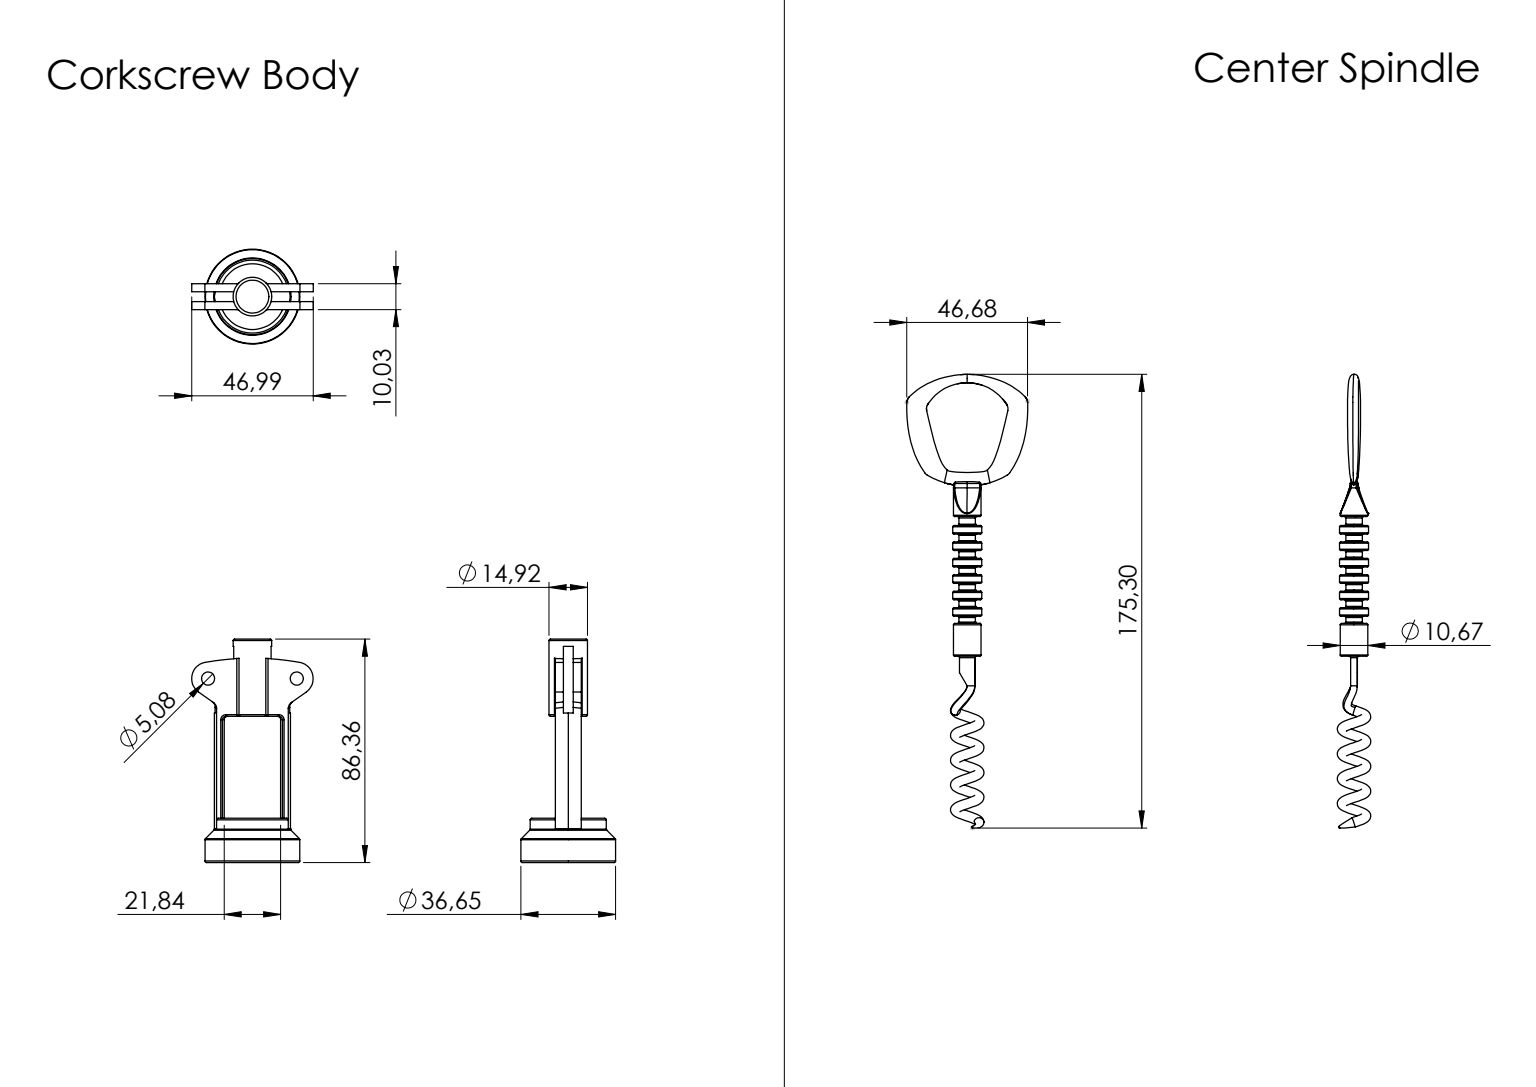
ISO-10303-21;
HEADER;
FILE_DESCRIPTION (('STEP AP214'),
    '1' );
FILE_NAME ('Center Spindle.step',
    '2026-10-06T14:27:08',
    ( '' ),
    ( '' ),
    'SwSTEP 2.0',
    'SolidWorks 2020',
    '' );
FILE_SCHEMA (( 'AUTOMOTIVE_DESIGN' ));
ENDSEC;

DATA;
#1=CARTESIAN_POINT ( 'NONE',  ( -2.902940568641317665, 107.8364052097302306, -4.470325690468441415 ) ) ;
#2=CARTESIAN_POINT ( 'NONE',  ( 4.750191988411978095, 117.8920247151937843, 0.9103219801276267731 ) ) ;
#3=CARTESIAN_POINT ( 'NONE',  ( 3.177488185987922709, -14.13217061847354472, 2.003775387181677026 ) ) ;
#4=CARTESIAN_POINT ( 'NONE',  ( -6.473539731754439863, 155.4519854478747902, -1.179574399179393440 ) ) ;
#5=CARTESIAN_POINT ( 'NONE',  ( -2.402553827781328089, 115.7029513687917017, -1.700315609833690900 ) ) ;
#6=CARTESIAN_POINT ( 'NONE',  ( -3.112628982284441737, 108.2625926757257844, 4.181986096990026880 ) ) ;
#8=CARTESIAN_POINT ( 'NONE',  ( 0.1065646865914872399, 105.8844662015456777, -5.332932678536313809 ) ) ;
#9=CARTESIAN_POINT ( 'NONE',  ( -8.921947645407078298, 154.9128698100208794, -1.713759150786742458 ) ) ;
#10=CARTESIAN_POINT ( 'NONE',  ( 15.73471677570929117, 120.8416612192442159, 0.3144170877234249706 ) ) ;
#11=CARTESIAN_POINT ( 'NONE',  ( -0.02969003158485089208, 157.1787724364823760, 1.485810588193620552 ) ) ;
#12=CARTESIAN_POINT ( 'NONE',  ( -2.946616183681363133, 115.7030909710271231, 1.559688585259455307 ) ) ;
#13=CARTESIAN_POINT ( 'NONE',  ( -5.328734912435950655, 121.3512789622145931, -0.03376412672994712899 ) ) ;
#14=CARTESIAN_POINT ( 'NONE',  ( 3.102408547967445696, -0.5812848888516047863, -3.453265078539196509 ) ) ;
#15=CARTESIAN_POINT ( 'NONE',  ( 22.61937536341548238, 150.3405807453409579, 1.175526429919688587 ) ) ;
#18=CARTESIAN_POINT ( 'NONE',  ( 3.256234316240316229, -15.49904601598017706, 3.966862439782909533 ) ) ;
#19=CARTESIAN_POINT ( 'NONE',  ( -19.06441997122223597, 145.0145856610025987, 1.755053680361626567 ) ) ;
#20=CARTESIAN_POINT ( 'NONE',  ( 0.9007433063219677516, 2.300345052497278608, 0.3717552062572989091 ) ) ;
#21=CARTESIAN_POINT ( 'NONE',  ( 0.003746264460233806812, 116.6481217037470373, -0.1874783927187336496 ) ) ;
#22=CARTESIAN_POINT ( 'NONE',  ( -0.8226642509504364931, 2.890957568680109446, -0.5268263738024351328 ) ) ;
#27=CARTESIAN_POINT ( 'NONE',  ( 4.040061035763102382, 117.6466181296975151, 0.9125624508345167030 ) ) ;
#29=CARTESIAN_POINT ( 'NONE',  ( -1.787077659700294863, 156.4219299504922844, 0.8362026816545217178 ) ) ;
#30=CARTESIAN_POINT ( 'NONE',  ( 3.821280252649200460, -11.76149679029331274, 0.6556923638117722053 ) ) ;
#31=CARTESIAN_POINT ( 'NONE',  ( 12.33128838443251674, 153.5964916033214820, -1.587645809864455471 ) ) ;
#32=CARTESIAN_POINT ( 'NONE',  ( -1.237267194679803950, 118.7146927282448132, -0.6928808259403732572 ) ) ;
#33=CARTESIAN_POINT ( 'NONE',  ( -5.946078212987909062, 28.42590610009758123, 0.3016625663984517924 ) ) ;
#34=CARTESIAN_POINT ( 'NONE',  ( 2.671714809844681238, -14.97371442308345380, 4.574436322856921144 ) ) ;
#35=CARTESIAN_POINT ( 'NONE',  ( -2.623680569203113766, 34.84621527371866989, 1.140749429358363987 ) ) ;
#36=CARTESIAN_POINT ( 'NONE',  ( 14.28939804845276740, 138.9852717218771261, -0.04639197223238045870 ) ) ;
#37=ORIENTED_EDGE ( 'NONE', *, *, #18826, .T. ) ;
#42=CARTESIAN_POINT ( 'NONE',  ( 15.65715779584547462, 120.8241032224722176, 0.2083191676592779373 ) ) ;
#43=CARTESIAN_POINT ( 'NONE',  ( -6.321818188556177276, 120.0717973201777511, 0.2011600071967686865 ) ) ;
#45=CARTESIAN_POINT ( 'NONE',  ( -1.563156853714933625, 118.1287640443500351, 0.8777957133630984732 ) ) ;
#47=CARTESIAN_POINT ( 'NONE',  ( -0.1480340175562135652, 37.01381769933495747, -0.7398847138023396663 ) ) ;
#48=CARTESIAN_POINT ( 'NONE',  ( 20.93418857319365500, 149.0309112320384486, 2.352213276463849034 ) ) ;
#49=CARTESIAN_POINT ( 'NONE',  ( -2.673854242087471356, 19.56896771519852862, 3.769861741755948348 ) ) ;
#50=CARTESIAN_POINT ( 'NONE',  ( -8.093932337251422027, 31.18171294578705854, -2.467657647566553258 ) ) ;
#51=CARTESIAN_POINT ( 'NONE',  ( -2.171567613555696941, 116.7785827647842751, -0.5120155132742859605 ) ) ;
#52=CARTESIAN_POINT ( 'NONE',  ( -2.327868625978157358, 124.9344662015457175, -0.04651635516647353863 ) ) ;
#55=CARTESIAN_POINT ( 'NONE',  ( 3.195898997675873598, 105.1238757837674314, 4.272339236703191823 ) ) ;
#56=CARTESIAN_POINT ( 'NONE',  ( 4.419457123578296454, 17.78516144714274105, -1.360477052881604143 ) ) ;
#59=CARTESIAN_POINT ( 'NONE',  ( 2.461817612451524084, -15.00653475910608492, 4.866425834902347702 ) ) ;
#60=CARTESIAN_POINT ( 'NONE',  ( 1.642663419667585778, 119.5945091202099348, -0.5769171603192788655 ) ) ;
#61=CARTESIAN_POINT ( 'NONE',  ( -19.82178279981189206, 128.7876384977266468, 0.3398896782655025928 ) ) ;
#62=ORIENTED_EDGE ( 'NONE', *, *, #26845, .T. ) ;
#66=DIRECTION ( 'NONE',  ( -4.017660918040594346E-17, 1.000000000000000000, 2.376309959284834438E-19 ) ) ;
#67=CARTESIAN_POINT ( 'NONE',  ( 6.083905389560601229, -14.65912421694762280, 0.09720023197589457153 ) ) ;
#68=CARTESIAN_POINT ( 'NONE',  ( -10.16662615958544258, 120.4647147465577461, 1.171017801134732306 ) ) ;
#70=CARTESIAN_POINT ( 'NONE',  ( 8.033985789952966527, 118.2752802814886053, -0.7207832311977435680 ) ) ;
#71=CARTESIAN_POINT ( 'NONE',  ( -0.9211762648548540433, 10.43857344512876040, -4.529598961101950927 ) ) ;
#74=EDGE_LOOP ( 'NONE', ( #32492, #14883, #24594, #27507 ) ) ;
#76=CARTESIAN_POINT ( 'NONE',  ( 0.4140400251255503261, 124.3520329708341023, 0.07144784443200485891 ) ) ;
#77=B_SPLINE_SURFACE_WITH_KNOTS ( 'NONE', 3, 3, ( 
 ( #14540, #40555, #8162, #21131, #40760, #17945, #30947, #37549, #8372, #19416, #22802, #3464, #6441, #12415, #15798, #3049, #32000, #22177, #35627, #273, #26019, #36045, #39028, #2839, #28807, #25407, #22595, #41823, #16428, #16007, #12820, #12617, #29006, #29432, #18996 ),
 ( #19831, #22385, #25604, #6860, #6034, #10045, #59, #38612, #9418, #35839, #19618, #35410, #16212, #32422, #23017, #6238, #6654, #19208, #2632, #3252, #41605, #32631, #32216, #38814, #42023, #29216, #13247, #25808, #13027, #9628, #26231, #38409, #9220, #39235, #9836 ),
 ( #15591, #28596, #35208, #26870, #26447, #30479, #39450, #29856, #33061, #694, #17063, #40089, #23872, #20042, #16640, #10253, #37096, #7710, #36677, #36467, #7498, #36892, #10469, #3892, #23226, #24086, #36258, #17280, #4316, #20458, #33274, #39878, #16856, #33487, #486 ),
 ( #4103, #13666, #30066, #7286, #903, #7914, #13877, #26658, #32846, #23438, #29648, #27081, #30269, #10884, #33696, #1110, #13459, #39665, #10675, #20248, #7079, #23657, #1323, #14078, #3676, #20672, #4520, #17482, #14280, #27290, #40305, #11098, #21294, #31110, #4939 ),
 ( #27704, #34322, #1947, #34530, #27909, #30900, #11305, #40711, #21497, #37923, #37498, #30685, #33904, #41344, #41127, #8113, #17898, #18520, #8746, #5150, #11507, #24493, #21088, #14906, #34732, #40916, #21708, #12146, #2370, #8323, #18105, #31311, #15115, #5356, #8537 ),
 ( #5563, #1740, #11722, #24709, #1535, #37714, #25138, #24925, #18309, #31526, #14490, #27503, #4733, #2155, #28118, #11933, #15328, #28335, #38142, #20879, #17685, #40511, #24290, #37295, #34112, #14699, #592, #26769, #26338, #33171, #13564, #29110, #29753, #3999, #6755 ),
 ( #10149, #19309, #22701, #16957, #32313, #6542, #9939, #19943, #29326, #23119, #22910, #25915, #35943, #35731, #35517, #19517, #6972, #20148, #10365, #3143, #38923, #29956, #26554, #23336, #13348, #16106, #32525, #19724, #9733, #42128, #382, #7189, #32962, #796, #3788 ),
 ( #32743, #170, #39344, #3356, #13140, #39560, #36155, #13772, #36373, #16323, #3576, #16537, #16748, #29548, #26132, #12924, #39133, #9522, #22489, #6338, #7389, #10573, #17998, #17787, #26978, #36783, #37396, #27595, #40197, #4423, #1220, #39988, #20775, #11404, #7813 ),
 ( #10779, #1425, #40604, #10992, #37191, #30371, #21185, #33374, #36573, #24391, #23760, #4627, #27183, #20350, #14382, #30996, #1636, #30586, #8213, #4206, #17170, #23552, #27391, #40402, #8013, #20984, #5043, #23974, #34005, #34214, #17582, #36992, #17381, #30169, #14179 ),
 ( #11196, #1837, #30786, #1010, #14590, #14801, #33799, #24182, #4835, #13974, #39779, #7599, #20561, #33590, #28228, #28442, #31422, #28011, #12468, #41234, #38459, #34415, #31637, #9277, #11830, #18415, #12037, #2687, #18203, #25028, #2264, #38031, #32055, #8851, #41020 ),
 ( #12253, #15228, #2893, #15439, #5675, #21815, #18633, #34841, #41448, #25246, #2047, #2478, #38249, #21389, #25463, #5248, #24817, #37812, #8637, #9066, #35060, #18843, #15012, #11613, #31204, #27804, #15644, #22032, #5881, #31847, #28649, #5455, #21600, #34628, #19050 ),
 ( #41660, #22235, #35263, #6087, #40812, #24597, #37604, #8431, #10316, #38669, #12878, #16274, #26288, #35685, #29494, #29278, #32271, #123, #29064, #41874, #42084, #13301, #26506, #16697, #25662, #3101, #39511, #20097, #32908, #6494, #335, #7140, #22651, #39296, #19472 ),
 ( #36109, #29702, #19678, #9476, #25867, #13087, #16062, #35469, #6710, #13517, #10103, #33121, #23075, #38873, #9685, #22440, #35899, #32479, #543, #26079, #39087, #3308, #9889, #23285, #22862, #36322, #32694, #15855, #3528, #16488, #28862, #19263, #12673, #6923, #19893 ),
 ( #6292, #3739, #33328, #961, #1591, #33962, #4373, #10730, #7553, #4158, #27134, #17742, #14132, #20937, #24347, #27557, #23711, #36730, #14335, #40357, #30538, #33541, #40147, #39727, #14548, #10526, #13930, #17120, #26925, #30324, #11152, #37147, #30121, #29912, #23496 ),
 ( #23929, #17333, #20513, #36523, #1168, #7969, #21140, #20729, #40564, #4791, #7342, #24139, #11362, #10940, #36944, #7765, #13725, #33753, #4579, #17537, #39938, #1377, #27345, #30742, #37354, #8172, #3950, #16911, #20301, #751, #26719, #18160, #24770, #5413, #9020 ),
 ( #2640, #38416, #21983, #11780, #5627, #25415, #40977, #18585, #37768, #9228, #8592, #18790, #18368, #21556, #5836, #17954, #28603, #12423, #31803, #27758, #1795, #25198, #31375, #34584, #40769, #2219, #15178, #21767, #14966, #28182, #12209, #24985, #34169, #35016, #41187 ),
 ( #31593, #11990, #2004, #24552, #37984, #34794, #15600, #8809, #14758, #4996, #30955, #38203, #21346, #31163, #41613, #11567, #2430, #15391, #28397, #34372, #41402, #37557, #8382, #5205, #27968, #3687, #42033, #12828, #32640, #16435, #6662, #9843, #67, #32429, #13037 ),
 ( #9635, #2847, #26027, #6246, #22810, #32007, #35418, #16648, #15807, #19215, #22603, #3473, #25816, #35848, #35635, #38622, #6449, #32225, #6042, #3057, #19625, #32855, #23025, #28815, #9425, #29655, #26456, #39245, #38824, #29442, #13467, #29013, #281, #19423, #39460 ),
 ( #36055, #39036, #41830, #16014, #3260, #22395, #12624, #13254, #19841, #26238, #22186, #10054, #16220, #29226, #25612, #6868, #495, #35216, #19004, #20465, #36474, #10683, #37103, #26666, #11104, #7506, #27510, #30074, #33282, #1541, #13675, #17692, #7717, #39674, #10477 ),
 ( #30486, #23446, #7294, #7921, #40311, #23664, #17071, #13885, #20255, #33494, #24093, #4324, #27296, #30691, #33911, #911, #26878, #20681, #4526, #36898, #40096, #30277, #17288, #1118, #14087, #23879, #10892, #4111, #39886, #27088, #3901, #20887, #16864, #36684, #33705 ),
 ( #17490, #1329, #14287, #14496, #4739, #10261, #23234, #36269, #7089, #20051, #29864, #33070, #704, #15553, #15125, #21933, #31536, #17905, #18531, #34962, #37723, #34742, #28128, #2380, #41354, #2166, #8120, #11515, #40924, #27711, #30909, #31322, #38152, #21718, #31750 ),
 ( #40720, #21094, #18320, #24500, #12156, #11730, #8547, #37505, #24719, #25148, #14706, #8965, #21506, #40518, #18112, #21301, #2593, #1747, #5785, #37933, #8331, #34330, #15340, #28345, #5158, #11944, #41138, #18740, #31117, #11310, #1954, #24297, #24935, #37303, #34118 ),
 ( #4945, #14914, #27918, #34539, #8756, #5573, #5365, #16167, #6400, #38774, #19370, #9585, #18, #29172, #2799, #15964, #22554, #22135, #26189, #35164, #25562, #28761, #38566, #12777, #35794, #19577, #15756, #12371, #5991, #32804, #3418, #32376, #32169, #3205, #32585 ),
 ( #18954, #19785, #31960, #12984, #25977, #38985, #28962, #35584, #12575, #9794, #38364, #41775, #22973, #9178, #9379, #41978, #22761, #6196, #6606, #25767, #22343, #16385, #35366, #25359, #19165, #29390, #39193, #230, #3005, #13206, #10001, #3635, #36003, #6815, #28555 ),
 ( #41563, #13413, #26831, #7457, #39838, #30229, #4270, #33021, #4062, #10635, #10210, #14240, #23180, #13623, #16814, #26614, #860, #23827, #7666, #3850, #443, #36215, #20836, #33654, #20414, #20207, #33443, #20624, #36429, #29816, #7036, #7874, #20003, #1068, #14036 ),
 ( #13833, #33234, #23614, #26402, #17233, #23397, #17021, #39621, #30020, #27040, #36635, #655, #1282, #40049, #27246, #10427, #10842, #40262, #7248, #36847, #4479, #17439, #30436, #11056, #24041, #37056, #33860, #16599, #29608, #39407, #24452, #1490, #41086, #21453, #24883 ),
 ( #8280, #18477, #30647, #41299, #25092, #31482, #40470, #14447, #37880, #31064, #21250, #11261, #18061, #37456, #34483, #27659, #34280, #8703, #37673, #8912, #5519, #11462, #5109, #14865, #18266, #11677, #14655, #37255, #1902, #5315, #21666, #27868, #27457, #17645, #38097 ),
 ( #31269, #2111, #12103, #34072, #34690, #21047, #21878, #15075, #24247, #2327, #40876, #24664, #4899, #8496, #15287, #28075, #11894, #28292, #4689, #8073, #17854, #30855, #1700, #40670, #12937, #29341, #32120, #38515, #15914, #2541, #22503, #41718, #35320, #2749, #6147 ) ),
 .UNSPECIFIED., .T., .F., .F.,
 ( 4, 2, 2, 2, 1, 2, 2, 2, 2, 2, 2, 1, 2, 2, 4 ),
 ( 4, 1, 1, 1, 1, 1, 1, 1, 1, 1, 1, 1, 1, 1, 1, 1, 1, 1, 1, 1, 1, 1, 1, 1, 1, 1, 1, 1, 1, 1, 1, 1, 4 ),
 ( 0.000000000000000000, 0.06249999999999900080, 0.1249999999999978906, 0.2499999999999956701, 0.2812499999999951150, 0.3749999999999934497, 0.4374999999999933387, 0.5000000000000000000, 0.5624999999999930056, 0.6249999999999928946, 0.7500000000000000000, 0.7812499999999951150, 0.8749999999999963363, 0.9374999999999982236, 1.000000000000000000 ),
 ( 0.000000000000000000, 0.02711375962671787321, 0.05385523109991235263, 0.08027126036152537614, 0.1064096946071439176, 0.1323192412471900226, 0.1580495177521483718, 0.1882118685537063907, 0.2182788543618764954, 0.2483346178351386324, 0.2784631806910429774, 0.3054937156393619513, 0.3327069032348308197, 0.3601597580799023035, 0.3879077415152338837, 0.4160045136367338525, 0.4445017332217630623, 0.4734489055539064517, 0.5028932750457014711, 0.5328797594123376724, 0.5634509204570880003, 0.5946469669818265080, 0.6265057848166851739, 0.6590629893014032792, 0.6923519956652609553, 0.7264041031822485728, 0.7612485893105871426, 0.7986318966073006065, 0.8369441774603861850, 0.8762126957585177900, 0.9164627945539034481, 0.9577180065289634392, 1.000000000000000000 ),
 .UNSPECIFIED. ) ;
#78=CARTESIAN_POINT ( 'NONE',  ( -11.07124803888946296, 123.5714170083676748, 1.086458317614992231 ) ) ;
#80=CARTESIAN_POINT ( 'NONE',  ( 14.75721126660338811, 152.8628051715174365, -1.735400109512246880 ) ) ;
#82=CARTESIAN_POINT ( 'NONE',  ( -13.57054970571782704, 121.9345505566020194, -1.704910367088877221 ) ) ;
#85=CARTESIAN_POINT ( 'NONE',  ( 4.532197386373657544, 118.1209942587670980, -0.4791226501333581411 ) ) ;
#87=CARTESIAN_POINT ( 'NONE',  ( 16.10174665100975488, 146.3760696504137684, -0.5323012926561621061 ) ) ;
#89=CARTESIAN_POINT ( 'NONE',  ( -17.42038752474488561, 148.2779598588913643, -2.227836471057101697 ) ) ;
#90=CARTESIAN_POINT ( 'NONE',  ( 3.162278034637682200, -15.50568859125470134, 4.121945908858189789 ) ) ;
#91=CARTESIAN_POINT ( 'NONE',  ( -3.552207995971087051, 105.1233060067599610, -3.981573230609858793 ) ) ;
#93=B_SPLINE_CURVE_WITH_KNOTS ( 'NONE', 3,
 ( #362, #13328, #570, #10344 ),
 .UNSPECIFIED., .F., .F.,
 ( 4, 4 ),
 ( 0.5010344700412979746, 1.000000000000000000 ),
 .UNSPECIFIED. ) ;
#94=CARTESIAN_POINT ( 'NONE',  ( -4.827457070893626856, 117.7658616683732618, 0.8357213340295019943 ) ) ;
#95=CARTESIAN_POINT ( 'NONE',  ( 7.266810130343707819, 121.1388872696715282, 1.097806971394259312 ) ) ;
#97=AXIS2_PLACEMENT_3D ( 'NONE', #15136, #24944, #28139 ) ;
#98=CARTESIAN_POINT ( 'NONE',  ( 1.523114390242035210, -9.429190846093893796, -8.291516064885865234 ) ) ;
#99=CARTESIAN_POINT ( 'NONE',  ( 4.578033532675482853, 121.1907927009877000, 0.1597499619731680698 ) ) ;
#105=CARTESIAN_POINT ( 'NONE',  ( -2.180832807216472435, 116.2031176879599599, -0.1302529176791268339 ) ) ;
#106=CARTESIAN_POINT ( 'NONE',  ( 13.43845804798103316, 156.9141898299356512, 0.2685323735513602261 ) ) ;
#110=CARTESIAN_POINT ( 'NONE',  ( 5.078986093043053707, 79.34146620154574236, 0.1014902294541244060 ) ) ;
#113=CYLINDRICAL_SURFACE ( 'NONE', #28014, 3.175000000000001155 ) ;
#116=CARTESIAN_POINT ( 'NONE',  ( -23.30518390908433091, 149.0397177335360652, -0.1341373440727923194 ) ) ;
#119=CARTESIAN_POINT ( 'NONE',  ( 6.067968699521611775, 121.4399612899160843, 0.1149339127001053201 ) ) ;
#121=CARTESIAN_POINT ( 'NONE',  ( 4.588798433226582318, 115.7029491485453150, -1.333296534009075662 ) ) ;
#122=CARTESIAN_POINT ( 'NONE',  ( -5.931002064882670233, 121.5392726388429168, -0.1896088198168328631 ) ) ;
#123=CARTESIAN_POINT ( 'NONE',  ( 4.852936394019410571, -14.31369683153947747, 4.236952399839363892 ) ) ;
#124=CARTESIAN_POINT ( 'NONE',  ( -13.60293432442229999, 121.5020190402118203, 1.066732574264078748 ) ) ;
#126=CARTESIAN_POINT ( 'NONE',  ( 16.12231377365572982, 121.3783152868344075, 0.5570369914769761621 ) ) ;
#127=CARTESIAN_POINT ( 'NONE',  ( 9.090272512956175888, 124.2201288364615266, 0.2714231486187235198 ) ) ;
#129=CARTESIAN_POINT ( 'NONE',  ( 0.7643174330569572072, 9.588751494893990923, -0.6113830025413525826 ) ) ;
#130=CARTESIAN_POINT ( 'NONE',  ( -13.61156529719784558, 119.6358206793323404, -0.4233406866235920885 ) ) ;
#131=DIRECTION ( 'NONE',  ( -5.206863593109713661E-17, 1.000000000000000000, -1.077750396879097183E-30 ) ) ;
#132=DIRECTION ( 'NONE',  ( -0.1538570343431813203, -0.9876883405951371042, -0.02827993697916746443 ) ) ;
#133=CARTESIAN_POINT ( 'NONE',  ( 8.672122787176258285, 118.2242029276344510, 0.9375713879804109530 ) ) ;
#134=ORIENTED_EDGE ( 'NONE', *, *, #31655, .T. ) ;
#136=CARTESIAN_POINT ( 'NONE',  ( 14.23594795111937295, 121.8555783441548073, 1.592150851459066319 ) ) ;
#137=CARTESIAN_POINT ( 'NONE',  ( 19.51325853822217127, 141.0981142166620259, -1.725252114789138203 ) ) ;
#138=CARTESIAN_POINT ( 'NONE',  ( -0.1482875670852983607, 5.528424516503947395, -0.9633795868741713564 ) ) ;
#139=CARTESIAN_POINT ( 'NONE',  ( -0.4581589521676752153, 10.92003791307801208, 8.418874016967684781 ) ) ;
#141=CARTESIAN_POINT ( 'NONE',  ( -12.23848595143957141, 156.6574886424908470, -1.779988832801368437 ) ) ;
#142=CARTESIAN_POINT ( 'NONE',  ( 4.767275108742798473, 117.8956358391749717, -0.7413279629693602102 ) ) ;
#144=CARTESIAN_POINT ( 'NONE',  ( 9.138499898145592937, 117.7878261280527425, 0.1826089763859914672 ) ) ;
#145=CARTESIAN_POINT ( 'NONE',  ( 4.403754988258198111, 120.5100497556178567, -0.5130326506441984513 ) ) ;
#146=CARTESIAN_POINT ( 'NONE',  ( -11.83770080265077951, 152.0103986367769551, -0.1887002032782128802 ) ) ;
#148=CARTESIAN_POINT ( 'NONE',  ( -16.28588378367234313, 151.0861551944122141, -2.361334407247334788 ) ) ;
#149=CARTESIAN_POINT ( 'NONE',  ( 5.396943489592968213, -15.24705710738187570, 2.503009974473451749 ) ) ;
#150=CARTESIAN_POINT ( 'NONE',  ( 4.782580095254411745, 118.5931160184169073, 0.9661571381561826488 ) ) ;
#153=CARTESIAN_POINT ( 'NONE',  ( 4.244755607818279763, 119.7015364213435333, 0.9259100998607280308 ) ) ;
#154=DIRECTION ( 'NONE',  ( -0.9998004120163609398, 0.000000000000000000, -0.01997839162482749689 ) ) ;
#157=CARTESIAN_POINT ( 'NONE',  ( -5.575611629172074757, 123.3023672762779910, -0.03632235649590531690 ) ) ;
#158=CARTESIAN_POINT ( 'NONE',  ( 7.184910528696541121, -14.53812136005497280, -4.413989948622978332 ) ) ;
#159=CARTESIAN_POINT ( 'NONE',  ( 9.525206088249063896, 124.2661852542617709, 0.6183897905712308907 ) ) ;
#160=CARTESIAN_POINT ( 'NONE',  ( 4.852593915752285270, 117.2114307359545649, -0.4396237197203589631 ) ) ;
#161=CARTESIAN_POINT ( 'NONE',  ( -4.854186777038641765, 117.7557277303023966, -0.9091791526384296329 ) ) ;
#164=ADVANCED_FACE ( 'NONE', ( #34633 ), #16332, .T. ) ;
#165=CARTESIAN_POINT ( 'NONE',  ( -15.96050253218469983, 121.0385544001969436, -0.3018840724360822847 ) ) ;
#167=CARTESIAN_POINT ( 'NONE',  ( 8.259156552716179434, 120.4369397177006960, -1.103309705185253842 ) ) ;
#168=CARTESIAN_POINT ( 'NONE',  ( 23.29144772315967771, 149.3526176766912101, 0.4654185560736371352 ) ) ;
#169=CARTESIAN_POINT ( 'NONE',  ( -9.418980095613695980, 123.9587481073520223, -0.7032982658115916053 ) ) ;
#170=CARTESIAN_POINT ( 'NONE',  ( 2.004955844419833877, -15.09631637516548075, 5.820374350103214134 ) ) ;
#172=CARTESIAN_POINT ( 'NONE',  ( 20.51686376604209983, 129.1072961674477710, 0.4099757654675942331 ) ) ;
#173=ORIENTED_EDGE ( 'NONE', *, *, #9182, .T. ) ;
#174=CARTESIAN_POINT ( 'NONE',  ( -0.9211762648548540433, 10.43857344512876040, -4.529598961101950927 ) ) ;
#175=CARTESIAN_POINT ( 'NONE',  ( -8.216926545874587262, 117.5004104479096583, -0.1641937475849288286 ) ) ;
#176=CARTESIAN_POINT ( 'NONE',  ( -16.86202032626315628, 155.2029898760372646, -0.3369432954968343275 ) ) ;
#178=CARTESIAN_POINT ( 'NONE',  ( -6.120715547033301007, 121.1078720221529466, 0.4856508595550485530 ) ) ;
#180=CARTESIAN_POINT ( 'NONE',  ( 3.087053954869741101, 14.59627045569285286, -3.440871586639639990 ) ) ;
#181=CARTESIAN_POINT ( 'NONE',  ( 21.46783008853678609, 136.6907720476960435, 1.692068800591147282 ) ) ;
#182=CARTESIAN_POINT ( 'NONE',  ( -0.08519874065850288614, 108.5751225745497948, 4.263693374914160117 ) ) ;
#184=CARTESIAN_POINT ( 'NONE',  ( 2.800559387825661606, 158.6924860557018064, -1.442603686385967032 ) ) ;
#185=CARTESIAN_POINT ( 'NONE',  ( 4.506137822554599381, 3.376467715207942533, 1.027655576270160243 ) ) ;
#186=CARTESIAN_POINT ( 'NONE',  ( -14.63850908477053991, 156.0817623197167450, -1.342817726712510318 ) ) ;
#188=CARTESIAN_POINT ( 'NONE',  ( -15.46148294186166439, 147.8441550597069352, 0.1409636975754419985 ) ) ;
#189=CARTESIAN_POINT ( 'NONE',  ( 3.228727248129140026, -15.23899909574484646, 5.612614099740361517 ) ) ;
#190=CARTESIAN_POINT ( 'NONE',  ( -6.615214180512292604E-14, 94.32746620154571815, -2.829521569843129660E-18 ) ) ;
#191=CARTESIAN_POINT ( 'NONE',  ( 2.969447359227861405, -13.80100253337253946, 0.9847735008004718793 ) ) ;
#193=CARTESIAN_POINT ( 'NONE',  ( 2.329084838958874748, 118.9063233352275972, 0.7992829875212342783 ) ) ;
#196=CARTESIAN_POINT ( 'NONE',  ( -22.74464968533201414, 149.4207734315791072, 0.6238039466385616461 ) ) ;
#197=CARTESIAN_POINT ( 'NONE',  ( 23.16228472148464235, 149.2833505036244048, -0.1324855245534189985 ) ) ;
#202=CARTESIAN_POINT ( 'NONE',  ( 2.109804961112711652, -15.28918944155240034, 5.362628413980365494 ) ) ;
#203=ADVANCED_FACE ( 'NONE', ( #18208 ), #14201, .F. ) ;
#205=DIRECTION ( 'NONE',  ( -5.206863593109713661E-17, 1.000000000000000000, -1.077750396879097183E-30 ) ) ;
#206=CARTESIAN_POINT ( 'NONE',  ( -4.535815920756029129, 118.0878757016629521, 0.6031417657034798818 ) ) ;
#209=ORIENTED_EDGE ( 'NONE', *, *, #20675, .T. ) ;
#210=CARTESIAN_POINT ( 'NONE',  ( -0.3650308193387738487, 118.7629491485454025, -1.279690690685891807 ) ) ;
#211=CARTESIAN_POINT ( 'NONE',  ( 6.034264073414651541, 119.2911550975486676, -1.026770045858946823 ) ) ;
#212=CARTESIAN_POINT ( 'NONE',  ( -3.903247448917784190, 109.8183322527596602, -3.677532532511333052 ) ) ;
#213=CARTESIAN_POINT ( 'NONE',  ( 4.607970095737445426, 117.9806936862427449, 0.9111728063042895398 ) ) ;
#215=CARTESIAN_POINT ( 'NONE',  ( -10.17133788503933900, 124.0743415861677903, -1.120692231141950934 ) ) ;
#217=CARTESIAN_POINT ( 'NONE',  ( -2.225528185412928295, 115.7029491485453576, -1.707866438218498040 ) ) ;
#218=CARTESIAN_POINT ( 'NONE',  ( -2.874359970738451509, 107.8415691140158543, 4.365465615796717103 ) ) ;
#219=CARTESIAN_POINT ( 'NONE',  ( -4.791894246051028539, 117.8359990171110780, -0.9363294005345770277 ) ) ;
#220=CARTESIAN_POINT ( 'NONE',  ( 5.257173101725930664, 116.1034411669277375, -1.028648520082846352 ) ) ;
#221=CARTESIAN_POINT ( 'NONE',  ( -10.56433624517455705, 123.7931190674884050, -1.348085882050163331 ) ) ;
#223=CARTESIAN_POINT ( 'NONE',  ( -0.01596947694136538129, 156.4635559983122448, 0.7991779281049289363 ) ) ;
#224=CARTESIAN_POINT ( 'NONE',  ( -2.827941042956166662, 115.7033332087140138, 1.571145331901102171 ) ) ;
#225=CARTESIAN_POINT ( 'NONE',  ( -15.78496548096122076, 146.2362003282640615, -0.2482417383768280028 ) ) ;
#226=CARTESIAN_POINT ( 'NONE',  ( 1.360477052538118681, -3.804838552850991817, 4.419457122809256511 ) ) ;
#227=CARTESIAN_POINT ( 'NONE',  ( 23.03149411880787767, 148.7220611141358404, 1.316198435982438797 ) ) ;
#230=CARTESIAN_POINT ( 'NONE',  ( 3.491209331645790837, -14.97137451562302601, 1.144833103274278230 ) ) ;
#231=CARTESIAN_POINT ( 'NONE',  ( -8.255438862926547827, 156.5149677146980309, 1.736665298733278906 ) ) ;
#232=CARTESIAN_POINT ( 'NONE',  ( 0.5639076275445228381, 13.94848098472073161, -0.7944722417661187475 ) ) ;
#233=CARTESIAN_POINT ( 'NONE',  ( -21.68922513019262510, 151.4054434770023363, -1.149106048033103011 ) ) ;
#235=CARTESIAN_POINT ( 'NONE',  ( 0.6857505489063979720, -9.425274534614802135, -0.6942005185601292094 ) ) ;
#236=ORIENTED_EDGE ( 'NONE', *, *, #38437, .F. ) ;
#238=CARTESIAN_POINT ( 'NONE',  ( 7.588497335288401757, 124.2943531750336490, 0.1606663149101728583 ) ) ;
#240=CARTESIAN_POINT ( 'NONE',  ( -11.01086703061210414, 126.1652090859982707, 0.5547642914263289926 ) ) ;
#241=CARTESIAN_POINT ( 'NONE',  ( 2.933303798676236696, -14.66982100897798524, 5.370674165220748364 ) ) ;
#242=CARTESIAN_POINT ( 'NONE',  ( 4.329049305160035388, 120.0471566133196291, -0.6733469523851639549 ) ) ;
#243=CARTESIAN_POINT ( 'NONE',  ( -16.05419991788312473, 128.5601350900737998, -2.191829208737125612 ) ) ;
#245=CARTESIAN_POINT ( 'NONE',  ( 2.663950356258127705, -13.19741034273377878, 0.1528337951401303463 ) ) ;
#246=CARTESIAN_POINT ( 'NONE',  ( -5.943370056925232348, 31.21256582444267380, 0.1301312493255015745 ) ) ;
#247=CARTESIAN_POINT ( 'NONE',  ( 11.97065782032992587, 130.4318746828361100, 0.03484989721007641927 ) ) ;
#249=CARTESIAN_POINT ( 'NONE',  ( -4.780654621982846741, 111.8765634536314906, 2.439804913899639605 ) ) ;
#251=CIRCLE ( 'NONE', #36280, 5.588000000000006295 ) ;
#254=AXIS2_PLACEMENT_3D ( 'NONE', #10805, #1032, #33194 ) ;
#255=CARTESIAN_POINT ( 'NONE',  ( 3.297133786507668418, 159.4684106755469202, 0.01890815954692008985 ) ) ;
#256=CARTESIAN_POINT ( 'NONE',  ( -6.540839804427584170, 120.6338824379019172, 0.1347920106280767472 ) ) ;
#258=CARTESIAN_POINT ( 'NONE',  ( -1.044188858242598439, 115.6909491485452435, 1.710615210114453166 ) ) ;
#259=CARTESIAN_POINT ( 'NONE',  ( 4.529186081025091681, -11.15152372915077095, -0.9203776863585164669 ) ) ;
#260=CARTESIAN_POINT ( 'NONE',  ( -2.340953058884871485, 34.37024003021338103, 0.7097582906893736832 ) ) ;
#262=CARTESIAN_POINT ( 'NONE',  ( 14.62144676724393300, 123.3142630313093377, 1.799443978378394648 ) ) ;
#263=CARTESIAN_POINT ( 'NONE',  ( -2.394960105286914942, 16.54535949628658997, -3.951836011466995036 ) ) ;
#264=CARTESIAN_POINT ( 'NONE',  ( -4.020893062959163267, -8.947226795047690473, 7.425401991387179379 ) ) ;
#265=CARTESIAN_POINT ( 'NONE',  ( -5.483673445576510375, 117.2147343480241091, -0.8092650553969497063 ) ) ;
#266=CARTESIAN_POINT ( 'NONE',  ( -0.8420595575569044255, 109.5507526474568607, -3.867914470699519658 ) ) ;
#269=CARTESIAN_POINT ( 'NONE',  ( -2.880622083164609215, 104.6144662015456959, 4.502939351893831876 ) ) ;
#270=CARTESIAN_POINT ( 'NONE',  ( 3.979181138743986601, 26.09377549647152961, 2.406711837290479661 ) ) ;
#271=CARTESIAN_POINT ( 'NONE',  ( 2.081416901521091933, -15.50639809317535089, 5.943648939154567934 ) ) ;
#273=CARTESIAN_POINT ( 'NONE',  ( 3.216700609619024931, -14.42020774479446921, 2.887214088933996337 ) ) ;
#274=CARTESIAN_POINT ( 'NONE',  ( 2.327868625978029016, 124.9344662015457175, 0.04651635516647314311 ) ) ;
#275=CARTESIAN_POINT ( 'NONE',  ( -14.42641459765142820, 120.3907653763288579, 0.3011401359519875198 ) ) ;
#276=VERTEX_POINT ( 'NONE', #11409 ) ;
#278=ORIENTED_EDGE ( 'NONE', *, *, #32111, .F. ) ;
#279=CARTESIAN_POINT ( 'NONE',  ( -5.174735437441460917, 115.7029491485453576, 1.071059064073374589 ) ) ;
#280=AXIS2_PLACEMENT_3D ( 'NONE', #23824, #4267, #36844 ) ;
#281=CARTESIAN_POINT ( 'NONE',  ( 5.898825546834660649, -14.84738759216856785, 0.02597052417917125600 ) ) ;
#282=CARTESIAN_POINT ( 'NONE',  ( -13.14453721617490523, 122.4605402651681487, 1.292199650740640138 ) ) ;
#283=CARTESIAN_POINT ( 'NONE',  ( 9.329873057606279829, 118.8811571165754941, -0.8296725728930305355 ) ) ;
#284=CARTESIAN_POINT ( 'NONE',  ( -4.627450822138572839, 2.892058097378844117, -0.1328416527703782657 ) ) ;
#288=CARTESIAN_POINT ( 'NONE',  ( 0.2094794444022589075, 111.5577547982948801, 3.149697633913104866 ) ) ;
#289=CARTESIAN_POINT ( 'NONE',  ( -4.765692302950382597, 117.6625622553268471, 0.9423543906840938789 ) ) ;
#290=CARTESIAN_POINT ( 'NONE',  ( -17.01014995307831867, 147.0740084267719396, 1.247012517048586844 ) ) ;
#291=CARTESIAN_POINT ( 'NONE',  ( 5.111850311340921493, 116.9863990472329931, 0.4425446553583142206 ) ) ;
#292=CARTESIAN_POINT ( 'NONE',  ( 5.080524353911745727, 119.7208665877771665, -0.8394179162009564044 ) ) ;
#293=CARTESIAN_POINT ( 'NONE',  ( 0.02969037535068572500, 158.7301711276701894, -1.485827791648137053 ) ) ;
#297=CARTESIAN_POINT ( 'NONE',  ( 4.483427315476480324, 118.1297255826064401, -0.5360345877169139239 ) ) ;
#298=CARTESIAN_POINT ( 'NONE',  ( 9.732488649496215061, 124.0009531390599591, -0.4956537337270181531 ) ) ;
#300=CARTESIAN_POINT ( 'NONE',  ( -1.368713796474945177, 119.6596719632383383, -0.6021288208518275065 ) ) ;
#301=CARTESIAN_POINT ( 'NONE',  ( 3.819321967970790599, -15.20641387874817418, 0.06971680219106241028 ) ) ;
#303=AXIS2_PLACEMENT_3D ( 'NONE', #10017, #38788, #25577 ) ;
#304=CARTESIAN_POINT ( 'NONE',  ( -4.782196433634765320, 105.1214876792004560, -2.388545300328469345 ) ) ;
#307=CARTESIAN_POINT ( 'NONE',  ( -4.980589814694351247, 117.5315369307823801, 0.7737963060445882668 ) ) ;
#308=CARTESIAN_POINT ( 'NONE',  ( 17.04317705290379692, 148.4623951536435698, 2.145728921095965358 ) ) ;
#309=CARTESIAN_POINT ( 'NONE',  ( -2.803395127021860223, 31.26063551530791074, 0.8708390753670083306 ) ) ;
#312=CARTESIAN_POINT ( 'NONE',  ( 8.369700380136936957, -11.69135346447765933, 0.7700151973242596037 ) ) ;
#313=CARTESIAN_POINT ( 'NONE',  ( 9.115443861533906400, 124.0847320388339625, 0.2671161660598814769 ) ) ;
#315=( BOUNDED_SURFACE ( )  B_SPLINE_SURFACE ( 3, 1, ( 
 ( #22075, #40860 ),
 ( #8688, #31254 ),
 ( #11879, #24648 ),
 ( #15059, #5300 ),
 ( #28059, #24868 ),
 ( #9112, #41495 ),
 ( #34264, #31896 ),
 ( #12300, #21650 ),
 ( #38293, #41069 ),
 ( #37864, #18888 ),
 ( #31468, #35102 ),
 ( #2311, #28277 ),
 ( #8896, #41282 ),
 ( #5720, #18676 ),
 ( #31683, #2733 ),
 ( #28487, #15688 ) ),
 .UNSPECIFIED., .T., .F., .T. ) 
 B_SPLINE_SURFACE_WITH_KNOTS ( ( 4, 1, 1, 1, 1, 1, 2, 1, 1, 1, 1, 1, 4 ),
 ( 2, 2 ),
 ( 0.000000000000000000, 0.02374999999999993783, 0.1365624999999999478, 0.2493749999999999578, 0.3621874999999999956, 0.4749999999999999778, 0.5000000000000000000, 0.5250000000000000222, 0.6378125000000000044, 0.7506249999999999867, 0.8634374999999999689, 0.9762499999999999512, 1.000000000000000000 ),
 ( 0.000000000000000000, 1.000000000000000000 ),
 .UNSPECIFIED. ) 
 GEOMETRIC_REPRESENTATION_ITEM ( )  RATIONAL_B_SPLINE_SURFACE ( (
 ( 1.000000000000000000, 1.000000000000000000),
 ( 1.000000000000000222, 1.000000000000000000),
 ( 0.8208939328743548591, 1.000000000000000000),
 ( 0.5876145654044752087, 1.000000000000000000),
 ( 0.4813067448364888867, 1.000000000000000000),
 ( 0.5852845309810671415, 1.000000000000000000),
 ( 0.8180077452667815496, 1.000000000000000000),
 ( 0.9982788296041308351, 1.000000000000000000),
 ( 0.9982788296041308351, 1.000000000000000000),
 ( 0.8180077452667815496, 1.000000000000000000),
 ( 0.5852845309810672525, 1.000000000000000000),
 ( 0.4813067448364889422, 1.000000000000000000),
 ( 0.5876145654044749866, 1.000000000000000000),
 ( 0.8208939328743545261, 1.000000000000000000),
 ( 1.000000000000000000, 1.000000000000000000),
 ( 1.000000000000000000, 1.000000000000000000) ) ) 
 REPRESENTATION_ITEM ( '' )  SURFACE ( )  );
#317=CARTESIAN_POINT ( 'NONE',  ( 5.564716835327648603, 116.6996553459067485, 0.05384121919325710742 ) ) ;
#320=DIRECTION ( 'NONE',  ( -5.206863593109713661E-17, 1.000000000000000000, -1.077750396879097183E-30 ) ) ;
#321=CARTESIAN_POINT ( 'NONE',  ( -4.855072294470598848, 115.7029491485453718, 1.279409886141107178 ) ) ;
#328=CARTESIAN_POINT ( 'NONE',  ( -6.912985389844515716, 117.2044255678715814, 0.04371034868568312443 ) ) ;
#331=CARTESIAN_POINT ( 'NONE',  ( -6.058547263772821267, 121.4334988323120683, -0.1247128170359407956 ) ) ;
#333=CARTESIAN_POINT ( 'NONE',  ( -5.332922648341591909, 115.7029491485453718, -0.1072025963776009894 ) ) ;
#334=CARTESIAN_POINT ( 'NONE',  ( -15.38115207166226561, 147.8278496344100859, -0.4352178850651138853 ) ) ;
#335=CARTESIAN_POINT ( 'NONE',  ( 5.987854329437395151, -12.83555092537783082, 1.339350064115379935 ) ) ;
#336=CARTESIAN_POINT ( 'NONE',  ( -20.77691070360842929, 149.9184980045912425, 1.462349339025473371 ) ) ;
#337=CARTESIAN_POINT ( 'NONE',  ( 1.325333094648095011, 19.28447512809159292, -4.440015753949128730 ) ) ;
#338=CARTESIAN_POINT ( 'NONE',  ( 23.02690842483876565, 149.8694456586574972, 0.9127416204503947528 ) ) ;
#339=CARTESIAN_POINT ( 'NONE',  ( 2.116771290498892899, -15.66388792789737217, 5.610892275307695520 ) ) ;
#340=CARTESIAN_POINT ( 'NONE',  ( 4.771882511409050842, 118.5266822147775940, -0.8399436299859415200 ) ) ;
#341=CARTESIAN_POINT ( 'NONE',  ( 0.8400667230086624748, -1.857414735510459547, 0.5005776846920441114 ) ) ;
#342=CARTESIAN_POINT ( 'NONE',  ( 0.001640166039734963777, 159.6041700698465036, -0.08208061555506483697 ) ) ;
#343=CARTESIAN_POINT ( 'NONE',  ( -0.1058213901579529159, 105.9761915687834914, 5.295735085524055030 ) ) ;
#345=ORIENTED_EDGE ( 'NONE', *, *, #41321, .T. ) ;
#346=CARTESIAN_POINT ( 'NONE',  ( -5.552382799689717707, 117.0635824090028194, 0.4511715980537314707 ) ) ;
#348=CARTESIAN_POINT ( 'NONE',  ( -7.569905091580626078, 156.0351187175861867, 1.610277000873165276 ) ) ;
#350=CARTESIAN_POINT ( 'NONE',  ( 16.25125256408137986, 125.3309463260932830, 1.843050201054562187 ) ) ;
#351=CARTESIAN_POINT ( 'NONE',  ( 1.119065284002195959, 158.2739225783580537, -1.587016747512054016 ) ) ;
#352=CARTESIAN_POINT ( 'NONE',  ( -0.6988831915142799112, -0.7227331674307564402, 0.6786060147580050828 ) ) ;
#353=CARTESIAN_POINT ( 'NONE',  ( -20.44519586420853585, 150.9797539340098069, -2.100688152434084799 ) ) ;
#354=CARTESIAN_POINT ( 'NONE',  ( 4.677671540821375373, 117.9838357377442293, -0.6916929324824377945 ) ) ;
#357=CARTESIAN_POINT ( 'NONE',  ( 16.46834812293193195, 148.4304801786341272, -1.248264531716813286 ) ) ;
#358=CARTESIAN_POINT ( 'NONE',  ( -0.0005468344959711694646, 156.3034662015456604, 0.02736583427618486872 ) ) ;
#360=CARTESIAN_POINT ( 'NONE',  ( -3.340139884075267851, 119.4525916976722897, -0.8552862985148331765 ) ) ;
#361=CARTESIAN_POINT ( 'NONE',  ( 5.741009826001572947, -15.03722989464144355, 1.207582410354154145 ) ) ;
#362=CARTESIAN_POINT ( 'NONE',  ( -5.332935381406168851, 115.7029491485442634, -0.1065653510733624160 ) ) ;
#366=CARTESIAN_POINT ( 'NONE',  ( -0.03153862713815891450, 157.4657262375360176, 1.578321868909182690 ) ) ;
#368=CARTESIAN_POINT ( 'NONE',  ( 5.011242901787458237, 115.7029491485453008, 1.398755999327908839 ) ) ;
#369=CARTESIAN_POINT ( 'NONE',  ( -2.226623034866326289, 116.5145642697238344, 1.365476420808193536 ) ) ;
#370=CARTESIAN_POINT ( 'NONE',  ( -3.240848860066210868, 23.83156553091082230, 7.781828003744739597 ) ) ;
#371=CARTESIAN_POINT ( 'NONE',  ( 4.491182069977868174, 120.9948550335633115, 0.4087774027959020229 ) ) ;
#372=CARTESIAN_POINT ( 'NONE',  ( 15.41192216945090898, 121.3506620944898060, -0.4643526128083734772 ) ) ;
#376=CARTESIAN_POINT ( 'NONE',  ( -3.302029177305334073, 159.4671159221996959, -0.06598240135525369754 ) ) ;
#379=CARTESIAN_POINT ( 'NONE',  ( -6.605722241764236280, 120.6764655449730981, -1.089203411656264553 ) ) ;
#380=CARTESIAN_POINT ( 'NONE',  ( 2.112156314984550143, -15.50190413873483664, 5.930787297944131176 ) ) ;
#381=CARTESIAN_POINT ( 'NONE',  ( -10.47888833811902920, 153.0637448873655728, -0.6176438153593468705 ) ) ;
#382=CARTESIAN_POINT ( 'NONE',  ( 4.301541689408341362, -12.13840576482722078, 1.420409876116004222 ) ) ;
#383=CARTESIAN_POINT ( 'NONE',  ( -15.08259856265902599, 121.6710330000183546, 0.7362983101480767845 ) ) ;
#384=CARTESIAN_POINT ( 'NONE',  ( -7.784012322544769269, 122.6313477034873074, -0.1555430911242075831 ) ) ;
#385=CARTESIAN_POINT ( 'NONE',  ( 15.19377495473398021, 156.0906695176550443, 0.3258312939631712868 ) ) ;
#387=CARTESIAN_POINT ( 'NONE',  ( -0.2480930319908794535, 10.21371511114847053, -4.635561276548324727 ) ) ;
#388=CARTESIAN_POINT ( 'NONE',  ( -2.732111087507159475, 116.5293111276780849, -0.05459408159141344169 ) ) ;
#389=DIRECTION ( 'NONE',  ( -0.9998004120163608288, 0.000000000000000000, -0.01997839162482747608 ) ) ;
#391=CARTESIAN_POINT ( 'NONE',  ( -5.945396627788727351, 120.3459718913957772, 0.7896226015759897354 ) ) ;
#393=CARTESIAN_POINT ( 'NONE',  ( 2.298459491326434900, 5.325542553220859787, -4.024866414273244430 ) ) ;
#394=CARTESIAN_POINT ( 'NONE',  ( 13.98195098595639152, 120.5923583732999873, 1.177051350580812894 ) ) ;
#395=CARTESIAN_POINT ( 'NONE',  ( -6.580517660824093636E-14, 85.69146620154573668, -4.881702850681514412E-18 ) ) ;
#397=CARTESIAN_POINT ( 'NONE',  ( 3.107221341096611855, 117.9340107969418341, -0.6831876054667451736 ) ) ;
#398=CARTESIAN_POINT ( 'NONE',  ( 4.615940417482057967, 3.801270455692813410, -0.2501868467277520436 ) ) ;
#399=CARTESIAN_POINT ( 'NONE',  ( -3.857972943339743388, 117.0975898859979054, -0.5726864223607189830 ) ) ;
#402=CARTESIAN_POINT ( 'NONE',  ( -15.34424630368622999, 148.0267799683202554, 0.1426181633603112453 ) ) ;
#403=ADVANCED_FACE ( 'NONE', ( #6714 ), #2778, .F. ) ;
#404=CARTESIAN_POINT ( 'NONE',  ( 2.294645149923727701, -15.44887909491890454, 5.922367448919703570 ) ) ;
#407=CARTESIAN_POINT ( 'NONE',  ( -0.4875235816601763972, 105.8261742744559513, -5.318508263945600945 ) ) ;
#409=CARTESIAN_POINT ( 'NONE',  ( 19.37512658372770602, 148.3988719805327037, 2.511650730565585299 ) ) ;
#410=CARTESIAN_POINT ( 'NONE',  ( 3.009276887026298031, 50.42904571186020490, -1.210121013456480377 ) ) ;
#411=CARTESIAN_POINT ( 'NONE',  ( 9.049782359939477772, 124.0675141969884692, 0.1808361888366267212 ) ) ;
#412=CARTESIAN_POINT ( 'NONE',  ( -6.906891541952466795, 117.5897289630162987, 0.4768185843253518463 ) ) ;
#413=CARTESIAN_POINT ( 'NONE',  ( -8.406874004389072397, 27.76653542065474056, -0.1818807619882521764 ) ) ;
#414=CARTESIAN_POINT ( 'NONE',  ( 18.50641704078256566, 154.1703991122031994, -0.1853567545699118246 ) ) ;
#418=CARTESIAN_POINT ( 'NONE',  ( 2.033723713787972009, -15.06201970758669262, 5.669216239185479012 ) ) ;
#421=CARTESIAN_POINT ( 'NONE',  ( -4.380715115686576233, 118.1845394087038272, 0.4311985218286477073 ) ) ;
#426=CARTESIAN_POINT ( 'NONE',  ( 8.373209961036389259, 119.8814485504210126, -1.110484165621906660 ) ) ;
#427=CARTESIAN_POINT ( 'NONE',  ( -7.277551686224490446, 123.0424313102424492, -0.2142739940110133801 ) ) ;
#428=CARTESIAN_POINT ( 'NONE',  ( 4.615868816244335981, 118.0368944136972971, 0.7918170276731736346 ) ) ;
#429=CARTESIAN_POINT ( 'NONE',  ( -15.92638198489195211, 148.2453349897154737, -1.585317681524597733 ) ) ;
#430=CARTESIAN_POINT ( 'NONE',  ( -2.661596506648667759, 115.7033367343655073, -1.688174420981334078 ) ) ;
#432=CARTESIAN_POINT ( 'NONE',  ( 5.069034061154215287, 114.3796182124986984, -1.753882200456532425 ) ) ;
#434=CARTESIAN_POINT ( 'NONE',  ( -13.21686059441255701, 128.5100244389050204, -1.738961528769450426 ) ) ;
#435=CARTESIAN_POINT ( 'NONE',  ( -6.529493367164978770E-14, 72.99146620154573384, -7.899616498973244731E-18 ) ) ;
#436=CARTESIAN_POINT ( 'NONE',  ( -0.02156508032628448243, 159.2730288250082538, 1.079204802879467850 ) ) ;
#438=CARTESIAN_POINT ( 'NONE',  ( 8.107080057029456555, 121.1657703571624012, -0.9663533087782769648 ) ) ;
#439=CARTESIAN_POINT ( 'NONE',  ( -9.093843756948800205, 124.2201256219595251, -0.09191904702568627628 ) ) ;
#440=CARTESIAN_POINT ( 'NONE',  ( 0.4343283552818534288, -9.202337043772711667, -4.603842121470758997 ) ) ;
#441=CARTESIAN_POINT ( 'NONE',  ( 15.72348727998148732, 121.4292885696920621, 0.9291061361373527117 ) ) ;
#443=CARTESIAN_POINT ( 'NONE',  ( 3.393951437975996743, -15.00105261681208901, 2.580228093083809071 ) ) ;
#444=CARTESIAN_POINT ( 'NONE',  ( -19.24794053165973295, 147.9830121424878939, 1.736014841626597693 ) ) ;
#445=CARTESIAN_POINT ( 'NONE',  ( 0.9605196170170531289, 3.153480984720312019, -0.1630338022177024171 ) ) ;
#446=CARTESIAN_POINT ( 'NONE',  ( -15.70934801585154439, 121.2535323456646523, -0.8362899507430229251 ) ) ;
#447=CARTESIAN_POINT ( 'NONE',  ( 0.9581433470387596962, -10.92824219907890360, 0.1848338584972420151 ) ) ;
#448=B_SPLINE_CURVE_WITH_KNOTS ( 'NONE', 3,
 ( #28992, #13011, #471, #26642, #39436, #9405, #45, #10239, #29633, #3877 ),
 .UNSPECIFIED., .F., .F.,
 ( 4, 2, 2, 2, 4 ),
 ( 0.0001363461699588103975, 0.001296643753711174303, 0.002456941337463538263, 0.003617238921215902223, 0.004777536504968266616 ),
 .UNSPECIFIED. ) ;
#450=VERTEX_POINT ( 'NONE', #12678 ) ;
#452=CARTESIAN_POINT ( 'NONE',  ( 7.253313547007579132, 123.0461458356614628, 0.2138788351844319036 ) ) ;
#453=CARTESIAN_POINT ( 'NONE',  ( -9.588254403178179786, 123.8224200044116827, 0.4900104160083063043 ) ) ;
#454=CARTESIAN_POINT ( 'NONE',  ( 3.745401017337624872, -13.88268793655436717, 4.204469449000409753 ) ) ;
#455=CARTESIAN_POINT ( 'NONE',  ( 17.22014391273205547, 144.2986879860016529, -1.480874425454277166 ) ) ;
#456=CARTESIAN_POINT ( 'NONE',  ( -12.70548372655400904, 122.4237789811383550, -1.817438969878694577 ) ) ;
#459=CARTESIAN_POINT ( 'NONE',  ( 3.197553254331486183, -13.99644925588092192, 2.254757065552156714 ) ) ;
#460=CARTESIAN_POINT ( 'NONE',  ( -5.685436017834463840, 31.78209642239458788, 1.206328258593732272 ) ) ;
#461=CARTESIAN_POINT ( 'NONE',  ( 11.88810549871044486, 151.9737369308441544, -0.07145411264644065119 ) ) ;
#462=ORIENTED_EDGE ( 'NONE', *, *, #9429, .T. ) ;
#463=CARTESIAN_POINT ( 'NONE',  ( -3.729000260451577731, 109.6950671057684588, 3.590446461533148170 ) ) ;
#465=CARTESIAN_POINT ( 'NONE',  ( 4.560443946511397506, -11.68866997254031936, 0.6947937310338139216 ) ) ;
#466=VECTOR ( 'NONE', #25714, 1000.000000000000000 ) ;
#469=CARTESIAN_POINT ( 'NONE',  ( 23.10641284836728815, 149.8968678342272653, 0.3080169626343542966 ) ) ;
#470=CARTESIAN_POINT ( 'NONE',  ( -4.503688181905225463, 111.2539628214143903, 2.957939639849824776 ) ) ;
#471=CARTESIAN_POINT ( 'NONE',  ( -3.877963262798508559, 118.0214462806859927, 0.8169714283994556903 ) ) ;
#473=CARTESIAN_POINT ( 'NONE',  ( -2.920903721094229244, 32.16307183204811082, 0.9800304932835676164 ) ) ;
#474=CARTESIAN_POINT ( 'NONE',  ( 6.753855533487119978, 118.7881172115286148, 1.217991184693928863 ) ) ;
#475=CARTESIAN_POINT ( 'NONE',  ( 3.308978306493741250, 24.09187545982852541, -3.235542752117448018 ) ) ;
#476=CARTESIAN_POINT ( 'NONE',  ( -4.294125178196657622, -12.16697637372164564, -7.253078015393731981 ) ) ;
#477=CARTESIAN_POINT ( 'NONE',  ( 5.557917761466073969, 117.8868906345641676, -0.8474712118571966490 ) ) ;
#478=CARTESIAN_POINT ( 'NONE',  ( -0.6699575554302183988, 116.0160817474902331, -1.654834682733560491 ) ) ;
#481=CARTESIAN_POINT ( 'NONE',  ( 0.8028203427309564821, 104.6144662015435216, 5.284712525425792506 ) ) ;
#483=CARTESIAN_POINT ( 'NONE',  ( -4.598301960400187127, 22.30806413504685537, 0.5496829067130363233 ) ) ;
#486=CARTESIAN_POINT ( 'NONE',  ( 2.744913772555794385, -12.89811552070117884, 0.2544447123532062038 ) ) ;
#487=CARTESIAN_POINT ( 'NONE',  ( 3.315449255180855204, 124.9344662015457743, 0.06625056644921985260 ) ) ;
#488=CARTESIAN_POINT ( 'NONE',  ( -19.54046365593634960, 128.7319734376252143, 0.5398260955622252721 ) ) ;
#489=CARTESIAN_POINT ( 'NONE',  ( 4.976458764963934023, 117.4076063131326606, -0.8841951503558329595 ) ) ;
#490=ORIENTED_EDGE ( 'NONE', *, *, #7890, .T. ) ;
#491=CARTESIAN_POINT ( 'NONE',  ( -6.589702033682734540E-14, 87.97746620154572383, -4.338478393988997516E-18 ) ) ;
#494=DIRECTION ( 'NONE',  ( -0.9998004120163608288, 0.000000000000000000, -0.01997839162482749342 ) ) ;
#495=CARTESIAN_POINT ( 'NONE',  ( 4.389818247250405037, -15.68135102926887470, 3.766867903159812681 ) ) ;
#496=CARTESIAN_POINT ( 'NONE',  ( -20.02944843481990844, 148.6304843473828043, 1.700276915703844427 ) ) ;
#497=CARTESIAN_POINT ( 'NONE',  ( 19.32406529451186117, 152.1947311750261065, -1.288948053361433033 ) ) ;
#498=CARTESIAN_POINT ( 'NONE',  ( 0.9442757308971110319, 28.15415565245834628, -0.2560175424543267297 ) ) ;
#501=CARTESIAN_POINT ( 'NONE',  ( -4.881263862402589027, 117.4111615705287477, -1.144645852924967455 ) ) ;
#503=CARTESIAN_POINT ( 'NONE',  ( 0.3562073053188078986, 119.8383472832136931, 0.7014361403029917286 ) ) ;
#504=CARTESIAN_POINT ( 'NONE',  ( 4.807157299559274399, 117.4049453230273343, 1.198158832445191724 ) ) ;
#505=CARTESIAN_POINT ( 'NONE',  ( -16.58715205660940128, 148.2569838091642964, 1.247478730927799928 ) ) ;
#507=CARTESIAN_POINT ( 'NONE',  ( 18.50543525367148945, 148.3462492009778373, -1.698196615343024574 ) ) ;
#508=CARTESIAN_POINT ( 'NONE',  ( -14.76979702826417196, 154.6636077862465015, -2.174438252133946481 ) ) ;
#511=CARTESIAN_POINT ( 'NONE',  ( 4.371200167350260735, 118.1836009977106272, -0.4408363070965656827 ) ) ;
#512=CARTESIAN_POINT ( 'NONE',  ( 8.277497327054904375, 122.7564308547279666, -0.2971990107970637895 ) ) ;
#513=B_SPLINE_CURVE_WITH_KNOTS ( 'NONE', 3,
 ( #3567, #25496, #16528, #3780, #22481, #13341 ),
 .UNSPECIFIED., .F., .F.,
 ( 4, 2, 4 ),
 ( 0.000000000000000000, 0.0001547602548093537271, 0.0003095205096187074543 ),
 .UNSPECIFIED. ) ;
#515=CARTESIAN_POINT ( 'NONE',  ( -17.73873607445684186, 146.7645792007554633, -2.242890973037755309 ) ) ;
#516=CARTESIAN_POINT ( 'NONE',  ( 2.233744238265779281, -15.22787141332636374, 5.055619554762198931 ) ) ;
#517=CARTESIAN_POINT ( 'NONE',  ( -3.676066591212550527, 105.1230425560760011, -3.867827736016857809 ) ) ;
#520=CARTESIAN_POINT ( 'NONE',  ( 2.298459491326434900, 5.325542553220859787, -4.024866414273244430 ) ) ;
#521=CARTESIAN_POINT ( 'NONE',  ( 17.47633463031920797, 147.2926247242496345, 2.162249527696345375 ) ) ;
#522=CARTESIAN_POINT ( 'NONE',  ( -2.535133856325437751, 31.19167863242842742, 1.091392955096686768 ) ) ;
#523=CARTESIAN_POINT ( 'NONE',  ( 3.263621351691376571, 8.939281053574255509, -3.290156819607050753 ) ) ;
#524=CARTESIAN_POINT ( 'NONE',  ( 11.89867495700680067, 130.3805625696445816, 0.3456363086864550627 ) ) ;
#528=CARTESIAN_POINT ( 'NONE',  ( 8.798384430222753849, 117.6845712652260545, 0.1566951038920376127 ) ) ;
#529=CARTESIAN_POINT ( 'NONE',  ( 5.078986093043054595, 66.13346620154574396, 0.1014902294541243921 ) ) ;
#530=CARTESIAN_POINT ( 'NONE',  ( -6.640726327341849406E-14, 100.6774662015457409, -1.320564745697255449E-18 ) ) ;
#536=CARTESIAN_POINT ( 'NONE',  ( -5.806485631242245482, 116.9771394561422539, 0.05772921648981179515 ) ) ;
#539=CARTESIAN_POINT ( 'NONE',  ( 6.066927103458539250, 121.4399465332669052, 0.1138985383779980987 ) ) ;
#540=ORIENTED_EDGE ( 'NONE', *, *, #11582, .F. ) ;
#541=CARTESIAN_POINT ( 'NONE',  ( -5.237832120027548832, 115.7029491485453860, -1.023639123012231034 ) ) ;
#542=CARTESIAN_POINT ( 'NONE',  ( -15.26387433774262803, 148.0131224598485744, -0.4327379813662101671 ) ) ;
#543=CARTESIAN_POINT ( 'NONE',  ( 5.090702275550843758, -14.49510550894771121, 4.025111979839017806 ) ) ;
#544=CARTESIAN_POINT ( 'NONE',  ( -18.63828149932700740, 131.8045874826418071, 1.403896228398082258 ) ) ;
#545=CARTESIAN_POINT ( 'NONE',  ( 3.465721614298269415, 18.43485028915299750, -3.064284189100199729 ) ) ;
#546=CARTESIAN_POINT ( 'NONE',  ( 14.67516008282137108, 120.3119357913517291, 0.6057029122735548832 ) ) ;
#548=CARTESIAN_POINT ( 'NONE',  ( 2.077680606031648836, -15.60673140158441718, 5.873410514533511595 ) ) ;
#549=CARTESIAN_POINT ( 'NONE',  ( 4.619096255015035624, 27.05588869245799089, -0.3994036469054788596 ) ) ;
#550=CARTESIAN_POINT ( 'NONE',  ( -0.9568942166608355171, -5.529307923341535869, 0.1941686039811585662 ) ) ;
#551=CARTESIAN_POINT ( 'NONE',  ( -23.31615218609863760, 149.0517038676186417, -0.6965919665178228470 ) ) ;
#554=CARTESIAN_POINT ( 'NONE',  ( 2.189241082030666696, 116.2106850124662998, 0.08689766813257669698 ) ) ;
#556=CARTESIAN_POINT ( 'NONE',  ( -17.70889067045670373, 148.6960320134204210, 1.618934763233637719 ) ) ;
#558=CARTESIAN_POINT ( 'NONE',  ( 13.54946078406806542, 121.5020190402118203, 1.609302047640725153 ) ) ;
#559=CARTESIAN_POINT ( 'NONE',  ( 10.86053312202623289, 155.9024031350590462, -1.736732359437422657 ) ) ;
#560=CARTESIAN_POINT ( 'NONE',  ( -0.9711860326002300647, -2.018343210913434493, -0.07513956953184577903 ) ) ;
#561=CARTESIAN_POINT ( 'NONE',  ( -14.08892660837143396, 121.3807765770047666, -1.491720297716245369 ) ) ;
#562=CARTESIAN_POINT ( 'NONE',  ( 4.543474876628542880, 118.0888849834743155, -0.5958067675172851185 ) ) ;
#563=CARTESIAN_POINT ( 'NONE',  ( -3.527324519276147541, 50.63946620154572997, 1.707870599815379364 ) ) ;
#565=CARTESIAN_POINT ( 'NONE',  ( 16.45208226155726550, 147.1833543704171348, -0.9460114105336799861 ) ) ;
#566=CARTESIAN_POINT ( 'NONE',  ( -4.591655703643919395, 121.2030596905490540, -0.06445270968432167957 ) ) ;
#568=CARTESIAN_POINT ( 'NONE',  ( -18.52244049926389025, 148.0519089404264150, -2.440181727699358483 ) ) ;
#569=CARTESIAN_POINT ( 'NONE',  ( 2.674787014790545481, -15.76824019788006304, 5.299902074303234123 ) ) ;
#570=CARTESIAN_POINT ( 'NONE',  ( -5.317765600491472178, 115.7029491485453718, 0.5108555054852879085 ) ) ;
#571=CARTESIAN_POINT ( 'NONE',  ( -4.547255095654547219, 118.0358984568298268, -0.8569604299583566398 ) ) ;
#574=CARTESIAN_POINT ( 'NONE',  ( 12.61679319894177809, 153.7453525671159298, 2.178569956567485200 ) ) ;
#576=( BOUNDED_CURVE ( )  B_SPLINE_CURVE ( 3, ( #39758, #26535, #19706, #13752, #26747, #39538, #23315 ),
 .UNSPECIFIED., .F., .T. ) 
 B_SPLINE_CURVE_WITH_KNOTS ( ( 4, 3, 4 ),
 ( 0.9253411388830656836, 0.9999999999991224797, 1.000260013143586590 ),
 .UNSPECIFIED. ) 
 CURVE ( )  GEOMETRIC_REPRESENTATION_ITEM ( )  RATIONAL_B_SPLINE_CURVE ( ( 0.7459561198782405089, 0.8157735584700518405, 0.9004548518439716709, 1.000000000000000000, 0.9996533158073767078, 0.9993068118996475402, 0.9989604882768124972 ) ) 
 REPRESENTATION_ITEM ( '' )  );
#577=CARTESIAN_POINT ( 'NONE',  ( 11.74288454345096788, 118.7273140689154616, 0.2346507796901760867 ) ) ;
#579=CARTESIAN_POINT ( 'NONE',  ( -5.114723271350774425, 118.2545999410811106, 0.5144770513779390875 ) ) ;
#580=CARTESIAN_POINT ( 'NONE',  ( -8.093932337251422027, 31.18171294578705854, -2.467657647566553258 ) ) ;
#581=CARTESIAN_POINT ( 'NONE',  ( 12.02994987064020371, 151.9703418938154584, 0.9209848757141020359 ) ) ;
#582=CARTESIAN_POINT ( 'NONE',  ( 14.73113557689540798, 120.8948172685174001, -0.5329945393104402740 ) ) ;
#587=CARTESIAN_POINT ( 'NONE',  ( -23.45022726768242549, 146.8469795362756258, -0.4427096500589554617 ) ) ;
#589=CARTESIAN_POINT ( 'NONE',  ( 6.820670703200751639, 121.2541756018108714, -0.6270318998841969416 ) ) ;
#590=CARTESIAN_POINT ( 'NONE',  ( -6.085514072855107208E-14, 88.48546620154573361, 9.693882645925084535E-17 ) ) ;
#591=CARTESIAN_POINT ( 'NONE',  ( -15.85571122620645390, 146.2799285973741519, -0.7709397856434241358 ) ) ;
#592=CARTESIAN_POINT ( 'NONE',  ( 3.951736590037845609, -12.73914099834651203, 2.215835717905272784 ) ) ;
#593=CARTESIAN_POINT ( 'NONE',  ( -14.74288075364469464, 121.6338672040446767, 0.8423781477486337321 ) ) ;
#594=CARTESIAN_POINT ( 'NONE',  ( -1.561582345843753217, 156.2588034088681184, -0.03120413162939504950 ) ) ;
#595=CARTESIAN_POINT ( 'NONE',  ( 8.067923148479861695, 158.6666700270975525, 0.2162342711943723572 ) ) ;
#596=ORIENTED_EDGE ( 'NONE', *, *, #19285, .T. ) ;
#597=CARTESIAN_POINT ( 'NONE',  ( -2.070226828232369254, -8.352695179381779411, -4.151654383260235726 ) ) ;
#598=CARTESIAN_POINT ( 'NONE',  ( 4.980330008247731755, 105.1217463992231984, 1.919414732010889413 ) ) ;
#600=CARTESIAN_POINT ( 'NONE',  ( 3.884039321165668746, 109.3893297329433381, 3.664381571631352141 ) ) ;
#601=CARTESIAN_POINT ( 'NONE',  ( 6.775796848276115725, 120.4130524060792169, 1.184928199607375943 ) ) ;
#602=CARTESIAN_POINT ( 'NONE',  ( 1.391598188199559161, 15.24595356501894017, -4.406646451508545503 ) ) ;
#603=CARTESIAN_POINT ( 'NONE',  ( 14.80859988127084925, 121.7713424311148032, 1.438396347550856991 ) ) ;
#606=CARTESIAN_POINT ( 'NONE',  ( 6.856369467415130536, 157.9234729166680040, -1.555392933271966927 ) ) ;
#607=CARTESIAN_POINT ( 'NONE',  ( 2.099109474952898236, -4.195072059908932616, -4.137704358558784712 ) ) ;
#608=CARTESIAN_POINT ( 'NONE',  ( -18.14731753714293205, 154.1160801429439857, -1.378418044792611319 ) ) ;
#611=ORIENTED_EDGE ( 'NONE', *, *, #26444, .T. ) ;
#612=CARTESIAN_POINT ( 'NONE',  ( -14.75792966017397312, 148.8440819608433969, 0.1510343195432204133 ) ) ;
#613=AXIS2_PLACEMENT_3D ( 'NONE', #33524, #14532, #31148 ) ;
#614=CARTESIAN_POINT ( 'NONE',  ( 3.432440172432007053, -15.40242305089609154, 5.447709670318832131 ) ) ;
#615=AXIS2_PLACEMENT_3D ( 'NONE', #13234, #13012, #26005 ) ;
#617=CARTESIAN_POINT ( 'NONE',  ( 3.075357915497110017, -13.94103813162880989, 1.416127232796946966 ) ) ;
#620=CARTESIAN_POINT ( 'NONE',  ( 19.13795181553994951, 149.5120288530235655, 2.492102325696694987 ) ) ;
#621=DIRECTION ( 'NONE',  ( -5.206863593109713661E-17, 1.000000000000000000, -1.077750396879097183E-30 ) ) ;
#622=DIRECTION ( 'NONE',  ( -4.017660918040594346E-17, 1.000000000000000000, 2.376309959284834438E-19 ) ) ;
#623=CARTESIAN_POINT ( 'NONE',  ( -22.36672427266407936, 142.2114994846844240, 0.8677673306393178798 ) ) ;
#624=CARTESIAN_POINT ( 'NONE',  ( 5.482275759465073506, 24.31437370403141784, -6.390863428313894978 ) ) ;
#625=CARTESIAN_POINT ( 'NONE',  ( 8.534279067096685267, 122.4751019636825049, 0.9739960529120708088 ) ) ;
#626=CARTESIAN_POINT ( 'NONE',  ( 21.27466159042545613, 132.4531229209162575, -0.1171209876626083529 ) ) ;
#628=CARTESIAN_POINT ( 'NONE',  ( -4.958249173792594888, 117.6484007699707206, 0.6696174729038590900 ) ) ;
#630=CARTESIAN_POINT ( 'NONE',  ( -4.757248705868250660, 117.4032733054483799, -1.206458839318209408 ) ) ;
#634=CARTESIAN_POINT ( 'NONE',  ( -4.483631243783302800, 118.1297507219403826, 0.5359420136376905619 ) ) ;
#635=DIRECTION ( 'NONE',  ( -4.017660918040594346E-17, 1.000000000000000000, 2.376309959284834438E-19 ) ) ;
#638=ADVANCED_FACE ( 'NONE', ( #39516 ), #20691, .T. ) ;
#639=CIRCLE ( 'NONE', #1999, 5.080000000000006288 ) ;
#640=CARTESIAN_POINT ( 'NONE',  ( 3.984814155878985797, 119.0966718691183956, -0.7651888519286457191 ) ) ;
#641=CARTESIAN_POINT ( 'NONE',  ( -2.913298842129383281, 107.8271213589905386, -4.473571949258134950 ) ) ;
#642=CARTESIAN_POINT ( 'NONE',  ( 4.528137707338466100, 118.0895881931546825, 0.7656966491790531126 ) ) ;
#643=CARTESIAN_POINT ( 'NONE',  ( -16.14046266016593023, 146.7365623387580342, -1.292066526867235776 ) ) ;
#645=DIRECTION ( 'NONE',  ( -0.01997839162482737546, -1.040247600000940825E-18, 0.9998004120163610509 ) ) ;
#646=CARTESIAN_POINT ( 'NONE',  ( 5.274668375481190274, 116.0897965414613964, -1.029904101180854514 ) ) ;
#647=CARTESIAN_POINT ( 'NONE',  ( -12.92681072397291864, 152.2092440956282076, -1.775214794609845326 ) ) ;
#648=CARTESIAN_POINT ( 'NONE',  ( -5.306918775014303868, 116.0444662015457169, 1.063204892635948307 ) ) ;
#649=CARTESIAN_POINT ( 'NONE',  ( -0.008148259816615344500, 159.5682499516715040, 0.4077722408685187649 ) ) ;
#650=DIRECTION ( 'NONE',  ( -4.017660918040594346E-17, 1.000000000000000000, 2.376309959284834438E-19 ) ) ;
#651=CARTESIAN_POINT ( 'NONE',  ( -4.198627658836969090, 155.8781008607725767, 0.05950270295165668161 ) ) ;
#652=CARTESIAN_POINT ( 'NONE',  ( 3.895047602890354010, -2.730319773039217690, 2.488009491782988469 ) ) ;
#653=CARTESIAN_POINT ( 'NONE',  ( 6.894332492628085340, 117.4533518774869947, 0.6472591412684411960 ) ) ;
#654=CARTESIAN_POINT ( 'NONE',  ( 5.219197883255967341, 105.1221402665274525, -1.156025970443059991 ) ) ;
#655=CARTESIAN_POINT ( 'NONE',  ( 2.944601773672358203, -15.01875103642165499, 4.065120351795452613 ) ) ;
#656=CARTESIAN_POINT ( 'NONE',  ( -11.73216920131865670, 154.7938929448963279, 1.733846838993656547 ) ) ;
#657=CARTESIAN_POINT ( 'NONE',  ( -0.8194340683325834762, 6.824753112428224355, -0.5254904297167376503 ) ) ;
#658=CARTESIAN_POINT ( 'NONE',  ( -23.13755856728675653, 142.6111785389246336, -1.063510652947476931 ) ) ;
#659=CARTESIAN_POINT ( 'NONE',  ( 0.8486417380921021936, -9.850041244260159701, -0.4793021190969105616 ) ) ;
#662=CARTESIAN_POINT ( 'NONE',  ( 5.131660560485880929, 115.4810986995850755, 1.508144361588664051 ) ) ;
#664=CARTESIAN_POINT ( 'NONE',  ( -1.530333064024551160, 120.5919059741422217, 0.2783515840389084728 ) ) ;
#665=CARTESIAN_POINT ( 'NONE',  ( 4.230101149094581459, -11.70512343023444402, 0.7321030916320588888 ) ) ;
#666=CARTESIAN_POINT ( 'NONE',  ( 17.26811951358304498, 148.1877419978735873, -1.462309189260816655 ) ) ;
#667=CARTESIAN_POINT ( 'NONE',  ( -13.59052456474564430, 154.1626644387825991, -2.292254590369200873 ) ) ;
#668=CARTESIAN_POINT ( 'NONE',  ( 1.938979755120314952, 104.6144662015456959, 4.428504999179026846 ) ) ;
#669=CARTESIAN_POINT ( 'NONE',  ( 3.220330141560203696, -14.30903721375789317, 2.546581355196453345 ) ) ;
#670=CARTESIAN_POINT ( 'NONE',  ( -4.860329684765736680, 117.5461367057571636, -1.119675193854307249 ) ) ;
#671=CARTESIAN_POINT ( 'NONE',  ( 9.105893302116596644, 123.9936668703698075, 0.02250835519154697345 ) ) ;
#673=CARTESIAN_POINT ( 'NONE',  ( -3.563491213075201891, 108.3861669196204360, 3.960735735213689157 ) ) ;
#678=CARTESIAN_POINT ( 'NONE',  ( 22.98049992366328809, 150.1579452496398801, 0.3057203305217678357 ) ) ;
#679=CARTESIAN_POINT ( 'NONE',  ( -5.302326897023659669, 116.4520502601644409, 0.8833424955642700249 ) ) ;
#680=CARTESIAN_POINT ( 'NONE',  ( -1.614223865627344434, 118.7629491485454167, 1.182319156186325548 ) ) ;
#682=CARTESIAN_POINT ( 'NONE',  ( -4.975175664203050907, 32.06598106186588382, 0.7459204072935275986 ) ) ;
#683=CARTESIAN_POINT ( 'NONE',  ( 17.00694855514563741, 128.5677977248401476, 2.111551361116177361 ) ) ;
#684=CARTESIAN_POINT ( 'NONE',  ( 4.518289034361447243, 23.24227448397437001, -0.9983406360900146659 ) ) ;
#685=CARTESIAN_POINT ( 'NONE',  ( 7.419718609332475623, 16.48482641057854892, 3.982871883899435250 ) ) ;
#686=CARTESIAN_POINT ( 'NONE',  ( -8.622446851455114469, 118.4541269161059773, -1.064047717557140116 ) ) ;
#687=CARTESIAN_POINT ( 'NONE',  ( -1.585818144368670746, 119.1892773189224783, -0.7268676395674203983 ) ) ;
#689=CARTESIAN_POINT ( 'NONE',  ( -3.682264917456323783, 84.67546620154573134, -0.07358041635423968885 ) ) ;
#690=CARTESIAN_POINT ( 'NONE',  ( -4.247245584637960647, 22.75789413176893206, 1.861891798430825862 ) ) ;
#693=CARTESIAN_POINT ( 'NONE',  ( -15.56076557484951906, 120.7233670659557419, -0.3109411287493939469 ) ) ;
#694=CARTESIAN_POINT ( 'NONE',  ( 2.781118144868611974, -14.77119122201073154, 4.489572933734862659 ) ) ;
#695=CARTESIAN_POINT ( 'NONE',  ( 3.315740949751757149, 124.7872298565087021, 0.06001882965729966185 ) ) ;
#696=CARTESIAN_POINT ( 'NONE',  ( -22.01496335533490978, 136.8935083344700558, 0.5016514318445888243 ) ) ;
#703=CARTESIAN_POINT ( 'NONE',  ( 1.122158211225881885, 34.81801111161350804, -0.09678150280622686841 ) ) ;
#704=CARTESIAN_POINT ( 'NONE',  ( 3.555176734920527437, -15.70662665601262020, 4.164229356387482817 ) ) ;
#705=CARTESIAN_POINT ( 'NONE',  ( -4.664640489119783240, 158.0471523224993859, 1.621167461353164807 ) ) ;
#706=CARTESIAN_POINT ( 'NONE',  ( 14.11223987312410522, 121.6707806233237363, -1.016201875498928153 ) ) ;
#707=CARTESIAN_POINT ( 'NONE',  ( 4.560200836559435977, -11.68919918208664122, 0.6963878748952898601 ) ) ;
#709=ORIENTED_EDGE ( 'NONE', *, *, #5033, .T. ) ;
#710=CARTESIAN_POINT ( 'NONE',  ( -4.784543075752243801, 117.4060574113812265, -1.200192385861798883 ) ) ;
#711=CARTESIAN_POINT ( 'NONE',  ( 2.096106201831287930, 122.9394440205640961, 0.1965313455681951260 ) ) ;
#712=CARTESIAN_POINT ( 'NONE',  ( -16.63213601294270561, 144.0643239018434940, 1.266953209168787176 ) ) ;
#714=CARTESIAN_POINT ( 'NONE',  ( 16.09548914235255168, 150.9843922791743296, -1.671617783681723424 ) ) ;
#715=CARTESIAN_POINT ( 'NONE',  ( -8.897726962874944689, 119.7003323559047061, -1.444919796022273051 ) ) ;
#716=DIRECTION ( 'NONE',  ( -4.017660918040594346E-17, 1.000000000000000000, 2.376309959284832031E-19 ) ) ;
#718=CARTESIAN_POINT ( 'NONE',  ( 4.529352846675309685, 118.1222063800068867, -0.4828943068153593865 ) ) ;
#719=CARTESIAN_POINT ( 'NONE',  ( 15.67979071779206457, 147.9168465093495399, -0.5330609057418901342 ) ) ;
#721=CARTESIAN_POINT ( 'NONE',  ( 3.208040786519721355, -14.49217647381938257, 1.686337311097440894 ) ) ;
#722=CARTESIAN_POINT ( 'NONE',  ( -4.030424611563636184, 105.1222741834141345, -3.510259462146176013 ) ) ;
#724=CARTESIAN_POINT ( 'NONE',  ( -1.290833045837797455, 0.8901568857254957834, 4.466177308409287505 ) ) ;
#725=CARTESIAN_POINT ( 'NONE',  ( 9.120583164541022470, 155.0058477609193801, 1.824713877226967984 ) ) ;
#726=CARTESIAN_POINT ( 'NONE',  ( 2.802822085653141837, 37.46604678162410096, -0.5169543402998219017 ) ) ;
#727=CARTESIAN_POINT ( 'NONE',  ( 2.003160574663116034, 15.61121511114846960, 4.187759092076685619 ) ) ;
#728=CARTESIAN_POINT ( 'NONE',  ( 14.68908181661150358, 148.8396455022467535, 0.5202010721049652453 ) ) ;
#729=CARTESIAN_POINT ( 'NONE',  ( -3.836572904814790075, 108.9297306800247895, 3.710741818055595775 ) ) ;
#730=EDGE_CURVE ( 'NONE', #19419, #35057, #10104, .T. ) ;
#732=CARTESIAN_POINT ( 'NONE',  ( 5.563298544691044789, 116.7240770658327449, -0.06738706188448287393 ) ) ;
#743=CARTESIAN_POINT ( 'NONE',  ( -15.83110339195400051, 121.2341309109925334, 0.1099079758964732340 ) ) ;
#744=ORIENTED_EDGE ( 'NONE', *, *, #5220, .T. ) ;
#746=CARTESIAN_POINT ( 'NONE',  ( 6.987640295846608396, 121.9536763068500846, 0.09064736684296234581 ) ) ;
#748=FACE_OUTER_BOUND ( 'NONE', #31178, .T. ) ;
#750=CARTESIAN_POINT ( 'NONE',  ( -9.144532176012628355, 124.1724329610943300, -0.2170005234668579974 ) ) ;
#751=CARTESIAN_POINT ( 'NONE',  ( 6.243909332557862513, -14.15813981987112946, 1.248599486541194681 ) ) ;
#752=CARTESIAN_POINT ( 'NONE',  ( -0.01023305610376992747, 117.8848902025789158, 0.5121039721716188486 ) ) ;
#753=CARTESIAN_POINT ( 'NONE',  ( -3.290491044589036740, 30.52917213649525507, -3.264312889705288878 ) ) ;
#754=CARTESIAN_POINT ( 'NONE',  ( 11.61197380483875818, 118.7506923092098674, 0.5208889651483786798 ) ) ;
#755=CARTESIAN_POINT ( 'NONE',  ( 15.63882844255756055, 147.2230043458672242, 0.5131701251512970074 ) ) ;
#756=CARTESIAN_POINT ( 'NONE',  ( 2.739727753987758252, 28.35525327666260864, -3.728201022356329553 ) ) ;
#757=CARTESIAN_POINT ( 'NONE',  ( -0.5327793704965378963, 2.243135046448306191, -0.8176680881360027797 ) ) ;
#758=CARTESIAN_POINT ( 'NONE',  ( 0.003073183581686570603, 116.5806198863164838, -0.1537946732117059789 ) ) ;
#760=CARTESIAN_POINT ( 'NONE',  ( 4.973296405157103806, 117.3984635962171126, 0.9753329598428331915 ) ) ;
#761=CARTESIAN_POINT ( 'NONE',  ( -2.216312923931310408, 116.2476184459632691, 0.05817610133434990283 ) ) ;
#762=CARTESIAN_POINT ( 'NONE',  ( -15.69153790699154349, 150.8349565870724120, 1.587821608835076725 ) ) ;
#764=CARTESIAN_POINT ( 'NONE',  ( 2.782193507150679590, 158.7847427699215928, 1.504205172470084895 ) ) ;
#765=CARTESIAN_POINT ( 'NONE',  ( 0.03245814172804981773, 158.1186941186938952, -1.624338139048501439 ) ) ;
#766=CARTESIAN_POINT ( 'NONE',  ( 0.8497018901738310204, -5.914940278964642140, -0.4796499176142879906 ) ) ;
#767=CARTESIAN_POINT ( 'NONE',  ( -2.957233306982606447, 159.1263692740743068, -1.212116333074086061 ) ) ;
#768=CARTESIAN_POINT ( 'NONE',  ( 4.620269582450577062, 118.0223433806428233, -0.6741668739178967584 ) ) ;
#770=CARTESIAN_POINT ( 'NONE',  ( 8.403980202277340439, 154.6912814427390970, -0.9387012965349952331 ) ) ;
#771=CARTESIAN_POINT ( 'NONE',  ( -2.829134042005175598, 121.0305217392013759, -0.03030232591675474305 ) ) ;
#773=CARTESIAN_POINT ( 'NONE',  ( -4.201129436297949660, 119.4047208153655646, -0.9741049750989214662 ) ) ;
#774=CARTESIAN_POINT ( 'NONE',  ( 1.930844028328122519, -15.65960119559217745, 5.531553210582124791 ) ) ;
#776=CARTESIAN_POINT ( 'NONE',  ( -4.688800654935717738, 117.9735489986441905, -0.8264284708620113218 ) ) ;
#777=CIRCLE ( 'NONE', #24537, 0.5079999999999997851 ) ;
#779=CARTESIAN_POINT ( 'NONE',  ( 4.065926199369043204, 118.2429491485453354, 0.3080910687088499467 ) ) ;
#780=CARTESIAN_POINT ( 'NONE',  ( 2.417314592637331394, 119.3768144667271542, 0.7569762546260364600 ) ) ;
#783=CARTESIAN_POINT ( 'NONE',  ( 17.31377588638417819, 122.7721875394316555, 0.3459704467065360944 ) ) ;
#784=CARTESIAN_POINT ( 'NONE',  ( 5.116497545627949783, 15.83618160547830911, 6.690270154343205711 ) ) ;
#785=CARTESIAN_POINT ( 'NONE',  ( 10.59645057104354926, 153.0636280899912549, 0.8695332296301788721 ) ) ;
#786=CARTESIAN_POINT ( 'NONE',  ( 22.63811803559990921, 149.3758529064199934, -0.7269731895922278975 ) ) ;
#788=ORIENTED_EDGE ( 'NONE', *, *, #21628, .T. ) ;
#790=EDGE_CURVE ( 'NONE', #20793, #10681, #4692, .T. ) ;
#791=CARTESIAN_POINT ( 'NONE',  ( -23.35271726849064322, 148.8653451956335516, -0.3123667622787952292 ) ) ;
#793=CARTESIAN_POINT ( 'NONE',  ( -5.638488239624087406, 120.9463007187987529, -0.6439909558628548192 ) ) ;
#795=CARTESIAN_POINT ( 'NONE',  ( -6.089391457280442843, 155.3491548655973133, -0.5861119247043796721 ) ) ;
#796=CARTESIAN_POINT ( 'NONE',  ( 4.230101149094581459, -11.70512343023444402, 0.7321030916320588888 ) ) ;
#797=CARTESIAN_POINT ( 'NONE',  ( -22.13784291382281566, 148.5290936231802448, 1.147597636374165342 ) ) ;
#800=CARTESIAN_POINT ( 'NONE',  ( 5.779653879267166339, 116.9360814311326777, 0.1581498910197089158 ) ) ;
#802=CARTESIAN_POINT ( 'NONE',  ( -2.395914033174281865, 1.367755174955888275, -3.957843245732672877 ) ) ;
#803=CARTESIAN_POINT ( 'NONE',  ( -16.17518884900012566, 121.2571949256804089, -0.3403554851049457319 ) ) ;
#805=DIRECTION ( 'NONE',  ( 0.01997839162482749689, 1.040247600000945640E-18, -0.9998004120163610509 ) ) ;
#806=CARTESIAN_POINT ( 'NONE',  ( -8.182749385635133876, 120.8045967382623473, 1.052528022748003167 ) ) ;
#807=CARTESIAN_POINT ( 'NONE',  ( -4.227217475240903077, -11.31673468295422147, -1.889206449475258509 ) ) ;
#808=CARTESIAN_POINT ( 'NONE',  ( 12.77893255256110372, 120.0678233105195716, 1.216039656670922398 ) ) ;
#811=CARTESIAN_POINT ( 'NONE',  ( 1.179722549733654091, 118.0995038195805904, -0.6028833020595596448 ) ) ;
#813=CARTESIAN_POINT ( 'NONE',  ( -4.324967070706027705, -0.5217348546298695711, 1.653223044864502222 ) ) ;
#814=CARTESIAN_POINT ( 'NONE',  ( -21.30289582938792847, 151.2846570542378117, -1.588627997894106247 ) ) ;
#816=CARTESIAN_POINT ( 'NONE',  ( -9.242439611670359767, 123.9961275534082148, 0.1349267066575720320 ) ) ;
#817=CARTESIAN_POINT ( 'NONE',  ( 6.086938242954471612, -13.85866328171454853, 1.967354546201298682 ) ) ;
#818=CARTESIAN_POINT ( 'NONE',  ( 5.586884702347364673, 92.04146620154574521, 0.1116392523995368424 ) ) ;
#819=CARTESIAN_POINT ( 'NONE',  ( -6.439703808512989190E-14, 63.33946620154573282, 4.463794035948134848E-29 ) ) ;
#821=CARTESIAN_POINT ( 'NONE',  ( 18.52749500581553477, 150.2488615152233820, 2.471439233876493446 ) ) ;
#822=CARTESIAN_POINT ( 'NONE',  ( 4.914877656105587356, 117.6230825708500305, 0.9484198851692730026 ) ) ;
#825=TOROIDAL_SURFACE ( 'NONE', #25283, 3.683000000000000718, 0.5080000000000000071 ) ;
#826=CARTESIAN_POINT ( 'NONE',  ( -0.007599820978812334323, 117.2191897141855179, 0.3803261187632672735 ) ) ;
#827=CARTESIAN_POINT ( 'NONE',  ( 1.329249052905784323, 1.652534479431654546, 8.327223686629459110 ) ) ;
#828=CARTESIAN_POINT ( 'NONE',  ( 16.04436118421907054, 148.0691544347876345, 1.589228464704729005 ) ) ;
#831=CARTESIAN_POINT ( 'NONE',  ( 21.71781664064052464, 151.4054434770023363, -0.2817300504337350020 ) ) ;
#832=CARTESIAN_POINT ( 'NONE',  ( 5.332935397695204749, 62.83146620154573014, 0.1065647409268304785 ) ) ;
#835=CARTESIAN_POINT ( 'NONE',  ( -4.426222872263863906, 117.3993836135536952, 1.092072450647614046 ) ) ;
#839=CARTESIAN_POINT ( 'NONE',  ( -4.462445684601345164, 118.1590134028923700, 0.4283344254013793928 ) ) ;
#840=CARTESIAN_POINT ( 'NONE',  ( 3.729890348113323650, 109.6950698699627225, -3.590377456412748636 ) ) ;
#844=CARTESIAN_POINT ( 'NONE',  ( 6.071325138224676898, 119.3725698982003394, -1.023810605546056074 ) ) ;
#845=CARTESIAN_POINT ( 'NONE',  ( -1.375939976466558967, 106.2431249238853894, -5.170880015306797084 ) ) ;
#846=CARTESIAN_POINT ( 'NONE',  ( 4.574376597671965250, 118.0199863044615256, 0.8705714316668682340 ) ) ;
#847=CARTESIAN_POINT ( 'NONE',  ( -6.483461908857862888, 121.4942169270607053, -0.6390524964423260901 ) ) ;
#848=CARTESIAN_POINT ( 'NONE',  ( -0.7503968993307388313, 115.7029095610640184, -1.755757167250588280 ) ) ;
#849=CARTESIAN_POINT ( 'NONE',  ( 0.8116844938904650419, 118.1651004003055618, -0.8535674157383565941 ) ) ;
#850=CARTESIAN_POINT ( 'NONE',  ( 5.793465281260485433, 118.4310156723767307, -0.4331262667984489556 ) ) ;
#851=CARTESIAN_POINT ( 'NONE',  ( -10.28893712963056117, 123.4707319107414492, -1.320145760562476678 ) ) ;
#855=CARTESIAN_POINT ( 'NONE',  ( 8.330184522151043325, 120.0920323058251000, -1.118340454250545735 ) ) ;
#856=CARTESIAN_POINT ( 'NONE',  ( -5.969990878950643065, 121.5454240333526599, -0.007965473844366978071 ) ) ;
#857=CARTESIAN_POINT ( 'NONE',  ( 4.886022116125724679, 117.7561648045584519, -0.7145573245312663024 ) ) ;
#858=CARTESIAN_POINT ( 'NONE',  ( 22.95323918608228198, 146.5883926500602001, 1.439717189780889806 ) ) ;
#860=CARTESIAN_POINT ( 'NONE',  ( 3.283982329611080608, -15.09957111342241731, 3.272784416514652239 ) ) ;
#861=CARTESIAN_POINT ( 'NONE',  ( -12.09213366837452419, 122.8144071692085504, 1.302296015248258110 ) ) ;
#862=CARTESIAN_POINT ( 'NONE',  ( -0.09096679801628397566, 0.3556511065658448656, 0.9697834404811940257 ) ) ;
#863=CARTESIAN_POINT ( 'NONE',  ( -1.385657586283601583, 159.5796833544862352, -0.3718886678235073240 ) ) ;
#865=CARTESIAN_POINT ( 'NONE',  ( 0.07244829501375356362, -8.348772924205562163, -0.9745465824848156267 ) ) ;
#868=CARTESIAN_POINT ( 'NONE',  ( 2.472230802051491150, 107.2388417251876547, 4.724420784806152795 ) ) ;
#869=CARTESIAN_POINT ( 'NONE',  ( -0.01133107913651526001, 156.3792106723807649, 0.5670535347366658652 ) ) ;
#870=EDGE_CURVE ( 'NONE', #12283, #10681, #20973, .T. ) ;
#871=CARTESIAN_POINT ( 'NONE',  ( 2.867264926914522949, -14.81558118910870903, 5.578245215537346979 ) ) ;
#872=CARTESIAN_POINT ( 'NONE',  ( 17.62053193735413714, 147.9903219242534078, -1.529691019407824815 ) ) ;
#873=CARTESIAN_POINT ( 'NONE',  ( -4.990993783036518749, 119.0545008048120366, -1.104648745759416073 ) ) ;
#875=CARTESIAN_POINT ( 'NONE',  ( 1.831848720338793202, -15.17974794010013007, 5.463771816453670382 ) ) ;
#876=CARTESIAN_POINT ( 'NONE',  ( -4.848458278871826010, 117.4106395692391516, -1.171953005487281096 ) ) ;
#878=CARTESIAN_POINT ( 'NONE',  ( 6.494470876743749344, 121.7611753534313550, 0.002333837952680517004 ) ) ;
#880=ORIENTED_EDGE ( 'NONE', *, *, #26050, .F. ) ;
#882=CARTESIAN_POINT ( 'NONE',  ( 3.744664645882537890, 109.0594030058402240, 3.805231549001048208 ) ) ;
#886=CARTESIAN_POINT ( 'NONE',  ( 15.18069129733350309, 156.1124880001465556, 0.1695137023582059255 ) ) ;
#888=CARTESIAN_POINT ( 'NONE',  ( 1.887249359699314732, -15.69731392916340340, 5.578901855154127176 ) ) ;
#890=CARTESIAN_POINT ( 'NONE',  ( -3.065505632821621251, 31.52364725955965952, 0.7739196574294696651 ) ) ;
#891=CARTESIAN_POINT ( 'NONE',  ( 20.20973109032203396, 149.9354415288716780, 2.375026552130124369 ) ) ;
#893=CARTESIAN_POINT ( 'NONE',  ( 6.048790893839320226, 16.06121166075865148, 5.875566521300903844 ) ) ;
#894=CARTESIAN_POINT ( 'NONE',  ( 5.512831477515243606, 117.4993864815744189, -0.7243090542875012527 ) ) ;
#895=CARTESIAN_POINT ( 'NONE',  ( -2.170296427606285050, 116.5145642697238344, -1.453337335755149784 ) ) ;
#897=CARTESIAN_POINT ( 'NONE',  ( -1.761767052800523148, 106.7073752071930102, -4.966636964334769644 ) ) ;
#898=CARTESIAN_POINT ( 'NONE',  ( -5.074705355603877699, 104.6144662015446869, 1.652004153191725999 ) ) ;
#900=CARTESIAN_POINT ( 'NONE',  ( 4.219463811995017188, -1.205994944679912306, -1.932895124392335573 ) ) ;
#903=CARTESIAN_POINT ( 'NONE',  ( 2.253193219399967973, -14.99063959920543532, 5.175666457621841410 ) ) ;
#904=CARTESIAN_POINT ( 'NONE',  ( 3.676218128927467799, 120.6652674781340551, -0.2791188998294427681 ) ) ;
#905=CARTESIAN_POINT ( 'NONE',  ( -16.51027305157944625, 155.2380866766625047, 0.5525915368032878749 ) ) ;
#907=CARTESIAN_POINT ( 'NONE',  ( 4.999551999793056645, 117.4036825309383119, -0.8308859279095415218 ) ) ;
#909=VERTEX_POINT ( 'NONE', #10455 ) ;
#910=CARTESIAN_POINT ( 'NONE',  ( -5.065021746985605589, 115.7029491485453576, 1.195979280658540755 ) ) ;
#911=CARTESIAN_POINT ( 'NONE',  ( 4.076841989731768479, -15.73006006892005360, 3.802225825406736259 ) ) ;
#912=CARTESIAN_POINT ( 'NONE',  ( -0.03153870137021549253, 158.4432089348667319, 1.578325583784928376 ) ) ;
#913=CARTESIAN_POINT ( 'NONE',  ( -0.8472427164685307766, -8.777537934218566207, -4.544909406875613733 ) ) ;
#917=CARTESIAN_POINT ( 'NONE',  ( 1.644890720626006386, 119.8612358676174949, 0.5912986496483325638 ) ) ;
#918=CARTESIAN_POINT ( 'NONE',  ( -16.72891957527401630, 148.5304741467402323, 1.365449702224204032 ) ) ;
#921=CARTESIAN_POINT ( 'NONE',  ( 11.41525058642613288, 122.8492764348241337, -1.228842657910305780 ) ) ;
#923=CARTESIAN_POINT ( 'NONE',  ( -2.647237659633569606, 158.4754809254847601, -1.642537635467619772 ) ) ;
#924=CARTESIAN_POINT ( 'NONE',  ( -6.136538366514222075E-14, 101.1854662015457365, 9.995674010754261804E-17 ) ) ;
#927=CARTESIAN_POINT ( 'NONE',  ( 4.387465901250098277, 118.1845649924603379, -0.4239173906933821345 ) ) ;
#928=CARTESIAN_POINT ( 'NONE',  ( 15.85992372348528434, 147.2950763206921181, -0.4080883723285143594 ) ) ;
#929=VERTEX_POINT ( 'NONE', #20445 ) ;
#930=CARTESIAN_POINT ( 'NONE',  ( 3.239928030326187258, -14.81799142783181367, -0.3301716407829758948 ) ) ;
#936=CARTESIAN_POINT ( 'NONE',  ( 3.235533175430977515, 2.501875212487111977, 3.308963532380430284 ) ) ;
#937=CARTESIAN_POINT ( 'NONE',  ( 12.21508602987348269, 126.0625018263836807, 1.612267168929819583 ) ) ;
#938=CARTESIAN_POINT ( 'NONE',  ( 2.151558901213805886, 36.10138897990322704, -0.07425415374395130663 ) ) ;
#939=CARTESIAN_POINT ( 'NONE',  ( -4.319812470756069445, 11.96289413176387129, -1.686699837767231536 ) ) ;
#940=CARTESIAN_POINT ( 'NONE',  ( 15.64085066085077536, 147.2198192248932571, 0.3637928714071058667 ) ) ;
#943=CARTESIAN_POINT ( 'NONE',  ( 8.796184242131879216, 117.7096009060177266, 0.009943947433590954663 ) ) ;
#944=CARTESIAN_POINT ( 'NONE',  ( 16.86202032626302483, 155.2029898760372646, 0.3369432954968345495 ) ) ;
#945=AXIS2_PLACEMENT_3D ( 'NONE', #37814, #8640, #17790 ) ;
#949=CARTESIAN_POINT ( 'NONE',  ( 0.1224881284885083327, 5.266211660758980173, 8.431793989537572642 ) ) ;
#953=CARTESIAN_POINT ( 'NONE',  ( 0.02135216056118049294, 118.1497763966934258, -1.068549427312639910 ) ) ;
#954=CARTESIAN_POINT ( 'NONE',  ( -15.62286502883001837, 121.0226940419799462, 0.1111101786179100326 ) ) ;
#957=CARTESIAN_POINT ( 'NONE',  ( 6.073369455593417676, 121.4395935480491318, 0.1192957112538572118 ) ) ;
#960=CARTESIAN_POINT ( 'NONE',  ( -15.72281364106782675, 146.8976350983841144, -0.3655119725415948984 ) ) ;
#961=CARTESIAN_POINT ( 'NONE',  ( 2.468517452056580463, -15.43523125850157562, 5.870468177969554446 ) ) ;
#962=CARTESIAN_POINT ( 'NONE',  ( -21.01144550848356829, 149.0309112320384486, 1.514039682450821545 ) ) ;
#963=CARTESIAN_POINT ( 'NONE',  ( -2.201963191602333225, 30.07953629247752758, -4.075912811544394998 ) ) ;
#964=CARTESIAN_POINT ( 'NONE',  ( -0.004910662370487759928, 159.5928157220454295, 0.2457496255665023166 ) ) ;
#965=CARTESIAN_POINT ( 'NONE',  ( 2.076497001697454436, -15.66584657922642876, 5.557590741999150374 ) ) ;
#966=CARTESIAN_POINT ( 'NONE',  ( 0.2838385327444274964, 29.22985346960623332, -4.617364983570896086 ) ) ;
#967=CARTESIAN_POINT ( 'NONE',  ( 0.9769954323678800012, -0.8923827921977626199, -0.09387087892739469364 ) ) ;
#968=CARTESIAN_POINT ( 'NONE',  ( -2.778732907383235862, 116.5968896900294709, -0.2040764120049695651 ) ) ;
#969=LINE ( 'NONE', #13938, #25666 ) ;
#972=CARTESIAN_POINT ( 'NONE',  ( 5.531187961632795691, 116.9767413707218253, 0.6070940273833828060 ) ) ;
#973=CARTESIAN_POINT ( 'NONE',  ( -17.67426794430100401, 144.4767212251450417, 1.594784396078125388 ) ) ;
#975=CARTESIAN_POINT ( 'NONE',  ( 21.00644369030274206, 149.3892802667211868, 2.301546136566545275 ) ) ;
#976=CARTESIAN_POINT ( 'NONE',  ( 19.35587726549907117, 148.6897983921382433, -1.735459330159158986 ) ) ;
#979=CARTESIAN_POINT ( 'NONE',  ( -0.8109939492151988505, -12.39128985057688936, -0.5387275711561630986 ) ) ;
#980=CARTESIAN_POINT ( 'NONE',  ( -2.096789228656116499, 117.6567184779878232, -0.6641637518095836468 ) ) ;
#982=CARTESIAN_POINT ( 'NONE',  ( 4.307776028491197451, 105.1217194734575884, 3.166495586438745846 ) ) ;
#983=CARTESIAN_POINT ( 'NONE',  ( 4.675694769581089538, 155.9604050671876792, -0.8934998238159542749 ) ) ;
#984=CARTESIAN_POINT ( 'NONE',  ( 7.826010746941338247, 122.3856571825914159, 0.6413869067663138246 ) ) ;
#985=ORIENTED_EDGE ( 'NONE', *, *, #37802, .F. ) ;
#986=CARTESIAN_POINT ( 'NONE',  ( 0.01051219832176353980, 119.4384375980492194, -0.5260733902271048645 ) ) ;
#987=CARTESIAN_POINT ( 'NONE',  ( 4.176612884749554944, -15.71584146423912820, 3.621469129306375656 ) ) ;
#990=CARTESIAN_POINT ( 'NONE',  ( -4.596683656305176058, 118.0615522034898106, -0.7278660542837124270 ) ) ;
#994=CARTESIAN_POINT ( 'NONE',  ( 14.20821676177088300, 128.5469532985352714, 2.008711173933039440 ) ) ;
#996=CARTESIAN_POINT ( 'NONE',  ( 2.732111087507031133, 116.5293111276780849, 0.05459408159141365680 ) ) ;
#997=CARTESIAN_POINT ( 'NONE',  ( 5.579263951540290201, 8.940976842658965751, -6.340258638080404019 ) ) ;
#998=CARTESIAN_POINT ( 'NONE',  ( -0.008148072696649801341, 156.3406798448389168, 0.4077628766201955579 ) ) ;
#999=CARTESIAN_POINT ( 'NONE',  ( 0.3623072504455067122, 117.0882377308211773, -0.3576919811193869370 ) ) ;
#1001=FACE_OUTER_BOUND ( 'NONE', #21889, .T. ) ;
#1002=CARTESIAN_POINT ( 'NONE',  ( -22.53566265713742567, 150.7862151120626777, -0.3736683405004930791 ) ) ;
#1005=CARTESIAN_POINT ( 'NONE',  ( 5.747156222950085436, 121.0755541023018935, -0.3521415724599298858 ) ) ;
#1009=CARTESIAN_POINT ( 'NONE',  ( -0.6211475606396847926, 120.8480686026657196, -0.1701230225530362405 ) ) ;
#1010=CARTESIAN_POINT ( 'NONE',  ( 2.417269819423324861, -15.13903239461346395, 5.861448462117607505 ) ) ;
#1011=CARTESIAN_POINT ( 'NONE',  ( -12.65084386183224829, 120.1953580586475567, 0.8051295378619942600 ) ) ;
#1012=CARTESIAN_POINT ( 'NONE',  ( -0.6412933796113865492, 156.3034662015457741, -0.01281456791805603290 ) ) ;
#1013=CARTESIAN_POINT ( 'NONE',  ( 11.72380150228539186, 118.7251779360019270, 0.2815772452395035597 ) ) ;
#1014=ORIENTED_EDGE ( 'NONE', *, *, #34488, .F. ) ;
#1015=CARTESIAN_POINT ( 'NONE',  ( 4.634220987317881679, -1.855718946426311078, -0.01876340930339078644 ) ) ;
#1016=CARTESIAN_POINT ( 'NONE',  ( -23.21309708346267797, 149.6303025714371131, -0.4895544115752260561 ) ) ;
#1018=CARTESIAN_POINT ( 'NONE',  ( 5.078986093043052819, 100.6774662015457409, 0.1014902294541237954 ) ) ;
#1019=ORIENTED_EDGE ( 'NONE', *, *, #19182, .T. ) ;
#1020=CARTESIAN_POINT ( 'NONE',  ( -6.355526478890559439, 119.3884140220176988, 1.006251212807348416 ) ) ;
#1021=CARTESIAN_POINT ( 'NONE',  ( 2.099109474952898236, -4.195072059908932616, -4.137704358558784712 ) ) ;
#1022=CARTESIAN_POINT ( 'NONE',  ( 3.017629403178959446, 159.2229145144301867, 1.079859862993577613 ) ) ;
#1024=CARTESIAN_POINT ( 'NONE',  ( -5.078986093043186933, 101.1854662015457365, -0.1014902294541231709 ) ) ;
#1025=CARTESIAN_POINT ( 'NONE',  ( 20.46179744412665613, 141.4490678312372722, -1.579512522682919418 ) ) ;
#1026=CARTESIAN_POINT ( 'NONE',  ( -3.769861741716944881, -2.021032284792064093, -2.673854242032364326 ) ) ;
#1027=CARTESIAN_POINT ( 'NONE',  ( -17.57666534335618636, 125.1652531886817172, -1.391946913312247958 ) ) ;
#1028=ORIENTED_EDGE ( 'NONE', *, *, #29131, .F. ) ;
#1030=CARTESIAN_POINT ( 'NONE',  ( -9.057492758458371540, 123.9289873439938674, -0.02221773104347207761 ) ) ;
#1031=CARTESIAN_POINT ( 'NONE',  ( 5.498302128480847983, -14.40662979408034694, 3.384674516772870234 ) ) ;
#1032=DIRECTION ( 'NONE',  ( 4.017660918040594346E-17, -1.000000000000000000, -2.376309959284834438E-19 ) ) ;
#1033=CARTESIAN_POINT ( 'NONE',  ( -3.798767985847472328, 109.6290767857702235, -3.753213138019654505 ) ) ;
#1035=CARTESIAN_POINT ( 'NONE',  ( 19.28990034181448010, 145.1342744731992127, 2.527759927608660639 ) ) ;
#1036=CARTESIAN_POINT ( 'NONE',  ( 4.864735862609903982, 117.7358714380141151, 0.9167521008204471133 ) ) ;
#1038=CARTESIAN_POINT ( 'NONE',  ( -0.3722574617743142356, 117.2097358735305050, 0.3924287308447402256 ) ) ;
#1039=CARTESIAN_POINT ( 'NONE',  ( 6.828157356468467221, 12.44753447943134184, 4.948315318077098901 ) ) ;
#1040=CARTESIAN_POINT ( 'NONE',  ( 5.158718007120178584, 120.8264575521020987, 0.6815868816981847100 ) ) ;
#1043=CARTESIAN_POINT ( 'NONE',  ( 15.19762206999197396, 120.8830733721255370, -0.2994679608661979797 ) ) ;
#1044=CARTESIAN_POINT ( 'NONE',  ( 4.858589416345391321, 117.7980557432572795, -0.7304706717345029743 ) ) ;
#1047=CARTESIAN_POINT ( 'NONE',  ( -4.019356026430203066, 117.3993838141520172, 1.158635538540764731 ) ) ;
#1050=CARTESIAN_POINT ( 'NONE',  ( -4.529539828068924301, 118.1222249965676383, 0.4827831673290448600 ) ) ;
#1051=DIRECTION ( 'NONE',  ( 0.9998004120163608288, -1.039227405372660929E-20, 0.01997839162482763914 ) ) ;
#1054=CARTESIAN_POINT ( 'NONE',  ( 6.127741334488804092, 119.4943318094760372, -1.015363485661166854 ) ) ;
#1055=CARTESIAN_POINT ( 'NONE',  ( -7.136594729663847225, 122.4194348751405101, -0.2521576392032935376 ) ) ;
#1056=CARTESIAN_POINT ( 'NONE',  ( 4.486670294817050930, 118.0822176383332902, 0.8003028680957253727 ) ) ;
#1057=CARTESIAN_POINT ( 'NONE',  ( -13.61103386154299599, 134.2686865373913463, -1.213594671188916729 ) ) ;
#1058=CARTESIAN_POINT ( 'NONE',  ( -1.071200444556306364, 115.7029399934560701, -1.745870039784299443 ) ) ;
#1059=DIRECTION ( 'NONE',  ( 0.9998004120163608288, 0.000000000000000000, 0.01997839162482736852 ) ) ;
#1060=CARTESIAN_POINT ( 'NONE',  ( 2.686051902181449513, 107.2142675576569530, -4.629644704627760454 ) ) ;
#1061=CARTESIAN_POINT ( 'NONE',  ( -6.507413728078120130, 121.1369950346570192, -0.8796459533030991373 ) ) ;
#1063=CARTESIAN_POINT ( 'NONE',  ( 8.020178813429859943, 121.5755450013093366, -0.8283951592328165914 ) ) ;
#1064=CARTESIAN_POINT ( 'NONE',  ( -6.997652640569123506, 121.9526520484695027, -0.1398297549648395144 ) ) ;
#1066=CARTESIAN_POINT ( 'NONE',  ( -0.009748065369249667503, 159.5507987164374981, 0.4878330526048098581 ) ) ;
#1068=CARTESIAN_POINT ( 'NONE',  ( 3.043194142253923928, -14.61827878651010515, -0.2680077959190000358 ) ) ;
#1069=CARTESIAN_POINT ( 'NONE',  ( -15.78846850359705556, 131.3838724160208926, 1.599517327752104423 ) ) ;
#1070=CARTESIAN_POINT ( 'NONE',  ( -0.3571511390000196573, -0.07365323586406080647, 0.9071407500242820721 ) ) ;
#1071=CARTESIAN_POINT ( 'NONE',  ( -23.02941925350885555, 142.5499849734818838, -1.196609915892170584 ) ) ;
#1072=CARTESIAN_POINT ( 'NONE',  ( -0.03357488772870852872, 24.54038786010652728, -0.9749811203568246043 ) ) ;
#1073=VERTEX_POINT ( 'NONE', #29634 ) ;
#1075=CARTESIAN_POINT ( 'NONE',  ( 5.888892352462119284, 118.9932487913337411, 0.5850130909721118488 ) ) ;
#1077=CARTESIAN_POINT ( 'NONE',  ( -15.94526953466043118, 147.3275361421020193, 0.5311500221062651628 ) ) ;
#1078=CARTESIAN_POINT ( 'NONE',  ( 4.035643413487081332, -14.09208526182970189, 4.581805149448960002 ) ) ;
#1079=CARTESIAN_POINT ( 'NONE',  ( 2.533752743581966005, 119.8406177399916714, -0.5716348071481810456 ) ) ;
#1081=CARTESIAN_POINT ( 'NONE',  ( -7.606098120227111181, 119.7866739149480253, -1.386975461113101549 ) ) ;
#1082=CARTESIAN_POINT ( 'NONE',  ( 3.658123981884035647, 115.7029863172577535, 1.617079049715255845 ) ) ;
#1083=EDGE_CURVE ( 'NONE', #35234, #17174, #37846, .T. ) ;
#1084=CARTESIAN_POINT ( 'NONE',  ( 2.906309357581933650, -13.72804873580029472, 0.7610837935892840189 ) ) ;
#1087=CARTESIAN_POINT ( 'NONE',  ( 4.566879893416641245, 121.1702857069421100, -0.02052890071062566171 ) ) ;
#1090=CARTESIAN_POINT ( 'NONE',  ( 2.611213466451486109, 107.7056043231343665, 4.533743039264392927 ) ) ;
#1093=CARTESIAN_POINT ( 'NONE',  ( 13.40764007945148428, 156.9487217736090940, 0.07645926402191062510 ) ) ;
#1094=CARTESIAN_POINT ( 'NONE',  ( -5.517349593794012463, 28.10803576007639393, 0.4164286583522215368 ) ) ;
#1095=CARTESIAN_POINT ( 'NONE',  ( 2.006295418716820933, -15.63691049494941865, 5.487271958674783789 ) ) ;
#1096=CARTESIAN_POINT ( 'NONE',  ( -6.654617103318593247E-14, 104.6144662015457243, 1.534725424433578570E-31 ) ) ;
#1097=CARTESIAN_POINT ( 'NONE',  ( -3.046231754824816118, 31.09810386281187533, 0.4001267285823233433 ) ) ;
#1098=CARTESIAN_POINT ( 'NONE',  ( 2.647237659633441265, 158.4754809254847601, 1.642537635467619994 ) ) ;
#1100=VERTEX_POINT ( 'NONE', #33261 ) ;
#1101=CARTESIAN_POINT ( 'NONE',  ( -0.5381045032992836097, 19.73597684265961050, -8.428375251626778919 ) ) ;
#1102=CARTESIAN_POINT ( 'NONE',  ( -8.658272382007252688, 118.2880589149417148, -0.9754036577767483118 ) ) ;
#1103=CARTESIAN_POINT ( 'NONE',  ( -5.810938089476440638, 124.3836500214474654, -0.1311214433933293733 ) ) ;
#1104=CARTESIAN_POINT ( 'NONE',  ( 4.784097136343040013, 117.4060489132068597, 1.200267903224836896 ) ) ;
#1106=CARTESIAN_POINT ( 'NONE',  ( -0.001261869788248145890, 124.3520329708341876, 0.06314912420803926729 ) ) ;
#1107=CARTESIAN_POINT ( 'NONE',  ( 4.586363120317823672, -1.655842793181455663, -0.6244342276643227718 ) ) ;
#1110=CARTESIAN_POINT ( 'NONE',  ( 3.240066224740343781, -14.18897675264189928, 3.749338592554243288 ) ) ;
#1112=CARTESIAN_POINT ( 'NONE',  ( 4.981054720647222211, 121.2162878128435892, -0.1538846217318251552 ) ) ;
#1113=CARTESIAN_POINT ( 'NONE',  ( -16.46484310285447350, 122.7513851185756693, 0.4780162726406277929 ) ) ;
#1114=CARTESIAN_POINT ( 'NONE',  ( 2.411581292501531415, 38.13423181323310729, 1.422810646954211666 ) ) ;
#1117=CARTESIAN_POINT ( 'NONE',  ( -5.314273266013044505, 104.6144662015457527, 0.4583182832411464291 ) ) ;
#1118=CARTESIAN_POINT ( 'NONE',  ( 4.698461193529555935, -15.58032547337365159, 2.177983573914926030 ) ) ;
#1119=CARTESIAN_POINT ( 'NONE',  ( -8.792132358471173248, 156.9002828235886966, 1.708777300431143731 ) ) ;
#1120=CARTESIAN_POINT ( 'NONE',  ( 0.09481320634720795393, -4.229605868409334057, 4.636458411128852930 ) ) ;
#1123=CARTESIAN_POINT ( 'NONE',  ( 0.3260985403865587773, 116.4813942609866899, 1.528836360202051381 ) ) ;
#1126=CARTESIAN_POINT ( 'NONE',  ( -10.51090385015224804, 123.6668265419868646, 0.9186085726806039187 ) ) ;
#1127=CARTESIAN_POINT ( 'NONE',  ( 4.610436209567292387, 117.9340757871244847, 0.9619774773656434297 ) ) ;
#1128=CARTESIAN_POINT ( 'NONE',  ( 10.01831529487285266, 155.4362223408194836, -1.706801840347523136 ) ) ;
#1129=CARTESIAN_POINT ( 'NONE',  ( -18.06424110348786982, 131.7244750738095149, -2.230326231357608879 ) ) ;
#1131=CIRCLE ( 'NONE', #24910, 0.5080000000000002292 ) ;
#1133=CARTESIAN_POINT ( 'NONE',  ( 4.292225393060463468, 118.2141433220078568, -0.3520200080934876019 ) ) ;
#1134=CARTESIAN_POINT ( 'NONE',  ( 10.62272853480718204, 153.0636280899912549, -0.4455235322555908817 ) ) ;
#1137=AXIS2_PLACEMENT_3D ( 'NONE', #21480, #17672, #24694 ) ;
#1138=CARTESIAN_POINT ( 'NONE',  ( 3.189131052002434963, -14.84934909478852205, 3.295817422932660890 ) ) ;
#1141=CARTESIAN_POINT ( 'NONE',  ( -4.422273941422524501, 8.986318502778324557, 1.404945367500548548 ) ) ;
#1142=CARTESIAN_POINT ( 'NONE',  ( 16.09426298050571802, 139.8573806175465961, 2.037321532313223660 ) ) ;
#1143=CARTESIAN_POINT ( 'NONE',  ( -2.585859724564241180, 30.03814370764511565, 1.303285975734316926 ) ) ;
#1144=CARTESIAN_POINT ( 'NONE',  ( -4.544942180623752215, 12.81246518813932589, 0.8472608254572608910 ) ) ;
#1145=CARTESIAN_POINT ( 'NONE',  ( 10.21163942101050459, 125.9885856776569426, 0.2414886939513459507 ) ) ;
#1149=CARTESIAN_POINT ( 'NONE',  ( -8.786561437352411019, 117.7207579526419607, -0.3770129002165002463 ) ) ;
#1151=CARTESIAN_POINT ( 'NONE',  ( 0.001261869788231272235, 124.3520329708341876, -0.06314912420803690807 ) ) ;
#1153=CARTESIAN_POINT ( 'NONE',  ( -0.4039975341914995299, 105.7852372210178942, 5.327039100247182191 ) ) ;
#1155=CARTESIAN_POINT ( 'NONE',  ( -3.946719713907086202, 4.502433826932805694, 7.497755479828382086 ) ) ;
#1156=CARTESIAN_POINT ( 'NONE',  ( 5.293178828769798727, 115.7029491485453150, 0.7217268129011673583 ) ) ;
#1159=CARTESIAN_POINT ( 'NONE',  ( 0.06282972276035359016, 111.5577547982949227, -3.144256248693377387 ) ) ;
#1160=CARTESIAN_POINT ( 'NONE',  ( -0.9434990333793340511, 116.6346273530297850, 0.1892539897508100366 ) ) ;
#1165=ADVANCED_FACE ( 'NONE', ( #20864 ), #5547, .T. ) ;
#1167=CARTESIAN_POINT ( 'NONE',  ( -0.6407465451154844560, 156.3034662015456888, -0.04018040219424089815 ) ) ;
#1168=CARTESIAN_POINT ( 'NONE',  ( 2.663097075550662662, -15.49037753074605739, 5.782289944512356783 ) ) ;
#1169=CARTESIAN_POINT ( 'NONE',  ( -15.01775385910461935, 123.1914926142276130, 1.125269324988862119 ) ) ;
#1170=CARTESIAN_POINT ( 'NONE',  ( -0.003746264460362601790, 116.6481217037470373, 0.1874783927187337884 ) ) ;
#1171=ADVANCED_FACE ( 'NONE', ( #21692 ), #34448, .T. ) ;
#1172=CARTESIAN_POINT ( 'NONE',  ( 9.009615515465577928, 124.1466948585039489, 0.3142177148139755349 ) ) ;
#1173=CARTESIAN_POINT ( 'NONE',  ( -2.201963191602333225, 30.07953629247752758, -4.075912811544394998 ) ) ;
#1174=CARTESIAN_POINT ( 'NONE',  ( -0.8573366540693068139, -6.603747334586292261, -0.4721712316449505620 ) ) ;
#1175=CARTESIAN_POINT ( 'NONE',  ( -16.12231377365586127, 121.3783152868344075, -0.5570369914769760511 ) ) ;
#1176=CARTESIAN_POINT ( 'NONE',  ( -4.856487665647835961, 117.8020098535915565, 0.7286641668683947470 ) ) ;
#1179=CARTESIAN_POINT ( 'NONE',  ( 8.773387014951435248, 117.7735162837325760, 0.4949019102697145844 ) ) ;
#1180=CARTESIAN_POINT ( 'NONE',  ( -11.08663849088108222, 154.4909003399924643, 1.626836423318808622 ) ) ;
#1182=CARTESIAN_POINT ( 'NONE',  ( 12.54292998015191962, 122.5542284311838870, -1.320227961537941086 ) ) ;
#1183=CARTESIAN_POINT ( 'NONE',  ( 0.7467592606654794851, -15.18718160513664195, -0.6397234560659120772 ) ) ;
#1184=CARTESIAN_POINT ( 'NONE',  ( -5.008743879648553055, 158.5910778905036977, -1.550406713891092192 ) ) ;
#1188=CARTESIAN_POINT ( 'NONE',  ( 4.303750855738976533, 104.6144662015456817, 2.191315714953503857 ) ) ;
#1189=CARTESIAN_POINT ( 'NONE',  ( 14.53352838467438524, 150.4300676932417389, -1.118949361739814519 ) ) ;
#1191=CARTESIAN_POINT ( 'NONE',  ( -9.538359384048678891, 124.8019839352694476, -0.1905991205270208266 ) ) ;
#1193=CARTESIAN_POINT ( 'NONE',  ( -11.58192335640140236, 123.0696236843973281, -1.706247406239837394 ) ) ;
#1194=CARTESIAN_POINT ( 'NONE',  ( 3.016856305723133236, -15.72087675955979869, 4.784217253217923016 ) ) ;
#1196=CARTESIAN_POINT ( 'NONE',  ( -4.512655319704103718, 118.1197172503268291, -0.6560251278375922590 ) ) ;
#1199=CARTESIAN_POINT ( 'NONE',  ( 4.108387141429195033, 118.2429491485453354, 0.3498641417436846868 ) ) ;
#1200=CARTESIAN_POINT ( 'NONE',  ( 10.24420426168399700, 122.2012759285571946, 1.550633339661970700 ) ) ;
#1201=CARTESIAN_POINT ( 'NONE',  ( -0.09153888643297225514, 38.16702564188061331, -1.140315812098650960 ) ) ;
#1202=CARTESIAN_POINT ( 'NONE',  ( 9.820189317990141831, 117.9942579372833933, 0.1809356799706722807 ) ) ;
#1203=CARTESIAN_POINT ( 'NONE',  ( 5.972130579385131810, 18.43406553185754504, -5.949252452957764170 ) ) ;
#1204=CARTESIAN_POINT ( 'NONE',  ( 15.64569453857172654, 147.5723176251010784, 0.9037163853702846472 ) ) ;
#1207=CARTESIAN_POINT ( 'NONE',  ( 15.30245393414157284, 121.3917326167944708, -0.5382413912410556334 ) ) ;
#1212=CARTESIAN_POINT ( 'NONE',  ( -15.89375338022620809, 121.0219768425927214, -0.2124277663179632014 ) ) ;
#1213=VERTEX_POINT ( 'NONE', #5340 ) ;
#1215=CARTESIAN_POINT ( 'NONE',  ( -6.899851155630319255, 121.8351476159203770, -0.4925943478833076372 ) ) ;
#1217=EDGE_LOOP ( 'NONE', ( #24235, #36966, #30547, #19520 ) ) ;
#1218=LINE ( 'NONE', #17379, #11060 ) ;
#1219=CARTESIAN_POINT ( 'NONE',  ( -15.84614414026255069, 146.9522167609303267, -0.9100203137935937159 ) ) ;
#1220=CARTESIAN_POINT ( 'NONE',  ( 4.676120195389507295, -12.14821529611620576, 1.449936329584695649 ) ) ;
#1221=CARTESIAN_POINT ( 'NONE',  ( -5.873718653373209975, 117.7475948868982698, 0.6546600694323945202 ) ) ;
#1223=CARTESIAN_POINT ( 'NONE',  ( 20.69515314362131519, 152.5608647341385335, 0.4887519660486651651 ) ) ;
#1224=EDGE_CURVE ( 'NONE', #33842, #2737, #27448, .T. ) ;
#1226=CARTESIAN_POINT ( 'NONE',  ( 2.522041008973656240, -3.380034811851383214, 3.874746376371965617 ) ) ;
#1227=CARTESIAN_POINT ( 'NONE',  ( -0.2932902739210894727, 116.4254261620736344, -0.01852769337193111918 ) ) ;
#1230=EDGE_CURVE ( 'NONE', #35682, #41397, #37280, .T. ) ;
#1231=AXIS2_PLACEMENT_3D ( 'NONE', #689, #10669, #23433 ) ;
#1232=VERTEX_POINT ( 'NONE', #4926 ) ;
#1233=CARTESIAN_POINT ( 'NONE',  ( 8.148461401976737406, 120.7335647551133917, 1.392322577989073773 ) ) ;
#1234=CARTESIAN_POINT ( 'NONE',  ( 0.9983407785579379023, 1.652274601622760741, 4.518288805521794238 ) ) ;
#1235=CARTESIAN_POINT ( 'NONE',  ( 5.842876937034568563, 117.7475948868982698, 0.8887855332765352001 ) ) ;
#1238=CARTESIAN_POINT ( 'NONE',  ( 14.84487292597011709, 154.6636077862465015, -1.582666667450879583 ) ) ;
#1239=CARTESIAN_POINT ( 'NONE',  ( 1.861163356255745915, -7.643417679262992870, 4.233688895527200735 ) ) ;
#1240=CARTESIAN_POINT ( 'NONE',  ( -10.25083424799711018, 157.8242135995235458, -1.281710951059998660 ) ) ;
#1243=CARTESIAN_POINT ( 'NONE',  ( -2.805605324221295938, 120.9854572005495044, 0.04483369291007284485 ) ) ;
#1244=CARTESIAN_POINT ( 'NONE',  ( 6.004855586296256931, -14.40561964533282335, 2.074926179989267094 ) ) ;
#1247=CARTESIAN_POINT ( 'NONE',  ( -0.4906820272735821220, 117.9496050520764783, -1.406625124191804410 ) ) ;
#1248=ORIENTED_EDGE ( 'NONE', *, *, #15383, .T. ) ;
#1249=CARTESIAN_POINT ( 'NONE',  ( 3.283742410131405443, 119.1333808041459577, 0.8926212079385046350 ) ) ;
#1251=B_SPLINE_CURVE_WITH_KNOTS ( 'NONE', 3,
 ( #37493, #15109, #11928, #28112, #40505, #34317, #24488, #37091, #14901, #34727, #41122, #30895 ),
 .UNSPECIFIED., .F., .F.,
 ( 4, 2, 2, 2, 2, 4 ),
 ( 0.6055624778641834904, 0.6081219722606592271, 0.7359737730006136180, 0.8019803297504601858, 0.8679868865003068645, 1.000000000000000000 ),
 .UNSPECIFIED. ) ;
#1252=CARTESIAN_POINT ( 'NONE',  ( 4.756879816653102111, 117.4006788688050449, 1.206942442746047783 ) ) ;
#1253=CARTESIAN_POINT ( 'NONE',  ( -11.23106549681889810, 119.1264784044212632, 0.5965447130870018544 ) ) ;
#1254=CARTESIAN_POINT ( 'NONE',  ( 7.384888961195664514, 14.16877864132934839, -4.050812539764339526 ) ) ;
#1255=CARTESIAN_POINT ( 'NONE',  ( 12.84263471596168138, 130.8243885708800747, 1.276791159582618240 ) ) ;
#1257=CARTESIAN_POINT ( 'NONE',  ( 15.73021646601966239, 121.2535323456646523, -0.2080526303901671648 ) ) ;
#1260=SURFACE_STYLE_FILL_AREA ( #17415 ) ;
#1263=CARTESIAN_POINT ( 'NONE',  ( -4.556770483176405762, 118.1065360176216501, 0.4935596350356394879 ) ) ;
#1267=CARTESIAN_POINT ( 'NONE',  ( 6.165645682523538618, 119.5752110173503695, -1.007953236233805283 ) ) ;
#1268=CARTESIAN_POINT ( 'NONE',  ( -7.499048524201011645, 123.6595150816924047, -0.1842243911843318704 ) ) ;
#1269=CARTESIAN_POINT ( 'NONE',  ( 4.563396916661870861, 118.0729906482839340, 0.7687451279623377376 ) ) ;
#1270=CARTESIAN_POINT ( 'NONE',  ( -9.561025033428087738, 123.8224200044116827, -0.8726585919039497874 ) ) ;
#1271=CARTESIAN_POINT ( 'NONE',  ( -0.06880952194489776963, 115.7029491485453008, -1.763577818935210040 ) ) ;
#1272=CARTESIAN_POINT ( 'NONE',  ( 3.403262595199820773, 117.9496052708406921, -1.151714290375731142 ) ) ;
#1273=CARTESIAN_POINT ( 'NONE',  ( -3.290491044589036740, 30.52917213649525507, -3.264312889705288878 ) ) ;
#1274=CARTESIAN_POINT ( 'NONE',  ( 0.02156534543286487207, 156.6359106937186709, -1.079218069903262300 ) ) ;
#1275=FACE_OUTER_BOUND ( 'NONE', #11841, .T. ) ;
#1277=CARTESIAN_POINT ( 'NONE',  ( 8.799660282941641043, 117.6859426315424599, 0.07877357120233691168 ) ) ;
#1278=CARTESIAN_POINT ( 'NONE',  ( -15.72791684456901962, 146.8976217498096162, -0.1132496748128679204 ) ) ;
#1279=CARTESIAN_POINT ( 'NONE',  ( -6.540217103314379345E-14, 82.64346620154573486, 2.383338306179204368E-29 ) ) ;
#1280=CARTESIAN_POINT ( 'NONE',  ( 2.883180212088789052, 116.9538966677400254, 0.4754005367760563705 ) ) ;
#1282=CARTESIAN_POINT ( 'NONE',  ( 3.009962208777686499, -14.98531826913061771, 3.912431539232285704 ) ) ;
#1283=CARTESIAN_POINT ( 'NONE',  ( -18.71424449056256378, 147.4429432625130119, 1.699796950208447788 ) ) ;
#1284=CARTESIAN_POINT ( 'NONE',  ( 0.9053751552131774627, -6.120233167431497812, -0.3594991891349857416 ) ) ;
#1285=CARTESIAN_POINT ( 'NONE',  ( -13.21954506825633402, 156.9672759736256467, -0.8747755986887105761 ) ) ;
#1286=CARTESIAN_POINT ( 'NONE',  ( 0.1873809172457601979, 14.59626481882237492, -0.9553521702420578743 ) ) ;
#1289=CARTESIAN_POINT ( 'NONE',  ( 1.370820134808094837, 106.2483430537416638, 5.168860673143087503 ) ) ;
#1291=CARTESIAN_POINT ( 'NONE',  ( -5.220694793870528372, 121.0999079655412203, 0.2922795305089894713 ) ) ;
#1292=CARTESIAN_POINT ( 'NONE',  ( 4.658995561375286698, -13.35466759734559083, 3.413121997863386881 ) ) ;
#1293=CARTESIAN_POINT ( 'NONE',  ( 3.531217591821261159, 156.5024071230465097, -1.273243333543745859 ) ) ;
#1297=CARTESIAN_POINT ( 'NONE',  ( 2.821697343786723877, -14.64683725402170289, 4.582568527534213843 ) ) ;
#1298=CARTESIAN_POINT ( 'NONE',  ( -4.963187677402431497, 117.4661819789754986, -0.9730286260216215455 ) ) ;
#1299=CARTESIAN_POINT ( 'NONE',  ( 8.537819074431615363, 123.3353292868209365, 0.08920952957173446107 ) ) ;
#1300=ORIENTED_EDGE ( 'NONE', *, *, #25394, .T. ) ;
#1301=CARTESIAN_POINT ( 'NONE',  ( 1.195985117830443034, 118.4063602595805946, 0.6806364119286733017 ) ) ;
#1302=CARTESIAN_POINT ( 'NONE',  ( 4.258623371604620012, 112.0483952545076818, 2.856521178696663554 ) ) ;
#1303=CARTESIAN_POINT ( 'NONE',  ( -5.517349593794012463, 28.10803576007639037, 0.4164286583522215368 ) ) ;
#1305=CARTESIAN_POINT ( 'NONE',  ( 2.784667331447688632, 116.5968896900294709, -0.09290643507641017929 ) ) ;
#1309=CARTESIAN_POINT ( 'NONE',  ( 1.985468892469562485, -15.55060482525283305, 5.976321803999622873 ) ) ;
#1311=CARTESIAN_POINT ( 'NONE',  ( -2.880736501481947265, 31.22451072257329585, 0.7774695130801791976 ) ) ;
#1312=CARTESIAN_POINT ( 'NONE',  ( 4.042996894205697522, 118.2594131075661608, 0.9467780975002215715 ) ) ;
#1314=CARTESIAN_POINT ( 'NONE',  ( 5.116497545627949783, 15.83618160547830911, 6.690270154343205711 ) ) ;
#1315=CARTESIAN_POINT ( 'NONE',  ( -2.430891878037258813, 117.4063284849774078, -0.7237017793962934320 ) ) ;
#1316=CARTESIAN_POINT ( 'NONE',  ( -2.258874542396802187, 118.3648483361698851, -0.8858652710056678092 ) ) ;
#1317=CARTESIAN_POINT ( 'NONE',  ( 4.957728306477804381, 117.4049568006667670, 1.028863336443936127 ) ) ;
#1318=CARTESIAN_POINT ( 'NONE',  ( -6.507153519498132566E-14, 76.29346620154572634, 3.067795752821199360E-29 ) ) ;
#1320=CARTESIAN_POINT ( 'NONE',  ( 3.728136974946417492, 6.765255174955887796, 2.739693761753763113 ) ) ;
#1322=CARTESIAN_POINT ( 'NONE',  ( -5.276743917130819916, 115.6909491485453003, 0.8116159901532213894 ) ) ;
#1323=CARTESIAN_POINT ( 'NONE',  ( 3.403332384622693052, -13.60094159685824877, 2.654810364998238192 ) ) ;
#1324=CARTESIAN_POINT ( 'NONE',  ( 1.889402974297992754, 108.8931014686503289, -4.028630146538900725 ) ) ;
#1325=CARTESIAN_POINT ( 'NONE',  ( 0.03201377673046572336, 33.52827609515317420, 3.383309648808628278 ) ) ;
#1328=CARTESIAN_POINT ( 'NONE',  ( -3.857386620090222262, 105.1226137608093438, -3.700239550084083895 ) ) ;
#1329=CARTESIAN_POINT ( 'NONE',  ( 1.959965285483297404, -15.65532139403495648, 5.519319896091174904 ) ) ;
#1330=CARTESIAN_POINT ( 'NONE',  ( -12.41883037655689037, 155.1253022143813496, 1.737092194502518616 ) ) ;
#1331=CARTESIAN_POINT ( 'NONE',  ( -3.178183004559932190, -7.902942162671289239, -3.366045245292264010 ) ) ;
#1334=CYLINDRICAL_SURFACE ( 'NONE', #23814, 5.588000000000006295 ) ;
#1335=CARTESIAN_POINT ( 'NONE',  ( 0.2359694434508981808, 106.4201689084969047, 5.118158396747612748 ) ) ;
#1336=CARTESIAN_POINT ( 'NONE',  ( -9.865641862003254658, 123.3250567171901082, 0.7964883383408416506 ) ) ;
#1339=CARTESIAN_POINT ( 'NONE',  ( 11.23500844718012992, 122.9575399027323073, -1.191779604289733285 ) ) ;
#1341=CARTESIAN_POINT ( 'NONE',  ( -13.31282764718934608, 122.3357896625302459, -1.791091420989350258 ) ) ;
#1343=CARTESIAN_POINT ( 'NONE',  ( 4.261500844742492689, 118.2248151516817956, -0.2975339631682852870 ) ) ;
#1344=CARTESIAN_POINT ( 'NONE',  ( 15.59522120955183055, 147.8873989650969918, -0.4103944809294444163 ) ) ;
#1346=CARTESIAN_POINT ( 'NONE',  ( 2.994295736468014280, -14.77441112906794984, 3.968895097548184037 ) ) ;
#1349=CARTESIAN_POINT ( 'NONE',  ( 2.362155674307470310, -13.89060443905824371, -3.983575812745122846 ) ) ;
#1350=CARTESIAN_POINT ( 'NONE',  ( 13.72925640114926082, 131.0408573235120571, 1.723107598632783066 ) ) ;
#1351=CARTESIAN_POINT ( 'NONE',  ( -3.646310357438999894, 28.62608726100145873, 1.835561881698716924 ) ) ;
#1352=CARTESIAN_POINT ( 'NONE',  ( -6.805961295028136071, 123.7298400107579255, -0.09869924339446545236 ) ) ;
#1353=CARTESIAN_POINT ( 'NONE',  ( 3.935102970030661673, 16.48578375386999539, 2.424025302511324309 ) ) ;
#1354=CARTESIAN_POINT ( 'NONE',  ( 5.300740673260364133, 121.3529869156830046, 0.1337733589788159816 ) ) ;
#1359=CARTESIAN_POINT ( 'NONE',  ( -2.174026700015069036, 116.2368718333218425, -0.1864608981796752329 ) ) ;
#1360=CARTESIAN_POINT ( 'NONE',  ( -6.374728672999452917E-14, 124.9344662015457317, 7.707042028354222152E-17 ) ) ;
#1362=CARTESIAN_POINT ( 'NONE',  ( -0.3831293027247411609, 105.9761014636926149, 5.290230343685635717 ) ) ;
#1363=CARTESIAN_POINT ( 'NONE',  ( -2.958531772299361595, 44.28946620154572855, -1.329372033065076675 ) ) ;
#1364=CARTESIAN_POINT ( 'NONE',  ( 5.007560425261973869, -3.380029175189206203, 6.774419414089246416 ) ) ;
#1366=FACE_OUTER_BOUND ( 'NONE', #35222, .T. ) ;
#1369=CARTESIAN_POINT ( 'NONE',  ( -4.973569738608247803, 117.3993868453981548, -0.9750659555622913643 ) ) ;
#1370=CARTESIAN_POINT ( 'NONE',  ( -13.44960824739634653, 119.6710471929552000, 0.1296808650140444663 ) ) ;
#1373=CARTESIAN_POINT ( 'NONE',  ( -5.078986093043185157, 72.99146620154573384, -0.1014902294541238092 ) ) ;
#1376=CARTESIAN_POINT ( 'NONE',  ( -6.503408402854686798, 121.7799126398724354, -0.1299535771408516782 ) ) ;
#1377=CARTESIAN_POINT ( 'NONE',  ( 5.498554953534677381, -14.76196523188227872, 3.265392988355040327 ) ) ;
#1378=CARTESIAN_POINT ( 'NONE',  ( -19.52548538990948757, 136.0480396440595996, 1.529100095608182830 ) ) ;
#1379=CARTESIAN_POINT ( 'NONE',  ( 15.93800727448848065, 121.3860667298135070, 0.7466885930842024344 ) ) ;
#1380=CARTESIAN_POINT ( 'NONE',  ( 20.36908824613697888, 132.1502320877631007, -0.7851131432546852862 ) ) ;
#1382=CARTESIAN_POINT ( 'NONE',  ( -21.88244685892446384, 151.4414241944827495, -0.6640443303913105000 ) ) ;
#1385=CARTESIAN_POINT ( 'NONE',  ( 4.973153348176213129, 117.3993868326347183, 0.9753024067320210655 ) ) ;
#1387=CARTESIAN_POINT ( 'NONE',  ( -2.184846125065896150, 116.1979711210248780, -0.02027492182686356156 ) ) ;
#1388=CARTESIAN_POINT ( 'NONE',  ( -3.455858276899955950, 119.9243055703230851, 0.6230356542855080004 ) ) ;
#1390=CARTESIAN_POINT ( 'NONE',  ( 19.63947405400084634, 148.8045834396381508, -1.723899180582558088 ) ) ;
#1391=CARTESIAN_POINT ( 'NONE',  ( 0.9474642044963531573, -6.343762114497205395, -0.2236011429025598352 ) ) ;
#1392=CARTESIAN_POINT ( 'NONE',  ( -14.34163035669555164, 121.9874158357064857, -1.600522166921893863 ) ) ;
#1394=AXIS2_PLACEMENT_3D ( 'NONE', #3654, #3026, #12796 ) ;
#1395=CARTESIAN_POINT ( 'NONE',  ( 12.75300196040200085, 152.1353413313561305, -1.119124812251137469 ) ) ;
#1396=CARTESIAN_POINT ( 'NONE',  ( -9.118174893680297544, 124.1671967267183589, -0.1822028344259497834 ) ) ;
#1398=CARTESIAN_POINT ( 'NONE',  ( -1.339510839693951239, 119.4570717772418220, -0.6353817622545779864 ) ) ;
#1399=CARTESIAN_POINT ( 'NONE',  ( 4.776532240430319654, -15.60394515218366251, 2.960345780779299663 ) ) ;
#1401=CARTESIAN_POINT ( 'NONE',  ( -4.350331169090538630, 118.1836411042714019, -0.6150010472375504467 ) ) ;
#1405=CARTESIAN_POINT ( 'NONE',  ( -0.02969003158484915736, 157.1787724364823760, 1.485810588193620774 ) ) ;
#1408=CARTESIAN_POINT ( 'NONE',  ( 5.772319165917887851, 116.9338547871927858, 0.1153446742911717754 ) ) ;
#1410=CARTESIAN_POINT ( 'NONE',  ( 6.774419413954826830, 18.20997082500984376, -5.007560425318187569 ) ) ;
#1411=CARTESIAN_POINT ( 'NONE',  ( 14.33905310436362690, 139.0340687859245463, 0.7442083991839667512 ) ) ;
#1412=CARTESIAN_POINT ( 'NONE',  ( 2.940475496281206969, 117.1197906563906344, -0.4390297717439133884 ) ) ;
#1417=CARTESIAN_POINT ( 'NONE',  ( -17.27060146982332611, 122.7565812399420651, -0.2921901055230265998 ) ) ;
#1418=ORIENTED_EDGE ( 'NONE', *, *, #18535, .T. ) ;
#1420=CARTESIAN_POINT ( 'NONE',  ( -5.784570514964185506, 121.1847750061955793, -0.5060016832306288848 ) ) ;
#1423=CARTESIAN_POINT ( 'NONE',  ( 3.987297185843972080, 118.7629491485453741, -0.9448535219813100072 ) ) ;
#1424=CARTESIAN_POINT ( 'NONE',  ( -8.876935545690720630, 123.7004864364556909, -0.3337242414277967750 ) ) ;
#1425=CARTESIAN_POINT ( 'NONE',  ( 2.039565395400614989, -15.13835760176744571, 5.886961163765535687 ) ) ;
#1426=CARTESIAN_POINT ( 'NONE',  ( -19.32406529451199262, 152.1947311750261065, 1.288948053361433255 ) ) ;
#1428=CARTESIAN_POINT ( 'NONE',  ( 17.22116264704559541, 122.7389118244895769, 0.4537515290936993684 ) ) ;
#1429=CARTESIAN_POINT ( 'NONE',  ( 15.37911286811759659, 147.8337517708649500, 0.3739466042392066147 ) ) ;
#1431=CARTESIAN_POINT ( 'NONE',  ( 3.501419995798253915, -2.955197114699519734, 3.043391175950921568 ) ) ;
#1432=CARTESIAN_POINT ( 'NONE',  ( -4.716951831472304235, 116.7562497393984415, -0.1081823505139635905 ) ) ;
#1433=DIRECTION ( 'NONE',  ( -0.9998004120163608288, 0.000000000000000000, -0.01997839162482747608 ) ) ;
#1434=EDGE_LOOP ( 'NONE', ( #35582, #8226, #15104, #26764, #32645, #9848, #37142, #40822, #14935, #33892, #11987, #1585, #611 ) ) ;
#1435=CARTESIAN_POINT ( 'NONE',  ( 6.391738861559880469, 119.5489620839046410, 1.259756172207089575 ) ) ;
#1436=( BOUNDED_CURVE ( )  B_SPLINE_CURVE ( 3, ( #33648, #13827, #33854, #14649 ),
 .UNSPECIFIED., .F., .F. ) 
 B_SPLINE_CURVE_WITH_KNOTS ( ( 4, 4 ),
 ( 0.09183118002780921163, 0.1539179638657816873 ),
 .UNSPECIFIED. ) 
 CURVE ( )  GEOMETRIC_REPRESENTATION_ITEM ( )  RATIONAL_B_SPLINE_CURVE ( ( 0.7001390048907335517, 0.6477646404348715858, 0.6056696592518493460, 0.5738540613416668323 ) ) 
 REPRESENTATION_ITEM ( '' )  );
#1437=CARTESIAN_POINT ( 'NONE',  ( -4.626086514281606554, -10.66701884381306087, 0.02375484599842511355 ) ) ;
#1438=CARTESIAN_POINT ( 'NONE',  ( 0.3664415811650883481, 117.3568105388816321, 0.4447864970249673089 ) ) ;
#1440=CARTESIAN_POINT ( 'NONE',  ( 20.67621894907592051, 148.5655811199389689, -1.615315227278341315 ) ) ;
#1441=CARTESIAN_POINT ( 'NONE',  ( -4.626086514281606554, -10.66701884381306087, 0.02375484599842511355 ) ) ;
#1442=CARTESIAN_POINT ( 'NONE',  ( -4.843103592331963192, 117.3073154462328063, -0.6875571908837336821 ) ) ;
#1446=CARTESIAN_POINT ( 'NONE',  ( -12.97778284513273483, 133.8854804328748571, -0.04088747601382857616 ) ) ;
#1447=CARTESIAN_POINT ( 'NONE',  ( 4.031817627494778122, -15.29123897636591778, 5.054998095871475527 ) ) ;
#1448=EDGE_CURVE ( 'NONE', #40423, #2340, #26112, .T. ) ;
#1451=CARTESIAN_POINT ( 'NONE',  ( -3.409246530723191171, 109.2372022974443126, -3.913087349919080804 ) ) ;
#1453=CARTESIAN_POINT ( 'NONE',  ( 14.93497932922872629, 152.9649416503947634, 2.345758529409812887 ) ) ;
#1456=CARTESIAN_POINT ( 'NONE',  ( -9.536130858166004032, 118.4542681464805298, 0.5810392422064989404 ) ) ;
#1457=EDGE_CURVE ( 'NONE', #26787, #35651, #16578, .T. ) ;
#1458=CARTESIAN_POINT ( 'NONE',  ( -8.331803066987694351, 8.350395779143005015, -1.420432620954584113 ) ) ;
#1459=CARTESIAN_POINT ( 'NONE',  ( 14.07483374865158687, 150.3034377993741657, 1.364178037702376223 ) ) ;
#1461=CARTESIAN_POINT ( 'NONE',  ( 22.79600589338267369, 150.0845277111093310, -0.2694608383616128311 ) ) ;
#1465=( NAMED_UNIT ( * ) SI_UNIT ( $, .STERADIAN. ) SOLID_ANGLE_UNIT ( ) );
#1469=CARTESIAN_POINT ( 'NONE',  ( -4.164425106054416403, 118.2394406760751622, 0.2263534819914557739 ) ) ;
#1470=CARTESIAN_POINT ( 'NONE',  ( 3.264763291910224741, 108.5668738132266071, -4.052445894262588055 ) ) ;
#1473=CARTESIAN_POINT ( 'NONE',  ( 6.184646281355417941, 119.6155407647441962, -1.003826558285236592 ) ) ;
#1474=CARTESIAN_POINT ( 'NONE',  ( -5.245364206137289820, 116.4655405006298849, -1.092799426751067005 ) ) ;
#1476=CARTESIAN_POINT ( 'NONE',  ( 4.299732312588651517, 118.2124281450362133, 0.4976895454704568511 ) ) ;
#1477=CARTESIAN_POINT ( 'NONE',  ( -9.839787852217179775, 124.1914461168675530, -0.8951504484210819346 ) ) ;
#1478=CARTESIAN_POINT ( 'NONE',  ( -0.7903546951415685307, 115.7028259477297922, -1.754549543117774446 ) ) ;
#1479=FACE_OUTER_BOUND ( 'NONE', #26209, .T. ) ;
#1480=ORIENTED_EDGE ( 'NONE', *, *, #26494, .F. ) ;
#1481=CARTESIAN_POINT ( 'NONE',  ( 3.592701615362551504, 108.6576027043044377, -3.989964801148524476 ) ) ;
#1482=CARTESIAN_POINT ( 'NONE',  ( -2.639528505629704647, 120.4390018212493914, -0.4929570044210888624 ) ) ;
#1483=CARTESIAN_POINT ( 'NONE',  ( -4.705839724742440389, 116.0444662015457595, 3.565396701626624143 ) ) ;
#1486=CARTESIAN_POINT ( 'NONE',  ( -9.426429330012480179, 124.7671717571762429, -0.04963531977156410840 ) ) ;
#1487=CARTESIAN_POINT ( 'NONE',  ( 4.349802767100347189, -10.92635770930747796, -1.576909098649299512 ) ) ;
#1488=CARTESIAN_POINT ( 'NONE',  ( 1.924101685567825903, 116.8467566806161386, 0.3833193769953583963 ) ) ;
#1490=CARTESIAN_POINT ( 'NONE',  ( 2.915559332840946816, -14.19431184016030301, 0.3483797586856177686 ) ) ;
#1491=CARTESIAN_POINT ( 'NONE',  ( 13.78108617287050564, 121.3979351292862816, -1.006787891297146409 ) ) ;
#1492=CARTESIAN_POINT ( 'NONE',  ( -2.445625216771193156, 119.3768144667271542, 0.6598031440805112169 ) ) ;
#1493=AXIS2_PLACEMENT_3D ( 'NONE', #33530, #39926, #36719 ) ;
#1494=CARTESIAN_POINT ( 'NONE',  ( -0.7897743334665792148, -0.9462621144725560374, 0.5691593732151654095 ) ) ;
#1495=CARTESIAN_POINT ( 'NONE',  ( -13.27770485956329694, 119.7426348059052685, -0.8357656065649388122 ) ) ;
#1496=CARTESIAN_POINT ( 'NONE',  ( 0.5056692551311988693, 10.92592451650425112, 0.8332994872028685052 ) ) ;
#1500=CARTESIAN_POINT ( 'NONE',  ( -8.332953031246923103, 122.7091975629380585, 0.3740907431100291003 ) ) ;
#1501=CARTESIAN_POINT ( 'NONE',  ( 3.638845723804262189, -14.60113053194242383, 5.212470003951681363 ) ) ;
#1502=CARTESIAN_POINT ( 'NONE',  ( 0.8386157876099215036, 156.7682548876429109, -1.206618248707299834 ) ) ;
#1505=CARTESIAN_POINT ( 'NONE',  ( 4.553366535818831551, 104.6144662015457811, 1.608775678111619145 ) ) ;
#1507=CARTESIAN_POINT ( 'NONE',  ( 3.258219809910011033, -14.04213616937880005, 2.843395319141139410 ) ) ;
#1508=CARTESIAN_POINT ( 'NONE',  ( -4.894673311264758020, 117.5446123977157100, -1.081256949576274273 ) ) ;
#1510=CARTESIAN_POINT ( 'NONE',  ( 7.045353508903499318, 122.0728772437221323, 0.1110369332536843695 ) ) ;
#1512=CARTESIAN_POINT ( 'NONE',  ( 20.12154232503847595, 149.0333503175929479, 2.470054797493932419 ) ) ;
#1513=CARTESIAN_POINT ( 'NONE',  ( 5.084164759140180401, 114.9388725758527272, 1.737832868923124607 ) ) ;
#1516=CARTESIAN_POINT ( 'NONE',  ( 0.03256023585714045571, 157.9544661776888290, -1.629447346748784220 ) ) ;
#1517=CARTESIAN_POINT ( 'NONE',  ( 6.908764576387254941, 117.1865127098105575, 0.01035743554829997824 ) ) ;
#1520=CARTESIAN_POINT ( 'NONE',  ( 1.910917866030142909, -15.65413017954154995, 5.882152347191063058 ) ) ;
#1521=CARTESIAN_POINT ( 'NONE',  ( 4.862091962581056137, 117.4116108956684030, 1.165648838277617338 ) ) ;
#1522=CARTESIAN_POINT ( 'NONE',  ( 1.534760489240974080, 36.16307923083526532, -0.6549077602738699877 ) ) ;
#1523=CARTESIAN_POINT ( 'NONE',  ( -4.629600663469410904, 117.9777096712006852, 0.7347564628851412927 ) ) ;
#1525=CARTESIAN_POINT ( 'NONE',  ( -8.041749784432907333, 11.96416136180153345, -2.598976288244244870 ) ) ;
#1526=CARTESIAN_POINT ( 'NONE',  ( 5.875440716348254711, 118.9244925334023151, -1.017365677016041081 ) ) ;
#1527=CARTESIAN_POINT ( 'NONE',  ( -2.364009027793917195, 119.4803856251332945, -0.6315868319338824310 ) ) ;
#1528=CARTESIAN_POINT ( 'NONE',  ( 4.895718167919051567, 117.6590296544187737, 0.9622844256249989403 ) ) ;
#1530=CARTESIAN_POINT ( 'NONE',  ( -0.01386859376332154337, 119.8383472832138779, 0.6940411431075991233 ) ) ;
#1532=CARTESIAN_POINT ( 'NONE',  ( -3.234384296441582762, 11.31316835407710819, -3.315160845070126427 ) ) ;
#1535=CARTESIAN_POINT ( 'NONE',  ( 2.317735183313462066, -14.86924938851764999, 5.343245562499194357 ) ) ;
#1536=CARTESIAN_POINT ( 'NONE',  ( 4.687267571633873864, 120.2198808273567892, -0.2753304537621711900 ) ) ;
#1537=CARTESIAN_POINT ( 'NONE',  ( -0.2179416487220206811, 33.83400432488151210, 3.531833526404775103 ) ) ;
#1538=CARTESIAN_POINT ( 'NONE',  ( -0.6554515820231663348, 115.7029491485453150, 1.735612802329033810 ) ) ;
#1540=CARTESIAN_POINT ( 'NONE',  ( -3.197619535514014011, 105.1239064336704985, -4.271075346114246329 ) ) ;
#1541=CARTESIAN_POINT ( 'NONE',  ( 5.270497567351643653, -15.36183412081716604, 0.7307456425073816098 ) ) ;
#1542=CARTESIAN_POINT ( 'NONE',  ( -19.87863739466945745, 147.4002846799066333, 1.728157425434577510 ) ) ;
#1543=CARTESIAN_POINT ( 'NONE',  ( -0.2773724154211913984, 24.90860930217742464, 0.9350043038818249830 ) ) ;
#1545=CIRCLE ( 'NONE', #9013, 3.683000000000001162 ) ;
#1548=CARTESIAN_POINT ( 'NONE',  ( 2.900991945634675773, 122.3314979878274045, 0.2533474610292540952 ) ) ;
#1550=CARTESIAN_POINT ( 'NONE',  ( -12.65121035427621266, 128.4643691153342218, 0.9906145297030367614 ) ) ;
#1552=CARTESIAN_POINT ( 'NONE',  ( 4.562811221412711227, 118.0737936952979794, -0.6153291334979017480 ) ) ;
#1553=CARTESIAN_POINT ( 'NONE',  ( 9.634306097685872317, 155.2307989660268959, -1.622952429610069247 ) ) ;
#1554=CARTESIAN_POINT ( 'NONE',  ( -9.074718672963452804, 157.1510513929294177, -1.991881423077542568 ) ) ;
#1557=CARTESIAN_POINT ( 'NONE',  ( 4.394285435036319853, 118.1841684474106984, -0.4164588777813547638 ) ) ;
#1558=CARTESIAN_POINT ( 'NONE',  ( 2.776805996813493049, 120.9068798055765370, -0.1259499506852532758 ) ) ;
#1560=CARTESIAN_POINT ( 'NONE',  ( 3.216763585201820153, -14.58149021785123978, 2.832987347109013676 ) ) ;
#1566=CARTESIAN_POINT ( 'NONE',  ( -1.319288878716189828, -8.717950886928733212, 4.428293336331323715 ) ) ;
#1567=CARTESIAN_POINT ( 'NONE',  ( 16.85437733762575618, 144.1809451582817587, 2.058110026898294365 ) ) ;
#1568=CARTESIAN_POINT ( 'NONE',  ( -2.299720509168451166, 30.37513842844993306, 3.096482033432269354 ) ) ;
#1569=CARTESIAN_POINT ( 'NONE',  ( -6.118667329350094164, 121.4157903421748301, 0.08376844782033875114 ) ) ;
#1570=CARTESIAN_POINT ( 'NONE',  ( 4.586363120317823672, -1.655842793181455663, -0.6244342276643227718 ) ) ;
#1571=CARTESIAN_POINT ( 'NONE',  ( 2.828086164579441952, 121.0305217392013759, 0.08274239724663745577 ) ) ;
#1575=CARTESIAN_POINT ( 'NONE',  ( 8.792662243298641656, 117.7335494595113943, -0.05956412395685332928 ) ) ;
#1576=CARTESIAN_POINT ( 'NONE',  ( 0.006734421714204561794, 121.9236798544229003, -0.3370180007450780391 ) ) ;
#1578=CARTESIAN_POINT ( 'NONE',  ( -2.178937547604698377, 106.5591908312060667, 4.866054723391081360 ) ) ;
#1580=CARTESIAN_POINT ( 'NONE',  ( 8.101632580580826470, 8.064395906452419993, -2.298819013970823999 ) ) ;
#1584=CARTESIAN_POINT ( 'NONE',  ( -0.008148259816615344500, 159.5682499516715040, 0.4077722408685187649 ) ) ;
#1585=ORIENTED_EDGE ( 'NONE', *, *, #14881, .T. ) ;
#1590=CARTESIAN_POINT ( 'NONE',  ( -13.59117098933512580, 150.2425924485890505, -0.2715839415562138481 ) ) ;
#1591=CARTESIAN_POINT ( 'NONE',  ( 2.665431962039443992, -15.40910046105366327, 5.814861676232141008 ) ) ;
#1592=CARTESIAN_POINT ( 'NONE',  ( -6.811759424595843271, 118.6475953829349379, 0.9158128249201543669 ) ) ;
#1594=CARTESIAN_POINT ( 'NONE',  ( 0.007599820978683539778, 117.2191897141855179, -0.3803261187632671625 ) ) ;
#1595=CARTESIAN_POINT ( 'NONE',  ( -2.707926769430928804, 11.08828375386998033, -3.745406074561137721 ) ) ;
#1596=CARTESIAN_POINT ( 'NONE',  ( -4.752142575032330285, 116.8068435238802465, -0.2604826270010437983 ) ) ;
#1598=VERTEX_POINT ( 'NONE', #17104 ) ;
#1599=CARTESIAN_POINT ( 'NONE',  ( 8.798071512540863282, 117.6842349196870572, 0.1758064070670784795 ) ) ;
#1600=CARTESIAN_POINT ( 'NONE',  ( -8.228482648312640535, 121.2453320564195280, 0.9666412201339350529 ) ) ;
#1603=CARTESIAN_POINT ( 'NONE',  ( 3.289525010481779255, 118.9727644790723531, -0.7721065173366223888 ) ) ;
#1604=CARTESIAN_POINT ( 'NONE',  ( -1.109551233970537343, 117.7697124030934077, -0.5969493375118321010 ) ) ;
#1607=CARTESIAN_POINT ( 'NONE',  ( 4.453624852893700137, 120.7762672505206041, -0.3811677228292793540 ) ) ;
#1608=ORIENTED_EDGE ( 'NONE', *, *, #24547, .F. ) ;
#1609=CARTESIAN_POINT ( 'NONE',  ( -17.79834178490407481, 144.5560955566678558, -2.349204209454022863 ) ) ;
#1610=CARTESIAN_POINT ( 'NONE',  ( 4.535010020878385895, -15.35856548043400238, 0.06517018677027014428 ) ) ;
#1611=CARTESIAN_POINT ( 'NONE',  ( -4.374336409094900624, 118.1842338761308753, -0.5915268427067872370 ) ) ;
#1614=CARTESIAN_POINT ( 'NONE',  ( -4.958806897238241085, 117.4102282907815606, 0.9054230299057887121 ) ) ;
#1615=CARTESIAN_POINT ( 'NONE',  ( 11.01279815837308895, 154.4909003399924643, 2.068435761307119147 ) ) ;
#1618=CARTESIAN_POINT ( 'NONE',  ( 10.83072783392011651, 157.9016520041087688, 0.1964268902508807535 ) ) ;
#1619=CARTESIAN_POINT ( 'NONE',  ( -5.777836206968382626, 13.68815862607732825, 6.147148275823971275 ) ) ;
#1620=CARTESIAN_POINT ( 'NONE',  ( 15.83982646870413191, 146.6055793175013093, 0.7699162700945606508 ) ) ;
#1624=CARTESIAN_POINT ( 'NONE',  ( -8.016647455044246584, 121.3928899876477772, -1.222747983602104904 ) ) ;
#1627=CARTESIAN_POINT ( 'NONE',  ( -13.64797835309731866, 119.6379125180634446, -0.1726152169769648581 ) ) ;
#1630=CARTESIAN_POINT ( 'NONE',  ( 6.874218592591693877, 121.5427147135433046, -0.4735844615521632717 ) ) ;
#1631=CARTESIAN_POINT ( 'NONE',  ( -8.366466113708746377, 119.9145198431060777, 1.112176479753330227 ) ) ;
#1633=ORIENTED_EDGE ( 'NONE', *, *, #10977, .F. ) ;
#1634=CARTESIAN_POINT ( 'NONE',  ( 0.5927366764262057552, 115.7030772134404799, -1.739505766195229564 ) ) ;
#1635=CARTESIAN_POINT ( 'NONE',  ( -9.155891339183989786, 123.9989874199980022, -0.4132670667758963079 ) ) ;
#1636=CARTESIAN_POINT ( 'NONE',  ( 4.246535372682106235, -13.89508586689386327, 4.277860383763752772 ) ) ;
#1637=CARTESIAN_POINT ( 'NONE',  ( -14.33513709642007861, 121.5541609676003389, 0.9327927267376099341 ) ) ;
#1639=CARTESIAN_POINT ( 'NONE',  ( 22.65355654554102216, 150.6414900647796173, 0.6056372710714960084 ) ) ;
#1640=CARTESIAN_POINT ( 'NONE',  ( 9.499210638188102962, 124.7903824246305362, 0.2360490693302050025 ) ) ;
#1641=ORIENTED_EDGE ( 'NONE', *, *, #10958, .F. ) ;
#1642=CARTESIAN_POINT ( 'NONE',  ( 0.7259983000635549244, 26.63096242550804860, 0.6518668477890779966 ) ) ;
#1644=CARTESIAN_POINT ( 'NONE',  ( -15.19377495473410811, 156.0906695176550443, -0.3258312939631710647 ) ) ;
#1646=DIRECTION ( 'NONE',  ( -0.9998004120163609398, -4.016384292689130894E-17, -0.01997839162482749689 ) ) ;
#1647=ORIENTED_EDGE ( 'NONE', *, *, #28787, .T. ) ;
#1648=CARTESIAN_POINT ( 'NONE',  ( 8.481912912939511884, 119.1148186440260588, 1.316834002904183620 ) ) ;
#1650=CARTESIAN_POINT ( 'NONE',  ( 20.53318969041745490, 136.3738900553462372, 2.061127768630951707 ) ) ;
#1652=CARTESIAN_POINT ( 'NONE',  ( 9.147047865982747439, 157.1510513929294177, -1.627767162235162379 ) ) ;
#1654=CARTESIAN_POINT ( 'NONE',  ( -8.398906084147393258, 18.04027321918359306, -0.8732425085428288103 ) ) ;
#1655=CARTESIAN_POINT ( 'NONE',  ( -9.442718531279867378, 118.5748184150550060, -1.042386753229704865 ) ) ;
#1656=CARTESIAN_POINT ( 'NONE',  ( 4.935068106205077854, 117.6551405386727538, -0.7499101476925047471 ) ) ;
#1658=CARTESIAN_POINT ( 'NONE',  ( -13.63867282259138669, 150.2122286517991085, 0.04772847129159333429 ) ) ;
#1659=CARTESIAN_POINT ( 'NONE',  ( 3.586901592285024698, -15.56753269123677086, 5.192771612050266050 ) ) ;
#1660=CARTESIAN_POINT ( 'NONE',  ( -6.263959367015712765, 28.84083519579221999, 0.1566845698765544637 ) ) ;
#1661=CIRCLE ( 'NONE', #9133, 3.175000000000001155 ) ;
#1662=CARTESIAN_POINT ( 'NONE',  ( -0.1787238347214931966, 117.9496057287605595, -1.408787723444971274 ) ) ;
#1664=CARTESIAN_POINT ( 'NONE',  ( 7.562035183886194112, 119.9600249249614592, 1.380075063195379315 ) ) ;
#1668=CARTESIAN_POINT ( 'NONE',  ( -1.918777129854518870, 121.7602717223048501, 0.2400857948923555418 ) ) ;
#1669=CARTESIAN_POINT ( 'NONE',  ( 8.395564333921381461, 13.51935342844394583, -0.6424836208785561498 ) ) ;
#1670=CARTESIAN_POINT ( 'NONE',  ( 9.559621201325379403, 153.9312916436033447, 1.179784447169990980 ) ) ;
#1671=CARTESIAN_POINT ( 'NONE',  ( -4.782995773917860127, 118.5930653697794384, -0.9660711341386800655 ) ) ;
#1673=CARTESIAN_POINT ( 'NONE',  ( 3.228502273016993218, 159.4348965051207756, -0.3922148187338911351 ) ) ;
#1674=CARTESIAN_POINT ( 'NONE',  ( 4.886022116125724679, 117.7561648045584519, -0.7145573245312663024 ) ) ;
#1678=CARTESIAN_POINT ( 'NONE',  ( -5.078986093043186045, 85.69146620154573668, -0.1014902294541237954 ) ) ;
#1679=CARTESIAN_POINT ( 'NONE',  ( -4.160016578962718370, 118.2392577574570112, 0.2314449875878247520 ) ) ;
#1680=CARTESIAN_POINT ( 'NONE',  ( 4.429857153230104316, 111.0465000998802907, -3.038205857650542630 ) ) ;
#1684=( BOUNDED_CURVE ( )  B_SPLINE_CURVE ( 3, ( #14501, #27516, #36903, #30914 ),
 .UNSPECIFIED., .F., .T. ) 
 B_SPLINE_CURVE_WITH_KNOTS ( ( 4, 4 ),
 ( 0.01144530851284876125, 0.09183118002780921163 ),
 .UNSPECIFIED. ) 
 CURVE ( )  GEOMETRIC_REPRESENTATION_ITEM ( )  RATIONAL_B_SPLINE_CURVE ( ( 0.9552667266446379646, 0.8529924504886332581, 0.7679498765706652685, 0.7001390048907338848 ) ) 
 REPRESENTATION_ITEM ( '' )  );
#1685=CARTESIAN_POINT ( 'NONE',  ( -4.183512250370689856, 119.3195231512375898, -0.9266158876289375401 ) ) ;
#1686=CARTESIAN_POINT ( 'NONE',  ( -5.281229466409689266, 116.7000894413872629, -1.021210189368793264 ) ) ;
#1687=CARTESIAN_POINT ( 'NONE',  ( 4.433936586972705207, 118.1614370034927646, 0.6150725568094654871 ) ) ;
#1688=CARTESIAN_POINT ( 'NONE',  ( -15.91132205781029008, 147.3275361421020193, -1.167720536598260805 ) ) ;
#1691=CARTESIAN_POINT ( 'NONE',  ( -0.8080508600641240768, 24.25718022715097888, 4.550674767031389401 ) ) ;
#1692=CARTESIAN_POINT ( 'NONE',  ( -14.37089176232999321, 134.5679602169015254, -1.683180344383908178 ) ) ;
#1695=CARTESIAN_POINT ( 'NONE',  ( -6.075447103849212382, 121.3874205645395961, 0.1528716657061620909 ) ) ;
#1698=CARTESIAN_POINT ( 'NONE',  ( 22.16805208646083258, 150.4821223471089411, 1.513879355785526570 ) ) ;
#1700=CARTESIAN_POINT ( 'NONE',  ( 3.212496809824684441, -14.25148094350509353, 2.370051959060230473 ) ) ;
#1701=CARTESIAN_POINT ( 'NONE',  ( 10.77577921906383374, 119.6772744462923157, -0.9367561965627279053 ) ) ;
#1702=CARTESIAN_POINT ( 'NONE',  ( -18.70798771669560523, 146.9271955717142930, 1.702497825003243648 ) ) ;
#1703=CARTESIAN_POINT ( 'NONE',  ( 0.8685042297821888857, -7.415843212509670934, 0.4410767154842855642 ) ) ;
#1704=CARTESIAN_POINT ( 'NONE',  ( -3.814135102937820321, 116.8938343318378088, -0.4443717020561034903 ) ) ;
#1706=CARTESIAN_POINT ( 'NONE',  ( 0.7683055643446228267, 21.07255974867073078, 0.6014680952941496850 ) ) ;
#1707=ORIENTED_EDGE ( 'NONE', *, *, #6569, .T. ) ;
#1709=CARTESIAN_POINT ( 'NONE',  ( -0.7006168245644571746, 156.3636429644085695, 0.4970284052464097324 ) ) ;
#1710=CARTESIAN_POINT ( 'NONE',  ( 4.667506617707346983, -11.86120359225895093, 0.9697133514482669803 ) ) ;
#1711=CARTESIAN_POINT ( 'NONE',  ( 10.54966536967459234, 123.3532649940754027, -0.9932924318631478622 ) ) ;
#1712=VERTEX_POINT ( 'NONE', #36305 ) ;
#1713=CARTESIAN_POINT ( 'NONE',  ( 0.4623142775939118598, 115.7034744490966602, 1.762871263781926601 ) ) ;
#1714=CARTESIAN_POINT ( 'NONE',  ( 2.715444768400132158, -14.72438443971033095, 4.720152092698882029 ) ) ;
#1715=CARTESIAN_POINT ( 'NONE',  ( -4.887146391587018357, 117.6636767201053289, -0.9828159811524803668 ) ) ;
#1716=CARTESIAN_POINT ( 'NONE',  ( 7.047330174099000644, 122.0696255612902519, 0.06645725506650276837 ) ) ;
#1719=CARTESIAN_POINT ( 'NONE',  ( 17.72814975036767038, 131.6735282812448986, 2.269257323068798904 ) ) ;
#1720=CYLINDRICAL_SURFACE ( 'NONE', #30618, 3.175000000000001155 ) ;
#1721=CARTESIAN_POINT ( 'NONE',  ( 0.01596947694123658501, 156.4635559983122448, -0.7991779281049287142 ) ) ;
#1722=CARTESIAN_POINT ( 'NONE',  ( 21.48671512862179611, 132.5742979909900328, 0.1330572995313749063 ) ) ;
#1723=CARTESIAN_POINT ( 'NONE',  ( -6.654617103318593247E-14, 104.6144662015457243, 1.534725424433578570E-31 ) ) ;
#1724=CARTESIAN_POINT ( 'NONE',  ( 1.989242623267584165, -15.37180843082167137, 6.016017301631105596 ) ) ;
#1726=CARTESIAN_POINT ( 'NONE',  ( -0.7387659178326329013, 32.94979111317254450, 0.8178967711910589689 ) ) ;
#1728=CARTESIAN_POINT ( 'NONE',  ( -4.711805129293004768, 117.9616559148864781, 0.6918731007553912127 ) ) ;
#1729=VERTEX_POINT ( 'NONE', #7748 ) ;
#1730=EDGE_LOOP ( 'NONE', ( #36348, #16513, #29077, #41244 ) ) ;
#1731=CARTESIAN_POINT ( 'NONE',  ( 5.274109024393328404, 115.7029491485453150, -0.8140283081321303404 ) ) ;
#1732=CARTESIAN_POINT ( 'NONE',  ( 5.647724574261765440, 118.2795828492321704, -0.9363071186805449475 ) ) ;
#1733=CARTESIAN_POINT ( 'NONE',  ( -2.266726881631651036, 118.5759350612125900, -0.8281820106640958024 ) ) ;
#1734=CARTESIAN_POINT ( 'NONE',  ( 4.723834500974907868, 117.6625160859792487, 1.132072396740811060 ) ) ;
#1736=CARTESIAN_POINT ( 'NONE',  ( -0.3766127027002308947, 114.7739974199301116, 2.035987775551920009 ) ) ;
#1737=CARTESIAN_POINT ( 'NONE',  ( 1.616848224653315569, 9.589005055319924864, -4.350374724214612243 ) ) ;
#1738=CARTESIAN_POINT ( 'NONE',  ( 4.980372089298493954, 117.4083386159582005, -0.8694277117261164367 ) ) ;
#1739=CARTESIAN_POINT ( 'NONE',  ( -1.217761333252803224, 106.0671965372247740, -5.195771519815528094 ) ) ;
#1740=CARTESIAN_POINT ( 'NONE',  ( 1.928300050954173450, -15.05328954375542772, 5.649432967411273765 ) ) ;
#1741=CARTESIAN_POINT ( 'NONE',  ( 5.461839458676641001, 117.5340897209903517, -0.6076615112082688341 ) ) ;
#1742=CARTESIAN_POINT ( 'NONE',  ( -2.296080426531199592, 33.88561480753556765, 4.023271960718671991 ) ) ;
#1743=CARTESIAN_POINT ( 'NONE',  ( -0.5727016603203397560, 115.7031860021946557, 1.740666313404392485 ) ) ;
#1744=CARTESIAN_POINT ( 'NONE',  ( -1.932895124392534303, 20.38400505531995321, -4.219463811995566083 ) ) ;
#1745=VERTEX_POINT ( 'NONE', #40754 ) ;
#1746=CARTESIAN_POINT ( 'NONE',  ( -4.843412999271194508, 105.1215046380817029, -2.263786507608671617 ) ) ;
#1747=CARTESIAN_POINT ( 'NONE',  ( 3.827285340041869155, -15.59443631323044421, 3.224486442507772388 ) ) ;
#1748=CARTESIAN_POINT ( 'NONE',  ( -0.4802819474809040812, 118.7114656741295988, 0.5981741851633315399 ) ) ;
#1750=CARTESIAN_POINT ( 'NONE',  ( 0.5005776846888100318, 19.73258526448893591, -0.8400667230076528380 ) ) ;
#1752=ORIENTED_EDGE ( 'NONE', *, *, #36346, .F. ) ;
#1754=CARTESIAN_POINT ( 'NONE',  ( 4.252685754339869284, 122.9893884486272526, 0.2003490066864924701 ) ) ;
#1756=CARTESIAN_POINT ( 'NONE',  ( -8.590326429123278373, 154.7538831414287870, 1.096848044820072143 ) ) ;
#1758=CARTESIAN_POINT ( 'NONE',  ( 4.705771658150993630, 117.9790676909462661, -0.6572654973250883215 ) ) ;
#1759=CARTESIAN_POINT ( 'NONE',  ( 5.624295920984120123, 156.7050554705274408, -1.628980406729419128 ) ) ;
#1760=CARTESIAN_POINT ( 'NONE',  ( -14.15513794057049779, 123.4894365733723447, -1.873888081047781595 ) ) ;
#1763=CARTESIAN_POINT ( 'NONE',  ( 4.171966789054940783, 118.2392508536157862, -0.2176385797143781942 ) ) ;
#1764=CARTESIAN_POINT ( 'NONE',  ( 8.223969002016808361, 122.7966848691156514, -0.2142357769474920459 ) ) ;
#1766=CARTESIAN_POINT ( 'NONE',  ( 3.178324225997528618, -14.33742748831649827, 1.935164598152447679 ) ) ;
#1767=CARTESIAN_POINT ( 'NONE',  ( 4.972946268020358218, 117.3993836135847033, 0.9764272678749694734 ) ) ;
#1770=CARTESIAN_POINT ( 'NONE',  ( 3.951836011467571907, -5.044640503713330837, -2.394960105287299523 ) ) ;
#1771=CARTESIAN_POINT ( 'NONE',  ( 17.23725050067783471, 146.8699245690979751, 2.055247338431126725 ) ) ;
#1772=CARTESIAN_POINT ( 'NONE',  ( -3.055152424816264478, 29.15171311842127011, 2.103066797612082262 ) ) ;
#1773=CARTESIAN_POINT ( 'NONE',  ( -4.073291749555337127, 117.6466181296975151, 0.7504383534773491071 ) ) ;
#1774=CARTESIAN_POINT ( 'NONE',  ( -4.637963820743935983, -6.603494994175692412, 0.1710436084038768345 ) ) ;
#1775=CARTESIAN_POINT ( 'NONE',  ( 4.232597188052644732, 155.8470599587123502, 0.1762653075193724439 ) ) ;
#1776=CARTESIAN_POINT ( 'NONE',  ( 8.344183819546742598, 4.025392264050483782, -1.191670311180863528 ) ) ;
#1778=CARTESIAN_POINT ( 'NONE',  ( -2.140641356428172770, 116.4937786673416866, -0.3810182028649428676 ) ) ;
#1784=CARTESIAN_POINT ( 'NONE',  ( 7.466160517099046601, -1.205741384250370363, -3.973931221679563919 ) ) ;
#1785=CARTESIAN_POINT ( 'NONE',  ( 3.314101028046484210, 118.1588881422629242, 0.7891393284369173644 ) ) ;
#1788=CARTESIAN_POINT ( 'NONE',  ( 0.1041500444719085511, 106.1822392402443143, -5.212094112990285133 ) ) ;
#1789=CARTESIAN_POINT ( 'NONE',  ( -10.70371904046275979, 157.9381250348597234, 0.2505172755855811784 ) ) ;
#1790=VERTEX_POINT ( 'NONE', #28383 ) ;
#1794=CARTESIAN_POINT ( 'NONE',  ( -1.624513285529166184, 120.9965111687125159, 0.001083860100774148216 ) ) ;
#1795=CARTESIAN_POINT ( 'NONE',  ( 5.341109902925343711, -14.98078892696824660, 3.412803344283087181 ) ) ;
#1796=CARTESIAN_POINT ( 'NONE',  ( -0.01081828485867829433, 118.1092738308834669, 0.5413912121690740431 ) ) ;
#1797=CARTESIAN_POINT ( 'NONE',  ( 4.883164212476692967, 117.4312795728108227, -0.5545796311387335420 ) ) ;
#1798=CARTESIAN_POINT ( 'NONE',  ( 4.419457123578296454, 17.78516144714274105, -1.360477052881604143 ) ) ;
#1799=CARTESIAN_POINT ( 'NONE',  ( -16.90643861817993354, 122.6916909566506320, -0.7822879649369940402 ) ) ;
#1802=AXIS2_PLACEMENT_3D ( 'NONE', #31412, #41438, #15845 ) ;
#1803=CARTESIAN_POINT ( 'NONE',  ( -5.563982112966385785, 116.7029361893387431, -0.03558650952807581452 ) ) ;
#1805=CARTESIAN_POINT ( 'NONE',  ( -9.157854976475398701, 121.7740273863187923, 1.020316602444926835 ) ) ;
#1807=CARTESIAN_POINT ( 'NONE',  ( 12.53898343483645483, 122.9501582372872406, -1.331292802868025316 ) ) ;
#1808=CARTESIAN_POINT ( 'NONE',  ( -4.913347341789825684, 118.0342071775839941, -0.9606804153092147747 ) ) ;
#1810=CARTESIAN_POINT ( 'NONE',  ( 0.7306116569919257620, 156.4221767039705071, -0.6844267650493706112 ) ) ;
#1812=CARTESIAN_POINT ( 'NONE',  ( -16.01586142131302637, 150.9843922791743296, -2.313278988710850470 ) ) ;
#1813=CARTESIAN_POINT ( 'NONE',  ( 3.179180861052679052, -15.64967171142420099, 4.365151252316144870 ) ) ;
#1814=CARTESIAN_POINT ( 'NONE',  ( -4.340471936078397874, 118.1815412487432866, -0.6239179087215906971 ) ) ;
#1817=CARTESIAN_POINT ( 'NONE',  ( 11.24613893767475581, 123.2561760277034324, 1.620791190024705175 ) ) ;
#1819=CARTESIAN_POINT ( 'NONE',  ( -5.224212249200172131, -8.128124378088662283, -6.605211778952579493 ) ) ;
#1820=CARTESIAN_POINT ( 'NONE',  ( 15.89661694251502233, 145.9828583539951126, 0.9138632209041560595 ) ) ;
#1825=CARTESIAN_POINT ( 'NONE',  ( -2.017383181376497969, 117.3993839202099849, 1.370540161117654421 ) ) ;
#1829=CARTESIAN_POINT ( 'NONE',  ( -4.745947329130700609, 116.7839080817633430, 0.02307940527355903035 ) ) ;
#1832=CARTESIAN_POINT ( 'NONE',  ( -7.899188505988096409, 121.9926928506463355, -0.9456170989852971109 ) ) ;
#1834=ORIENTED_EDGE ( 'NONE', *, *, #16784, .F. ) ;
#1835=CARTESIAN_POINT ( 'NONE',  ( 4.758501140356155901, 118.7629491485453741, -0.8044719740567526367 ) ) ;
#1836=CARTESIAN_POINT ( 'NONE',  ( -11.87576104716911907, 151.9737369308441544, -0.5463127210923325316 ) ) ;
#1837=CARTESIAN_POINT ( 'NONE',  ( 2.069070256058832324, -15.20480250118845511, 5.930115229603830862 ) ) ;
#1838=CARTESIAN_POINT ( 'NONE',  ( -3.003295232750944344, 159.1263692740743068, 1.093010787580665832 ) ) ;
#1840=DIRECTION ( 'NONE',  ( -0.9998004120163608288, 0.000000000000000000, -0.01997839162482749342 ) ) ;
#1841=CARTESIAN_POINT ( 'NONE',  ( 13.64397932274287584, 119.6379125180634446, 0.3727430486357818928 ) ) ;
#1842=CARTESIAN_POINT ( 'NONE',  ( 8.025551358755512510, 122.8503416937399351, 0.2015751188716342623 ) ) ;
#1843=CARTESIAN_POINT ( 'NONE',  ( -5.005799711115156647, 117.5941877228957537, 0.5449465340951143988 ) ) ;
#1844=CARTESIAN_POINT ( 'NONE',  ( -0.2409191691226134635, 30.52881386638012629, -0.9476172785465332149 ) ) ;
#1845=CARTESIAN_POINT ( 'NONE',  ( -8.213135470206685440, 117.5064756823292385, -0.2531991783344218483 ) ) ;
#1846=DIRECTION ( 'NONE',  ( -4.017660918040594346E-17, 1.000000000000000000, 2.376309959284834438E-19 ) ) ;
#1850=CARTESIAN_POINT ( 'NONE',  ( -5.969389315549677555, 118.6093026330748614, 0.9569931481840777687 ) ) ;
#1852=CARTESIAN_POINT ( 'NONE',  ( 3.006067730437935293, 117.5448765310053005, 0.7098943453401750370 ) ) ;
#1855=CARTESIAN_POINT ( 'NONE',  ( 18.89434961005710534, 135.8679125664981484, -1.636908753694952257 ) ) ;
#1856=CARTESIAN_POINT ( 'NONE',  ( -8.392384909494198908, 27.87760190725155951, 0.4359655409547527616 ) ) ;
#1857=CARTESIAN_POINT ( 'NONE',  ( -1.008854969157164216, 117.0751458430253393, -0.4193480094219990129 ) ) ;
#1858=CARTESIAN_POINT ( 'NONE',  ( 4.919889287388610200, 117.6395836675350353, -0.8280294640748854240 ) ) ;
#1861=CARTESIAN_POINT ( 'NONE',  ( -9.105893302116724541, 123.9936668703698075, -0.02250835519154683814 ) ) ;
#1862=CARTESIAN_POINT ( 'NONE',  ( -12.39214084994788756, 122.8403290575659526, -1.822206477283890624 ) ) ;
#1863=CARTESIAN_POINT ( 'NONE',  ( 6.169188725349925129, -14.24425063093240418, 1.535968726618487379 ) ) ;
#1864=DIRECTION ( 'NONE',  ( 0.9998004120163608288, 0.000000000000000000, 0.01997839162482749342 ) ) ;
#1865=CARTESIAN_POINT ( 'NONE',  ( -1.567216851204632500, 117.9496054947997692, -1.374611063050779514 ) ) ;
#1866=EDGE_LOOP ( 'NONE', ( #30676, #16869 ) ) ;
#1867=CARTESIAN_POINT ( 'NONE',  ( 19.09005709338556400, 148.2829752965438956, 2.500029303593213736 ) ) ;
#1871=CARTESIAN_POINT ( 'NONE',  ( -2.328636301501583628, 124.8000875644994068, -0.03907356579384855394 ) ) ;
#1872=CARTESIAN_POINT ( 'NONE',  ( -6.911983299595774177, -11.51556667111630894, -4.837919318831837678 ) ) ;
#1873=CARTESIAN_POINT ( 'NONE',  ( 11.86571527151339822, 128.3619849303985632, 1.073981288313974991 ) ) ;
#1875=CARTESIAN_POINT ( 'NONE',  ( 20.43054131464308298, 152.5480347002736607, -0.4178791510274245113 ) ) ;
#1878=PRESENTATION_STYLE_ASSIGNMENT (( #30622 ) ) ;
#1879=CARTESIAN_POINT ( 'NONE',  ( 1.824656174747253168, -15.25388738520313225, 5.420764384989097628 ) ) ;
#1880=CARTESIAN_POINT ( 'NONE',  ( -4.117142285576561811, 118.2429491485453354, 0.1876306250578462509 ) ) ;
#1881=CARTESIAN_POINT ( 'NONE',  ( -11.74288454345109756, 118.7273140689154616, -0.2346507796901759202 ) ) ;
#1885=CARTESIAN_POINT ( 'NONE',  ( -6.174373104427945513, 119.6968065231476857, -1.242162679386602520 ) ) ;
#1886=FACE_OUTER_BOUND ( 'NONE', #34234, .T. ) ;
#1887=CARTESIAN_POINT ( 'NONE',  ( 4.224925902082478757, 118.2240476267590736, 0.4891913066779954300 ) ) ;
#1888=CARTESIAN_POINT ( 'NONE',  ( -12.10601879509736634, 151.9817061558079274, -1.041216838735509187 ) ) ;
#1890=CARTESIAN_POINT ( 'NONE',  ( 18.86374853661768825, 125.3403196291361610, 0.3769425889880999581 ) ) ;
#1891=EDGE_CURVE ( 'NONE', #17493, #17052, #5614, .T. ) ;
#1893=CARTESIAN_POINT ( 'NONE',  ( -4.247245584637960647, 22.75789413176893206, 1.861891798430825862 ) ) ;
#1894=CARTESIAN_POINT ( 'NONE',  ( -3.522522545432727359, 120.3814187630814132, -0.6186928868410387361 ) ) ;
#1895=CARTESIAN_POINT ( 'NONE',  ( 3.174366308151882254, 69.94346620154573202, 0.06343139340882769650 ) ) ;
#1898=CARTESIAN_POINT ( 'NONE',  ( -6.991872955157565350, 121.9342904866002186, -0.005970709178320789817 ) ) ;
#1900=CARTESIAN_POINT ( 'NONE',  ( 22.03992273305654237, 150.6352520364973486, 1.509874617927603024 ) ) ;
#1901=CARTESIAN_POINT ( 'NONE',  ( 4.130807148828959718, 104.6144662015457385, -2.502011538036419402 ) ) ;
#1902=CARTESIAN_POINT ( 'NONE',  ( 3.028202472743143581, -14.11696900735987015, 1.123381337427139526 ) ) ;
#1903=CARTESIAN_POINT ( 'NONE',  ( 21.42146139051182985, 149.1985357531029308, -1.383244442692061149 ) ) ;
#1904=CARTESIAN_POINT ( 'NONE',  ( -0.01081828683970047049, 119.3136608367422866, 0.5413913113077200023 ) ) ;
#1905=CARTESIAN_POINT ( 'NONE',  ( 1.653223041919489544, 21.06826514481450729, 4.324967054831568625 ) ) ;
#1906=CARTESIAN_POINT ( 'NONE',  ( -14.40286820143220936, 120.3907653763288579, -0.8772178161575924227 ) ) ;
#1908=CARTESIAN_POINT ( 'NONE',  ( -0.1559983344249278314, 9.848737885527594216, 0.9609112391775298523 ) ) ;
#1909=EDGE_LOOP ( 'NONE', ( #42053, #40651, #8623, #21459 ) ) ;
#1912=CARTESIAN_POINT ( 'NONE',  ( -9.756861847786568731, 124.2227999206177032, 0.4199055954619892450 ) ) ;
#1913=CARTESIAN_POINT ( 'NONE',  ( 5.228661469329079381, -12.87456325985388084, 2.426867231591100182 ) ) ;
#1914=CARTESIAN_POINT ( 'NONE',  ( 2.563812760316453332, 119.9929590031203901, -0.5332384965226230067 ) ) ;
#1915=ORIENTED_EDGE ( 'NONE', *, *, #26964, .T. ) ;
#1916=CARTESIAN_POINT ( 'NONE',  ( 1.123125151977883318, 115.7029491485453718, 1.744272880635622247 ) ) ;
#1917=ORIENTED_EDGE ( 'NONE', *, *, #29167, .T. ) ;
#1918=CARTESIAN_POINT ( 'NONE',  ( 3.334874478900925254, -13.11215654211414439, 1.739483084651320066 ) ) ;
#1919=CARTESIAN_POINT ( 'NONE',  ( -4.780916927273618278, 117.8747006157190214, -0.8582680989615314449 ) ) ;
#1920=CARTESIAN_POINT ( 'NONE',  ( 9.145901261935787119, 124.1724329610943300, 0.1484858654357239516 ) ) ;
#1921=ORIENTED_EDGE ( 'NONE', *, *, #7173, .T. ) ;
#1922=CARTESIAN_POINT ( 'NONE',  ( 10.11172965818656166, 120.4647147465577461, 1.576227610178518201 ) ) ;
#1924=DIRECTION ( 'NONE',  ( 4.017660918040594346E-17, -1.000000000000000000, -2.376309959284834438E-19 ) ) ;
#1926=CARTESIAN_POINT ( 'NONE',  ( -4.800085724567965784, 115.7029491485459545, -1.472342921364490298 ) ) ;
#1927=CARTESIAN_POINT ( 'NONE',  ( 23.32536756748174867, 149.0517038676186417, 0.2354165988066211079 ) ) ;
#1929=( BOUNDED_SURFACE ( )  B_SPLINE_SURFACE ( 3, 2, ( 
 ( #33401, #8037, #14410 ),
 ( #17193, #40014, #10806 ),
 ( #34033, #1662, #11018 ),
 ( #23788, #23998, #17402 ),
 ( #36809, #4445, #14616 ),
 ( #37019, #1247, #17608 ),
 ( #27417, #27620, #21418 ),
 ( #8666, #2290, #25054 ),
 ( #37636, #12281, #25487 ),
 ( #9092, #18441, #41475 ),
 ( #34444, #14827, #24845 ),
 ( #41685, #1865, #31447 ),
 ( #5907, #31874, #18868 ),
 ( #27832, #31023, #12067 ),
 ( #25270, #40838, #18658 ),
 ( #21839, #31231, #2715 ),
 ( #5277, #11641, #28675 ),
 ( #35085, #24626, #8460 ),
 ( #31663, #18229, #11858 ),
 ( #8241, #38274, #12492 ) ),
 .UNSPECIFIED., .F., .F., .T. ) 
 B_SPLINE_SURFACE_WITH_KNOTS ( ( 4, 2, 2, 2, 2, 2, 2, 2, 2, 4 ),
 ( 3, 3 ),
 ( -1.951563910473907981E-17, 0.0002906966660415815436, 0.0004360449990623821003, 0.0005813933320831826028, 0.0008720899981247837163, 0.001162786664166384721, 0.002325573328332788958, 0.002906966660415991402, 0.003488359992499193412, 0.004651146656665597866 ),
 ( 0.000000000000000000, 0.7115408901999051849 ),
 .UNSPECIFIED. ) 
 GEOMETRIC_REPRESENTATION_ITEM ( )  RATIONAL_B_SPLINE_SURFACE ( (
 ( 1.000000000000000000, 0.8295190474764645439, 0.9016464323943773618),
 ( 1.000000000000000000, 0.8295190474764645439, 0.9016464323943773618),
 ( 1.000000000000000000, 0.8295191844949277860, 0.9016465114428253713),
 ( 1.000000000000000000, 0.8295189621554358572, 0.9016463831711215571),
 ( 1.000000000000000000, 0.8295186834253872599, 0.9016462223666781295),
 ( 1.000000000000000000, 0.8295188167253252365, 0.9016462992698410783),
 ( 1.000000000000000000, 0.8295190048409176731, 0.9016464077971535485),
 ( 1.000000000000000000, 0.8295192071976853487, 0.9016465245404596818),
 ( 1.000000000000000000, 0.8295190396943252775, 0.9016464279047196051),
 ( 1.000000000000000000, 0.8295190584192864147, 0.9016464387074907272),
 ( 1.000000000000000000, 0.8295190452658104396, 0.9016464311190108827),
 ( 1.000000000000000000, 0.8295190572912768401, 0.9016464380567215109),
 ( 1.000000000000000000, 0.8295191187437633840, 0.9016464735097805550),
 ( 1.000000000000000000, 0.8295190147136782821, 0.9016464134929291774),
 ( 1.000000000000000000, 0.8295185759670760106, 0.9016461603720204998),
 ( 1.000000000000000000, 0.8295184858515097792, 0.9016461083827084222),
 ( 1.000000000000000000, 0.8295190237822920309, 0.9016464187247776874),
 ( 1.000000000000000000, 0.8295190933398598476, 0.9016464588538057878),
 ( 1.000000000000000000, 0.8295190474770748335, 0.9016464323947295245),
 ( 1.000000000000000000, 0.8295190474770748335, 0.9016464323947295245) ) ) 
 REPRESENTATION_ITEM ( '' )  SURFACE ( )  );
#1932=EDGE_CURVE ( 'NONE', #25709, #5098, #38932, .T. ) ;
#1933=CARTESIAN_POINT ( 'NONE',  ( 1.986764264153795478, -15.15368377650233533, 5.911265622359163530 ) ) ;
#1936=CARTESIAN_POINT ( 'NONE',  ( -4.735645682745369456, 117.8440288062297441, 0.8352900991755182192 ) ) ;
#1939=CARTESIAN_POINT ( 'NONE',  ( 8.527773727094952960, 119.1143268667826476, -0.9731819787258109145 ) ) ;
#1940=CARTESIAN_POINT ( 'NONE',  ( -3.998531074477553293, 117.0582680968029905, -1.101271957883942942 ) ) ;
#1941=CARTESIAN_POINT ( 'NONE',  ( 4.962772945303370875, 117.4661736183843317, 0.9732638675253090232 ) ) ;
#1943=CARTESIAN_POINT ( 'NONE',  ( -0.07831152689304127223, 109.4728569552520838, 3.919029035233798641 ) ) ;
#1947=CARTESIAN_POINT ( 'NONE',  ( 1.990724735134854262, -15.09768785095407040, 5.370787383207776600 ) ) ;
#1948=CARTESIAN_POINT ( 'NONE',  ( 5.187812668267121730, 115.4810986995850755, -1.301936727496811441 ) ) ;
#1949=CARTESIAN_POINT ( 'NONE',  ( 0.9515549220119206009, 38.57169665032974848, 1.406172627325484203 ) ) ;
#1950=CARTESIAN_POINT ( 'NONE',  ( -0.4316363188167808840, 115.7034387397185213, 1.748257578123638245 ) ) ;
#1951=CARTESIAN_POINT ( 'NONE',  ( 4.326043401919948295, 8.289558097378858292, -1.648119079657388353 ) ) ;
#1953=CARTESIAN_POINT ( 'NONE',  ( -2.761919320456341698, 105.1243152825708620, -4.564426355482043896 ) ) ;
#1954=CARTESIAN_POINT ( 'NONE',  ( 4.220783105811589664, -15.35787857112312693, 0.3368293509108917783 ) ) ;
#1955=CARTESIAN_POINT ( 'NONE',  ( -15.53591925045088651, 153.1703808545849483, 1.736877461573578030 ) ) ;
#1956=CARTESIAN_POINT ( 'NONE',  ( 0.9071407760921452734, 21.51634675185595924, 0.3571511405359465430 ) ) ;
#1957=CARTESIAN_POINT ( 'NONE',  ( -0.9163883642843115851, 13.89126970375589032, 0.3362141533434955809 ) ) ;
#1961=CARTESIAN_POINT ( 'NONE',  ( 2.642867612521250908, 121.0686911241271702, 0.3905210903889254070 ) ) ;
#1963=CARTESIAN_POINT ( 'NONE',  ( -9.666892607209499388, 123.4354624054469980, 0.6853163995640745298 ) ) ;
#1965=CARTESIAN_POINT ( 'NONE',  ( 3.325379330704291814, -12.45968715000887705, 0.9553361148970926919 ) ) ;
#1966=CARTESIAN_POINT ( 'NONE',  ( 2.217461812776179819, 157.2504501563031738, -1.545323669738358552 ) ) ;
#1967=CARTESIAN_POINT ( 'NONE',  ( -19.82367009662587520, 149.5711785761137662, -2.459487706365388604 ) ) ;
#1969=CARTESIAN_POINT ( 'NONE',  ( 4.074910602682932925, 118.2429491485453497, -0.1454311599470141936 ) ) ;
#1970=CARTESIAN_POINT ( 'NONE',  ( 6.492529462933093853, 121.6679077367135591, -0.1901135952749836711 ) ) ;
#1972=ORIENTED_EDGE ( 'NONE', *, *, #22219, .T. ) ;
#1973=CARTESIAN_POINT ( 'NONE',  ( 3.046489168745748266, -14.83993489217504091, 3.784491786591300588 ) ) ;
#1978=CARTESIAN_POINT ( 'NONE',  ( 2.099109474952898236, -4.195072059908932616, -4.137704358558784712 ) ) ;
#1979=CARTESIAN_POINT ( 'NONE',  ( 1.456364663599907905, 120.2326517397585377, 0.4672470943647334396 ) ) ;
#1980=CARTESIAN_POINT ( 'NONE',  ( -3.216045294022573664, 29.79186273158684983, 3.430717191674401700 ) ) ;
#1981=CARTESIAN_POINT ( 'NONE',  ( -2.055333930833691092, 107.8038693663528278, 4.443139710053165103 ) ) ;
#1982=EDGE_CURVE ( 'NONE', #17903, #12743, #14742, .T. ) ;
#1983=CARTESIAN_POINT ( 'NONE',  ( 3.501419995798253915, -2.955197114699519734, 3.043391175950921568 ) ) ;
#1984=CARTESIAN_POINT ( 'NONE',  ( -0.5321123018419734452, 37.22158963861809156, -0.7300149017649124605 ) ) ;
#1986=CARTESIAN_POINT ( 'NONE',  ( -4.386519595447357922, 0.5779702600499575516, 7.231359419481246498 ) ) ;
#1988=CARTESIAN_POINT ( 'NONE',  ( 2.158285020023808176, 116.4043711044980540, -0.2448377587554940171 ) ) ;
#1991=CARTESIAN_POINT ( 'NONE',  ( -6.442297258278467886, 29.65178619621697464, 0.8020365093557799696 ) ) ;
#1992=CARTESIAN_POINT ( 'NONE',  ( 0.6763034141103227981, -4.228338640871131204, 8.424193199533098309 ) ) ;
#1993=CARTESIAN_POINT ( 'NONE',  ( 0.3349063509247137138, 117.3993832491035363, 1.495621030033295940 ) ) ;
#1994=DIRECTION ( 'NONE',  ( -0.9998004120163608288, 1.039227405372657318E-20, -0.01997839162482760098 ) ) ;
#1995=CARTESIAN_POINT ( 'NONE',  ( 0.3785707606481875653, 120.7331730230137623, -0.5164240810526171677 ) ) ;
#1996=CARTESIAN_POINT ( 'NONE',  ( -21.78567168733534842, 151.4242408681541008, 0.1492089687398850950 ) ) ;
#1999=AXIS2_PLACEMENT_3D ( 'NONE', #32311, #42126, #2936 ) ;
#2003=CARTESIAN_POINT ( 'NONE',  ( -15.72550100231863368, 145.6881679641610674, -0.3142329346387550681 ) ) ;
#2004=CARTESIAN_POINT ( 'NONE',  ( 2.285161673027230389, -15.58026522864758334, 5.856586201423784388 ) ) ;
#2005=CARTESIAN_POINT ( 'NONE',  ( -7.864631202759968964, 118.9574329095587757, 0.9664042006415775043 ) ) ;
#2006=CARTESIAN_POINT ( 'NONE',  ( 19.81309253913735802, 152.3633698111425758, -1.013446639353942968 ) ) ;
#2007=CARTESIAN_POINT ( 'NONE',  ( -1.287880193524239658, 20.15907059199006923, -4.440276399826991849 ) ) ;
#2008=CARTESIAN_POINT ( 'NONE',  ( -18.54376275836462185, 154.1690995007799927, -0.7937872377295739357 ) ) ;
#2011=CARTESIAN_POINT ( 'NONE',  ( 2.182859927827073498, 116.1873359508715566, 0.04703207412767947126 ) ) ;
#2013=CARTESIAN_POINT ( 'NONE',  ( -6.588241325444357699, 120.6599796251122427, 0.8186057014055782011 ) ) ;
#2015=CARTESIAN_POINT ( 'NONE',  ( 18.49981012119508605, 140.7300538122508726, -1.765484999878022654 ) ) ;
#2016=CARTESIAN_POINT ( 'NONE',  ( -16.06052414861355970, 125.3625853296581312, -1.884096674228965540 ) ) ;
#2018=CARTESIAN_POINT ( 'NONE',  ( 0.01596947694123658501, 156.4635559983122448, -0.7991779281049287142 ) ) ;
#2020=CARTESIAN_POINT ( 'NONE',  ( -4.261081698622679603, 119.8084884740358547, -0.9035344350157260562 ) ) ;
#2021=CARTESIAN_POINT ( 'NONE',  ( 4.136722333222721204, -15.50381924862055705, 2.038268645697551396 ) ) ;
#2022=CARTESIAN_POINT ( 'NONE',  ( -4.441848593430714587, 118.1590354598291270, -0.6062622877682531941 ) ) ;
#2025=CARTESIAN_POINT ( 'NONE',  ( -5.007446857918051109, 117.4001727933947450, 0.7824604973016788811 ) ) ;
#2026=CARTESIAN_POINT ( 'NONE',  ( 17.73735868213781330, 147.0764175921665640, 2.241444305069557164 ) ) ;
#2027=DIRECTION ( 'NONE',  ( -5.206863593109713661E-17, 1.000000000000000000, -1.077750396879097183E-30 ) ) ;
#2031=CARTESIAN_POINT ( 'NONE',  ( -4.212901951478492890, -8.356617434558033963, -7.328762184035659821 ) ) ;
#2032=CARTESIAN_POINT ( 'NONE',  ( 15.49830880841120795, 147.8629129908177049, 0.8994996151558262154 ) ) ;
#2039=CARTESIAN_POINT ( 'NONE',  ( -15.61624682818917265, 120.8175431576145940, -0.1535658744814573373 ) ) ;
#2042=CARTESIAN_POINT ( 'NONE',  ( 7.903461424171575267, 122.1176562113792983, -0.5506078847746120886 ) ) ;
#2043=CARTESIAN_POINT ( 'NONE',  ( -8.019189887688819240, 121.5801876769127432, 0.8265596201061200521 ) ) ;
#2045=CARTESIAN_POINT ( 'NONE',  ( -5.078986093043185157, 72.48346620154573827, -0.1014902294541238092 ) ) ;
#2046=CARTESIAN_POINT ( 'NONE',  ( 0.001786757842161811136, 120.9379535345006076, -0.08941666878750617609 ) ) ;
#2047=CARTESIAN_POINT ( 'NONE',  ( 3.754230566796173285, -14.80532124960526374, 5.272564796848507207 ) ) ;
#2048=CARTESIAN_POINT ( 'NONE',  ( -17.30645727728363426, 153.8449085212272678, 1.293747054194649637 ) ) ;
#2050=CARTESIAN_POINT ( 'NONE',  ( 23.37772998923890100, 142.7868430859564626, 0.6200176421473860833 ) ) ;
#2051=CARTESIAN_POINT ( 'NONE',  ( 9.014329603292043913, 124.0612904411588318, 0.2246157754502237647 ) ) ;
#2053=CARTESIAN_POINT ( 'NONE',  ( -0.9703616065139187841, 22.75662690174698355, -0.1248384507273650884 ) ) ;
#2054=CARTESIAN_POINT ( 'NONE',  ( -18.81533481972616428, 125.3161215262879580, -0.4318114027375014041 ) ) ;
#2055=DIRECTION ( 'NONE',  ( -0.9998004120163608288, 0.000000000000000000, -0.01997839162482749342 ) ) ;
#2056=CIRCLE ( 'NONE', #1394, 5.334000000000001407 ) ;
#2058=ORIENTED_EDGE ( 'NONE', *, *, #8373, .F. ) ;
#2059=CARTESIAN_POINT ( 'NONE',  ( -5.866213452989303079, 118.3783053522630979, 0.9224362309636404689 ) ) ;
#2060=CARTESIAN_POINT ( 'NONE',  ( 2.913282581332740762, -14.11548038430587937, -3.586046950971230274 ) ) ;
#2061=CARTESIAN_POINT ( 'NONE',  ( 14.13476661394972211, 155.9232964860746620, 1.730687652093988671 ) ) ;
#2063=CARTESIAN_POINT ( 'NONE',  ( 20.34707623724158054, 149.4216517587604756, -1.615871423115795125 ) ) ;
#2064=CARTESIAN_POINT ( 'NONE',  ( -3.436282163690115077, 26.04026231355703658, -7.687665148811276161 ) ) ;
#2065=CARTESIAN_POINT ( 'NONE',  ( -22.07432572979854157, 148.5290936231802448, -2.031061984987305280 ) ) ;
#2066=CARTESIAN_POINT ( 'NONE',  ( 4.869185350499654952, 117.6445503307796798, -0.8938492170851732865 ) ) ;
#2067=CARTESIAN_POINT ( 'NONE',  ( 1.973215784349658497, 106.6933082031156772, 4.964841027628618342 ) ) ;
#2069=CARTESIAN_POINT ( 'NONE',  ( -15.40211203110487759, 147.8297367799732456, -0.07919316026241125794 ) ) ;
#2070=CARTESIAN_POINT ( 'NONE',  ( -19.51070465195341797, 147.4874203640471535, -2.520207112597399934 ) ) ;
#2071=CARTESIAN_POINT ( 'NONE',  ( 2.090134903116885656, -15.63197564439436427, 5.828951795168951122 ) ) ;
#2075=CARTESIAN_POINT ( 'NONE',  ( 9.618126185770233150, 121.1143850344477215, 1.566364589618396419 ) ) ;
#2079=CARTESIAN_POINT ( 'NONE',  ( -0.4023205627561269870, 108.3383513567250986, 4.340400160729728896 ) ) ;
#2080=CARTESIAN_POINT ( 'NONE',  ( 2.927854471352651533, -7.645316342317141967, 7.903470162911977681 ) ) ;
#2081=CARTESIAN_POINT ( 'NONE',  ( 12.31319552751066659, 152.0262389575480881, 1.296791798139147023 ) ) ;
#2082=CARTESIAN_POINT ( 'NONE',  ( -4.787717183442803837, 118.5930653697794384, -0.9403843580293530513 ) ) ;
#2084=CARTESIAN_POINT ( 'NONE',  ( 18.36446446646845487, 154.1536317137893661, -0.4323159980074336994 ) ) ;
#2090=CARTESIAN_POINT ( 'NONE',  ( -4.287468807849243113, 118.2136502785617154, 0.3571622525904151746 ) ) ;
#2091=CARTESIAN_POINT ( 'NONE',  ( -21.68875320759065062, 132.7412702629105468, -0.4333929054516005852 ) ) ;
#2092=EDGE_LOOP ( 'NONE', ( #21526, #19689, #30798, #12030 ) ) ;
#2094=CARTESIAN_POINT ( 'NONE',  ( -4.013207239964067696, 119.1603065593399720, -0.9237844164917737855 ) ) ;
#2095=CARTESIAN_POINT ( 'NONE',  ( -1.381059818124894312, 106.2379067940291293, -5.172899357470507553 ) ) ;
#2096=CARTESIAN_POINT ( 'NONE',  ( 4.350168497188355410, 118.1836287563303358, 0.6150604927752495454 ) ) ;
#2097=CARTESIAN_POINT ( 'NONE',  ( -14.64564643111563846, 139.2174805014774392, -1.155614491733865989 ) ) ;
#2101=ORIENTED_EDGE ( 'NONE', *, *, #26310, .T. ) ;
#2102=CARTESIAN_POINT ( 'NONE',  ( 3.400481176189167343, 25.78150505744974552, 3.158589348000393482 ) ) ;
#2106=CARTESIAN_POINT ( 'NONE',  ( -3.682264917456324227, 94.83546620154572793, -0.07358041635423923088 ) ) ;
#2107=CARTESIAN_POINT ( 'NONE',  ( -7.810501765866526114, 122.5295832722994191, 0.1257769165047209758 ) ) ;
#2109=CARTESIAN_POINT ( 'NONE',  ( 5.495761340641351467, 159.0395019988757781, 0.8742782617121154232 ) ) ;
#2111=CARTESIAN_POINT ( 'NONE',  ( 1.852819980464847305, -15.24972552306870455, 5.408883774200016425 ) ) ;
#2112=CARTESIAN_POINT ( 'NONE',  ( 16.31190729917912563, 125.3309463260932830, -1.192360770973151851 ) ) ;
#2113=AXIS2_PLACEMENT_3D ( 'NONE', #41531, #15095, #8516 ) ;
#2114=CARTESIAN_POINT ( 'NONE',  ( -11.41525058642626256, 122.8492764348241337, 1.228842657910306002 ) ) ;
#2115=CARTESIAN_POINT ( 'NONE',  ( 0.7725963012898818816, -15.30024676335969325, -0.5870848125168374176 ) ) ;
#2116=CARTESIAN_POINT ( 'NONE',  ( -4.821777392514813521, 117.1414559920645644, -0.5894805283384125794 ) ) ;
#2117=CARTESIAN_POINT ( 'NONE',  ( 0.8451309169872193161, 21.29487494764119759, 0.4837088869917456346 ) ) ;
#2120=CARTESIAN_POINT ( 'NONE',  ( -0.6220149250935740337, 120.7813932625355307, 0.1825499261673581841 ) ) ;
#2122=CARTESIAN_POINT ( 'NONE',  ( 2.821817058828279823, -15.16010343277639194, 5.768636546787819341 ) ) ;
#2123=CARTESIAN_POINT ( 'NONE',  ( 17.27955699683393576, 146.3482411845097886, -1.367784599882192254 ) ) ;
#2125=CARTESIAN_POINT ( 'NONE',  ( 1.943291158100776572, 115.7022449525728263, 1.718216098553282833 ) ) ;
#2126=CARTESIAN_POINT ( 'NONE',  ( -4.724190901440335821, 117.9428858324453984, -0.8166581812100317528 ) ) ;
#2128=CARTESIAN_POINT ( 'NONE',  ( 6.497458072406196550, 121.7745328324513139, 0.05723077286956951282 ) ) ;
#2130=CARTESIAN_POINT ( 'NONE',  ( 11.20355582914602266, 156.1341193432522800, 2.130866455309296192 ) ) ;
#2135=CARTESIAN_POINT ( 'NONE',  ( -3.174366308152011928, 65.62546620154573418, -0.06343139340882732180 ) ) ;
#2136=CARTESIAN_POINT ( 'NONE',  ( 18.59469708476128602, 154.1615476314759974, 0.06268175667117116545 ) ) ;
#2137=CARTESIAN_POINT ( 'NONE',  ( 0.07831152689291247249, 109.4728569552520838, -3.919029035233798641 ) ) ;
#2139=CARTESIAN_POINT ( 'NONE',  ( 1.887010163324958523, -15.42916175108831389, 5.374230824943217577 ) ) ;
#2140=DIRECTION ( 'NONE',  ( -0.01997839162482749342, -1.040247600000944484E-18, 0.9998004120163608288 ) ) ;
#2143=CARTESIAN_POINT ( 'NONE',  ( -4.846938226398710192, 117.8246799134837914, 0.6898159354236798047 ) ) ;
#2147=CARTESIAN_POINT ( 'NONE',  ( 8.513471249619389170, 119.1860349514362838, -0.9933054490459751751 ) ) ;
#2148=CARTESIAN_POINT ( 'NONE',  ( -6.475519728870542835, 122.5560431351108974, -0.2403424393823894445 ) ) ;
#2149=CARTESIAN_POINT ( 'NONE',  ( 4.716832267211478857, 117.7257293850826585, 1.100839505850291999 ) ) ;
#2151=CARTESIAN_POINT ( 'NONE',  ( -0.3351388899281586009, 111.5577547982948801, 3.138814863473581962 ) ) ;
#2152=CARTESIAN_POINT ( 'NONE',  ( 3.895047602890354010, -2.730319773039217690, 2.488009491782988469 ) ) ;
#2154=LINE ( 'NONE', #41343, #29394 ) ;
#2155=CARTESIAN_POINT ( 'NONE',  ( 3.383663933261424006, -14.10150345098371005, 4.318103191797684204 ) ) ;
#2156=CARTESIAN_POINT ( 'NONE',  ( 5.259129974998846713, 118.7524313932052991, -0.4270625282899581099 ) ) ;
#2157=CARTESIAN_POINT ( 'NONE',  ( -14.38208595515612664, 131.1674235819977241, -1.945708262771122854 ) ) ;
#2158=CARTESIAN_POINT ( 'NONE',  ( -6.997652642833405601, 121.9526520506185676, -0.1398297539000763479 ) ) ;
#2159=CARTESIAN_POINT ( 'NONE',  ( -4.945311175443938723, 30.81497459379012227, 3.823255950980341655 ) ) ;
#2161=CARTESIAN_POINT ( 'NONE',  ( -1.039409186399214535, 115.7029401452854671, 1.708810721072470784 ) ) ;
#2162=CARTESIAN_POINT ( 'NONE',  ( -0.5093740622119584671, 14.76157059199007016, 4.595130897425484306 ) ) ;
#2163=CARTESIAN_POINT ( 'NONE',  ( 13.28278499026787784, 156.9705208988102640, 0.7618315876160811628 ) ) ;
#2165=CARTESIAN_POINT ( 'NONE',  ( 0.2403197276938094373, 104.6144662015456674, -5.339994071284486665 ) ) ;
#2166=CARTESIAN_POINT ( 'NONE',  ( 4.466571682983457414, -15.50692525667736454, 1.643437993322231838 ) ) ;
#2167=CARTESIAN_POINT ( 'NONE',  ( -8.634969826329047748, 120.3810071108087243, 1.137220218559220841 ) ) ;
#2168=CARTESIAN_POINT ( 'NONE',  ( -0.6564745402265276253, 25.61689014148909393, -0.7196881648562951650 ) ) ;
#2170=CARTESIAN_POINT ( 'NONE',  ( -0.8868740923517060004, 23.60745955286466824, 0.4068859645678858938 ) ) ;
#2172=VERTEX_POINT ( 'NONE', #22589 ) ;
#2174=DIRECTION ( 'NONE',  ( -0.9998004120163609398, -4.016384292689130894E-17, -0.01997839162482749689 ) ) ;
#2175=CARTESIAN_POINT ( 'NONE',  ( 1.232226514448922616, 109.2701902778323557, 3.967559291276892885 ) ) ;
#2176=CARTESIAN_POINT ( 'NONE',  ( -10.18692116311738438, 123.6566696788710686, 0.8138387218406053503 ) ) ;
#2178=CARTESIAN_POINT ( 'NONE',  ( 2.022490532284443088, -15.01207906941262671, 5.472131392975311925 ) ) ;
#2179=CARTESIAN_POINT ( 'NONE',  ( 12.49185498700837016, 153.6617311634574037, -1.629683330142263076 ) ) ;
#2181=CARTESIAN_POINT ( 'NONE',  ( -12.79701950029137691, 155.3440856034525837, -2.194532851538729012 ) ) ;
#2184=CARTESIAN_POINT ( 'NONE',  ( -8.935197197525255319, 123.9063447689825779, -0.1785465045940570206 ) ) ;
#2185=CARTESIAN_POINT ( 'NONE',  ( -0.7326219338007132764, 37.28220708697721619, 2.048504824603448959 ) ) ;
#2186=CARTESIAN_POINT ( 'NONE',  ( 15.92039698932583569, 146.6311637152522565, -0.2762755564230129912 ) ) ;
#2188=CARTESIAN_POINT ( 'NONE',  ( 3.186936940905604754, -14.67134942876716153, 3.163583609075255598 ) ) ;
#2190=( BOUNDED_CURVE ( )  B_SPLINE_CURVE ( 3, ( #1660, #40630, #31021, #41257 ),
 .UNSPECIFIED., .F., .T. ) 
 B_SPLINE_CURVE_WITH_KNOTS ( ( 4, 4 ),
 ( 0.6881516260757224446, 0.7252176650374851929 ),
 .UNSPECIFIED. ) 
 CURVE ( )  GEOMETRIC_REPRESENTATION_ITEM ( )  RATIONAL_B_SPLINE_CURVE ( ( 0.5306017708566714841, 0.5183752415894662402, 0.5098124223071008876, 0.5049133130095754263 ) ) 
 REPRESENTATION_ITEM ( '' )  );
#2191=CARTESIAN_POINT ( 'NONE',  ( 2.383981540283352629, 36.81846344528510429, 1.803752045214196853 ) ) ;
#2193=CARTESIAN_POINT ( 'NONE',  ( -1.997604609866625580, -12.39122764300357105, -4.168859717980781809 ) ) ;
#2194=CARTESIAN_POINT ( 'NONE',  ( 4.379744549753488592, 120.5100497556178567, 0.6885478749808132681 ) ) ;
#2195=CARTESIAN_POINT ( 'NONE',  ( -3.110005066758847025, 28.42684073856939619, 0.3580217987620312736 ) ) ;
#2196=CARTESIAN_POINT ( 'NONE',  ( -5.907561988889506566, 118.9932487913337411, 0.3492918592308485448 ) ) ;
#2198=CARTESIAN_POINT ( 'NONE',  ( 2.522041008973656240, -3.380034811851383214, 3.874746376371965617 ) ) ;
#2199=CARTESIAN_POINT ( 'NONE',  ( 2.836071964827284297, 121.0300505300837415, 0.05667146733340969189 ) ) ;
#2200=CARTESIAN_POINT ( 'NONE',  ( 8.265420891810833837, -5.467761657695628053, -1.740095136296691214 ) ) ;
#2202=CARTESIAN_POINT ( 'NONE',  ( 5.525492539046071627, 117.0090066130893547, -0.4571800171334148843 ) ) ;
#2203=CARTESIAN_POINT ( 'NONE',  ( -0.9036232957556743495, 122.5862318000603182, -0.2430700419085213837 ) ) ;
#2205=CARTESIAN_POINT ( 'NONE',  ( -3.456281358658260583, 50.63946620154572997, -1.847419665314800508 ) ) ;
#2206=CARTESIAN_POINT ( 'NONE',  ( -2.033853377119958061, -8.777475726645231902, -8.175041553700232555 ) ) ;
#2207=CARTESIAN_POINT ( 'NONE',  ( 0.7927169096838266871, 117.9394488418538174, 1.400391285740484104 ) ) ;
#2210=CARTESIAN_POINT ( 'NONE',  ( 0.4698238578430272705, 109.1907409294041429, -4.006476130220050891 ) ) ;
#2211=CARTESIAN_POINT ( 'NONE',  ( -23.15061725546907212, 148.7607265879045144, 0.2678260907677696978 ) ) ;
#2212=EDGE_CURVE ( 'NONE', #18094, #36577, #5178, .T. ) ;
#2213=ORIENTED_EDGE ( 'NONE', *, *, #18348, .T. ) ;
#2217=DIRECTION ( 'NONE',  ( 4.017660918040594346E-17, -1.000000000000000000, -2.376309959284832031E-19 ) ) ;
#2218=CARTESIAN_POINT ( 'NONE',  ( -11.82813386268903955, 130.3161362890850512, -0.2363542639706542603 ) ) ;
#2219=CARTESIAN_POINT ( 'NONE',  ( 5.861737433447875567, -14.68024823731529871, 2.247769314782747774 ) ) ;
#2220=CARTESIAN_POINT ( 'NONE',  ( -20.59592450876364111, 149.8464234248869786, 1.516103928358539354 ) ) ;
#2221=CARTESIAN_POINT ( 'NONE',  ( 22.12956052442012833, 150.1365687424457178, -0.8564216397177741857 ) ) ;
#2222=CARTESIAN_POINT ( 'NONE',  ( -4.319812470756069445, 11.96289413176387129, -1.686699837767231536 ) ) ;
#2223=CARTESIAN_POINT ( 'NONE',  ( -21.82265835376372820, 151.4369626909183637, -0.8820245880042205666 ) ) ;
#2225=EDGE_LOOP ( 'NONE', ( #11497, #24620, #32981, #34647 ) ) ;
#2226=CARTESIAN_POINT ( 'NONE',  ( -8.798540845223380202, 117.6856535658803864, -0.1377603156279901264 ) ) ;
#2227=DIRECTION ( 'NONE',  ( 4.017660918040594346E-17, -1.000000000000000000, -2.376309959284834438E-19 ) ) ;
#2228=CARTESIAN_POINT ( 'NONE',  ( -0.5414988153860592623, 119.6443647996702566, 0.5124704023889978810 ) ) ;
#2231=CARTESIAN_POINT ( 'NONE',  ( 18.33246729151843724, 150.1405190176936344, -1.740612831648467695 ) ) ;
#2232=CARTESIAN_POINT ( 'NONE',  ( -13.53750608930591959, 121.6867650304669013, -1.656372850109685047 ) ) ;
#2234=AXIS2_PLACEMENT_3D ( 'NONE', #11988, #28602, #8590 ) ;
#2235=EDGE_CURVE ( 'NONE', #1712, #17404, #41159, .T. ) ;
#2236=CARTESIAN_POINT ( 'NONE',  ( 7.748985956666678554, 122.1869765257964673, -0.4223483383238798017 ) ) ;
#2237=EDGE_LOOP ( 'NONE', ( #5526, #41184 ) ) ;
#2238=CARTESIAN_POINT ( 'NONE',  ( -12.92173176740960550, 125.9520529675768898, -1.821380522590920314 ) ) ;
#2239=CARTESIAN_POINT ( 'NONE',  ( 2.004873297308811253, -15.47002699807756265, 5.272742632645636363 ) ) ;
#2240=CARTESIAN_POINT ( 'NONE',  ( -4.156053678908833149, 118.2394346424153753, -0.3882629985390713134 ) ) ;
#2242=TOROIDAL_SURFACE ( 'NONE', #20571, 5.080000000000005400, 0.5080000000000000071 ) ;
#2244=CARTESIAN_POINT ( 'NONE',  ( 3.403275764582821772, 119.7942873563901713, 0.7909988017435812813 ) ) ;
#2246=CARTESIAN_POINT ( 'NONE',  ( 1.765626013768924807, -4.031643488171090972, 8.243228240708695864 ) ) ;
#2247=CARTESIAN_POINT ( 'NONE',  ( 15.80138807371428378, 145.9351319680867221, 0.6472794460535243877 ) ) ;
#2250=CARTESIAN_POINT ( 'NONE',  ( -0.3944222225486587186, 117.3993832485554094, 1.481046348585886241 ) ) ;
#2256=CARTESIAN_POINT ( 'NONE',  ( -1.829002187088467624, 116.5125207362610951, 0.06620492630546143120 ) ) ;
#2257=ORIENTED_EDGE ( 'NONE', *, *, #13992, .T. ) ;
#2259=CARTESIAN_POINT ( 'NONE',  ( 7.829869863957400256, 122.4471846315678079, -0.2494498989964459290 ) ) ;
#2262=CARTESIAN_POINT ( 'NONE',  ( 2.065091541609473058, 115.7028726122111948, -1.634879014494797334 ) ) ;
#2263=CARTESIAN_POINT ( 'NONE',  ( -9.301463764468643092, 124.2035065715909496, -0.4191708393134263577 ) ) ;
#2264=CARTESIAN_POINT ( 'NONE',  ( 5.365742231761132963, -12.30384844886438245, 1.459887348375163096 ) ) ;
#2265=CARTESIAN_POINT ( 'NONE',  ( -21.81117068996452701, 146.0876064316611860, 1.285479812297503965 ) ) ;
#2267=AXIS2_PLACEMENT_3D ( 'NONE', #13762, #23962, #39769 ) ;
#2268=CARTESIAN_POINT ( 'NONE',  ( 13.61156529719771768, 119.6358206793323404, 0.4233406866235921995 ) ) ;
#2269=CARTESIAN_POINT ( 'NONE',  ( 5.952364314655516075, 121.5461442270676287, 0.1560439712719428051 ) ) ;
#2271=CARTESIAN_POINT ( 'NONE',  ( -0.7497900579835341528, 31.49133049583988608, -0.6186479539722394838 ) ) ;
#2272=CARTESIAN_POINT ( 'NONE',  ( -14.87533653215399099, 120.3210621052586475, -0.3471466443384769174 ) ) ;
#2276=CARTESIAN_POINT ( 'NONE',  ( 8.299051278477378446, 119.9935803421679026, 1.450008147901515221 ) ) ;
#2278=CARTESIAN_POINT ( 'NONE',  ( 21.50396862640721807, 149.5883454796168621, 2.135274339423805401 ) ) ;
#2279=CARTESIAN_POINT ( 'NONE',  ( 20.18403667007061841, 149.6821479856479300, -1.616815787834455787 ) ) ;
#2280=CARTESIAN_POINT ( 'NONE',  ( 3.417104117279694098, -14.34023910220586906, -3.129441506049576383 ) ) ;
#2281=CARTESIAN_POINT ( 'NONE',  ( -0.3664415811652171340, 117.3568105388816321, -0.4447864970249671979 ) ) ;
#2282=CARTESIAN_POINT ( 'NONE',  ( 4.981436116827920202, 117.5302645918864073, -0.7678635597125215151 ) ) ;
#2284=CARTESIAN_POINT ( 'NONE',  ( 3.916844122728723843, 109.8065891650451249, 3.681372831196203066 ) ) ;
#2285=CARTESIAN_POINT ( 'NONE',  ( -4.254723467274468263, 155.8413357349917021, 0.07908073517333538693 ) ) ;
#2286=CARTESIAN_POINT ( 'NONE',  ( -10.36135117696322538, 155.6679353847891321, -2.160796112024522486 ) ) ;
#2287=CARTESIAN_POINT ( 'NONE',  ( 5.089472049306802859, -15.08631191614791334, 3.825519591672899455 ) ) ;
#2290=CARTESIAN_POINT ( 'NONE',  ( -0.6939310137895168262, 117.9496057704760972, -1.401774709011093245 ) ) ;
#2291=CIRCLE ( 'NONE', #254, 3.683000000000001162 ) ;
#2293=CARTESIAN_POINT ( 'NONE',  ( 17.74096168611281144, 140.4837523222294351, 2.437162785362842587 ) ) ;
#2295=CARTESIAN_POINT ( 'NONE',  ( -3.072892473034376959, 118.0774402770256444, -0.9619640826930374589 ) ) ;
#2297=CARTESIAN_POINT ( 'NONE',  ( -0.4698238578431560564, 109.1907409294041429, 4.006476130220050891 ) ) ;
#2298=CARTESIAN_POINT ( 'NONE',  ( -7.485859564062662841, -11.32103332335322499, -3.896386919873200405 ) ) ;
#2299=CARTESIAN_POINT ( 'NONE',  ( -0.01133107913651179230, 156.3792106723807649, 0.5670535347366658652 ) ) ;
#2301=CARTESIAN_POINT ( 'NONE',  ( 22.83860824214428575, 149.7823008822066697, -0.3949144739309157770 ) ) ;
#2304=CARTESIAN_POINT ( 'NONE',  ( -8.793872193760559952, 117.6946653426936962, -0.2789185993360862037 ) ) ;
#2306=CARTESIAN_POINT ( 'NONE',  ( -4.319384318635175468, 118.2117244580575601, 0.3218571067570579758 ) ) ;
#2307=CARTESIAN_POINT ( 'NONE',  ( -15.56076557482332490, 120.7233670659379214, -0.3109411287488703657 ) ) ;
#2310=CARTESIAN_POINT ( 'NONE',  ( -8.219350291155233634, 120.3834793910760510, -1.437375401876854308 ) ) ;
#2311=CARTESIAN_POINT ( 'NONE',  ( 0.09347673290359038989, 104.6144662015457385, -6.110098594576430564 ) ) ;
#2312=VECTOR ( 'NONE', #35901, 1000.000000000000000 ) ;
#2313=CARTESIAN_POINT ( 'NONE',  ( -2.711066548582671931, 120.7183352303693340, -0.3631387678457470014 ) ) ;
#2317=CARTESIAN_POINT ( 'NONE',  ( 4.037907715354051241, 27.70556447992504445, -2.267523456217593214 ) ) ;
#2319=DIRECTION ( 'NONE',  ( 0.9998004120163610509, 4.016384292689131511E-17, 0.01997839162482749689 ) ) ;
#2323=CARTESIAN_POINT ( 'NONE',  ( 7.785296811173602727, 122.6196569424365066, 0.2112341757090067940 ) ) ;
#2324=CARTESIAN_POINT ( 'NONE',  ( 4.466176584706416541, 22.48015689762229030, 1.290832665783417488 ) ) ;
#2325=CARTESIAN_POINT ( 'NONE',  ( 14.11323155926160666, 120.5239346615589540, 1.094216903015625242 ) ) ;
#2326=CARTESIAN_POINT ( 'NONE',  ( -2.496980690863166430, 104.6144662015454543, -4.139511689303219555 ) ) ;
#2327=CARTESIAN_POINT ( 'NONE',  ( 2.769760999665409340, -14.92388480464812872, 4.423285184949336646 ) ) ;
#2328=CARTESIAN_POINT ( 'NONE',  ( 13.73828690980672995, 121.6032371815301900, -1.070726600328922418 ) ) ;
#2329=CARTESIAN_POINT ( 'NONE',  ( -13.41341228195548574, 125.8771108566470502, 1.381187796596252459 ) ) ;
#2330=CARTESIAN_POINT ( 'NONE',  ( -3.182929088426432074, 26.46582164074821009, -3.363547984189534379 ) ) ;
#2331=CARTESIAN_POINT ( 'NONE',  ( -8.117713882137797654, 117.8329967196738153, -0.7633534655056999352 ) ) ;
#2333=CARTESIAN_POINT ( 'NONE',  ( -0.4659799999662124215, -3.540968264561009882, -0.8578381542037093466 ) ) ;
#2334=VERTEX_POINT ( 'NONE', #19409 ) ;
#2336=CARTESIAN_POINT ( 'NONE',  ( -15.41453346427796944, 143.5427300040290106, 0.2938895485367989946 ) ) ;
#2337=CARTESIAN_POINT ( 'NONE',  ( 4.239944546232853106, -14.55591092887127758, 4.867068800921800609 ) ) ;
#2338=CARTESIAN_POINT ( 'NONE',  ( 10.60975745311338692, 123.7931190674884050, -0.9249770984159892961 ) ) ;
#2340=VERTEX_POINT ( 'NONE', #25401 ) ;
#2342=CARTESIAN_POINT ( 'NONE',  ( 1.847932960219115017, 115.7026903297836355, 1.721340370546041720 ) ) ;
#2344=CARTESIAN_POINT ( 'NONE',  ( -4.734376237147363220, 117.7615504634655252, -1.071976335040407902 ) ) ;
#2345=CARTESIAN_POINT ( 'NONE',  ( 9.163388821854780986, 124.2347608867413413, 0.1831063163140474459 ) ) ;
#2347=CARTESIAN_POINT ( 'NONE',  ( 19.42145995676300529, 149.0830822498907082, 2.502058577541587781 ) ) ;
#2348=CARTESIAN_POINT ( 'NONE',  ( -6.431420355030265265E-14, 156.3034662015457172, 9.897580308537652682E-17 ) ) ;
#2352=CARTESIAN_POINT ( 'NONE',  ( 15.92845220574645992, 121.2232988859741027, -0.005268350931750691128 ) ) ;
#2353=CARTESIAN_POINT ( 'NONE',  ( -3.682264917456324671, 101.6934662015457320, -0.07358041635423923088 ) ) ;
#2355=CARTESIAN_POINT ( 'NONE',  ( 1.871273403468687091, -15.33072671635390982, 5.367422375955600344 ) ) ;
#2358=CARTESIAN_POINT ( 'NONE',  ( -4.892936701456676474, 117.7439554820887224, 0.7242864044084754704 ) ) ;
#2360=CARTESIAN_POINT ( 'NONE',  ( -0.8085694520786111950, 118.7629491485454025, 1.239635759033087314 ) ) ;
#2361=CARTESIAN_POINT ( 'NONE',  ( -5.604943360455993506, 118.2794056816863986, -1.161089605505309041 ) ) ;
#2362=CARTESIAN_POINT ( 'NONE',  ( -4.076169972524864349, 117.8719421043398370, -0.8561738758874234412 ) ) ;
#2363=CARTESIAN_POINT ( 'NONE',  ( 4.907969887652551932, 117.6281236953606566, 0.9703093435619695173 ) ) ;
#2364=CARTESIAN_POINT ( 'NONE',  ( 3.187143392547471255, -14.52651900126690876, 3.212499789951002604 ) ) ;
#2365=CARTESIAN_POINT ( 'NONE',  ( -0.8039382690413905408, 120.8419495465347069, 0.4447074479469317887 ) ) ;
#2366=B_SPLINE_CURVE_WITH_KNOTS ( 'NONE', 3,
 ( #29855, #23016, #20041, #32421, #3675, #13026, #16639, #39027 ),
 .UNSPECIFIED., .F., .F.,
 ( 4, 2, 2, 4 ),
 ( -5.999999999990650338E-08, 0.002398869872785528400, 0.003598334809178291988, 0.004797799745571056443 ),
 .UNSPECIFIED. ) ;
#2367=CARTESIAN_POINT ( 'NONE',  ( -4.595132424582489605, -6.828429371805166959, -0.5093739664528403877 ) ) ;
#2370=CARTESIAN_POINT ( 'NONE',  ( 3.449548791184131602, -12.83738641323306595, 1.613555780903996206 ) ) ;
#2371=CARTESIAN_POINT ( 'NONE',  ( 7.070147686296559542, 122.4340714744230496, 0.03157745743911253428 ) ) ;
#2372=CARTESIAN_POINT ( 'NONE',  ( -6.550279792842376381, 120.6599796251122427, -1.081144621291421082 ) ) ;
#2373=CARTESIAN_POINT ( 'NONE',  ( 5.150502540934155604, 116.8624420608055630, -0.04745483869977647207 ) ) ;
#2374=CARTESIAN_POINT ( 'NONE',  ( 0.1736941791105798827, 37.94092622093888423, 1.710797978410913300 ) ) ;
#2375=CARTESIAN_POINT ( 'NONE',  ( -1.232253463169212360, 115.7029489552889601, 1.695155158364408665 ) ) ;
#2376=CARTESIAN_POINT ( 'NONE',  ( -4.603678009535974169, 12.38766144714272066, -0.4343361176327051321 ) ) ;
#2377=CARTESIAN_POINT ( 'NONE',  ( 23.13755856728662508, 142.6111785389246336, 1.063510652947477153 ) ) ;
#2379=CARTESIAN_POINT ( 'NONE',  ( 1.773199387803063853, 105.1239297914698625, -5.032115150572375128 ) ) ;
#2380=CARTESIAN_POINT ( 'NONE',  ( 4.393930847168488363, -15.54918382657802312, 2.099248807845041309 ) ) ;
#2381=CARTESIAN_POINT ( 'NONE',  ( -8.434619947227433912, 156.6436466068687423, 1.738452918000226610 ) ) ;
#2382=CARTESIAN_POINT ( 'NONE',  ( 0.8148283262528154269, -11.57344599616632763, 0.5628321559398594687 ) ) ;
#2383=CARTESIAN_POINT ( 'NONE',  ( -0.4102451260098727293, 24.68626973166569982, 0.8857237506759965129 ) ) ;
#2387=ORIENTED_EDGE ( 'NONE', *, *, #38483, .F. ) ;
#2389=CARTESIAN_POINT ( 'NONE',  ( 3.997939770797755532, 117.2022048034790487, 1.046317678458332567 ) ) ;
#2390=CARTESIAN_POINT ( 'NONE',  ( -16.36402192804845512, 147.4903123243063590, 0.9458667783343727153 ) ) ;
#2392=CARTESIAN_POINT ( 'NONE',  ( 3.771727509258866906, -13.52648377956064429, 3.452274064300702605 ) ) ;
#2393=CARTESIAN_POINT ( 'NONE',  ( 17.96630583390848912, 147.4621342421176848, -1.576657649719084064 ) ) ;
#2394=CARTESIAN_POINT ( 'NONE',  ( -4.596153127770238100, 158.0471523224993859, -1.806220157282541150 ) ) ;
#2395=DIRECTION ( 'NONE',  ( -5.206863593109713661E-17, 1.000000000000000000, -1.077750396879097183E-30 ) ) ;
#2396=CARTESIAN_POINT ( 'NONE',  ( 2.994295736468014280, -14.77441112906794984, 3.968895097548184037 ) ) ;
#2397=CARTESIAN_POINT ( 'NONE',  ( -0.008457519121241168295, 39.20946620154573026, 0.4232488410869258977 ) ) ;
#2398=CARTESIAN_POINT ( 'NONE',  ( 0.6274479277950415490, 120.8480686026657196, -0.1451731132019951631 ) ) ;
#2400=FACE_OUTER_BOUND ( 'NONE', #27885, .T. ) ;
#2402=CARTESIAN_POINT ( 'NONE',  ( 1.733480476724572172, 35.69352191795299944, 2.306000102516378991 ) ) ;
#2404=CARTESIAN_POINT ( 'NONE',  ( -2.276242205911199523, 25.81146128161704567, -8.137376054096339573 ) ) ;
#2405=CARTESIAN_POINT ( 'NONE',  ( 12.69811389000554236, 152.1353413313561305, 1.627698677231679492 ) ) ;
#2406=FACE_OUTER_BOUND ( 'NONE', #31534, .T. ) ;
#2407=CARTESIAN_POINT ( 'NONE',  ( 5.755666581048775043, 159.1151184437813981, 0.09834937626042362935 ) ) ;
#2408=CARTESIAN_POINT ( 'NONE',  ( -3.556334529073039707, 108.6891572770382624, 3.980722479600266706 ) ) ;
#2409=CARTESIAN_POINT ( 'NONE',  ( 4.219463811995017188, -1.205994944679912306, -1.932895124392335573 ) ) ;
#2410=CARTESIAN_POINT ( 'NONE',  ( 9.118174893680169646, 124.1671967267183589, 0.1822028344259500054 ) ) ;
#2413=CARTESIAN_POINT ( 'NONE',  ( 6.464508713081113633, 4.871470569706378484, -5.424950676754816570 ) ) ;
#2415=CARTESIAN_POINT ( 'NONE',  ( 5.543381447479352353, 116.8569150493630673, -0.3072380764452348201 ) ) ;
#2416=CARTESIAN_POINT ( 'NONE',  ( -0.8524833535544004137, 121.9014879524050343, -0.3240522193994317401 ) ) ;
#2417=DIRECTION ( 'NONE',  ( 0.9998004120163609398, 0.000000000000000000, 0.01997839162482749689 ) ) ;
#2419=CARTESIAN_POINT ( 'NONE',  ( 6.518667233416390872, -10.50300228728784901, -5.332001816399940530 ) ) ;
#2420=CARTESIAN_POINT ( 'NONE',  ( 0.5321472206583588438, 118.1588881331645524, 0.9064177333157917849 ) ) ;
#2423=CARTESIAN_POINT ( 'NONE',  ( 0.7818436192037604426, 120.2878791493615296, -0.5419007644741467011 ) ) ;
#2424=CARTESIAN_POINT ( 'NONE',  ( -14.99898601413122812, 156.1447123740162226, 0.3355057415613001970 ) ) ;
#2429=CARTESIAN_POINT ( 'NONE',  ( -0.6511158059023082201, 120.9972571290847156, 0.05313384682098968442 ) ) ;
#2430=CARTESIAN_POINT ( 'NONE',  ( 4.717164877559400615, -15.39354034361711854, 4.072675418279473547 ) ) ;
#2431=CARTESIAN_POINT ( 'NONE',  ( -19.23923079580238493, 135.9655892003723636, 1.583918808943347800 ) ) ;
#2432=CARTESIAN_POINT ( 'NONE',  ( 14.20701772348842340, 121.1589565784038456, -0.8306491748466005021 ) ) ;
#2433=CARTESIAN_POINT ( 'NONE',  ( -4.247245584637960647, 22.75789413176893206, 1.861891798430825862 ) ) ;
#2435=CARTESIAN_POINT ( 'NONE',  ( -15.93800727448861210, 121.3860667298135070, -0.7466885930842023233 ) ) ;
#2437=ORIENTED_EDGE ( 'NONE', *, *, #31655, .F. ) ;
#2438=CARTESIAN_POINT ( 'NONE',  ( -0.005880675324201318707, 122.2435587914035295, 0.2942930402744693419 ) ) ;
#2441=CARTESIAN_POINT ( 'NONE',  ( -3.484775907859313904, 120.0787590019544098, 0.5801956493991066166 ) ) ;
#2443=CARTESIAN_POINT ( 'NONE',  ( 18.94125265848531825, 149.4003703399637288, -1.737001818219200411 ) ) ;
#2444=CARTESIAN_POINT ( 'NONE',  ( -3.077448401760676244, 117.9340107969418341, -0.8067720256249977240 ) ) ;
#2447=CARTESIAN_POINT ( 'NONE',  ( 9.503290916780938957, 123.5188755717998816, -0.5781397488420938480 ) ) ;
#2449=CARTESIAN_POINT ( 'NONE',  ( -7.499533598998470829, 156.0351187175861867, -1.911400249181836042 ) ) ;
#2450=CARTESIAN_POINT ( 'NONE',  ( 4.161657294200716173, -15.28457189793756754, -0.5145498944859950852 ) ) ;
#2451=CARTESIAN_POINT ( 'NONE',  ( -4.253023843880794352, 118.2240548184727089, -0.4605302936478082865 ) ) ;
#2453=CARTESIAN_POINT ( 'NONE',  ( -4.854232772743657165, 117.4081466956269395, 0.9971777887500445914 ) ) ;
#2454=CARTESIAN_POINT ( 'NONE',  ( 13.78929608597934831, 128.5353789189983900, 1.909663635655581615 ) ) ;
#2456=CARTESIAN_POINT ( 'NONE',  ( -5.746845633966660039, 1.589972373264088246, -6.161128625535090109 ) ) ;
#2457=CARTESIAN_POINT ( 'NONE',  ( 5.263358945736606564, 121.3020066425206807, 0.2711714534586360248 ) ) ;
#2459=EDGE_CURVE ( 'NONE', #35057, #21265, #38404, .T. ) ;
#2462=CARTESIAN_POINT ( 'NONE',  ( -0.4467517591321596981, 117.3993820567716142, 1.478547820748352448 ) ) ;
#2465=CARTESIAN_POINT ( 'NONE',  ( -7.971903862541391383, 121.6201495393203800, -1.129789807432725279 ) ) ;
#2469=CARTESIAN_POINT ( 'NONE',  ( -8.048392397359151573, 158.6767594643193604, 0.003330354478299033406 ) ) ;
#2473=CARTESIAN_POINT ( 'NONE',  ( -6.036974320247253445, 121.4378217842577783, -0.1460419162834154239 ) ) ;
#2475=EDGE_LOOP ( 'NONE', ( #14245, #27709 ) ) ;
#2476=CARTESIAN_POINT ( 'NONE',  ( 2.411409958355576588, 115.7029272791032781, -1.607700095068150592 ) ) ;
#2477=CARTESIAN_POINT ( 'NONE',  ( -1.577167647222679436, 156.2580631240469415, -0.1709568888171391354 ) ) ;
#2478=CARTESIAN_POINT ( 'NONE',  ( 3.928490385995774936, -14.72231570353084429, 5.141255514400237203 ) ) ;
#2479=CARTESIAN_POINT ( 'NONE',  ( -13.78108617287063353, 121.3979351292862816, 1.006787891297146409 ) ) ;
#2481=CARTESIAN_POINT ( 'NONE',  ( 15.16003043525265248, 156.1230782244120121, 0.5028385762316639473 ) ) ;
#2482=CARTESIAN_POINT ( 'NONE',  ( 1.555436498865683026, 156.2615671560531609, 0.1081568999835344491 ) ) ;
#2484=CARTESIAN_POINT ( 'NONE',  ( -0.9658880162092680077, 3.969362202269336226, 0.1338930134723784471 ) ) ;
#2485=CARTESIAN_POINT ( 'NONE',  ( -3.714261611334668700, 116.6275173757784813, -0.1151834636560011560 ) ) ;
#2490=CARTESIAN_POINT ( 'NONE',  ( 8.375419374246291682, 119.6241210904774874, 1.419676489699448929 ) ) ;
#2491=CARTESIAN_POINT ( 'NONE',  ( 4.409325496788552456, -14.99073161069602911, -1.440227693534741782 ) ) ;
#2492=CARTESIAN_POINT ( 'NONE',  ( 13.41577631804572412, 120.9245410081625209, 1.450210030139598594 ) ) ;
#2493=CARTESIAN_POINT ( 'NONE',  ( 6.603547431282811964, 157.6773268839678508, -1.653176294384505418 ) ) ;
#2494=CARTESIAN_POINT ( 'NONE',  ( 1.818839793882075728, -13.69063247836898611, -4.255424433905749204 ) ) ;
#2495=CARTESIAN_POINT ( 'NONE',  ( -18.89746971955500854, 128.6554162386474047, -1.621015360058189358 ) ) ;
#2496=CARTESIAN_POINT ( 'NONE',  ( 4.772809636307222547, 117.7613819223621334, -0.8822393946220054017 ) ) ;
#2497=CARTESIAN_POINT ( 'NONE',  ( 5.451337559846638037, 117.5214873295501405, 0.8265904065678292278 ) ) ;
#2498=CARTESIAN_POINT ( 'NONE',  ( -15.74722489594621777, 146.9052959264698757, -0.08484200870240315995 ) ) ;
#2499=CARTESIAN_POINT ( 'NONE',  ( -9.618126185770362824, 121.1143850344477215, -1.566364589618396197 ) ) ;
#2500=CARTESIAN_POINT ( 'NONE',  ( 3.779930934242227369, -15.54964480308611208, 5.049599803682278676 ) ) ;
#2501=CARTESIAN_POINT ( 'NONE',  ( 4.732128828421237721, 118.5931160184169073, 1.019631307593062974 ) ) ;
#2502=AXIS2_PLACEMENT_3D ( 'NONE', #22755, #650, #20408 ) ;
#2507=CARTESIAN_POINT ( 'NONE',  ( 0.4867666382966649441, 119.1670848682014281, 0.5956043695837971441 ) ) ;
#2509=CARTESIAN_POINT ( 'NONE',  ( 4.701335245683265995, 117.7901595215496258, 1.087246424278794477 ) ) ;
#2510=CARTESIAN_POINT ( 'NONE',  ( -2.738288815229088069, 121.4869043954268903, 0.2316524989510643784 ) ) ;
#2511=CARTESIAN_POINT ( 'NONE',  ( 8.265420891810833837, -5.467761657695628053, -1.740095136296691214 ) ) ;
#2512=CARTESIAN_POINT ( 'NONE',  ( 12.19070665030413281, 151.9982576965888654, 1.154562729007634792 ) ) ;
#2514=CARTESIAN_POINT ( 'NONE',  ( 22.99243123797615951, 146.5883926500602001, -0.5216133500896583675 ) ) ;
#2520=CARTESIAN_POINT ( 'NONE',  ( 5.149530563680449369, 114.9388725758769709, -1.533339281550282207 ) ) ;
#2524=CARTESIAN_POINT ( 'NONE',  ( 4.622740841563977021, 119.7018045729082587, -0.7338303597469464368 ) ) ;
#2525=CARTESIAN_POINT ( 'NONE',  ( -0.6715300310780568660, 105.9424719104300436, -5.313162126831953103 ) ) ;
#2527=CARTESIAN_POINT ( 'NONE',  ( -7.694217360203188250, 122.2455405838764335, -0.6631844599531893092 ) ) ;
#2529=CARTESIAN_POINT ( 'NONE',  ( 23.44919332464148454, 146.8469795362756258, 0.4944523877934686173 ) ) ;
#2531=CARTESIAN_POINT ( 'NONE',  ( 1.325333094648095011, 19.28447512809159292, -4.440015753949128730 ) ) ;
#2533=CARTESIAN_POINT ( 'NONE',  ( -5.008697454415233175, 117.3984623471881292, 0.7756180019310896512 ) ) ;
#2534=LINE ( 'NONE', #37667, #7479 ) ;
#2537=CARTESIAN_POINT ( 'NONE',  ( -6.991991784399644416, 121.9291801892613734, 0.01265143332250801347 ) ) ;
#2538=CARTESIAN_POINT ( 'NONE',  ( -4.295268622494708310, 18.69437521248495671, 1.722957355393906598 ) ) ;
#2539=CARTESIAN_POINT ( 'NONE',  ( 3.132853369507592411, 159.3671203531505114, 0.7742396785067985343 ) ) ;
#2541=CARTESIAN_POINT ( 'NONE',  ( 2.969447359227861405, -13.80100253337253946, 0.9847735008004718793 ) ) ;
#2542=CARTESIAN_POINT ( 'NONE',  ( 12.10120965742738441, 156.5645100661158153, -1.400626166162074693 ) ) ;
#2543=CARTESIAN_POINT ( 'NONE',  ( -15.45240368193238290, 131.3329289045130679, 1.560586129702050684 ) ) ;
#2544=CARTESIAN_POINT ( 'NONE',  ( 1.027636191897724816, 24.96647085856908532, -4.506105791511280323 ) ) ;
#2545=CARTESIAN_POINT ( 'NONE',  ( -20.30524341716979464, 152.5255278361454145, -1.346157490925044220 ) ) ;
#2546=CARTESIAN_POINT ( 'NONE',  ( -0.9748693424575083366, -1.807339741155509660, 0.05984739681150109264 ) ) ;
#2549=CARTESIAN_POINT ( 'NONE',  ( -5.244198393876603248, 121.2166884500396833, 0.1799464770355448662 ) ) ;
#2550=CARTESIAN_POINT ( 'NONE',  ( 3.373230072307711325, -14.96631539557509427, 5.513067843180951222 ) ) ;
#2551=CARTESIAN_POINT ( 'NONE',  ( 16.86000824444443325, 147.6865045845431723, -1.246329746872388622 ) ) ;
#2553=CARTESIAN_POINT ( 'NONE',  ( 0.8518381835474642116, 115.7029491485453150, 1.752614281141236852 ) ) ;
#2555=CARTESIAN_POINT ( 'NONE',  ( -4.745317454387270040, 117.7319129980786840, -1.087429732257703119 ) ) ;
#2556=CARTESIAN_POINT ( 'NONE',  ( 8.041889123127029748, 122.8518031662551948, 0.1606960833125207211 ) ) ;
#2558=CARTESIAN_POINT ( 'NONE',  ( 2.271387047178972995, 118.5910164976458532, 0.7981300483413861224 ) ) ;
#2562=CARTESIAN_POINT ( 'NONE',  ( 0.004910621514677531059, 156.3161161488371533, -0.2457475809811480449 ) ) ;
#2564=CARTESIAN_POINT ( 'NONE',  ( 15.71820687823851159, 121.0099257824619627, -0.007297392930742286829 ) ) ;
#2568=CARTESIAN_POINT ( 'NONE',  ( 1.999402950501548482, -15.06364915300781249, 5.759057916224358920 ) ) ;
#2569=EDGE_CURVE ( 'NONE', #18840, #37319, #31325, .T. ) ;
#2572=CARTESIAN_POINT ( 'NONE',  ( -4.623643573307993471, 118.0606194745544997, 0.5411930361001372480 ) ) ;
#2574=CARTESIAN_POINT ( 'NONE',  ( -1.110165644321341460, 118.7629491485454025, 1.217933052008355554 ) ) ;
#2575=CARTESIAN_POINT ( 'NONE',  ( 6.006868049574960899, 119.2300460209637407, -1.027315805567093898 ) ) ;
#2576=CARTESIAN_POINT ( 'NONE',  ( -1.786380800136868618, 106.8720524443079967, -4.898415999051429992 ) ) ;
#2577=CARTESIAN_POINT ( 'NONE',  ( 4.760004222690300324, 117.7660308155148385, 1.056159522374921167 ) ) ;
#2579=CARTESIAN_POINT ( 'NONE',  ( -0.3799753109755704683, 121.9236798544226730, 0.3295597595137201297 ) ) ;
#2580=AXIS2_PLACEMENT_3D ( 'NONE', #3590, #3800, #33186 ) ;
#2581=CARTESIAN_POINT ( 'NONE',  ( 3.745621265272091716, -10.50169880513956322, -2.708184146228840294 ) ) ;
#2582=CARTESIAN_POINT ( 'NONE',  ( 4.853781638280933564, 117.4081357529187528, -0.9972794204146671060 ) ) ;
#2584=CARTESIAN_POINT ( 'NONE',  ( 2.741226102065047687, 109.4146836159258669, -3.767795064178312892 ) ) ;
#2585=CARTESIAN_POINT ( 'NONE',  ( -17.50754485026813256, 146.9817191466759141, -2.164442782320840308 ) ) ;
#2586=CARTESIAN_POINT ( 'NONE',  ( 6.075452776647331632, 121.4405985945170130, 0.1207385346877154486 ) ) ;
#2587=CARTESIAN_POINT ( 'NONE',  ( -1.386537629721184883, 36.36735770096321829, 2.585368322340788172 ) ) ;
#2588=CARTESIAN_POINT ( 'NONE',  ( -3.567118561776222219, 115.7029539238351816, 1.489719890727359441 ) ) ;
#2589=CARTESIAN_POINT ( 'NONE',  ( -3.609430071560130848, 3.966570591990036032, 2.889066364458971137 ) ) ;
#2590=CARTESIAN_POINT ( 'NONE',  ( 14.49621620279156708, 120.3567457872619997, 0.7930654045677066888 ) ) ;
#2591=VERTEX_POINT ( 'NONE', #36671 ) ;
#2592=CARTESIAN_POINT ( 'NONE',  ( 1.151853689421055149, 104.6144662015457811, -4.696227499264772121 ) ) ;
#2593=CARTESIAN_POINT ( 'NONE',  ( 3.754758974503722868, -15.60599068302642678, 3.401513958955031836 ) ) ;
#2594=CARTESIAN_POINT ( 'NONE',  ( -12.19007131875819283, 155.0146010091537221, 1.747022140133383417 ) ) ;
#2595=CARTESIAN_POINT ( 'NONE',  ( -0.8611515851325071136, 16.54815110656625166, -0.4551624184793268135 ) ) ;
#2596=CARTESIAN_POINT ( 'NONE',  ( 0.7643174330569572072, 9.588751494893990923, -0.6113830025413525826 ) ) ;
#2599=DIRECTION ( 'NONE',  ( -0.01997839162482749342, -1.040247600000944484E-18, 0.9998004120163608288 ) ) ;
#2600=CARTESIAN_POINT ( 'NONE',  ( 2.588518934355891865, 109.4146836159258669, 3.874296054094246600 ) ) ;
#2602=CARTESIAN_POINT ( 'NONE',  ( -4.675694769581217436, 155.9604050671876792, 0.8934998238159543860 ) ) ;
#2603=DIRECTION ( 'NONE',  ( 0.9998004120163610509, 5.205824365704083805E-17, 0.01997839162482760444 ) ) ;
#2604=CARTESIAN_POINT ( 'NONE',  ( 3.213330078112610177, -12.77372567451348573, 1.108568753689092690 ) ) ;
#2605=CARTESIAN_POINT ( 'NONE',  ( 16.98580377952195875, 140.1729163700083518, -1.602912605581681582 ) ) ;
#2606=CARTESIAN_POINT ( 'NONE',  ( -18.80649797369244425, 150.3568762430427910, -2.459390564378663768 ) ) ;
#2608=CARTESIAN_POINT ( 'NONE',  ( 7.971934240893917334, 121.6199950850121496, 1.129854539203151154 ) ) ;
#2609=CARTESIAN_POINT ( 'NONE',  ( 4.074910602682932925, 118.2429491485453354, -0.1454311599470142491 ) ) ;
#2610=CARTESIAN_POINT ( 'NONE',  ( 15.77919907218838702, 145.7191243368997675, -0.01646358168407709502 ) ) ;
#2612=CARTESIAN_POINT ( 'NONE',  ( 2.768561164044480272, -13.57843041371762460, 0.3119852368007841603 ) ) ;
#2613=FACE_BOUND ( 'NONE', #9801, .T. ) ;
#2616=CARTESIAN_POINT ( 'NONE',  ( -6.895871986696200828, 19.14539577913392066, 4.887076909655228896 ) ) ;
#2617=CARTESIAN_POINT ( 'NONE',  ( 11.45052794940109742, 153.2879862121713757, 1.711174725579351685 ) ) ;
#2619=CARTESIAN_POINT ( 'NONE',  ( 23.40703704692311504, 142.8142681763856388, 0.3922439843285879801 ) ) ;
#2620=CARTESIAN_POINT ( 'NONE',  ( -4.828659834973932696, 112.7831754354443348, 2.372633244901563465 ) ) ;
#2623=CARTESIAN_POINT ( 'NONE',  ( 15.52687642492882070, 147.5330934759543879, 0.3102639428822866474 ) ) ;
#2624=CARTESIAN_POINT ( 'NONE',  ( 5.057098040335121780, -7.207523253290371024, 6.778223571298113370 ) ) ;
#2625=CARTESIAN_POINT ( 'NONE',  ( 8.758500698815293362, 117.9284149219992912, -0.3497163369972981495 ) ) ;
#2626=CARTESIAN_POINT ( 'NONE',  ( 0.07831152689639594988, 109.4728569552520838, -3.919029035233729363 ) ) ;
#2629=CARTESIAN_POINT ( 'NONE',  ( 8.408789229792210662, -11.58028725773715628, 0.1531400924992341317 ) ) ;
#2630=CARTESIAN_POINT ( 'NONE',  ( 0.1815206473440567347, 118.1588882195315477, 0.9095569039822347657 ) ) ;
#2632=CARTESIAN_POINT ( 'NONE',  ( 3.205266406700632675, -14.32095172213143641, 3.103221849221895035 ) ) ;
#2633=CARTESIAN_POINT ( 'NONE',  ( 0.3786798576916004522, 121.5961256765096152, -0.3764709079149203830 ) ) ;
#2634=CARTESIAN_POINT ( 'NONE',  ( -13.17783411699405605, 156.9583929045107595, 0.4564371790988702715 ) ) ;
#2638=FACE_BOUND ( 'NONE', #27144, .T. ) ;
#2639=CARTESIAN_POINT ( 'NONE',  ( -5.961919564881704936, 121.5457840906684908, -0.04491390701585241951 ) ) ;
#2640=CARTESIAN_POINT ( 'NONE',  ( 2.074264724554232053, -15.58053249244904848, 5.900626476732238501 ) ) ;
#2641=CARTESIAN_POINT ( 'NONE',  ( -11.80709641148050437, 120.8928578745602209, 1.148978701482600062 ) ) ;
#2642=CARTESIAN_POINT ( 'NONE',  ( 14.55736095115755724, 121.4416029531759591, -0.8377414905974124304 ) ) ;
#2643=CARTESIAN_POINT ( 'NONE',  ( -1.544744425833544099, 4.816215111148435923, 4.377641278133862279 ) ) ;
#2647=CARTESIAN_POINT ( 'NONE',  ( -5.517349593794012463, 28.10803576007639037, 0.4164286583522215368 ) ) ;
#2648=CARTESIAN_POINT ( 'NONE',  ( -9.755129750886823103, 122.6450757329969434, 0.9482731561257335962 ) ) ;
#2649=DIRECTION ( 'NONE',  ( -0.08582482245076952787, -4.468781434041244531E-18, -0.9963102427714443099 ) ) ;
#2651=CARTESIAN_POINT ( 'NONE',  ( 18.65843730539381085, 148.7425187291823363, -1.723213218779726441 ) ) ;
#2653=CARTESIAN_POINT ( 'NONE',  ( -4.923251988582253880, 158.4862278396301178, -1.623903838676621358 ) ) ;
#2655=CARTESIAN_POINT ( 'NONE',  ( 8.332953031246793429, 122.7091975629380585, -0.3740907431100289893 ) ) ;
#2656=ORIENTED_EDGE ( 'NONE', *, *, #19285, .F. ) ;
#2657=CARTESIAN_POINT ( 'NONE',  ( -18.11030164959035815, 147.2296321676236062, -2.344458923443068166 ) ) ;
#2658=CARTESIAN_POINT ( 'NONE',  ( 3.256234316240316229, -15.49904601598017706, 3.966862439782909533 ) ) ;
#2659=CARTESIAN_POINT ( 'NONE',  ( -4.065972646788793554, 118.2429491485453070, -0.3080848862740693250 ) ) ;
#2661=CARTESIAN_POINT ( 'NONE',  ( -4.866475353371516377, 117.6758284370217211, 0.8741549091480164124 ) ) ;
#2662=CARTESIAN_POINT ( 'NONE',  ( 17.54535662205662305, 147.9903219242534078, 2.232389162988360987 ) ) ;
#2663=CARTESIAN_POINT ( 'NONE',  ( 1.122158211225882551, 34.81801111161350804, -0.09678150280622697943 ) ) ;
#2665=CARTESIAN_POINT ( 'NONE',  ( -2.029258473809828711, 23.83235028914373288, 4.157303687431403993 ) ) ;
#2666=CARTESIAN_POINT ( 'NONE',  ( 13.62587875280878613, 150.2122286517991085, 0.5925390977946543014 ) ) ;
#2671=CARTESIAN_POINT ( 'NONE',  ( -1.049266738966821100, 117.3993836600691338, 1.438942573323084062 ) ) ;
#2679=CARTESIAN_POINT ( 'NONE',  ( -21.89150648822684175, 151.4414241944827495, -0.2106634337039129667 ) ) ;
#2682=CARTESIAN_POINT ( 'NONE',  ( 6.944753498707676442, 121.9193963520664568, -0.07675506838304683999 ) ) ;
#2684=ORIENTED_EDGE ( 'NONE', *, *, #3283, .T. ) ;
#2685=CARTESIAN_POINT ( 'NONE',  ( 1.944750467032260843, 115.7029431225055447, -1.643889904354718601 ) ) ;
#2686=CARTESIAN_POINT ( 'NONE',  ( -11.96249418807715337, 130.4318746828361100, -0.4433914376541253088 ) ) ;
#2687=CARTESIAN_POINT ( 'NONE',  ( 5.272318886577700425, -12.73938755324596706, 2.198237985477529577 ) ) ;
#2688=CARTESIAN_POINT ( 'NONE',  ( -4.947803190686721919, 118.0342071775839941, 0.7636311594363676125 ) ) ;
#2690=CARTESIAN_POINT ( 'NONE',  ( 15.38042280020263597, 120.6961994932685798, 0.5371754898667550071 ) ) ;
#2691=CARTESIAN_POINT ( 'NONE',  ( 15.52499971488611052, 147.5364857366073750, 0.4437653257291759856 ) ) ;
#2692=CARTESIAN_POINT ( 'NONE',  ( -4.886900518740532995, 117.7626867099871930, 0.6841186648097229428 ) ) ;
#2693=CARTESIAN_POINT ( 'NONE',  ( -0.9549105556349912760, 13.03813504644791976, -0.2014467441264284064 ) ) ;
#2694=CARTESIAN_POINT ( 'NONE',  ( -23.10830587629928701, 149.8995197111492814, -0.5387578213853484455 ) ) ;
#2698=CARTESIAN_POINT ( 'NONE',  ( -5.639246004011813973, 117.7088169978700165, 0.7550884821962456916 ) ) ;
#2699=ADVANCED_FACE ( 'NONE', ( #3885 ), #22115, .T. ) ;
#2701=CARTESIAN_POINT ( 'NONE',  ( 17.24095835932491383, 153.8449085212272678, 1.984086636893841460 ) ) ;
#2702=CARTESIAN_POINT ( 'NONE',  ( 13.96578288426879944, 123.5874490550988014, -1.342688313448305415 ) ) ;
#2703=CARTESIAN_POINT ( 'NONE',  ( -8.202033116754899211, 17.84503447943221843, -1.958624548878737492 ) ) ;
#2704=CARTESIAN_POINT ( 'NONE',  ( -22.06201951068911882, 142.1041199125429557, -1.893492075525809115 ) ) ;
#2705=CARTESIAN_POINT ( 'NONE',  ( 4.712915829303078397, 117.8947333706760645, -0.7958967948868717057 ) ) ;
#2706=CARTESIAN_POINT ( 'NONE',  ( 5.402623002109011807, 117.1681999988027911, 0.9004238350613811281 ) ) ;
#2708=CARTESIAN_POINT ( 'NONE',  ( -4.236260012103463701, 155.8470599587123502, 0.007037385900262245995 ) ) ;
#2709=CARTESIAN_POINT ( 'NONE',  ( -7.518309192797278051, 120.1328256275108828, -1.363123692563724232 ) ) ;
#2712=CARTESIAN_POINT ( 'NONE',  ( 5.755466747078162193, -14.97439463182292840, 1.832642420680269613 ) ) ;
#2713=CARTESIAN_POINT ( 'NONE',  ( 4.787502628886421974, 118.5931160184169073, 0.9394847329858636575 ) ) ;
#2714=EDGE_CURVE ( 'NONE', #19419, #30834, #21788, .T. ) ;
#2715=CARTESIAN_POINT ( 'NONE',  ( -3.116415352288768759, 118.1651002505946764, -0.7896273181905824057 ) ) ;
#2717=CARTESIAN_POINT ( 'NONE',  ( 18.92921826512563754, 147.2511928822236769, 2.484298966539742359 ) ) ;
#2718=CARTESIAN_POINT ( 'NONE',  ( -15.72550100231844006, 145.6881679641599021, -0.3142329346387510713 ) ) ;
#2720=CARTESIAN_POINT ( 'NONE',  ( -5.284455934300128277, 122.2451909684448310, 0.05007199584899540284 ) ) ;
#2721=CARTESIAN_POINT ( 'NONE',  ( -5.729511908840139611, -2.247816343263548511, -6.181412921048518250 ) ) ;
#2722=CARTESIAN_POINT ( 'NONE',  ( 13.47315239181489055, 134.2048320552371763, 1.097568958570526387 ) ) ;
#2723=CARTESIAN_POINT ( 'NONE',  ( 13.17783411699392815, 156.9583929045107595, -0.4564371790988700495 ) ) ;
#2726=CARTESIAN_POINT ( 'NONE',  ( -2.177780859526504464, 116.2183971991849063, -0.1591026366872899112 ) ) ;
#2727=VECTOR ( 'NONE', #26317, 1000.000000000000000 ) ;
#2729=CARTESIAN_POINT ( 'NONE',  ( -14.91134437181082717, 120.3281135998953459, -0.2979641475761141134 ) ) ;
#2730=ORIENTED_EDGE ( 'NONE', *, *, #25110, .T. ) ;
#2732=CARTESIAN_POINT ( 'NONE',  ( -4.472347561024065499, 119.5957418731920825, -0.9224546268043867236 ) ) ;
#2733=CARTESIAN_POINT ( 'NONE',  ( -5.329475387727676150, 116.0444662015457311, -0.2797177882896795809 ) ) ;
#2734=CARTESIAN_POINT ( 'NONE',  ( -8.743035643995797912, 123.3024417045633498, -0.5730362264965973562 ) ) ;
#2735=CARTESIAN_POINT ( 'NONE',  ( -6.997652642833405601, 121.9526520506185676, -0.1398297539000763479 ) ) ;
#2736=CARTESIAN_POINT ( 'NONE',  ( 22.76738278397251136, 137.3906169244638136, 0.4549464913834384561 ) ) ;
#2737=VERTEX_POINT ( 'NONE', #27162 ) ;
#2738=CARTESIAN_POINT ( 'NONE',  ( -0.8823465807374654135, 5.041073445128725794, 4.537322665494407659 ) ) ;
#2740=CARTESIAN_POINT ( 'NONE',  ( -4.923150864362091816, 117.4111644033810364, 0.9486898195072187567 ) ) ;
#2744=CARTESIAN_POINT ( 'NONE',  ( -7.015191267815401588, 121.6841711688571905, 0.3965527081801285547 ) ) ;
#2745=CARTESIAN_POINT ( 'NONE',  ( 3.287934792154566299, 21.71798121574904172, 3.254339964430349230 ) ) ;
#2747=CARTESIAN_POINT ( 'NONE',  ( 14.55652921886106022, 120.9595740141730289, 1.205336527378881417 ) ) ;
#2748=CARTESIAN_POINT ( 'NONE',  ( -0.09923067678108841994, 104.6144662015456248, -4.835257341052268565 ) ) ;
#2749=CARTESIAN_POINT ( 'NONE',  ( 2.664052010559913253, -13.52006206191685322, 0.08958796903007473778 ) ) ;
#2750=CARTESIAN_POINT ( 'NONE',  ( 4.957730756931379545, 118.1424809852657773, -0.7901079947696816319 ) ) ;
#2751=CARTESIAN_POINT ( 'NONE',  ( -18.42722449710342048, 147.3262642721504960, 1.661950199828387875 ) ) ;
#2752=CARTESIAN_POINT ( 'NONE',  ( -0.2501726036287156840, 25.39126883368370002, -4.616104092076634302 ) ) ;
#2753=CARTESIAN_POINT ( 'NONE',  ( -19.50329963654034060, 128.7319734376252143, -1.320013405138365181 ) ) ;
#2756=CARTESIAN_POINT ( 'NONE',  ( -9.094799215789770130, 123.6795089456687577, 0.2292421281602769478 ) ) ;
#2758=CARTESIAN_POINT ( 'NONE',  ( 2.103176148521523459, -15.33886314497087611, 5.964097425510020756 ) ) ;
#2759=CARTESIAN_POINT ( 'NONE',  ( 0.2925446776148338812, 115.7029491485453860, 1.764546176662535659 ) ) ;
#2761=CARTESIAN_POINT ( 'NONE',  ( -4.585787403902434001, 118.0415163171067832, -0.8248535577628890447 ) ) ;
#2762=CARTESIAN_POINT ( 'NONE',  ( 9.118174893680169646, 124.1671967267183589, 0.1822028344259499499 ) ) ;
#2763=ORIENTED_EDGE ( 'NONE', *, *, #24028, .F. ) ;
#2764=CARTESIAN_POINT ( 'NONE',  ( 3.201321489863619529, 118.6508749770327995, 0.9018090777949859804 ) ) ;
#2768=CARTESIAN_POINT ( 'NONE',  ( 5.007034960109912447, 117.4001718673160468, -0.7827158424842978190 ) ) ;
#2769=CARTESIAN_POINT ( 'NONE',  ( 5.719359222665080011, 159.1232349745254453, -0.1048325176007952469 ) ) ;
#2774=CARTESIAN_POINT ( 'NONE',  ( 2.129294072315917052, -15.09917489183357198, 5.751238432448014137 ) ) ;
#2777=CARTESIAN_POINT ( 'NONE',  ( -4.690708456685893424, 118.0052805208300413, 0.5844499725986116445 ) ) ;
#2778=B_SPLINE_SURFACE_WITH_KNOTS ( 'NONE', 1, 3, ( 
 ( #13093, #12884, #26293, #38878, #19683, #32699, #32276, #32060, #22867, #3535, #19269, #9282, #19899, #38675 ),
 ( #16494, #35690, #3313, #29500, #26085, #19055, #39301, #28867, #12474, #340, #9481, #22445, #6499, #23080 ) ),
 .UNSPECIFIED., .F., .F., .F.,
 ( 2, 2 ),
 ( 4, 3, 2, 2, 3, 4 ),
 ( 0.000000000000000000, 1.000000000000000000 ),
 ( -0.01000000000000000021, 0.000000000000000000, 0.2500000000000000000, 0.5000000000000000000, 1.000000000000000000, 1.016448397156630046 ),
 .UNSPECIFIED. ) ;
#2781=CARTESIAN_POINT ( 'NONE',  ( -1.060522822118417086, 118.7629491485454167, -1.261313721580232805 ) ) ;
#2782=CARTESIAN_POINT ( 'NONE',  ( -8.390773680403903256, 119.5504231609327093, -1.407582209411027296 ) ) ;
#2783=CARTESIAN_POINT ( 'NONE',  ( -6.294717182677882938, 121.9812576474260055, -0.2818399057506478789 ) ) ;
#2784=CARTESIAN_POINT ( 'NONE',  ( 4.656059677840232780, 118.0096173734262806, 0.7826279643646096851 ) ) ;
#2786=CARTESIAN_POINT ( 'NONE',  ( -12.05573777011654890, 128.3964238929853252, -1.202367467897995867 ) ) ;
#2787=CARTESIAN_POINT ( 'NONE',  ( -4.187759052228169132, -5.978784877027076838, 2.003160513425938483 ) ) ;
#2790=CARTESIAN_POINT ( 'NONE',  ( 5.927223324825469319, 118.9825038774357466, -0.3493763292145122268 ) ) ;
#2791=CARTESIAN_POINT ( 'NONE',  ( -10.71484998910098341, 123.2317624570580534, -1.496280440855931815 ) ) ;
#2793=CARTESIAN_POINT ( 'NONE',  ( -2.714942736419990510, 34.21952868525605851, 3.834609254973532444 ) ) ;
#2795=CARTESIAN_POINT ( 'NONE',  ( 4.627880361116947228, 7.839802885307131319, -0.3238752845059330032 ) ) ;
#2796=CARTESIAN_POINT ( 'NONE',  ( 22.25501949494949372, 137.0232865695268458, 1.151097374996565614 ) ) ;
#2798=CARTESIAN_POINT ( 'NONE',  ( 4.372714196296951350, 104.6144662015534834, -3.059664787259841923 ) ) ;
#2799=CARTESIAN_POINT ( 'NONE',  ( 3.418015357486716699, -15.48303273933827917, 3.654867857709153345 ) ) ;
#2800=CARTESIAN_POINT ( 'NONE',  ( -19.06420633224123407, 149.2349160008635351, 1.736338202726219526 ) ) ;
#2801=CARTESIAN_POINT ( 'NONE',  ( 0.1071387893147941056, 24.31912984647217968, -0.9680276682219529638 ) ) ;
#2802=CARTESIAN_POINT ( 'NONE',  ( 0.9699771559235883522, 8.716109271805494885, -0.1015519487743763993 ) ) ;
#2805=CARTESIAN_POINT ( 'NONE',  ( -4.469853575504566301, 31.48943071249222214, -0.6923489671027511783 ) ) ;
#2806=CARTESIAN_POINT ( 'NONE',  ( 6.931894935422154624, 124.3275308867733600, 0.1497658092569641719 ) ) ;
#2807=CARTESIAN_POINT ( 'NONE',  ( -15.79191249938960162, 148.1776054874778197, 0.7900072561285060857 ) ) ;
#2808=DIRECTION ( 'NONE',  ( -0.5064479475276348897, 0.8622111466057285067, -0.01012003527073121814 ) ) ;
#2809=CARTESIAN_POINT ( 'NONE',  ( 2.845270837621566518, -14.55731563485390723, 4.954299782322259205 ) ) ;
#2810=CARTESIAN_POINT ( 'NONE',  ( 17.90094693680099169, 147.7668373613703352, -1.576197898085537563 ) ) ;
#2811=CARTESIAN_POINT ( 'NONE',  ( -4.492596771379940179, 157.9011380394538833, -1.833279187945892730 ) ) ;
#2815=CARTESIAN_POINT ( 'NONE',  ( 7.954247503138311970, 121.7101248947803356, 1.090747642478792745 ) ) ;
#2816=CARTESIAN_POINT ( 'NONE',  ( 4.074910602682932925, 118.2429491485453354, -0.1454311599470142491 ) ) ;
#2817=CARTESIAN_POINT ( 'NONE',  ( 15.57078937218316206, 147.5402044622178153, -0.01782986306386590697 ) ) ;
#2822=CARTESIAN_POINT ( 'NONE',  ( -3.928768625441322104, 16.54256788600693895, -7.448509604454663702 ) ) ;
#2823=CARTESIAN_POINT ( 'NONE',  ( 4.757797086070312709, 156.0326374431741385, 1.238355579604160095 ) ) ;
#2824=CARTESIAN_POINT ( 'NONE',  ( 15.19943428492308080, 148.1072807477730748, 0.3037208696559882681 ) ) ;
#2825=CARTESIAN_POINT ( 'NONE',  ( 16.86121613381884288, 155.2078297922403465, 0.3138802613840052658 ) ) ;
#2826=CARTESIAN_POINT ( 'NONE',  ( -5.235361408262325433, 116.2637919873444190, 0.9632728985350241802 ) ) ;
#2828=CARTESIAN_POINT ( 'NONE',  ( 3.758730197597703437, 121.0943292417197199, 0.07510837462871998438 ) ) ;
#2829=CARTESIAN_POINT ( 'NONE',  ( 12.77966252534833203, 121.3369795956499928, 1.646308105693409685 ) ) ;
#2830=CARTESIAN_POINT ( 'NONE',  ( 3.722543281321895936, 25.13347685689727484, 7.580879713197038683 ) ) ;
#2831=CARTESIAN_POINT ( 'NONE',  ( 2.211048372675892715, 116.8625674272878712, -0.4564130614398590469 ) ) ;
#2832=CARTESIAN_POINT ( 'NONE',  ( 0.01180776362021594868, 120.3637084677655764, -0.5909087754569243289 ) ) ;
#2835=CIRCLE ( 'NONE', #10996, 5.588000000000006295 ) ;
#2836=CARTESIAN_POINT ( 'NONE',  ( 3.211436584971100849, 28.15539441671475274, -3.345526564039049688 ) ) ;
#2839=CARTESIAN_POINT ( 'NONE',  ( 3.198224922426783579, -14.19254063666773291, 2.189163805996276579 ) ) ;
#2840=CARTESIAN_POINT ( 'NONE',  ( 1.052442600544414963, 124.5996987749017109, -0.008430925479885281390 ) ) ;
#2841=CARTESIAN_POINT ( 'NONE',  ( -1.382728874883544234, 159.5452856091935132, 0.4834108180186511006 ) ) ;
#2845=CARTESIAN_POINT ( 'NONE',  ( -3.682264917456323339, 72.48346620154573827, -0.07358041635423968885 ) ) ;
#2847=CARTESIAN_POINT ( 'NONE',  ( 2.079639979227050350, -15.65372482070806548, 5.795360105834356013 ) ) ;
#2848=CARTESIAN_POINT ( 'NONE',  ( -2.710741864450691097, 158.4754809254847601, 1.535472453293832640 ) ) ;
#2849=CARTESIAN_POINT ( 'NONE',  ( 20.76678851138485271, 151.0745573368290593, -1.154740394482948185 ) ) ;
#2850=CARTESIAN_POINT ( 'NONE',  ( -1.861891798414337940, 1.167894131763866250, -4.247245584637167504 ) ) ;
#2854=CARTESIAN_POINT ( 'NONE',  ( 0.3606724330767769882, 121.2597428844643161, 0.4428036157107449466 ) ) ;
#2856=CARTESIAN_POINT ( 'NONE',  ( -16.92314199871296054, 144.1809451582817587, 1.383154804529856952 ) ) ;
#2858=CARTESIAN_POINT ( 'NONE',  ( 5.904616261062731297, 156.9788419092994047, -1.696979819435221248 ) ) ;
#2859=AXIS2_PLACEMENT_3D ( 'NONE', #24574, #40999, #27779 ) ;
#2860=CARTESIAN_POINT ( 'NONE',  ( -16.44465323483264640, 153.5550899668227203, -2.240181424793372678 ) ) ;
#2863=CARTESIAN_POINT ( 'NONE',  ( 14.80764902091315349, 139.2804412874323248, -0.6846718672572658093 ) ) ;
#2865=CARTESIAN_POINT ( 'NONE',  ( -13.78152227852080181, 152.5163154464351294, -2.142015651154440370 ) ) ;
#2866=CARTESIAN_POINT ( 'NONE',  ( 3.466386268343554899, -14.94433061298855492, 0.9111787176236659791 ) ) ;
#2868=CARTESIAN_POINT ( 'NONE',  ( -4.065972646788793554, 118.2429491485453070, -0.3080848862740693250 ) ) ;
#2870=CARTESIAN_POINT ( 'NONE',  ( -4.773199170040517636, 117.7614384816488240, 0.8821210834465519346 ) ) ;
#2871=CARTESIAN_POINT ( 'NONE',  ( 17.42038752474475416, 148.2779598588913643, 2.227836471057101697 ) ) ;
#2873=CARTESIAN_POINT ( 'NONE',  ( 0.9564925537785137211, 29.00497265395555857, -4.523030980006896407 ) ) ;
#2874=CARTESIAN_POINT ( 'NONE',  ( 9.229262982541557747, 124.0999252189730697, 0.4162339757116151340 ) ) ;
#2877=ORIENTED_EDGE ( 'NONE', *, *, #41566, .T. ) ;
#2881=CARTESIAN_POINT ( 'NONE',  ( -8.682987951664228987, 118.1671358045530695, -0.9199987475528748071 ) ) ;
#2884=CARTESIAN_POINT ( 'NONE',  ( -15.38960455597353416, 120.6961994932685798, -0.07768288530491206101 ) ) ;
#2887=CARTESIAN_POINT ( 'NONE',  ( 7.812860049219216840, 122.5196119963270291, -0.1414684944325806104 ) ) ;
#2891=CARTESIAN_POINT ( 'NONE',  ( 2.044657339584382783, 115.7029490950255592, -1.636397532061663496 ) ) ;
#2892=CARTESIAN_POINT ( 'NONE',  ( 0.002459394112954048622, 156.3065584682211124, -0.1230781383047672012 ) ) ;
#2893=CARTESIAN_POINT ( 'NONE',  ( 2.287996554222524903, -15.35138490607948469, 5.941601703801219436 ) ) ;
#2894=CARTESIAN_POINT ( 'NONE',  ( -21.42146139051196130, 149.1985357531029308, 1.383244442692061371 ) ) ;
#2897=CARTESIAN_POINT ( 'NONE',  ( 23.31615218609850615, 149.0517038676186417, 0.6965919665178230691 ) ) ;
#2898=CARTESIAN_POINT ( 'NONE',  ( 7.041682102342773142, 122.0731594768587343, 0.2571765663980097871 ) ) ;
#2900=CARTESIAN_POINT ( 'NONE',  ( -0.5883093083485460006, 14.76436220226899465, 0.7776626239079347247 ) ) ;
#2901=CARTESIAN_POINT ( 'NONE',  ( -3.735388766125086857, 116.6566025657135413, -0.1875874814615930974 ) ) ;
#2904=CARTESIAN_POINT ( 'NONE',  ( 2.508634252739555759, 116.7753849408351243, 0.5210829680955889609 ) ) ;
#2907=CARTESIAN_POINT ( 'NONE',  ( -0.009931510163752330436, 117.7854482299006378, 0.4970133802592049954 ) ) ;
#2908=CARTESIAN_POINT ( 'NONE',  ( 11.07050914993712709, 156.0189320485970086, -1.715486126203028316 ) ) ;
#2909=CARTESIAN_POINT ( 'NONE',  ( 5.057590804293729647, 14.82039226405042243, -6.742867120243351664 ) ) ;
#2910=CARTESIAN_POINT ( 'NONE',  ( -20.86915823776865153, 136.4823663107028722, -1.950121757083878027 ) ) ;
#2911=CARTESIAN_POINT ( 'NONE',  ( 4.732332605385225044, 117.8971787801968674, -0.7794400467109126041 ) ) ;
#2914=AXIS2_PLACEMENT_3D ( 'NONE', #14992, #15203, #41001 ) ;
#2915=CARTESIAN_POINT ( 'NONE',  ( -9.188648150231783163, 124.1858035287836231, -0.09819667026458960002 ) ) ;
#2916=CARTESIAN_POINT ( 'NONE',  ( -15.10275521329014126, 128.5586215118215705, -2.151272397954998805 ) ) ;
#2917=CARTESIAN_POINT ( 'NONE',  ( 2.745816630209086728, -15.73397280162352985, 5.435574744647863277 ) ) ;
#2921=CARTESIAN_POINT ( 'NONE',  ( 8.426631749355106393, 120.7201681212196291, 1.435507493075423913 ) ) ;
#2925=CARTESIAN_POINT ( 'NONE',  ( -3.788670433418693140, 121.1194860566822626, 0.2213384591549591440 ) ) ;
#2926=CARTESIAN_POINT ( 'NONE',  ( 8.184481992144968743, -14.99546276350015717, -2.142971516962156819 ) ) ;
#2927=CARTESIAN_POINT ( 'NONE',  ( 9.518183030555334767, 123.9284174147966269, 0.7933090623874852199 ) ) ;
#2928=CARTESIAN_POINT ( 'NONE',  ( 0.006370369177266787912, 117.0014201992989058, -0.3187993231787207837 ) ) ;
#2933=CARTESIAN_POINT ( 'NONE',  ( -23.34374616560295834, 149.0672090665632936, -0.4407082534803007379 ) ) ;
#2935=CARTESIAN_POINT ( 'NONE',  ( -6.287620022660915353, 119.9368201151051494, -1.217206256648388996 ) ) ;
#2936=DIRECTION ( 'NONE',  ( -0.9998004120163608288, 0.000000000000000000, -0.01997839162482749342 ) ) ;
#2937=CARTESIAN_POINT ( 'NONE',  ( -2.749413646642218101, 120.8469057251343060, -0.2833394764088548734 ) ) ;
#2939=CARTESIAN_POINT ( 'NONE',  ( 1.421603664355671315, 159.6054662015457666, 0.02840702444251847966 ) ) ;
#2941=CARTESIAN_POINT ( 'NONE',  ( 4.076717266748975277, 8.489475128091552136, -2.202413229635628689 ) ) ;
#2943=CARTESIAN_POINT ( 'NONE',  ( -4.977065986284164190, 117.4065423621357382, 0.8841140845778143742 ) ) ;
#2945=CARTESIAN_POINT ( 'NONE',  ( 3.174366308151881810, 71.97546620154574271, 0.06343139340882768262 ) ) ;
#2946=CARTESIAN_POINT ( 'NONE',  ( 5.993962039581884227, 120.5133896973282361, 0.9940668381815480625 ) ) ;
#2947=CARTESIAN_POINT ( 'NONE',  ( -3.469956624915944587, 9.623539240006554252, 3.074419811715999984 ) ) ;
#2948=CARTESIAN_POINT ( 'NONE',  ( 22.54389841724620425, 148.7221180073953235, 1.757920738659724869 ) ) ;
#2950=CARTESIAN_POINT ( 'NONE',  ( 0.9116540650998883333, 106.1659180060823644, 5.214520442167681402 ) ) ;
#2951=CARTESIAN_POINT ( 'NONE',  ( 0.4229338353207374723, 117.8786474493541050, -0.5307671053780917969 ) ) ;
#2953=CARTESIAN_POINT ( 'NONE',  ( 2.551181839206869917, 14.82117702134586779, -3.857898856385788999 ) ) ;
#2954=CARTESIAN_POINT ( 'NONE',  ( -21.51154278844960999, 151.3526640061693342, -1.384567357891492989 ) ) ;
#2957=CARTESIAN_POINT ( 'NONE',  ( -1.653377498379716481, 156.2910218135955631, 0.4236837486942557351 ) ) ;
#2958=CARTESIAN_POINT ( 'NONE',  ( 3.016199308703121140, -15.16462411293013979, 5.702656747445028707 ) ) ;
#2959=DIRECTION ( 'NONE',  ( 0.9998004120163609398, 4.016384292689130894E-17, 0.01997839162482749689 ) ) ;
#2961=CARTESIAN_POINT ( 'NONE',  ( -4.641563771631805224, 117.9844563754833899, -0.8830158030444785755 ) ) ;
#2963=CARTESIAN_POINT ( 'NONE',  ( 3.758730197597703437, 121.0943292417197199, 0.07510837462872009540 ) ) ;
#2965=CARTESIAN_POINT ( 'NONE',  ( 19.41896158923237081, 149.6234262069624492, 2.479904253118717428 ) ) ;
#2967=CARTESIAN_POINT ( 'NONE',  ( 8.981069108608807028, 123.9698733229553937, 0.1794631345465902139 ) ) ;
#2968=CARTESIAN_POINT ( 'NONE',  ( -8.125192968412418892, 117.9016134627522945, 0.4934282302770854334 ) ) ;
#2969=CARTESIAN_POINT ( 'NONE',  ( 4.889703507614793665, 117.4101837603834468, -0.9754936775373431734 ) ) ;
#2970=CARTESIAN_POINT ( 'NONE',  ( 5.835061174465369760, 117.1115750087645608, -0.2489150398414469723 ) ) ;
#2971=EDGE_CURVE ( 'NONE', #11359, #20793, #32764, .T. ) ;
#2973=CIRCLE ( 'NONE', #4357, 5.080000000000006288 ) ;
#2976=CARTESIAN_POINT ( 'NONE',  ( -4.937650010152420776, 117.4076175032476499, -1.082176492592219041 ) ) ;
#2979=CIRCLE ( 'NONE', #36979, 3.683000000000001162 ) ;
#2980=CARTESIAN_POINT ( 'NONE',  ( -4.687306205058505704, 118.0075146718663461, 0.5901339194766732632 ) ) ;
#2984=ADVANCED_FACE ( 'NONE', ( #28204 ), #15672, .T. ) ;
#2985=CARTESIAN_POINT ( 'NONE',  ( -3.396746297042179563, 118.5725545226142401, -0.9267210084873370723 ) ) ;
#2986=CARTESIAN_POINT ( 'NONE',  ( -5.908534618824000439, 118.9825038774357466, -0.5858829404670614638 ) ) ;
#2987=CARTESIAN_POINT ( 'NONE',  ( 4.734060133346893906, 117.8958279061648255, 0.9307166829614513803 ) ) ;
#2988=CARTESIAN_POINT ( 'NONE',  ( 3.221735024265227398, -14.36526069886394730, 2.718910799868354378 ) ) ;
#2989=CARTESIAN_POINT ( 'NONE',  ( -16.46997841215784675, 146.2355833862463328, -1.608729380348347560 ) ) ;
#2991=CARTESIAN_POINT ( 'NONE',  ( -3.489676481241766659, 115.7029491485453434, -1.632600653323997175 ) ) ;
#2992=EDGE_CURVE ( 'NONE', #24363, #30281, #34138, .T. ) ;
#2993=CARTESIAN_POINT ( 'NONE',  ( -4.660682439260153131, 113.7930424115631070, 2.024998540755147403 ) ) ;
#2995=CARTESIAN_POINT ( 'NONE',  ( 7.093755517943316491, 122.4291926079955317, 0.03209900709771758981 ) ) ;
#2996=CARTESIAN_POINT ( 'NONE',  ( 0.02615319344467511437, 156.8698190429800832, -1.308812744920978322 ) ) ;
#2998=CARTESIAN_POINT ( 'NONE',  ( -6.446885413170102552, 29.42808026494702389, 0.2842954123359194840 ) ) ;
#2999=CARTESIAN_POINT ( 'NONE',  ( -3.151729977245023573, 115.7029491485453860, 1.538670711546385572 ) ) ;
#3000=CARTESIAN_POINT ( 'NONE',  ( 4.224370802630715183, -2.505441902618962935, 1.893578447770203566 ) ) ;
#3001=CARTESIAN_POINT ( 'NONE',  ( 5.618954885708931535, 159.1014311945586712, 0.6070295849213357409 ) ) ;
#3005=CARTESIAN_POINT ( 'NONE',  ( 3.466386268343554899, -14.94433061298855492, 0.9111787176236659791 ) ) ;
#3006=CARTESIAN_POINT ( 'NONE',  ( -8.713776656587379321, 120.2102557752085232, 1.142027078586575595 ) ) ;
#3007=CARTESIAN_POINT ( 'NONE',  ( 0.8997923272943838535, 13.09534505249760805, -0.3740510727227569499 ) ) ;
#3008=CARTESIAN_POINT ( 'NONE',  ( -0.006055453635351584415, 1.369653838947524349, -0.9756124606672940125 ) ) ;
#3010=EDGE_LOOP ( 'NONE', ( #40516, #27985, #744, #41049, #27638, #34437, #8513, #1972, #1418, #39890 ) ) ;
#3013=CARTESIAN_POINT ( 'NONE',  ( 3.014030426305779553, 115.9530684888725460, 1.587286815012126207 ) ) ;
#3015=CARTESIAN_POINT ( 'NONE',  ( -0.006077178772743973764, 120.4695998130595598, 0.3041268764237435862 ) ) ;
#3017=CARTESIAN_POINT ( 'NONE',  ( 2.668130780779813360, -14.68804970414791455, 5.313657848291281738 ) ) ;
#3018=CARTESIAN_POINT ( 'NONE',  ( 8.280704432558463779, 121.1361926620737393, -1.000371422393417475 ) ) ;
#3020=CARTESIAN_POINT ( 'NONE',  ( -14.77311812546558123, 125.6006210965460781, -2.040279103193882282 ) ) ;
#3022=CARTESIAN_POINT ( 'NONE',  ( 8.564519932783092315, 118.7250576737585845, 1.182609549202882082 ) ) ;
#3023=CARTESIAN_POINT ( 'NONE',  ( -5.530486672362699530, 32.07197567765449975, 2.641630925256825080 ) ) ;
#3024=CARTESIAN_POINT ( 'NONE',  ( 6.058098509843102164, 155.3491655920357459, -0.2313079102920780339 ) ) ;
#3025=ORIENTED_EDGE ( 'NONE', *, *, #12507, .F. ) ;
#3026=DIRECTION ( 'NONE',  ( 5.206863593109713661E-17, -1.000000000000000000, 1.077750396879097183E-30 ) ) ;
#3027=CARTESIAN_POINT ( 'NONE',  ( -6.615214180512292604E-14, 94.32746620154571815, -2.829521569843129660E-18 ) ) ;
#3028=AXIS2_PLACEMENT_3D ( 'NONE', #42158, #3174, #32994 ) ;
#3031=CARTESIAN_POINT ( 'NONE',  ( 9.757351933493456642, 123.8372022493589100, 0.9812814142356128810 ) ) ;
#3033=CARTESIAN_POINT ( 'NONE',  ( 1.806356699219098250, 116.4728921782852922, -0.003255218499346594716 ) ) ;
#3034=CARTESIAN_POINT ( 'NONE',  ( -4.488494058616981697, 111.2667756541687538, 2.954587190001159325 ) ) ;
#3035=CARTESIAN_POINT ( 'NONE',  ( -4.375468101073169969, 118.7629491485454309, 0.8819984256705631909 ) ) ;
#3037=CARTESIAN_POINT ( 'NONE',  ( -0.5257358919991518276, 34.34849739310375583, 0.2665863176793757394 ) ) ;
#3038=CARTESIAN_POINT ( 'NONE',  ( 20.83122434882616858, 148.6614476615901594, 2.397187407820276395 ) ) ;
#3039=CARTESIAN_POINT ( 'NONE',  ( -3.632229383214316876, 17.08265688572556584, -2.901706292871565562 ) ) ;
#3040=CARTESIAN_POINT ( 'NONE',  ( 7.100331465950064036, 27.70181474634058461, -4.559502152892632942 ) ) ;
#3041=CARTESIAN_POINT ( 'NONE',  ( 2.181699532838504929, 116.7361444524075864, -0.4061292330571752984 ) ) ;
#3042=CARTESIAN_POINT ( 'NONE',  ( -0.2537530607705146823, 113.0327356262573915, -2.627782494400415558 ) ) ;
#3044=CARTESIAN_POINT ( 'NONE',  ( 2.874628747758903646, 107.8418180396803336, -4.365346587048165361 ) ) ;
#3045=CARTESIAN_POINT ( 'NONE',  ( 2.609247996698298877, 104.6144662015478843, 4.655519476068421980 ) ) ;
#3046=CARTESIAN_POINT ( 'NONE',  ( 3.874746376330849618, 18.20996518813934628, -2.522041008920607563 ) ) ;
#3049=CARTESIAN_POINT ( 'NONE',  ( 3.131015516031846690, -14.62848841321586946, 3.524024012273756501 ) ) ;
#3050=CARTESIAN_POINT ( 'NONE',  ( 2.504607545376390298, 120.2382744777187611, -0.4047138806074997985 ) ) ;
#3051=CARTESIAN_POINT ( 'NONE',  ( -14.93494801707998576, 120.8072429308574414, 0.3831319127562622384 ) ) ;
#3055=EDGE_LOOP ( 'NONE', ( #23597, #21939, #2058, #29396 ) ) ;
#3057=CARTESIAN_POINT ( 'NONE',  ( 5.007622726684139991, -15.39085649315211057, 3.402342850907996041 ) ) ;
#3058=CARTESIAN_POINT ( 'NONE',  ( -13.10063739191627086, 155.4510764517707742, 1.634185922311342631 ) ) ;
#3059=CARTESIAN_POINT ( 'NONE',  ( 17.11036550247942145, 125.2153959547233910, -0.9255656842583630528 ) ) ;
#3060=CARTESIAN_POINT ( 'NONE',  ( 2.229080734463354307, 9.364070591990056869, -4.050418370856919914 ) ) ;
#3064=CARTESIAN_POINT ( 'NONE',  ( -0.01111760956581894950, 120.5507043431653784, 0.5563706444132522355 ) ) ;
#3065=( NAMED_UNIT ( * ) PLANE_ANGLE_UNIT ( ) SI_UNIT ( $, .RADIAN. ) );
#3066=CARTESIAN_POINT ( 'NONE',  ( -16.40043613793208621, 149.3997711511537148, 1.468335723160356654 ) ) ;
#3068=CARTESIAN_POINT ( 'NONE',  ( 10.22873863908706404, 155.5514087735115822, -1.732306429912916723 ) ) ;
#3069=CARTESIAN_POINT ( 'NONE',  ( -2.740693480742399490, 158.6924860557018064, -1.553331106148862384 ) ) ;
#3072=CARTESIAN_POINT ( 'NONE',  ( 4.599907942160887053, 118.0774652753429450, -0.5280204677610548236 ) ) ;
#3073=CARTESIAN_POINT ( 'NONE',  ( 11.75634259954068739, 128.3321206738457647, -0.5010001888332089592 ) ) ;
#3075=CARTESIAN_POINT ( 'NONE',  ( -15.43964774321195144, 150.7699688800196611, -2.159935508548367356 ) ) ;
#3076=CARTESIAN_POINT ( 'NONE',  ( 3.246941722412215459, -15.25025356868572857, 3.602141857564104210 ) ) ;
#3077=DIRECTION ( 'NONE',  ( 0.9998004120163609398, 0.000000000000000000, 0.01997839162482749689 ) ) ;
#3078=CARTESIAN_POINT ( 'NONE',  ( -4.801647862234980302, 117.4032733357427105, 1.015449305853463491 ) ) ;
#3079=CARTESIAN_POINT ( 'NONE',  ( -4.797757306094807994, 117.7649951200880025, 0.8642570761844743377 ) ) ;
#3080=CARTESIAN_POINT ( 'NONE',  ( 1.975234429548441195, 156.8313070664539168, 1.415192030232629072 ) ) ;
#3081=CARTESIAN_POINT ( 'NONE',  ( 0.1949087904810299920, 33.82644263972942156, 0.4054292462034601585 ) ) ;
#3082=CARTESIAN_POINT ( 'NONE',  ( 8.369577038434204752, -11.69170392490758381, 0.7719616968112763544 ) ) ;
#3083=CARTESIAN_POINT ( 'NONE',  ( 15.29340151118736735, 148.0176312819745874, 0.6334265850898870287 ) ) ;
#3087=CARTESIAN_POINT ( 'NONE',  ( -0.4175747659228876696, 118.1588898423965048, 0.8928943804540209195 ) ) ;
#3091=CARTESIAN_POINT ( 'NONE',  ( 2.081416901521091933, -15.50639809317535089, 5.943648939154567934 ) ) ;
#3094=CARTESIAN_POINT ( 'NONE',  ( -3.754954749907463807, 116.6824454826851820, 0.08209545411912770596 ) ) ;
#3095=EDGE_LOOP ( 'NONE', ( #4542, #38939, #15926, #25195 ) ) ;
#3097=CARTESIAN_POINT ( 'NONE',  ( -7.817668890232951640, 122.4248663112730782, -0.5901703440876553408 ) ) ;
#3099=CARTESIAN_POINT ( 'NONE',  ( 2.338193611591690146, 115.7028059236074142, -1.613667146768946958 ) ) ;
#3100=CARTESIAN_POINT ( 'NONE',  ( -1.603837441938277930, 120.9755568995931156, -0.09629321774905863496 ) ) ;
#3101=CARTESIAN_POINT ( 'NONE',  ( 5.673832624563095450, -13.47712647082498272, 2.605829897212420754 ) ) ;
#3102=CARTESIAN_POINT ( 'NONE',  ( -0.009513433763575551705, 117.6614778598761291, 0.4760911276077181564 ) ) ;
#3104=CARTESIAN_POINT ( 'NONE',  ( 22.79149376799268722, 150.3987591554885626, 0.7843734907460314654 ) ) ;
#3105=CARTESIAN_POINT ( 'NONE',  ( 15.78018659616589581, 146.2345701426180824, 0.4496550483759581551 ) ) ;
#3107=CARTESIAN_POINT ( 'NONE',  ( -0.2244654480080381653, 11.31155722793083918, -0.9512810396025579429 ) ) ;
#3108=CARTESIAN_POINT ( 'NONE',  ( -16.10347893962658361, 121.2391669109744186, -0.4275719782727095408 ) ) ;
#3112=CARTESIAN_POINT ( 'NONE',  ( 5.533182690628008160, 117.2225855060814013, 0.7735903190986758160 ) ) ;
#3115=CARTESIAN_POINT ( 'NONE',  ( 21.10167996235824717, 141.7209635633906259, 2.240609589767335486 ) ) ;
#3116=CARTESIAN_POINT ( 'NONE',  ( 6.464497043865751635, 157.5392376370035095, -1.685792624679405494 ) ) ;
#3117=CARTESIAN_POINT ( 'NONE',  ( -8.002357889267953439, 8.121853428443936096, -2.619265908643666929 ) ) ;
#3118=CARTESIAN_POINT ( 'NONE',  ( -13.94627971010885403, 121.2764344996515717, -1.482775695869144483 ) ) ;
#3119=CARTESIAN_POINT ( 'NONE',  ( 4.735283304133474758, 117.8439692571760986, -0.8354117580122082387 ) ) ;
#3120=CARTESIAN_POINT ( 'NONE',  ( 0.6715300310779280801, 105.9424719104300436, 5.313162126831953103 ) ) ;
#3121=CARTESIAN_POINT ( 'NONE',  ( -1.612929917264666502, 120.9971453638330985, -0.006532979378300230941 ) ) ;
#3122=CARTESIAN_POINT ( 'NONE',  ( -14.67610382776227418, 152.8628051715174365, -2.323547792494559339 ) ) ;
#3123=CARTESIAN_POINT ( 'NONE',  ( 3.255875469058810978, -15.74984210207193414, 5.086368125509904026 ) ) ;
#3127=B_SPLINE_SURFACE_WITH_KNOTS ( 'NONE', 1, 3, ( 
 ( #10981, #39979, #23751, #36982, #4413, #7380, #29950, #36772, #20764, #13764, #36366, #4616, #17777, #17572, #14371, #27381, #10565, #33995 ),
 ( #40391, #30774, #13558, #26547, #10357, #23329, #20141, #33163, #14789, #25234, #21377, #34403, #12025, #17987, #41437, #21174, #27585, #11815 ) ),
 .UNSPECIFIED., .F., .F., .F.,
 ( 2, 2 ),
 ( 4, 2, 2, 2, 2, 2, 2, 2, 4 ),
 ( 0.000000000000000000, 1.000000000000000000 ),
 ( 0.000000000000000000, 0.06250000000000000000, 0.1250000000000000000, 0.1875000000000000000, 0.2500000000000000000, 0.3750000000000000000, 0.5000000000000000000, 0.7500000000000000000, 1.000000000000000000 ),
 .UNSPECIFIED. ) ;
#3128=CARTESIAN_POINT ( 'NONE',  ( -0.01051219832189233434, 119.4384375980492194, 0.5260733902271049756 ) ) ;
#3131=CARTESIAN_POINT ( 'NONE',  ( -1.980194564007182745, 113.2583846565721757, 2.436415359710689010 ) ) ;
#3132=CARTESIAN_POINT ( 'NONE',  ( 1.359589829139859152, 24.67768052395325284, 8.332721669750835503 ) ) ;
#3133=CARTESIAN_POINT ( 'NONE',  ( 12.10601879509723844, 151.9817061558079274, 1.041216838735509409 ) ) ;
#3134=AXIS2_PLACEMENT_3D ( 'NONE', #33597, #36580, #389 ) ;
#3135=CARTESIAN_POINT ( 'NONE',  ( 22.21083362159523134, 150.4821223471089411, -0.6270836034604136966 ) ) ;
#3136=DIRECTION ( 'NONE',  ( 0.9998004120163608288, 0.000000000000000000, 0.01997839162482762526 ) ) ;
#3138=CARTESIAN_POINT ( 'NONE',  ( -4.717508175643587265, 116.7562497393984415, -0.08034061319516418165 ) ) ;
#3139=VERTEX_POINT ( 'NONE', #18883 ) ;
#3140=CARTESIAN_POINT ( 'NONE',  ( -6.546631412653550086, 120.5239780760649211, -1.124119359349389002 ) ) ;
#3141=CARTESIAN_POINT ( 'NONE',  ( 23.21373371908085304, 149.6306211361744829, 0.4638656453230914356 ) ) ;
#3142=CARTESIAN_POINT ( 'NONE',  ( -15.56637720654312851, 147.8873989650969918, -1.033077377765619698 ) ) ;
#3143=CARTESIAN_POINT ( 'NONE',  ( 4.031918519141627577, -13.48391852982397410, 3.589295450856327729 ) ) ;
#3145=CARTESIAN_POINT ( 'NONE',  ( 18.84770637050841202, 125.3331924886369961, 0.3953412214710180783 ) ) ;
#3147=CARTESIAN_POINT ( 'NONE',  ( 4.627880361116947228, 7.839802885307131319, -0.3238752845059330032 ) ) ;
#3148=CARTESIAN_POINT ( 'NONE',  ( -3.703049682113393359, 116.6240124373522065, -0.07399574541707862330 ) ) ;
#3149=CARTESIAN_POINT ( 'NONE',  ( -4.902142009400407119, 117.4083702128866804, 0.9678786404911806640 ) ) ;
#3151=CARTESIAN_POINT ( 'NONE',  ( -4.506407954616146405, 27.87871297014265792, 0.5132454074226986407 ) ) ;
#3152=CARTESIAN_POINT ( 'NONE',  ( -6.073003016519146868, 120.6640402819336515, 0.7109903207712315876 ) ) ;
#3153=CARTESIAN_POINT ( 'NONE',  ( -1.220754042303205500, 16.12054255322086860, -4.471266627502475721 ) ) ;
#3154=CARTESIAN_POINT ( 'NONE',  ( -0.006942562093360102847, 117.0978366787122127, 0.3474341964894884782 ) ) ;
#3155=CARTESIAN_POINT ( 'NONE',  ( 15.76285804746337504, 145.9067145067647289, 0.3149794173055761592 ) ) ;
#3157=CARTESIAN_POINT ( 'NONE',  ( 13.77700084449465301, 121.8522644830672590, -1.120765626652496127 ) ) ;
#3158=CARTESIAN_POINT ( 'NONE',  ( -2.426139246716550346, 10.07336736126799437, 3.943011612146583023 ) ) ;
#3159=CARTESIAN_POINT ( 'NONE',  ( 0.01289612358321986542, 159.5048567107479585, -0.6453747585945881493 ) ) ;
#3163=CARTESIAN_POINT ( 'NONE',  ( -0.6274479277951703349, 120.8480686026657196, 0.1451731132019953019 ) ) ;
#3165=CARTESIAN_POINT ( 'NONE',  ( 4.021138818454151220, -15.00176662281678475, 5.141887924562631440 ) ) ;
#3168=CARTESIAN_POINT ( 'NONE',  ( 4.110343450561533274, 118.7489093234570561, 1.002437571585374831 ) ) ;
#3170=DIRECTION ( 'NONE',  ( -0.9998004120163608288, 0.000000000000000000, -0.01997839162482749342 ) ) ;
#3171=CARTESIAN_POINT ( 'NONE',  ( -20.14555658732733079, 152.4688535085772685, 0.7444337660854593031 ) ) ;
#3172=CARTESIAN_POINT ( 'NONE',  ( 4.825435570034072086, 117.4745258938095134, -0.9995196418742542388 ) ) ;
#3173=CARTESIAN_POINT ( 'NONE',  ( 1.399407963385772113, 159.5796833544862352, -0.3162364300534755701 ) ) ;
#3174=DIRECTION ( 'NONE',  ( 4.017660918040594346E-17, -1.000000000000000000, -2.376309959284834438E-19 ) ) ;
#3177=CARTESIAN_POINT ( 'NONE',  ( 1.898988921116985251, -15.25340086675062956, 5.381265105722330411 ) ) ;
#3180=FACE_OUTER_BOUND ( 'NONE', #20121, .T. ) ;
#3182=CARTESIAN_POINT ( 'NONE',  ( -4.601728189754446419, 118.0704954893843990, 0.5721313084656637349 ) ) ;
#3187=CARTESIAN_POINT ( 'NONE',  ( -5.887631883382205444, 119.0670759175282001, -1.260654324767885859 ) ) ;
#3188=CARTESIAN_POINT ( 'NONE',  ( -3.394470486402190623, 108.6891572770382624, -4.119616105806037432 ) ) ;
#3189=CARTESIAN_POINT ( 'NONE',  ( 4.764019565006264223, 117.8854380970585680, 0.8884589727399109238 ) ) ;
#3190=CARTESIAN_POINT ( 'NONE',  ( 2.664052010559913253, -13.52006206191685322, 0.08958796903007473778 ) ) ;
#3191=CARTESIAN_POINT ( 'NONE',  ( -16.40115699206388555, 147.1833543704171348, -1.602497317185074710 ) ) ;
#3192=CARTESIAN_POINT ( 'NONE',  ( -2.812965544484426594, 115.7033311652958787, -1.680242139021033143 ) ) ;
#3195=CARTESIAN_POINT ( 'NONE',  ( 1.571019246621431664, 106.2535611835979239, -5.108158685570669988 ) ) ;
#3196=CARTESIAN_POINT ( 'NONE',  ( -11.12341512264673682, 124.6236798342360856, -1.410428355923976529 ) ) ;
#3199=CARTESIAN_POINT ( 'NONE',  ( -0.02615319344480911481, 156.8698190429800832, 1.308812744920978322 ) ) ;
#3200=CARTESIAN_POINT ( 'NONE',  ( -3.795109032377635749, 115.7029491485453576, 1.459792008210426539 ) ) ;
#3201=CARTESIAN_POINT ( 'NONE',  ( 2.522041008973656240, -3.380034811851382770, 3.874746376371965173 ) ) ;
#3202=CARTESIAN_POINT ( 'NONE',  ( 3.210256534570805620, 159.4348965051207756, 0.5208765431038288041 ) ) ;
#3203=VERTEX_POINT ( 'NONE', #28483 ) ;
#3205=CARTESIAN_POINT ( 'NONE',  ( 3.752486096903807855, -15.17702595220350759, -0.4382564666907802220 ) ) ;
#3206=CARTESIAN_POINT ( 'NONE',  ( -18.05326814683172287, 150.0321773811041339, 1.740468527814021282 ) ) ;
#3207=CARTESIAN_POINT ( 'NONE',  ( -0.6470182227010313758, 8.987660258844066163, 0.7316552229444387434 ) ) ;
#3208=CIRCLE ( 'NONE', #11338, 3.175000000000001155 ) ;
#3209=CARTESIAN_POINT ( 'NONE',  ( -1.853717367163283836, 116.5907236856068181, -0.2192087907590278273 ) ) ;
#3210=AXIS2_PLACEMENT_3D ( 'NONE', #15167, #11982, #24976 ) ;
#3211=CARTESIAN_POINT ( 'NONE',  ( 0.9752960398044887569, 8.493769703755262412, 0.04006526980912952091 ) ) ;
#3212=ORIENTED_EDGE ( 'NONE', *, *, #4040, .T. ) ;
#3215=CARTESIAN_POINT ( 'NONE',  ( 4.076169972524736451, 117.8719421043398370, 0.8561738758874235522 ) ) ;
#3217=CARTESIAN_POINT ( 'NONE',  ( -2.684237737021801795, 120.5579296053302727, 0.3360084551914350182 ) ) ;
#3218=CARTESIAN_POINT ( 'NONE',  ( 1.975269416564901404, -15.10067923695700109, 5.832845082603779652 ) ) ;
#3219=CARTESIAN_POINT ( 'NONE',  ( 5.414978495245504675, 156.5090806470891209, -1.537019876316039868 ) ) ;
#3221=CARTESIAN_POINT ( 'NONE',  ( -17.65052098649054813, 151.6044147853587845, -2.418251502674879205 ) ) ;
#3223=CARTESIAN_POINT ( 'NONE',  ( 2.233078627056604759, -15.14192004606506536, 5.083345892419886880 ) ) ;
#3224=CARTESIAN_POINT ( 'NONE',  ( -1.804899523998967803, 35.85624791583304471, 1.055339088927661262 ) ) ;
#3226=CARTESIAN_POINT ( 'NONE',  ( 9.203139800278290039, 153.8854248570426080, -0.2095608753156673887 ) ) ;
#3230=EDGE_CURVE ( 'NONE', #25709, #9800, #4902, .T. ) ;
#3235=CARTESIAN_POINT ( 'NONE',  ( 1.419391870195661376, 159.6052071245950970, -0.01540741456718461473 ) ) ;
#3236=CARTESIAN_POINT ( 'NONE',  ( -7.328771362700684300, 123.0350022594044219, -0.07777345538050987883 ) ) ;
#3238=CARTESIAN_POINT ( 'NONE',  ( -6.733080298864849599E-14, 123.6644662015457214, 4.141858957710797243E-18 ) ) ;
#3240=CARTESIAN_POINT ( 'NONE',  ( 0.8256988760359594837, 37.88232708988313391, -1.149614905092997796 ) ) ;
#3241=CARTESIAN_POINT ( 'NONE',  ( 14.79112219052226784, 123.2524255416106342, 1.763561952744266081 ) ) ;
#3242=CARTESIAN_POINT ( 'NONE',  ( -0.2501726036287156840, 25.39126883368370002, -4.616104092076634302 ) ) ;
#3243=CARTESIAN_POINT ( 'NONE',  ( -3.184215270518052421, -12.39116543543024562, -7.798991864805400631 ) ) ;
#3244=CARTESIAN_POINT ( 'NONE',  ( -8.715807593838684753, 118.0255461215873254, -0.7900476978637416270 ) ) ;
#3245=CARTESIAN_POINT ( 'NONE',  ( -0.7524737301091138919, 120.0979018405971175, -0.6085003676253138982 ) ) ;
#3247=CARTESIAN_POINT ( 'NONE',  ( 0.2371669961381878411, 105.9788885827711340, -5.291421317388997458 ) ) ;
#3248=CARTESIAN_POINT ( 'NONE',  ( 2.608302318560305366, 105.1243950483077185, 4.653828818123431077 ) ) ;
#3249=CARTESIAN_POINT ( 'NONE',  ( 0.6590154617207463206, 19.50938314818779062, -4.574821423538240950 ) ) ;
#3252=CARTESIAN_POINT ( 'NONE',  ( 3.216637634036228821, -14.25892527173770752, 2.941440830758975888 ) ) ;
#3253=CARTESIAN_POINT ( 'NONE',  ( 3.292372560053815178, 124.4927030837263118, 0.04348745598417508296 ) ) ;
#3254=CARTESIAN_POINT ( 'NONE',  ( -22.15286039372332993, 136.9573810088325843, 0.3857095667871865974 ) ) ;
#3256=ORIENTED_EDGE ( 'NONE', *, *, #25445, .F. ) ;
#3260=CARTESIAN_POINT ( 'NONE',  ( 2.577823224604873786, -15.72362945599133077, 5.534267358606157039 ) ) ;
#3261=CARTESIAN_POINT ( 'NONE',  ( -14.47132921234248748, 123.3930721568691382, 1.260850717050816083 ) ) ;
#3262=CARTESIAN_POINT ( 'NONE',  ( 15.81089186882080710, 155.0373533369262589, -1.166412807380551309 ) ) ;
#3263=CARTESIAN_POINT ( 'NONE',  ( 4.076717266748975277, 8.489475128091552136, -2.202413229635628689 ) ) ;
#3268=CARTESIAN_POINT ( 'NONE',  ( -0.003073426023290456131, 123.4679809879534247, 0.1538068059577046287 ) ) ;
#3270=CARTESIAN_POINT ( 'NONE',  ( -17.57956382101115622, 146.6691408387931688, 1.464727724346842397 ) ) ;
#3272=CARTESIAN_POINT ( 'NONE',  ( 12.30591244053531774, 123.0735437985678971, -1.316165607245708413 ) ) ;
#3273=CARTESIAN_POINT ( 'NONE',  ( -13.36424875645665900, 155.6061939908119882, -2.069718186823301664 ) ) ;
#3275=AXIS2_PLACEMENT_3D ( 'NONE', #6670, #19223, #39468 ) ;
#3277=CARTESIAN_POINT ( 'NONE',  ( 4.486692410979344459, 118.1299448241766186, -0.5327426128926098237 ) ) ;
#3278=CARTESIAN_POINT ( 'NONE',  ( 16.05525886874792718, 145.8417561620165372, -0.5351738620951715930 ) ) ;
#3280=CARTESIAN_POINT ( 'NONE',  ( -17.70445710129711259, 147.3864036964934598, -2.239206817186280229 ) ) ;
#3281=CARTESIAN_POINT ( 'NONE',  ( 3.462569250300066681, -15.15729918637651075, 2.757833548007345037 ) ) ;
#3282=CARTESIAN_POINT ( 'NONE',  ( 3.032540074886261205, 105.1244957488249980, -4.437742800387862729 ) ) ;
#3283=EDGE_CURVE ( 'NONE', #40944, #23764, #32088, .T. ) ;
#3285=CARTESIAN_POINT ( 'NONE',  ( -4.776051034590975242, 117.6653734182690556, 0.9389516368186912043 ) ) ;
#3286=CARTESIAN_POINT ( 'NONE',  ( 10.53370020345040103, 154.2769816202975051, 1.888232850154635045 ) ) ;
#3288=CARTESIAN_POINT ( 'NONE',  ( 8.408789229792210662, -11.58028725773715628, 0.1531400924992341317 ) ) ;
#3289=CARTESIAN_POINT ( 'NONE',  ( 15.80103543825234880, 146.2514283349100594, 0.5462135236119776138 ) ) ;
#3296=LINE ( 'NONE', #321, #32462 ) ;
#3302=CARTESIAN_POINT ( 'NONE',  ( -14.68764241912311519, 120.3119357913517291, 0.01896423869846143237 ) ) ;
#3305=CARTESIAN_POINT ( 'NONE',  ( -6.059742184461669900, 121.4333258338537291, -0.1238882853059191380 ) ) ;
#3307=CARTESIAN_POINT ( 'NONE',  ( -15.65552799280940022, 147.2250547476223801, -0.5422809309331373395 ) ) ;
#3308=CARTESIAN_POINT ( 'NONE',  ( 5.456921283009238621, -14.23391906346564717, 3.426434758229824240 ) ) ;
#3309=CARTESIAN_POINT ( 'NONE',  ( -12.17409717887521303, 120.5818589831333441, 1.028275848330292952 ) ) ;
#3311=CARTESIAN_POINT ( 'NONE',  ( 15.13553065988576307, 156.1345691653134509, 0.5893329488795889803 ) ) ;
#3312=CARTESIAN_POINT ( 'NONE',  ( 0.6398660015929856781, 156.3034662015459446, 0.08424640074850882343 ) ) ;
#3313=CARTESIAN_POINT ( 'NONE',  ( 4.831486089547707863, 118.5266822147775940, -0.7499602601522077361 ) ) ;
#3314=CARTESIAN_POINT ( 'NONE',  ( 0.05241920358452190065, 15.83596528477922405, 0.9742995972537078497 ) ) ;
#3315=CARTESIAN_POINT ( 'NONE',  ( -5.738526254234522561, 159.1207877133979309, -0.2162537097210230630 ) ) ;
#3316=DIRECTION ( 'NONE',  ( -0.9998004120163609398, 0.000000000000000000, -0.01997839162482749689 ) ) ;
#3319=CARTESIAN_POINT ( 'NONE',  ( 2.394807681685032552, 116.5915636595390623, 0.4284483426437976639 ) ) ;
#3322=CARTESIAN_POINT ( 'NONE',  ( 21.52870603658934812, 148.1022500232506616, 2.247031159961964342 ) ) ;
#3323=CARTESIAN_POINT ( 'NONE',  ( 12.49437611722087205, 122.1796674805547980, -1.295212323302052937 ) ) ;
#3324=CARTESIAN_POINT ( 'NONE',  ( -0.9744428630873758213, 7.697845052497760854, 0.001242513977635927719 ) ) ;
#3325=CARTESIAN_POINT ( 'NONE',  ( 6.022233187337456606, 12.22246943312702427, 5.887876567768997482 ) ) ;
#3327=CARTESIAN_POINT ( 'NONE',  ( -21.50396862640735307, 149.5883454796168621, -2.135274339423805401 ) ) ;
#3328=CARTESIAN_POINT ( 'NONE',  ( 4.703873350422621336, 117.8348676116459472, -0.8530165572518777495 ) ) ;
#3330=CARTESIAN_POINT ( 'NONE',  ( 3.544426656953406862, 120.3814187630814132, -0.4774784233729820193 ) ) ;
#3331=CARTESIAN_POINT ( 'NONE',  ( -0.0005023639978753125738, 120.9974662015457056, 0.02514034870427569318 ) ) ;
#3333=CARTESIAN_POINT ( 'NONE',  ( -4.079782966556147805, 157.3082466949932723, -1.825029598092313687 ) ) ;
#3335=CARTESIAN_POINT ( 'NONE',  ( 6.125566448072323311, -14.60357603047697594, -0.1915981853098273624 ) ) ;
#3336=CARTESIAN_POINT ( 'NONE',  ( 5.240472681551541889, 115.6909491485453145, 1.017784315483886814 ) ) ;
#3337=EDGE_CURVE ( 'NONE', #10933, #31748, #29980, .T. ) ;
#3340=CARTESIAN_POINT ( 'NONE',  ( 4.224706347173564858, 119.5670751559891585, 0.9504096833562339919 ) ) ;
#3345=CARTESIAN_POINT ( 'NONE',  ( -2.274554406286753316, 117.6064948828932444, 1.027890184761801384 ) ) ;
#3346=CARTESIAN_POINT ( 'NONE',  ( 6.528609751734300914, 25.78175851779908356, 5.377075232920663694 ) ) ;
#3347=CARTESIAN_POINT ( 'NONE',  ( 9.400309931224008153, 124.0858766813489780, 0.6109843400649571654 ) ) ;
#3348=CARTESIAN_POINT ( 'NONE',  ( 1.955870317219520871, 116.9162416783649689, -0.3393494064863859516 ) ) ;
#3350=FACE_OUTER_BOUND ( 'NONE', #5948, .T. ) ;
#3351=CARTESIAN_POINT ( 'NONE',  ( -11.73725613052212324, 118.7267541726749869, -0.2187512536375164351 ) ) ;
#3353=CARTESIAN_POINT ( 'NONE',  ( 8.152322075550674896, 120.9500479307340299, -1.022460547729552083 ) ) ;
#3355=CARTESIAN_POINT ( 'NONE',  ( -10.59645057104367716, 153.0636280899912549, -0.8695332296301786501 ) ) ;
#3356=CARTESIAN_POINT ( 'NONE',  ( 2.309263497243444263, -14.96449433386182193, 5.702862618531368888 ) ) ;
#3357=CARTESIAN_POINT ( 'NONE',  ( -5.148936812350190628, 116.8706406773187894, 0.04504664567876282694 ) ) ;
#3358=CARTESIAN_POINT ( 'NONE',  ( 17.29877781292318417, 122.7677429521249053, 0.3633837628929261210 ) ) ;
#3360=CARTESIAN_POINT ( 'NONE',  ( -2.406711483539481389, 4.503775517365914638, 3.979180414515509412 ) ) ;
#3361=CARTESIAN_POINT ( 'NONE',  ( -6.439947148575337965E-14, 116.4254662015457313, 1.493913655526859821E-16 ) ) ;
#3362=CARTESIAN_POINT ( 'NONE',  ( -4.902238121359880019, 117.4071601550653838, 0.9680467791073505968 ) ) ;
#3364=CARTESIAN_POINT ( 'NONE',  ( 7.898376164620551698, 121.9960575332709425, 0.9517411587677502283 ) ) ;
#3366=CARTESIAN_POINT ( 'NONE',  ( 1.368391094521330897, 11.37271669962338372, 4.434453701053673313 ) ) ;
#3367=CARTESIAN_POINT ( 'NONE',  ( 1.027358375535017521, 117.1967307433898640, 0.4586652788708822093 ) ) ;
#3371=CARTESIAN_POINT ( 'NONE',  ( 20.76034172958447499, 149.5879773183856685, -1.515053003442401458 ) ) ;
#3372=CARTESIAN_POINT ( 'NONE',  ( -3.833338661037195561, 9.423677021345861604, 2.587938769098377279 ) ) ;
#3373=CARTESIAN_POINT ( 'NONE',  ( -20.09973570640927676, 152.4688535085772685, -1.548630484586873024 ) ) ;
#3375=CARTESIAN_POINT ( 'NONE',  ( -15.33898570969108910, 143.5038931315047535, 0.1524207748662386730 ) ) ;
#3376=CARTESIAN_POINT ( 'NONE',  ( 5.208971126070756519, -14.02307540452116186, 3.677211492609324228 ) ) ;
#3378=CARTESIAN_POINT ( 'NONE',  ( 3.150244473240279675, -14.07033042043420146, 1.813758411523331393 ) ) ;
#3381=CARTESIAN_POINT ( 'NONE',  ( 4.285767465938623566, 157.6046910967438066, 1.850878756276731485 ) ) ;
#3384=CARTESIAN_POINT ( 'NONE',  ( -22.52700986351724310, 149.9757045183965261, 0.6247156920787648726 ) ) ;
#3386=CARTESIAN_POINT ( 'NONE',  ( 1.881116149107284752, 116.6503132507590124, -0.1904188032791131469 ) ) ;
#3394=DIRECTION ( 'NONE',  ( -0.9998004120163609398, 0.000000000000000000, -0.01997839162482749689 ) ) ;
#3395=CARTESIAN_POINT ( 'NONE',  ( -4.656930922224128189, 118.0313578534626089, 0.5881568660916046687 ) ) ;
#3398=CARTESIAN_POINT ( 'NONE',  ( 0.02551629668039365542, 118.7629491485454025, -1.276939826301569658 ) ) ;
#3399=CARTESIAN_POINT ( 'NONE',  ( -3.418166037675369306, 118.5938114843297342, -0.9285938376095641544 ) ) ;
#3400=CARTESIAN_POINT ( 'NONE',  ( -4.713882987175448847, 112.7966860322829206, -2.559857038700545928 ) ) ;
#3401=CARTESIAN_POINT ( 'NONE',  ( 4.706919409142078514, 117.7550815031327573, 1.085396228939788932 ) ) ;
#3403=CARTESIAN_POINT ( 'NONE',  ( -9.757351933493584539, 123.8372022493589100, -0.9812814142356128810 ) ) ;
#3404=CARTESIAN_POINT ( 'NONE',  ( -3.088186736232249263, 115.7029548917814026, -1.663143839991825468 ) ) ;
#3406=DIRECTION ( 'NONE',  ( 5.206863593109713661E-17, -1.000000000000000000, 1.077750396879097183E-30 ) ) ;
#3407=CARTESIAN_POINT ( 'NONE',  ( 0.8777885371162424955, 105.9485402691003060, -5.279836415571006469 ) ) ;
#3408=CARTESIAN_POINT ( 'NONE',  ( -16.06787389343327277, 149.3012944676311804, -2.013231008103360864 ) ) ;
#3410=CARTESIAN_POINT ( 'NONE',  ( -0.03153862713815891450, 157.4657262375360176, 1.578321868909182690 ) ) ;
#3412=CARTESIAN_POINT ( 'NONE',  ( -2.879335978063669810, 156.0997340136324851, -0.01403285518562221064 ) ) ;
#3413=ADVANCED_FACE ( 'NONE', ( #4985 ), #17943, .T. ) ;
#3414=CARTESIAN_POINT ( 'NONE',  ( -3.812863311134618183, 2.017465188139291765, -2.614655560905410958 ) ) ;
#3415=CARTESIAN_POINT ( 'NONE',  ( 7.903286925170525556, 158.6683511845044734, 0.6884992853041227434 ) ) ;
#3416=ORIENTED_EDGE ( 'NONE', *, *, #10958, .T. ) ;
#3417=CARTESIAN_POINT ( 'NONE',  ( 4.808131379915038472, 104.6144662015457669, -0.4149153341867673483 ) ) ;
#3418=CARTESIAN_POINT ( 'NONE',  ( 3.847030120444227208, -15.22745156820166912, 0.3463556848800000143 ) ) ;
#3419=CARTESIAN_POINT ( 'NONE',  ( -5.877700541659460320, 119.5807162246413498, 0.9453723347071266714 ) ) ;
#3420=CARTESIAN_POINT ( 'NONE',  ( 0.1873809172457601979, 14.59626481882237492, -0.9553521702420578743 ) ) ;
#3421=CARTESIAN_POINT ( 'NONE',  ( -22.84108495963322838, 150.1122123445777277, -1.048654020290956224 ) ) ;
#3422=CARTESIAN_POINT ( 'NONE',  ( 0.8051319862491574941, 7.640635046448309708, 0.5515409728216702501 ) ) ;
#3428=CARTESIAN_POINT ( 'NONE',  ( 1.786380800136739833, 106.8720524443079967, 4.898415999051429992 ) ) ;
#3429=CARTESIAN_POINT ( 'NONE',  ( -10.29759560803370277, 124.8461398015159745, 0.5204633524205696249 ) ) ;
#3430=CARTESIAN_POINT ( 'NONE',  ( 4.137648320759505616, -13.26899632091267733, 3.249298663494996298 ) ) ;
#3431=CARTESIAN_POINT ( 'NONE',  ( 11.07124803888933506, 123.5714170083676748, -1.086458317614992231 ) ) ;
#3432=CARTESIAN_POINT ( 'NONE',  ( -2.300165013716055196, 118.7486697826011977, -0.8022418554901108445 ) ) ;
#3435=CARTESIAN_POINT ( 'NONE',  ( 2.356490753556696571, -15.00856118213019030, 5.009515689243722925 ) ) ;
#3436=CARTESIAN_POINT ( 'NONE',  ( -0.09153888643297225514, 38.16702564188061331, -1.140315812098650960 ) ) ;
#3437=CARTESIAN_POINT ( 'NONE',  ( 7.884012465051688956, 154.6027768716304820, -0.2197914096094749914 ) ) ;
#3439=CARTESIAN_POINT ( 'NONE',  ( -4.659482878567669850, 112.0093730493838819, 2.672389468958488834 ) ) ;
#3440=DIRECTION ( 'NONE',  ( -0.9998004119305863302, -1.254898720634597213E-08, -0.01997839591733275785 ) ) ;
#3444=ADVANCED_FACE ( 'NONE', ( #27748 ), #14962, .T. ) ;
#3446=CARTESIAN_POINT ( 'NONE',  ( 13.64797835309719076, 119.6379125180634446, 0.1726152169769649691 ) ) ;
#3447=CARTESIAN_POINT ( 'NONE',  ( -6.943414100881930118, 121.8132169909553966, 0.01755787080488258392 ) ) ;
#3449=CARTESIAN_POINT ( 'NONE',  ( -2.253372707275640430, 115.6909491485452577, 1.622700018657069920 ) ) ;
#3450=CARTESIAN_POINT ( 'NONE',  ( 1.686640475165922748, -9.627085671684914914, -4.319569293544198274 ) ) ;
#3451=CARTESIAN_POINT ( 'NONE',  ( -4.854047724237823047, 31.68081860726809751, -0.1332975631430312891 ) ) ;
#3452=CARTESIAN_POINT ( 'NONE',  ( 10.46214381725860498, 120.0128241960130424, 1.483189230905844758 ) ) ;
#3454=CARTESIAN_POINT ( 'NONE',  ( -0.8806307086779237014, 20.21867702141905099, 4.540528814573361771 ) ) ;
#3455=CARTESIAN_POINT ( 'NONE',  ( -2.299398447937291756, 29.65396322172144039, -8.101725167555347440 ) ) ;
#3456=CARTESIAN_POINT ( 'NONE',  ( -8.699715645159683319, 118.0981485975619734, -0.8502983169828192134 ) ) ;
#3457=CARTESIAN_POINT ( 'NONE',  ( -0.7855309748069307929, 120.8419495465347069, -0.4764688261655855017 ) ) ;
#3458=CARTESIAN_POINT ( 'NONE',  ( -23.34372044208206631, 149.0681261006343163, -0.4664630893998606975 ) ) ;
#3459=CARTESIAN_POINT ( 'NONE',  ( 1.119229806841262498, 106.1659139100990785, -5.173940658946511562 ) ) ;
#3460=CARTESIAN_POINT ( 'NONE',  ( -1.280639713796333012, 104.6144662015413331, 5.189622541085106455 ) ) ;
#3461=CARTESIAN_POINT ( 'NONE',  ( 3.043391175932955495, 18.63480288530714191, -3.501419995799015528 ) ) ;
#3462=DIRECTION ( 'NONE',  ( 0.9998004120163608288, 0.000000000000000000, 0.01997839162482750383 ) ) ;
#3464=CARTESIAN_POINT ( 'NONE',  ( 2.931439949929583122, -14.82325452411255640, 4.117531814738872420 ) ) ;
#3467=CARTESIAN_POINT ( 'NONE',  ( 2.121281617406954645, 114.8832439220486350, -1.889083087725354826 ) ) ;
#3468=CARTESIAN_POINT ( 'NONE',  ( -23.06568927493573895, 148.7220611141358404, 0.3950670065760724659 ) ) ;
#3472=CARTESIAN_POINT ( 'NONE',  ( -5.250802080936233907, 115.7029491485453718, 0.9230947160017799469 ) ) ;
#3473=CARTESIAN_POINT ( 'NONE',  ( 3.918620257527314799, -15.59263167233598857, 4.836928646374421881 ) ) ;
#3474=CARTESIAN_POINT ( 'NONE',  ( -5.882864265865931586, 118.8996324090661147, 0.9452689120681909696 ) ) ;
#3475=AXIS2_PLACEMENT_3D ( 'NONE', #16288, #25880, #29078 ) ;
#3476=CARTESIAN_POINT ( 'NONE',  ( 9.838452836889429065, 157.5983698538113629, -1.280564089889915547 ) ) ;
#3479=CARTESIAN_POINT ( 'NONE',  ( -0.8823465807374654135, 5.041073445128725794, 4.537322665494407659 ) ) ;
#3481=VERTEX_POINT ( 'NONE', #31998 ) ;
#3483=CARTESIAN_POINT ( 'NONE',  ( 0.3783624953763569110, 110.0486234891351245, 3.695659563127995373 ) ) ;
#3484=CARTESIAN_POINT ( 'NONE',  ( -4.646525074885831330, 117.9326234303812555, 0.7781659370121971619 ) ) ;
#3485=B_SPLINE_SURFACE_WITH_KNOTS ( 'NONE', 3, 3, ( 
 ( #9925, #19711, #32731, #13551, #996, #7797, #17566, #1408, #30569, #23958, #26541, #577, #23746, #40385, #36976, #39548, #30353, #4611, #33574, #783, #14364, #16733, #33157, #10351, #11180, #4408, #27375, #40178, #7174, #36765, #23322, #36358, #23531, #10974, #37174, #20758, #24165, #13758, #33783, #19928, #32945, #3774, #17365, #13960, #29737, #7584, #26755 ),
 ( #20335, #20545, #10559, #20133, #3985, #39973, #27168, #16945, #30155, #29943, #1202, #26959, #39764, #14162, #36558, #10764, #7375, #33360, #4193, #17155, #41592, #22368, #38180, #25179, #12802, #33989, #28792, #9403, #12400, #17770, #21166, #8994, #37380, #27579, #30768, #5813, #38393, #9204, #2825, #8195, #34198, #1618, #31566, #2407, #25589, #35393, #42005 ),
 ( #22163, #14574, #5022, #3033, #40586, #18560, #21962, #6019, #25793, #6222, #31987, #18769, #7998, #11386, #15367, #28373, #18983, #24372, #41380, #15784, #20966, #12186, #34992, #31778, #2619, #15579, #19192, #41804, #35193, #12602, #38596, #28584, #32199, #25390, #15988, #28989, #4816, #33256, #17046, #10028, #16838, #6425, #10451, #22998, #255, #3235, #36029 ),
 ( #3658, #22578, #39646, #16194, #39432, #32614, #19398, #20026, #7270, #13008, #29631, #6841, #3446, #29415, #39220, #42, #32403, #13231, #26001, #19812, #39011, #32829, #35821, #36450, #26639, #16624, #29199, #30046, #29838, #23422, #469, #678, #20232, #9820, #22786, #26214, #4087, #6635, #19602, #886, #16409, #35609, #13441, #13857, #26428, #38798, #10237 ),
 ( #23206, #9610, #36241, #7061, #33044, #3875, #13647, #11286, #1517, #4923, #14473, #4296, #34305, #17261, #20861, #31089, #10658, #30669, #30881, #4502, #40072, #14263, #11488, #33886, #23855, #27273, #24273, #1927, #24475, #8096, #37078, #26854, #33469, #10868, #33680, #37277, #30252, #36875, #21070, #39861, #1093, #7691, #17465, #20651, #40288, #37479, #34095 ),
 ( #27483, #30461, #8305, #11080, #1305, #40694, #23638, #21275, #5134, #24066, #17878, #36660, #18085, #7898, #4714, #14061, #17669, #7482, #20441, #40492, #27065, #27685, #1722, #14679, #8726, #24689, #38331, #25535, #31292, #5758, #12127, #21688, #5542, #15310, #18290, #37697, #18500, #2136, #25116, #15097, #28315, #11916, #12545, #2769, #41324, #8519, #35337 ),
 ( #38119, #5963, #15725, #28098, #21477, #31504, #22313, #41110, #24905, #38536, #34510, #40898, #34712, #28730, #37905, #14888, #2564, #2352, #8934, #21902, #9351, #34931, #6166, #32139, #5336, #35135, #41533, #31720, #18921, #15524, #18710, #19135, #28526, #12339, #27891, #11702, #25328, #31932, #9150, #22107, #41742, #29787, #9969, #29139, #26161, #26371, #35759 ),
 ( #12750, #32776, #9764, #3386, #16353, #12952, #29360, #3606, #6575, #26585, #19338, #22942, #10181, #7220, #13173, #9551, #13383, #39163, #35553, #16569, #36403, #35970, #626, #19543, #32553, #15935, #6786, #16785, #197, #19753, #20182, #28931, #23150, #3822, #29580, #25736, #16138, #414, #32345, #22523, #38744, #39379, #36188, #7008, #19976, #3173, #42156 ),
 ( #41949, #32993, #39595, #13597, #10399, #25943, #23370, #2970, #6368, #22729, #38954, #37227, #37429, #37030, #29991, #16992, #14628, #1257, #33411, #4243, #33626, #4455, #27220, #7846, #40642, #20386, #8046, #8250, #27013, #24010, #14212, #1461, #11436, #30202, #40234, #831, #20807, #33833, #24424, #26803, #11029, #21019, #30826, #27631, #1673, #34042, #39812 ),
 ( #33206, #4870, #10605, #14421, #17828, #4661, #14007, #4031, #13806, #17205, #23585, #36609, #17617, #7428, #11233, #1043, #30619, #40022, #10816, #36818, #24217, #23799, #7637, #20596, #17412, #30408, #27428, #40440, #25495, #34878, #2301, #31034, #8885, #28049, #21427, #8472, #1875, #2084, #18034, #12291, #2723, #15261, #18452, #34456, #12077, #31457, #18878 ),
 ( #25278, #38493, #25065, #14837, #5082, #15681, #28265, #5288, #18238, #21637, #34663, #41272, #38068, #28684, #31240, #38283, #21222, #15047, #21849, #5710, #31674, #41693, #41058, #18667, #27842, #2514, #15478, #12503, #40849, #28479, #9102, #31887, #34252, #11651, #22067, #24636, #37647, #41484, #11868, #35094, #24858, #5916, #37854, #8677, #5491, #19934, #6125 ),
 ( #28894, #16738, #41909, #3348, #13554, #35297, #13130, #13340, #29101, #22480, #38911, #36147, #16314, #35508, #32517, #32735, #42120, #372, #6328, #9930, #19090, #19298, #3779, #32094, #32304, #9723, #6747, #26544, #6962, #3566, #19506, #9311, #15890, #3135, #16095, #19715, #12709, #12913, #16527, #22273, #25698, #25906, #22689, #35722, #6531, #32950, #29536 ),
 ( #2928, #26327, #10141, #26120, #38704, #29318, #160, #9511, #39124, #22898, #35935, #39333, #23111, #29742, #582, #23961, #33160, #1207, #33787, #17368, #23536, #17570, #23326, #26758, #7177, #14368, #30358, #4614, #40183, #786, #20548, #16948, #3989, #33363, #10978, #11183, #36980, #40389, #36562, #7800, #30572, #27379, #39551, #14165, #10769, #20138, #4411 ),
 ( #7378, #999, #27172, #4196, #1412, #13761, #7587, #20762, #10354, #23749, #29946, #36362, #39768, #30158, #10563, #20339, #17158, #13963, #26966, #39976, #33578, #36769, #1380, #34374, #30542, #17957, #14551, #34586, #34171, #11364, #21558, #33756, #2221, #28184, #21142, #27970, #17541, #5415, #4999, #24350, #14338, #30957, #41189, #27348, #14760, #4582, #8594 ),
 ( #1594, #40361, #31165, #18370, #24141, #40771, #1797, #27559, #40566, #8175, #11156, #37149, #37356, #7971, #27761, #20940, #11569, #4793, #31377, #37770, #24555, #33965, #11992, #40980, #15181, #37559, #11782, #24987, #17744, #30744, #8385, #7769, #21349, #5207, #20732, #18162, #2006, #14968, #24772, #5839, #37987, #25614, #12211, #25417, #21985, #19006, #19217 ),
 ( #35018, #38624, #5629, #9022, #32431, #18587, #18792, #38418, #35421, #70, #22605, #32227, #6044, #13039, #2432, #31805, #2642, #6248, #41404, #15602, #3059, #8811, #25201, #28607, #41615, #12425, #9230, #35637, #31596, #22397, #15393, #32010, #22188, #6451, #35218, #2849, #9637, #21770, #3262, #16222, #15809, #16016, #28399, #19425, #28817, #41832, #38205 ),
 ( #12626, #9427, #34796, #38827, #29015, #42035, #12830, #25818, #29228, #37256, #283, #16866, #23236, #32857, #16650, #26458, #29444, #6664, #29657, #13256, #36271, #26240, #39462, #23027, #24248, #14448, #10264, #19627, #4900, #4690, #27458, #7091, #17646, #40471, #39248, #32642, #497, #34073, #10056, #36057, #8074, #3476, #9845, #3689, #11262, #6871, #26029 ),
 ( #17855, #30648, #16437, #36476, #21048, #39676, #19843, #30856, #22812, #13469, #20053, #1701, #10479, #39038, #1491, #33072, #706, #3903, #29866, #13677, #35850, #26668, #23448, #7296, #20837, #33861, #35117, #41300, #41511, #34905, #1903, #31483, #18062, #21251, #18267, #5737, #31913, #31700, #18903, #37674, #2542, #28503, #5944, #14656, #28293, #37881, #24453 ),
 ( #15076, #24665, #28076, #15288, #5316, #38308, #31065, #34691, #21879, #27660, #24884, #34281, #25093, #8704, #5110, #2328, #40671, #21667, #12317, #31270, #2112, #11463, #5520, #25305, #8913, #18478, #12104, #38098, #18690, #15503, #9129, #37457, #27869, #41087, #14866, #40877, #8281, #11895, #22090, #11678, #8497, #21454, #34484, #12525, #25720, #41719, #35956 ),
 ( #42144, #2951, #35744, #12938, #397, #22504, #2750, #6770, #6988, #6556, #25516, #28710, #26353, #25928, #15915, #28915, #3157, #16121, #38936, #19531, #10164, #32121, #19736, #19957, #38727, #32538, #9747, #13153, #23132, #41930, #22716, #38516, #3371, #16337, #36170, #9333, #29342, #32757, #13364, #39359, #15705, #3591, #22296, #35321, #184, #6148, #16552 ),
 ( #29561, #26146, #9535, #19114, #12731, #35534, #6353, #19324, #32328, #29124, #39148, #9952, #22925, #23778, #30184, #30602, #10588, #32976, #37008, #37209, #36799, #29770, #16763, #14400, #1025, #33187, #4015, #33390, #4224, #26994, #7617, #40418, #20162, #7827, #8029, #26783, #20578, #13989, #1238, #11214, #29971, #40005, #606, #33604, #4437, #24198, #26568 ),
 ( #39794, #20789, #811, #3801, #17395, #7204, #20368, #10796, #27408, #23566, #13580, #39575, #10381, #11010, #30387, #14194, #23989, #27199, #23350, #36388, #16972, #40212, #13787, #36588, #33814, #4641, #7406, #17185, #17598, #1440, #28027, #5059, #2063, #2279, #11628, #12054, #18015, #21615, #30803, #34230, #15456, #1652, #31012, #21404, #18429, #25259, #5689 ),
 ( #38264, #31219, #27612, #31437, #15027, #11420, #8655, #12270, #41037, #18646, #24615, #37623, #34025, #11846, #34857, #15243, #24833, #37828, #28244, #41248, #21828, #34642, #14607, #1855, #34432, #8231, #40622, #24406, #18218, #5470, #25043, #38046, #21204, #14818, #37412, #31653, #5266, #8446, #27820, #8866, #41463, #40829, #2493, #4850, #28457, #21000, #17806 ),
 ( #32495, #19693, #25477, #42099, #6307, #15871, #41890, #9491, #12483, #31862, #12688, #38473, #19279, #9291, #22456, #6103, #6725, #39102, #35485, #2702, #29512, #29294, #9905, #32287, #137, #22877, #22252, #15659, #25678, #16505, #35278, #19066, #32710, #28663, #35075, #28877, #35915, #32072, #9081, #38889, #2908, #38685, #3116, #3544, #16076, #351, #26304 ),
 ( #35700, #25882, #13104, #9701, #41675, #13318, #29080, #12894, #22046, #5896, #22667, #26096, #6511, #19486, #3323, #18858, #16290, #23302, #20316, #20527, #29927, #30335, #36339, #39952, #6939, #10332, #33766, #19910, #7155, #39743, #36746, #1390, #23940, #33557, #7357, #14346, #3756, #20114, #3966, #7567, #559, #33136, #4389, #39313, #13534, #16927, #765 ),
 ( #36957, #32925, #23727, #16714, #33343, #13741, #7778, #23511, #26735, #10953, #23091, #4591, #17550, #10542, #17347, #29717, #1182, #20741, #10746, #36538, #30551, #36125, #4173, #26522, #10120, #14145, #39528, #27148, #17135, #13943, #30137, #976, #26941, #40160, #2443, #2231, #31605, #8183, #15191, #41200, #18597, #27357, #40988, #8395, #37158, #14978, #34181 ),
 ( #27770, #27980, #17967, #8820, #1603, #5217, #34595, #40369, #37568, #33973, #37780, #21357, #17752, #11791, #11164, #34383, #12004, #30966, #1807, #24149, #18171, #24996, #21567, #31174, #2015, #24782, #5424, #28194, #8605, #7980, #40575, #40781, #14559, #4801, #20949, #24564, #18379, #31388, #37996, #27566, #11372, #30752, #21151, #24359, #21779, #34805, #5639 ),
 ( #37364, #5007, #14768, #11579, #6256, #12637, #22199, #6054, #15819, #18803, #38214, #19015, #31814, #25624, #15610, #28827, #12433, #13047, #3272, #41841, #9031, #35860, #35647, #16233, #38634, #6461, #29237, #28615, #21996, #32020, #22823, #41625, #2651, #26038, #35028, #41414, #35228, #80, #25426, #15404, #3068, #38427, #2858, #9438, #9853, #25210, #9241 ),
 ( #39047, #22406, #35431, #19226, #32236, #16026, #6673, #29026, #28408, #19435, #19638, #42045, #12220, #5848, #32653, #12841, #25827, #38836, #9646, #22613, #32441, #20265, #10900, #32867, #7515, #20692, #39471, #36485, #13687, #13895, #23890, #507, #26679, #29453, #33293, #7306, #36908, #39259, #39686, #33503, #1128, #27096, #14097, #20476, #10065, #26249, #4122 ),
 ( #23036, #26887, #30287, #17082, #26467, #40106, #292, #16659, #36068, #7725, #30083, #3488, #23673, #3699, #921, #6883, #19853, #7100, #36692, #16447, #4332, #13265, #10275, #17297, #29666, #13480, #23246, #39896, #10488, #36279, #10693, #20061, #3913, #33082, #16875, #29876, #714, #23458, #7931, #11530, #40937, #37947, #1759, #40322, #1966, #14719, #24103 ),
 ( #27721, #18332, #37315, #24310, #4538, #24511, #5377, #27930, #40730, #8343, #31129, #11745, #34552, #37518, #1339, #4751, #34129, #20900, #11114, #14296, #30921, #21311, #34341, #24732, #33921, #17704, #37735, #18124, #5170, #8559, #14930, #37111, #41149, #30703, #21519, #8772, #17499, #31335, #2179, #11321, #1553, #21105, #15138, #28141, #14508, #11955, #24946 ),
 ( #33716, #27307, #27522, #30497, #40529, #8131, #4956, #17915, #25989, #6412, #3018, #31973, #38998, #28357, #5797, #28568, #32185, #25164, #31762, #15975, #21732, #38164, #18753, #41576, #2605, #35177, #19384, #15352, #6208, #2393, #2810, #12385, #32388, #6004, #25372, #35595, #5588, #16181, #31, #18966, #41991, #31547, #3219, #15771, #38376, #41365, #28776 ),
 ( #41786, #18544, #22566, #12168, #22354, #15564, #8978, #28972, #29184, #21945, #12586, #25575, #9190, #22146, #38579, #34974, #9391, #35379, #19179, #12788, #25778, #38786, #9596, #12995, #34754, #10223, #32598, #30239, #30031, #10645, #20014, #872, #39850, #22987, #16396, #26415, #17246, #10014, #26202, #7467, #29402, #35806, #16612, #23626, #19797, #9807, #39633 ),
 ( #3861, #4282, #29620, #1079, #27052, #242, #33033, #26625, #7258, #13844, #36645, #13634, #19588, #36014, #23192, #39206, #13219, #3431, #7048, #10438, #23409, #4073, #6828, #32817, #3647, #455, #6620, #26842, #33454, #16825, #29827, #13427, #666, #36440, #20427, #39419, #22775, #14048, #36226, #20218, #33244, #17033, #21464, #8084, #40273, #11068, #40480 ),
 ( #14666, #5325, #27258, #1914, #15085, #33872, #30865, #21057, #8291, #18278, #37067, #34083, #23839, #27670, #1711, #31279, #33666, #4910, #27878, #37684, #34494, #8506, #14876, #4490, #20636, #40681, #2123, #40887, #17449, #21261, #24675, #11473, #20847, #40059, #36860, #24052, #30448, #10852, #24462, #7677, #18073, #7885, #37467, #1293, #14250, #1502, #31074 ),
 ( #4702, #17656, #11689, #30657, #14458, #27470, #34291, #17865, #11274, #5120, #24257, #37265, #38107, #28514, #29301, #18699, #10125, #2338, #5952, #35921, #32931, #38320, #34701, #39108, #9139, #18487, #16299, #19916, #22098, #13323, #31710, #2551, #41097, #18912, #357, #22883, #25315, #34917, #15512, #41521, #31493, #8715, #12327, #15297, #35126, #28303, #32501 ),
 ( #41309, #32718, #3761, #21888, #3330, #145, #9913, #6948, #25104, #13111, #11904, #26103, #6731, #28086, #21677, #19699, #16511, #26311, #23097, #39319, #3552, #5530, #12114, #29517, #24893, #36130, #8923, #37890, #5747, #30341, #39752, #27363, #13539, #29932, #39533, #37162, #1189, #1395, #36964, #3972, #33563, #20119, #23310, #20322, #7785, #33976, #33771 ),
 ( #4598, #30556, #7984, #20954, #14150, #39959, #26528, #4396, #23517, #17142, #26742, #30144, #17352, #7364, #40374, #33144, #36753, #23946, #16720, #26946, #36345, #27153, #10751, #7160, #40167, #29723, #23733, #14351, #33349, #4178, #565, #7572, #11169, #10959, #20533, #20746, #17554, #24153, #10339, #16933, #770, #13747, #983, #10548, #36545, #13949, #2018 ),
 ( #41203, #5012, #34185, #14564, #27773, #1607, #38001, #28412, #40992, #14982, #17971, #37783, #27984, #2447, #24567, #4805, #30757, #41417, #25215, #18175, #25000, #27569, #18602, #31177, #8399, #11375, #11796, #38218, #40578, #24785, #24362, #5643, #37368, #5427, #40784, #8186, #28198, #15407, #21155, #8608, #21572, #11584, #37573, #5221, #30970, #1810, #21360 ),
 ( #14773, #34598, #34386, #12224, #34809, #18383, #31391, #9036, #8823, #31608, #2236, #21783, #22000, #15195, #12007, #17756, #298, #35233, #9245, #32659, #12437, #18807, #41845, #22828, #2863, #35032, #22619, #22202, #22410, #29031, #29459, #12641, #26254, #10070, #25430, #13052, #19440, #9651, #26043, #35653, #38430, #13270, #6058, #42052, #39264, #31817, #38842 ),
 ( #19018, #35437, #19644, #12847, #32025, #16031, #16239, #25629, #39053, #15824, #6466, #2655, #28832, #5851, #15613, #38639, #6261, #32446, #28618, #3494, #29242, #3073, #41629, #9444, #19232, #32242, #3278, #25833, #87, #9858, #35865, #6678, #16453, #719, #33087, #36490, #20696, #16664, #7519, #3705, #33299, #29881, #7730, #7310, #26684, #36912, #14102 ),
 ( #36286, #17504, #29671, #20066, #23464, #20481, #27312, #33720, #4340, #4127, #40326, #512, #7107, #13694, #33507, #26473, #3918, #17301, #23042, #39477, #16880, #39694, #10494, #20270, #4545, #13486, #30292, #10281, #17087, #30089, #30502, #928, #13901, #1344, #6890, #14300, #36073, #26891, #1134, #32874, #19858, #39903, #10698, #23252, #23678, #36698, #27101 ),
 ( #23895, #40112, #10905, #4961, #20906, #34556, #21737, #27527, #1970, #8347, #17921, #1764, #11535, #14516, #33927, #14724, #40533, #21317, #11327, #24517, #8137, #8777, #41154, #37523, #4758, #31554, #31341, #11960, #34345, #2186, #24952, #24314, #17709, #27725, #18550, #37321, #21110, #34760, #30708, #37115, #30926, #37953, #34135, #11120, #40943, #40734, #5175 ),
 ( #18128, #2398, #28363, #1558, #15144, #37740, #27936, #28147, #11749, #31133, #15357, #14934, #24737, #24108, #7935, #8563, #5594, #21524, #5381, #18337, #25994, #6214, #25377, #22359, #22571, #31978, #8983, #22152, #38170, #32393, #22780, #35384, #38586, #41582, #32190, #9395, #39003, #18971, #41370, #3226, #3437, #3024, #21951, #25170, #35811, #19185, #12390 ),
 ( #41793, #15980, #28978, #6627, #28574, #16186, #16402, #35183, #41997, #12794, #9602, #19594, #38383, #25783, #34981, #38791, #35601, #32604, #5803, #6418, #29190, #9814, #12174, #18758, #36, #31768, #2610, #19389, #15569, #13001, #9195, #6009, #2817, #15776, #28781, #12592, #25580, #461, #10020, #7683, #13849, #14054, #7474, #16618, #4080, #32822, #36019 ),
 ( #4496, #4288, #33673, #10229, #17253, #1087, #20642, #29407, #878, #10444, #39212, #17038, #36232, #29833, #39423, #671, #30037, #20020, #10858, #3651, #7263, #36652, #247, #39638, #6833, #39855, #23415, #19804, #26848, #13225, #36445, #27058, #33038, #3866, #26208, #20223, #40066, #23632, #33250, #10651, #20433, #33461, #30245, #23847, #22992, #13434, #13639 ),
 ( #36868, #29625, #26420, #26632, #16831, #23198, #7053, #24264, #2128, #1716, #21062, #31285, #1299, #11909, #37897, #30872, #37690, #27264, #15091, #14672, #34088, #24057, #27676, #8719, #40281, #24469, #14255, #18283, #37072, #18078, #11279, #11073, #40892, #28092, #33880, #8299, #40688, #37270, #8090, #17871, #20852, #7891, #4917, #4708, #11480, #17661, #37472 ),
 ( #5329, #21268, #30662, #21681, #8512, #41103, #34297, #21471, #24898, #1510, #14464, #5127, #34705, #27476, #40485, #17457, #31081, #1920, #14882, #30455, #27884, #11696, #24682, #34501, #25319, #5956, #38736, #15517, #35545, #6361, #12120, #6157, #25526, #28722, #35330, #41732, #25109, #9544, #38113, #18915, #5535, #31497, #12538, #32131, #28519, #5751, #38325 ),
 ( #18703, #31925, #19125, #41526, #2963, #31714, #38527, #15302, #34924, #22514, #28308, #2556, #9143, #9343, #18493, #25729, #15925, #2762, #2345, #12332, #22100, #35129, #28923, #15717, #22306, #41941, #41315, #12741, #8927, #21895, #11408, #14806, #41238, #37196, #28016, #24186, #11617, #24604, #8017, #11834, #37609, #34010, #31208, #34846, #8435, #28232, #5047 ),
 ( #34420, #15233, #37816, #21393, #18207, #41026, #21604, #2269, #5253, #11200, #14594, #1842, #30790, #20988, #4839, #40816, #2051, #15016, #8643, #1640, #27599, #17793, #24395, #40406, #34632, #25032, #24821, #5459, #40609, #18419, #31427, #12043, #21191, #1429, #38035, #5679, #8855, #37400, #27395, #21819, #18637, #8218, #34218, #27808, #14388, #18002, #31000 ),
 ( #35689, #6713, #25467, #22444, #41878, #42088, #9893, #28653, #12677, #15444, #6297, #35473, #22866, #25250, #25667, #19476, #29283, #13092, #127, #6498, #38254, #12257, #19268, #35904, #32484, #9071, #12883, #16278, #3105, #12473, #26084, #28447, #2691, #22036, #31642, #16066, #39091, #9689, #18848, #32275, #35064, #5886, #35267, #22656, #2482, #3312, #41452 ),
 ( #31852, #15648, #29069, #38674, #41665, #25871, #38463, #32059, #9281, #2898, #38877, #22241, #6091, #19054, #9480, #15860, #28866, #1172, #29916, #19898, #32913, #20101, #33125, #13730, #36527, #27137, #6927, #23716, #36948, #13522, #10531, #755, #30126, #40150, #16701, #26724, #3534, #7347, #23500, #10943, #13305, #39732, #7557, #17336, #14135, #30327, #36734 ) ),
 .UNSPECIFIED., .F., .F., .F.,
 ( 4, 1, 1, 1, 1, 1, 1, 1, 1, 1, 1, 1, 1, 1, 1, 1, 1, 1, 1, 1, 1, 1, 1, 1, 1, 1, 1, 1, 1, 1, 1, 1, 1, 1, 1, 1, 1, 1, 1, 1, 1, 1, 1, 1, 1, 1, 3, 4 ),
 ( 4, 1, 1, 1, 1, 1, 1, 1, 1, 1, 1, 1, 2, 1, 1, 1, 2, 1, 1, 1, 1, 1, 2, 1, 1, 1, 1, 1, 1, 1, 2, 1, 1, 1, 1, 1, 1, 1, 1, 1, 4 ),
 ( 0.000000000000000000, 0.007812500000000000000, 0.01562500000000000000, 0.02343750000000000000, 0.03125000000000000000, 0.04687500000000000000, 0.06250000000000000000, 0.07812500000000000000, 0.09375000000000000000, 0.1093750000000000000, 0.1250000000000000000, 0.1406250000000000000, 0.1562500000000000000, 0.1875000000000000000, 0.2187500000000000000, 0.2500000000000000000, 0.2812500000000000000, 0.3125000000000000000, 0.3281250000000000000, 0.3437500000000000000, 0.3750000000000000000, 0.4062500000000000000, 0.4375000000000000000, 0.4687500000000000000, 0.5000000000000000000, 0.5312500000000000000, 0.5625000000000000000, 0.5937500000000000000, 0.6250000000000000000, 0.6562500000000000000, 0.6718750000000000000, 0.6875000000000000000, 0.7187500000000000000, 0.7500000000000000000, 0.7812500000000000000, 0.8125000000000000000, 0.8437500000000000000, 0.8750000000000000000, 0.8906250000000000000, 0.9062500000000000000, 0.9218750000000000000, 0.9375000000000000000, 0.9531250000000000000, 0.9687500000000000000, 0.9765625000000000000, 0.9843750000000000000, 1.000000000000000000, 1.020392624918932789 ),
 ( 0.000000000000000000, 0.01539374999999999945, 0.03078749999999999890, 0.04618125000000002089, 0.06157499999999999779, 0.07696875000000003020, 0.09236250000000004179, 0.1077562499999999979, 0.1231499999999999956, 0.1431375000000000008, 0.1631250000000000200, 0.1831125000000000114, 0.2031000000000000028, 0.2063375000000000070, 0.2095750000000000113, 0.2128125000000000155, 0.2160500000000000198, 0.2667375000000000163, 0.3174250000000000682, 0.3681125000000000647, 0.4188000000000000611, 0.5201750000000000540, 0.6215500000000000469, 0.6266374999999999584, 0.6317250000000000920, 0.6368124999999997815, 0.6418999999999999151, 0.6469874999999999376, 0.6520749999999999602, 0.6571624999999999828, 0.6622500000000000053, 0.7044687500000000879, 0.7466875000000001705, 0.7889062500000000311, 0.8010555555555555207, 0.8311249999999998916, 0.8733437499999998632, 0.9155625000000000568, 0.9403166666666666895, 0.9577812500000000284, 1.000000000000000000 ),
 .UNSPECIFIED. ) ;
#3486=CARTESIAN_POINT ( 'NONE',  ( -10.40651172546669301, 123.5464890276372785, 0.9122707376378308419 ) ) ;
#3487=DIRECTION ( 'NONE',  ( -4.017660918040594346E-17, 1.000000000000000000, 2.376309959284834438E-19 ) ) ;
#3488=CARTESIAN_POINT ( 'NONE',  ( 9.425666535144223701, 121.4347015428822374, -1.122958709584367831 ) ) ;
#3489=AXIS2_PLACEMENT_3D ( 'NONE', #21685, #5132, #18708 ) ;
#3490=CARTESIAN_POINT ( 'NONE',  ( -20.78747236883577543, 145.7124547906547889, -2.408930808681182256 ) ) ;
#3493=CARTESIAN_POINT ( 'NONE',  ( 4.527352789474797135, 118.1161674766824206, -0.5309711699598146373 ) ) ;
#3494=CARTESIAN_POINT ( 'NONE',  ( 10.17757484390027756, 124.8647468421599598, -0.4356504197092352926 ) ) ;
#3496=CARTESIAN_POINT ( 'NONE',  ( -10.71652553037534794, 154.3566586077636487, -1.965850361453045814 ) ) ;
#3497=CARTESIAN_POINT ( 'NONE',  ( 3.057239904206551895, -15.51127639645041789, 4.278020201805971645 ) ) ;
#3498=DIRECTION ( 'NONE',  ( -5.206863593109713661E-17, 1.000000000000000000, -1.077750396879097183E-30 ) ) ;
#3501=CARTESIAN_POINT ( 'NONE',  ( -4.942855899094846350, 117.6285334314414399, 0.7732941537803618148 ) ) ;
#3502=CARTESIAN_POINT ( 'NONE',  ( 6.550279792842248483, 120.6599796251122427, 1.081144621291421304 ) ) ;
#3503=CARTESIAN_POINT ( 'NONE',  ( -2.667392527469404140, 31.33771804890096746, 0.9893360403373157030 ) ) ;
#3504=AXIS2_PLACEMENT_3D ( 'NONE', #14295, #27306, #40321 ) ;
#3505=CARTESIAN_POINT ( 'NONE',  ( 3.400481176189167343, 25.78150505744974552, 3.158589348000393482 ) ) ;
#3506=CARTESIAN_POINT ( 'NONE',  ( 8.827910802434928428, 123.6950213215744583, 0.2595790122280457468 ) ) ;
#3511=CARTESIAN_POINT ( 'NONE',  ( 3.302029177305205732, 159.4671159221996959, 0.06598240135525389183 ) ) ;
#3512=CIRCLE ( 'NONE', #16406, 5.080000000000006288 ) ;
#3514=CARTESIAN_POINT ( 'NONE',  ( -8.438946883131665189, 119.3197881592811029, -1.362662033712001453 ) ) ;
#3516=CARTESIAN_POINT ( 'NONE',  ( -4.074955089416341991, 118.2429491485453354, 0.1454234154749719787 ) ) ;
#3520=CARTESIAN_POINT ( 'NONE',  ( -13.57554913733971347, 119.6371495169912436, -0.05144635950012913655 ) ) ;
#3523=CARTESIAN_POINT ( 'NONE',  ( 6.979485140712072599, 121.9514898806366006, 0.06293811663084028507 ) ) ;
#3524=ADVANCED_FACE ( 'NONE', ( #23015, #6652 ), #38610, .F. ) ;
#3525=ORIENTED_EDGE ( 'NONE', *, *, #6317, .T. ) ;
#3526=CARTESIAN_POINT ( 'NONE',  ( 4.357800360384668004, 115.7036734823842323, -1.373096195996742264 ) ) ;
#3527=CARTESIAN_POINT ( 'NONE',  ( -1.611903344789388903, 120.9971453638330985, -0.05790686387416373038 ) ) ;
#3528=CARTESIAN_POINT ( 'NONE',  ( 6.098373624802439608, -13.52034412102339012, 1.767782016118699895 ) ) ;
#3530=CARTESIAN_POINT ( 'NONE',  ( -21.28061085028127764, 148.8133262010608462, 1.460188425234498100 ) ) ;
#3532=CARTESIAN_POINT ( 'NONE',  ( -0.003073183581815366015, 116.5806198863164838, 0.1537946732117061177 ) ) ;
#3534=CARTESIAN_POINT ( 'NONE',  ( 13.58627218224582656, 150.2694722113990338, 0.4661934924574481776 ) ) ;
#3535=CARTESIAN_POINT ( 'NONE',  ( 4.965622106538171820, 115.6909491485453145, -1.258976657945148458 ) ) ;
#3536=CARTESIAN_POINT ( 'NONE',  ( 0.7743132463278736832, -9.628960163071635492, -0.5975928149734356376 ) ) ;
#3537=CARTESIAN_POINT ( 'NONE',  ( -23.32994265436209602, 149.0590277239482475, -0.6203886826157011258 ) ) ;
#3539=CARTESIAN_POINT ( 'NONE',  ( -8.727017694313293106, 118.0966776702152004, 0.5009128790051901037 ) ) ;
#3541=CARTESIAN_POINT ( 'NONE',  ( -11.64084037886373224, 123.0696236843973281, 1.242201319703144291 ) ) ;
#3543=CARTESIAN_POINT ( 'NONE',  ( 7.913941031674588622, 118.5968412048868288, 1.173277403367298577 ) ) ;
#3544=CARTESIAN_POINT ( 'NONE',  ( 4.562247774926673216, 157.9011380394538833, -1.652341844578318231 ) ) ;
#3545=CARTESIAN_POINT ( 'NONE',  ( -0.9635192623308774795, 7.475506455475952272, -0.1398073520734665620 ) ) ;
#3547=CARTESIAN_POINT ( 'NONE',  ( -21.70872022418687308, 149.0176745010074342, -2.143008773150906432 ) ) ;
#3548=CARTESIAN_POINT ( 'NONE',  ( 4.846611013106016941, 117.8246425087505713, -0.6900207181998705419 ) ) ;
#3549=AXIS2_PLACEMENT_3D ( 'NONE', #20288, #32680, #42071 ) ;
#3552=CARTESIAN_POINT ( 'NONE',  ( 11.70197428064578737, 126.1299551460304542, -0.9179571146301047646 ) ) ;
#3553=CARTESIAN_POINT ( 'NONE',  ( -5.966562942538025993, 155.3820107761045790, -0.07923228615413194231 ) ) ;
#3554=ORIENTED_EDGE ( 'NONE', *, *, #35530, .T. ) ;
#3555=CARTESIAN_POINT ( 'NONE',  ( 0.03153862713803012863, 157.4657262375360176, -1.578321868909182246 ) ) ;
#3556=CARTESIAN_POINT ( 'NONE',  ( 2.279390105945505507, -15.60765617898064761, 5.834426787525912594 ) ) ;
#3559=ORIENTED_EDGE ( 'NONE', *, *, #27736, .F. ) ;
#3560=CARTESIAN_POINT ( 'NONE',  ( 18.35242356974463718, 147.0160646422468744, 2.398428600884452866 ) ) ;
#3561=CARTESIAN_POINT ( 'NONE',  ( -15.77133435453296606, 146.5691041611200660, -0.3151487940933135334 ) ) ;
#3563=CARTESIAN_POINT ( 'NONE',  ( -3.258544586981842794, 118.6786177306206014, 0.6136036933997359721 ) ) ;
#3564=CARTESIAN_POINT ( 'NONE',  ( 8.062851560922409178, 27.27981867468588462, -2.430221966868060690 ) ) ;
#3565=CARTESIAN_POINT ( 'NONE',  ( 15.96902210417518475, 146.0164801329953548, 1.048924711619907191 ) ) ;
#3566=CARTESIAN_POINT ( 'NONE',  ( 22.74464968533188269, 149.4207734315791072, -0.6238039466385614240 ) ) ;
#3567=CARTESIAN_POINT ( 'NONE',  ( 4.610436209567292387, 117.9340757871244847, 0.9619774773656434297 ) ) ;
#3569=AXIS2_PLACEMENT_3D ( 'NONE', #12145, #18308, #25137 ) ;
#3570=UNCERTAINTY_MEASURE_WITH_UNIT (LENGTH_MEASURE( 1.000000000000000082E-05 ), #19633, 'distance_accuracy_value', 'NONE');
#3571=CARTESIAN_POINT ( 'NONE',  ( -1.806356699219227036, 116.4728921782852922, 0.003255218499346703570 ) ) ;
#3572=EDGE_LOOP ( 'NONE', ( #40114, #32875, #2213, #32243, #14251, #31489, #20934, #6341, #3416 ) ) ;
#3573=CARTESIAN_POINT ( 'NONE',  ( -5.594070761475127718, 120.8783406922565860, -0.6737976942813748149 ) ) ;
#3574=CARTESIAN_POINT ( 'NONE',  ( 5.498428541007762682, -14.58429751298133326, 3.325033752563948841 ) ) ;
#3575=CARTESIAN_POINT ( 'NONE',  ( -4.509850150708960115, 121.0527503406816123, -0.3565835012282696503 ) ) ;
#3576=CARTESIAN_POINT ( 'NONE',  ( 3.392078256862109953, -14.39927144874259035, 5.014931565121842461 ) ) ;
#3578=CARTESIAN_POINT ( 'NONE',  ( 16.86029543505349082, 155.2078297922403465, 0.3599557924993779801 ) ) ;
#3579=ADVANCED_FACE ( 'NONE', ( #22593 ), #26229, .F. ) ;
#3581=CARTESIAN_POINT ( 'NONE',  ( -1.178223178616622402, 14.53665720681882689, 4.476207649055042204 ) ) ;
#3582=CARTESIAN_POINT ( 'NONE',  ( -15.56076557482332490, 120.7233670659379214, -0.3109411287488704767 ) ) ;
#3584=CIRCLE ( 'NONE', #2914, 3.683000000000001162 ) ;
#3585=CARTESIAN_POINT ( 'NONE',  ( 2.928857528687646372, 107.6124775248579937, 4.448914392086990688 ) ) ;
#3586=CARTESIAN_POINT ( 'NONE',  ( -7.018365211845482676, 121.6248220782754146, 0.4451966353337011295 ) ) ;
#3587=CARTESIAN_POINT ( 'NONE',  ( 0.7325351754718939512, 15.47086736126800766, -4.571311019245588803 ) ) ;
#3588=CARTESIAN_POINT ( 'NONE',  ( 22.34249146463927715, 149.5981344557702641, 1.749037778780574426 ) ) ;
#3590=CARTESIAN_POINT ( 'NONE',  ( -5.078986093043185157, 68.92746620154572668, -0.1014902294541231847 ) ) ;
#3591=CARTESIAN_POINT ( 'NONE',  ( 9.409928955097466741, 157.3305555497073271, -1.526371511294253303 ) ) ;
#3592=CARTESIAN_POINT ( 'NONE',  ( -0.5832499861179958334, 10.72304255322087307, 4.598074068532726599 ) ) ;
#3593=CARTESIAN_POINT ( 'NONE',  ( -21.67644226493410287, 136.7703657609320658, -1.576579429902727814 ) ) ;
#3595=CARTESIAN_POINT ( 'NONE',  ( -6.058098509843230950, 155.3491655920357459, 0.2313079102920782559 ) ) ;
#3596=CARTESIAN_POINT ( 'NONE',  ( 4.583978111877545558, -14.49189839317011064, 4.572462404262108038 ) ) ;
#3600=CARTESIAN_POINT ( 'NONE',  ( 0.4661379286530221155, 118.8635629087341954, 0.6143748731645415351 ) ) ;
#3601=CARTESIAN_POINT ( 'NONE',  ( 3.223859242259402791, 50.63946620154572997, -1.416295642791934650 ) ) ;
#3602=DIRECTION ( 'NONE',  ( -0.9998004120163608288, 0.000000000000000000, -0.01997839162482749342 ) ) ;
#3603=CARTESIAN_POINT ( 'NONE',  ( -22.76023949468089214, 146.4845460041848355, 0.7370798038890575832 ) ) ;
#3604=CARTESIAN_POINT ( 'NONE',  ( 4.144591825430580911, 15.01708852069707945, -7.363685156706923252 ) ) ;
#3605=AXIS2_PLACEMENT_3D ( 'NONE', #20595, #33624, #40021 ) ;
#3606=CARTESIAN_POINT ( 'NONE',  ( 5.826550815406353223, 117.0573985505404693, -0.1859578237674346934 ) ) ;
#3610=CARTESIAN_POINT ( 'NONE',  ( 1.880425555005761362, -15.05705604436505318, 5.673589828627330967 ) ) ;
#3612=CARTESIAN_POINT ( 'NONE',  ( -4.757346424997288103, 117.3993836135861386, -1.207075064218979810 ) ) ;
#3613=CARTESIAN_POINT ( 'NONE',  ( -4.408801154305764136, 118.1814785907497480, 0.3997980591957170371 ) ) ;
#3617=CARTESIAN_POINT ( 'NONE',  ( -1.984596792730465076, 115.6909491485466646, -1.718749578237781073 ) ) ;
#3618=CARTESIAN_POINT ( 'NONE',  ( -6.126668539192166030, 119.5961181856799556, -1.251232543939694519 ) ) ;
#3619=CARTESIAN_POINT ( 'NONE',  ( -2.472230802051619936, 107.2388417251876547, -4.724420784806152795 ) ) ;
#3620=CARTESIAN_POINT ( 'NONE',  ( 4.495330299262407792, 118.0850605857251452, 0.7940255090980337105 ) ) ;
#3622=CARTESIAN_POINT ( 'NONE',  ( -12.48065534322216941, 152.0704867801853766, -1.458211671286261835 ) ) ;
#3623=AXIS2_PLACEMENT_3D ( 'NONE', #16863, #39673, #494 ) ;
#3624=CARTESIAN_POINT ( 'NONE',  ( -3.722927991306443918, 115.7030846131066397, -1.610849859475568024 ) ) ;
#3625=CARTESIAN_POINT ( 'NONE',  ( -0.7530120751189652850, 106.0529022055765296, 5.240410227246371733 ) ) ;
#3626=CARTESIAN_POINT ( 'NONE',  ( 7.588858076165080568, 124.2943531750336490, 0.1426133663090956294 ) ) ;
#3627=CARTESIAN_POINT ( 'NONE',  ( -17.23442203377900128, 146.5563353440282981, -2.056614067264090462 ) ) ;
#3630=CARTESIAN_POINT ( 'NONE',  ( 8.366466113708492358, 119.9145198431062340, -1.112176479753337333 ) ) ;
#3631=CARTESIAN_POINT ( 'NONE',  ( -12.80217232463537336, 133.7150629370494244, -0.1325446241630061361 ) ) ;
#3632=CARTESIAN_POINT ( 'NONE',  ( -1.504723661876595786, -8.552649586842417051, -4.374500482163298898 ) ) ;
#3633=CARTESIAN_POINT ( 'NONE',  ( 18.33253411489121731, 154.1536317137893661, 1.165609363665846665 ) ) ;
#3635=CARTESIAN_POINT ( 'NONE',  ( 3.347262984424072219, -14.85936863781750539, 0.1546827838429291613 ) ) ;
#3636=CARTESIAN_POINT ( 'NONE',  ( -4.214263934994832539, 119.2415290214368042, 0.8241011934941721018 ) ) ;
#3637=CARTESIAN_POINT ( 'NONE',  ( -0.5928395319016861453, 6.288998576159460008, -0.7801151024821093571 ) ) ;
#3638=CARTESIAN_POINT ( 'NONE',  ( -15.04006788896557012, 156.1474796653986630, -0.8176042244810638460 ) ) ;
#3639=VECTOR ( 'NONE', #14630, 1000.000000000000000 ) ;
#3640=CARTESIAN_POINT ( 'NONE',  ( -0.7776641127062334791, -6.825634839940509124, -0.5883101582535473772 ) ) ;
#3642=VERTEX_POINT ( 'NONE', #39026 ) ;
#3644=CARTESIAN_POINT ( 'NONE',  ( 5.349033702192260264, 117.2069880336854197, 0.8964318704791016668 ) ) ;
#3645=CARTESIAN_POINT ( 'NONE',  ( -7.748985956666807340, 122.1869765257964673, 0.4223483383238799682 ) ) ;
#3646=CARTESIAN_POINT ( 'NONE',  ( 4.218352450475082449, -13.04292013931325478, 2.887648331721151873 ) ) ;
#3647=CARTESIAN_POINT ( 'NONE',  ( 16.48900842742850870, 139.9843038322558186, -1.489460148179643673 ) ) ;
#3648=CARTESIAN_POINT ( 'NONE',  ( -19.73710541150947506, 148.2167131080949787, -2.515028838702476399 ) ) ;
#3649=CARTESIAN_POINT ( 'NONE',  ( 3.177488185987922709, -14.13217061847354472, 2.003775387181677026 ) ) ;
#3650=CARTESIAN_POINT ( 'NONE',  ( -4.679832524073478162, 32.47693947602098063, 1.143146696348500413 ) ) ;
#3651=CARTESIAN_POINT ( 'NONE',  ( 9.679874449561324923, 124.8500477395539576, 0.02572261534930073840 ) ) ;
#3654=CARTESIAN_POINT ( 'NONE',  ( -6.437058721807690810E-14, 62.83146620154573014, 4.519164521849267879E-29 ) ) ;
#3658=CARTESIAN_POINT ( 'NONE',  ( 0.001319893060084358647, 116.4580521601689185, -0.06605284600166361209 ) ) ;
#3660=VECTOR ( 'NONE', #1051, 1000.000000000000227 ) ;
#3661=CARTESIAN_POINT ( 'NONE',  ( -3.987655724683881076, 118.7629491485398319, 0.9447994846549702119 ) ) ;
#3663=CARTESIAN_POINT ( 'NONE',  ( 2.424293868422599640, 38.64141628508733817, -1.187741880963723462 ) ) ;
#3664=CARTESIAN_POINT ( 'NONE',  ( 19.67869083727173773, 136.1149058410947532, 2.266608711299010093 ) ) ;
#3665=CARTESIAN_POINT ( 'NONE',  ( 4.453423564604278795, 13.74662854910535792, -1.294644163995742225 ) ) ;
#3666=CARTESIAN_POINT ( 'NONE',  ( 8.431793794909870243, 26.85621209503467455, -0.1224882448600171925 ) ) ;
#3667=B_SPLINE_CURVE_WITH_KNOTS ( 'NONE', 3,
 ( #24949, #27932, #41367, #5172 ),
 .UNSPECIFIED., .F., .F.,
 ( 4, 4 ),
 ( 0.6010210485952584003, 1.000000000000000000 ),
 .UNSPECIFIED. ) ;
#3668=CARTESIAN_POINT ( 'NONE',  ( 5.512878477348360562, 117.1944552775264583, -0.5780071930592981522 ) ) ;
#3669=CARTESIAN_POINT ( 'NONE',  ( -2.033169340630109012, 122.5452913651401587, -0.2335185838714207707 ) ) ;
#3671=CARTESIAN_POINT ( 'NONE',  ( -3.542958166033328027, 109.5877865956762918, -3.777787172267635274 ) ) ;
#3672=CARTESIAN_POINT ( 'NONE',  ( 1.647191011186240006, 104.6144662015456817, 4.545328325604496733 ) ) ;
#3673=CARTESIAN_POINT ( 'NONE',  ( -3.957843245660688680, 22.95775517496322848, 2.395914033147342970 ) ) ;
#3674=CARTESIAN_POINT ( 'NONE',  ( -3.466430381603673005, 50.13146620154573441, -1.339521056010489319 ) ) ;
#3675=CARTESIAN_POINT ( 'NONE',  ( -1.569967658166198543, 117.3993836205931700, -1.461707296722773775 ) ) ;
#3676=CARTESIAN_POINT ( 'NONE',  ( 3.394644278243977187, -13.41358914320520057, 2.304069835958892032 ) ) ;
#3679=CARTESIAN_POINT ( 'NONE',  ( 0.9959059386942926695, 109.5507526474568607, -3.831187545969640951 ) ) ;
#3680=CARTESIAN_POINT ( 'NONE',  ( -22.91546036685028653, 149.1739538623130272, 0.5130544771887699529 ) ) ;
#3682=ORIENTED_EDGE ( 'NONE', *, *, #26631, .F. ) ;
#3685=CARTESIAN_POINT ( 'NONE',  ( -6.442660433036017764, 29.32943145771791649, -0.01012415147099491285 ) ) ;
#3687=CARTESIAN_POINT ( 'NONE',  ( 5.680254533628135150, -15.02324869320220735, 2.089386157847644920 ) ) ;
#3688=CARTESIAN_POINT ( 'NONE',  ( -19.92238394974720350, 148.9191654756151024, 1.700261758071553775 ) ) ;
#3689=CARTESIAN_POINT ( 'NONE',  ( 5.164160201466080125, 158.7070047875298826, -1.240540739692758576 ) ) ;
#3690=CARTESIAN_POINT ( 'NONE',  ( -4.288638401707804526, -7.253218809911426312, -1.756103832032595680 ) ) ;
#3692=ORIENTED_EDGE ( 'NONE', *, *, #11857, .T. ) ;
#3694=CARTESIAN_POINT ( 'NONE',  ( 0.6121664022496100532, 114.3327162918516962, 2.181662845130500905 ) ) ;
#3695=CARTESIAN_POINT ( 'NONE',  ( -4.799585727462988949, 117.4716807894286461, 1.004530280717990331 ) ) ;
#3697=CARTESIAN_POINT ( 'NONE',  ( -16.13547353508420557, 149.3012944676311804, 1.369731486774125262 ) ) ;
#3699=CARTESIAN_POINT ( 'NONE',  ( 11.06957317628260995, 122.5598569164413334, -1.209814958810230712 ) ) ;
#3700=CARTESIAN_POINT ( 'NONE',  ( -4.930931983215480763, 118.2512723699127832, -1.012396356527061503 ) ) ;
#3703=VERTEX_POINT ( 'NONE', #271 ) ;
#3704=CARTESIAN_POINT ( 'NONE',  ( 4.364081292726229577, 118.1821858711944486, -0.4478306246164636129 ) ) ;
#3705=CARTESIAN_POINT ( 'NONE',  ( 9.401300499464312566, 153.8930958044198576, -0.5598851911991605812 ) ) ;
#3706=ORIENTED_EDGE ( 'NONE', *, *, #30257, .F. ) ;
#3707=CARTESIAN_POINT ( 'NONE',  ( -17.26689864452599110, 148.5513402141484391, -2.222558794446809927 ) ) ;
#3708=CARTESIAN_POINT ( 'NONE',  ( 3.228916932056940858, -14.69740968606676823, 0.4668019137946345376 ) ) ;
#3710=CARTESIAN_POINT ( 'NONE',  ( -3.174366308152011484, 63.84746620154572838, -0.06343139340882730792 ) ) ;
#3713=CARTESIAN_POINT ( 'NONE',  ( 4.577905313181523717, 13.52175256873284326, -0.6256056815880789435 ) ) ;
#3714=CARTESIAN_POINT ( 'NONE',  ( 1.409834354326054529, 119.9358631726476574, 0.5453972335014175554 ) ) ;
#3715=CARTESIAN_POINT ( 'NONE',  ( -3.148634455474564220, 30.89457961443325118, -0.4672107454865900844 ) ) ;
#3717=CARTESIAN_POINT ( 'NONE',  ( -2.707926769430928804, 11.08828375386998033, -3.745406074561137721 ) ) ;
#3718=CARTESIAN_POINT ( 'NONE',  ( 8.575029486087361263, 123.3373102669514765, 0.3234659723512186003 ) ) ;
#3721=CARTESIAN_POINT ( 'NONE',  ( -2.182332153769093619, 116.1897970674740748, -0.04360822100399409929 ) ) ;
#3722=DIRECTION ( 'NONE',  ( -0.003125310045706406609, -0.9876883405951376593, 0.1564032425800100379 ) ) ;
#3727=DIRECTION ( 'NONE',  ( -0.9998004120163608288, 0.000000000000000000, -0.01997839162482747608 ) ) ;
#3732=CARTESIAN_POINT ( 'NONE',  ( -15.55989727259158606, 120.8127473925414108, -0.08007127899889533718 ) ) ;
#3735=CARTESIAN_POINT ( 'NONE',  ( 7.793436386033940622, 122.5978578380440638, 0.02760177019608184637 ) ) ;
#3736=ORIENTED_EDGE ( 'NONE', *, *, #24238, .T. ) ;
#3738=CARTESIAN_POINT ( 'NONE',  ( -11.84172335778374041, 151.9972573545839225, -0.3576891575424541725 ) ) ;
#3739=CARTESIAN_POINT ( 'NONE',  ( 2.113928706699719218, -15.46215275738946282, 5.949113654003534535 ) ) ;
#3740=CARTESIAN_POINT ( 'NONE',  ( -17.54996479678720434, 128.5781302034472162, 1.330722490425295668 ) ) ;
#3741=CARTESIAN_POINT ( 'NONE',  ( 4.037907715354051241, 27.70556447992504445, -2.267523456217593214 ) ) ;
#3742=CARTESIAN_POINT ( 'NONE',  ( 18.54376275836449040, 154.1690995007799927, 0.7937872377295740467 ) ) ;
#3743=CARTESIAN_POINT ( 'NONE',  ( 2.189939624171645338, -15.48487759952872622, 5.886065356993532838 ) ) ;
#3745=CARTESIAN_POINT ( 'NONE',  ( -0.2812775050834619428, 1.806455656379289287, -0.9370761103187740249 ) ) ;
#3746=CARTESIAN_POINT ( 'NONE',  ( -23.33231982438486085, 148.8574307740229585, -0.6970557703302364683 ) ) ;
#3747=DIRECTION ( 'NONE',  ( 4.017660918040594346E-17, -1.000000000000000000, -2.376309959284834438E-19 ) ) ;
#3751=CARTESIAN_POINT ( 'NONE',  ( 8.785006194573600879, 117.7265864523129721, 0.3950309330525467733 ) ) ;
#3752=VERTEX_POINT ( 'NONE', #33485 ) ;
#3753=CARTESIAN_POINT ( 'NONE',  ( -10.76835564758012609, 122.7614441063800399, 1.139041423164458333 ) ) ;
#3755=CARTESIAN_POINT ( 'NONE',  ( 21.29267830536744555, 148.0064520001644723, 2.314741142932118745 ) ) ;
#3756=CARTESIAN_POINT ( 'NONE',  ( 17.46034360794347506, 151.5007859583534753, -1.733980983366192330 ) ) ;
#3757=CARTESIAN_POINT ( 'NONE',  ( 0.9605196170170531289, 3.153480984720312019, -0.1630338022177024171 ) ) ;
#3758=CARTESIAN_POINT ( 'NONE',  ( -17.24095835932504528, 153.8449085212272678, -1.984086636893841460 ) ) ;
#3759=CARTESIAN_POINT ( 'NONE',  ( 4.614683254511476207, 118.0411034907158978, -0.6410491579301769161 ) ) ;
#3760=CARTESIAN_POINT ( 'NONE',  ( 4.497658079232150996, 104.6144662015457527, 1.758835774424003962 ) ) ;
#3761=CARTESIAN_POINT ( 'NONE',  ( 1.473868052710539889, 120.2326517397585377, -0.4086940711265544257 ) ) ;
#3762=CARTESIAN_POINT ( 'NONE',  ( -8.770618086121094947, 123.6813396614493712, -0.1752578222716850431 ) ) ;
#3764=CARTESIAN_POINT ( 'NONE',  ( -13.63191106101887407, 125.8243951943327517, -1.964466803988918153 ) ) ;
#3765=CARTESIAN_POINT ( 'NONE',  ( 4.930802857217395641, -15.55747185075553851, 2.516589264972601825 ) ) ;
#3766=CARTESIAN_POINT ( 'NONE',  ( -4.801647862234980302, 117.4032733357427105, 1.015449305853463491 ) ) ;
#3767=CARTESIAN_POINT ( 'NONE',  ( -4.553380338773690639, 118.0136081097811029, -0.8849348180924038187 ) ) ;
#3771=CARTESIAN_POINT ( 'NONE',  ( 18.05261769607643174, 144.6555253171603397, 2.402359405240795276 ) ) ;
#3774=CARTESIAN_POINT ( 'NONE',  ( 10.83330528665002923, 157.8980211815716928, 0.2164752214609689529 ) ) ;
#3775=CARTESIAN_POINT ( 'NONE',  ( -4.148164184366740059, 118.0988315448752530, 0.6394906134413954613 ) ) ;
#3777=CARTESIAN_POINT ( 'NONE',  ( -1.087716277807347254, 29.42523365726748708, -8.383486966309323662 ) ) ;
#3778=CARTESIAN_POINT ( 'NONE',  ( 15.98475566209939913, 146.3393691146323761, 1.048177900600803625 ) ) ;
#3779=CARTESIAN_POINT ( 'NONE',  ( 20.72298665840521892, 132.2482564273973935, -0.5730191400310227223 ) ) ;
#3780=CARTESIAN_POINT ( 'NONE',  ( 4.788875734160475517, 117.8399135866531680, 0.9345395952325853406 ) ) ;
#3782=CARTESIAN_POINT ( 'NONE',  ( -1.421603664355800101, 159.6054662015457666, -0.02840702444251828190 ) ) ;
#3785=CARTESIAN_POINT ( 'NONE',  ( -6.683353917540686417, 120.8996509036314819, -1.027146486415592586 ) ) ;
#3786=CARTESIAN_POINT ( 'NONE',  ( 22.53527615164647457, 150.7831677823004952, 0.4503084484864791626 ) ) ;
#3787=CARTESIAN_POINT ( 'NONE',  ( -8.161245858290207877, 122.8283871457973362, -0.4521822771171595812 ) ) ;
#3788=CARTESIAN_POINT ( 'NONE',  ( 4.240324834746892257, -11.68880992198167945, 0.6883502328505933798 ) ) ;
#3789=CARTESIAN_POINT ( 'NONE',  ( -22.35542929045595528, 148.9358926463403918, 0.9984386947210763807 ) ) ;
#3791=CARTESIAN_POINT ( 'NONE',  ( 18.62929286701944420, 154.1293031355326946, 0.4449488992651827735 ) ) ;
#3793=CARTESIAN_POINT ( 'NONE',  ( -3.416230376366909294, -5.529048218071860532, 3.121479803864907865 ) ) ;
#3794=CARTESIAN_POINT ( 'NONE',  ( 4.783155644945383145, 105.1214970594926257, 2.386995739668397398 ) ) ;
#3795=CARTESIAN_POINT ( 'NONE',  ( 4.646169936107913401, 117.9325745699973282, -0.7782960047779410306 ) ) ;
#3796=CARTESIAN_POINT ( 'NONE',  ( -4.948559212928203443, 119.0884032316885737, 0.9007675068828924214 ) ) ;
#3797=CARTESIAN_POINT ( 'NONE',  ( 4.623297697159335584, 3.588818502778304609, 0.3943307014320480697 ) ) ;
#3798=CARTESIAN_POINT ( 'NONE',  ( 14.34385702226353132, 155.9958976045614349, 1.592240502911361766 ) ) ;
#3799=CARTESIAN_POINT ( 'NONE',  ( 15.38000172824457046, 147.8312228276848543, 0.3073290369001837052 ) ) ;
#3800=DIRECTION ( 'NONE',  ( -0.01997839162482737546, -1.040247600000940825E-18, 0.9998004120163610509 ) ) ;
#3801=CARTESIAN_POINT ( 'NONE',  ( 2.213227627077498205, 118.1205262787358663, -0.6644466414026560797 ) ) ;
#3802=CARTESIAN_POINT ( 'NONE',  ( -3.522755225739859775, -9.592572062075928940, 3.019445982675781348 ) ) ;
#3803=CARTESIAN_POINT ( 'NONE',  ( -22.71086789718629717, 148.5871737753741115, -1.637050152828072092 ) ) ;
#3805=CARTESIAN_POINT ( 'NONE',  ( -9.163388821854908883, 124.2347608867413413, -0.1831063163140473349 ) ) ;
#3807=CARTESIAN_POINT ( 'NONE',  ( -1.609565093910659161, 156.2658572007470639, 0.2453390865415089050 ) ) ;
#3808=CARTESIAN_POINT ( 'NONE',  ( 4.956269154958684808, -14.57630274377035029, 4.209183869072664841 ) ) ;
#3809=( BOUNDED_CURVE ( )  B_SPLINE_CURVE ( 3, ( #22267, #35717, #35930, #19501 ),
 .UNSPECIFIED., .F., .T. ) 
 B_SPLINE_CURVE_WITH_KNOTS ( ( 4, 4 ),
 ( 0.2498838476046065238, 0.5001855759278981406 ),
 .UNSPECIFIED. ) 
 CURVE ( )  GEOMETRIC_REPRESENTATION_ITEM ( )  RATIONAL_B_SPLINE_CURVE ( ( 0.5000007283237750677, 0.4995979372591229373, 0.6662643611511979147, 1.000000000000000000 ) ) 
 REPRESENTATION_ITEM ( '' )  );
#3811=CARTESIAN_POINT ( 'NONE',  ( -1.039005592983597070, 105.9869000721054846, -5.237171080062087647 ) ) ;
#3814=CARTESIAN_POINT ( 'NONE',  ( 10.78248307147193685, 155.9024031350590462, 2.169211330499416057 ) ) ;
#3816=CARTESIAN_POINT ( 'NONE',  ( 9.118174893680169646, 124.1671967267183589, 0.1822028344259500054 ) ) ;
#3817=CARTESIAN_POINT ( 'NONE',  ( -0.01443894962468954962, 159.4760848062415732, 0.7225840825867287931 ) ) ;
#3819=CARTESIAN_POINT ( 'NONE',  ( 0.2322036383927537639, 20.64316925235604216, 8.417729739967510838 ) ) ;
#3820=CARTESIAN_POINT ( 'NONE',  ( 4.409042980950512280, 120.6578283891288379, 0.6218799582752132515 ) ) ;
#3822=CARTESIAN_POINT ( 'NONE',  ( 22.54544115201711563, 150.6069110094195764, -0.1392563518891843932 ) ) ;
#3823=DIRECTION ( 'NONE',  ( 0.9998004120163610509, 5.205824365704083805E-17, 0.01997839162482749689 ) ) ;
#3826=CARTESIAN_POINT ( 'NONE',  ( 1.424304860752266144, 106.0679449480461329, -5.142703936578335799 ) ) ;
#3829=CARTESIAN_POINT ( 'NONE',  ( -4.547855832773509910, 118.1104907970478024, 0.5056323322026208267 ) ) ;
#3834=CARTESIAN_POINT ( 'NONE',  ( -6.041464496458629263, 119.4136938840325399, -1.263443438576810518 ) ) ;
#3835=CARTESIAN_POINT ( 'NONE',  ( -7.424629525399851104, 123.6670498955208473, -0.1830506623709852454 ) ) ;
#3836=CARTESIAN_POINT ( 'NONE',  ( 4.534800580971761974, 118.0743626807513209, 0.7973481318499234805 ) ) ;
#3837=CARTESIAN_POINT ( 'NONE',  ( -16.08743688339782807, 147.0533492130506943, -1.289446542218032565 ) ) ;
#3840=CARTESIAN_POINT ( 'NONE',  ( 0.1065646865914872399, 105.8844662015456777, -5.332932678536313809 ) ) ;
#3841=CARTESIAN_POINT ( 'NONE',  ( -16.56824576912640623, 144.0643239018434940, -1.930375849691871704 ) ) ;
#3842=CARTESIAN_POINT ( 'NONE',  ( 5.256943553860875973, 116.0444662015457027, 1.293952898321280021 ) ) ;
#3843=CARTESIAN_POINT ( 'NONE',  ( -0.001640166039862459230, 159.6041700698465036, 0.08208061555506504514 ) ) ;
#3845=CARTESIAN_POINT ( 'NONE',  ( 8.026787933082662363, 121.5445110286361086, -0.8405406253987532939 ) ) ;
#3846=CARTESIAN_POINT ( 'NONE',  ( -2.856921527171903286, 121.0288202834496190, 0.01139528386683224398 ) ) ;
#3847=CARTESIAN_POINT ( 'NONE',  ( -4.627450822138572839, 2.892058097378844117, -0.1328416527703782657 ) ) ;
#3848=CARTESIAN_POINT ( 'NONE',  ( 21.51154278844947854, 151.3526640061693342, 1.384567357891493211 ) ) ;
#3850=CARTESIAN_POINT ( 'NONE',  ( 3.375754317642519098, -15.02680299829225952, 2.760009546110721246 ) ) ;
#3851=CARTESIAN_POINT ( 'NONE',  ( -16.64003893621130459, 151.1890201267100906, 1.733044620493700894 ) ) ;
#3852=CARTESIAN_POINT ( 'NONE',  ( 0.9680108232324700079, 2.729151709021603978, 0.1071397942825247085 ) ) ;
#3853=CARTESIAN_POINT ( 'NONE',  ( -21.11962238282699644, 132.3956117394162106, -1.087766252141818102 ) ) ;
#3854=CARTESIAN_POINT ( 'NONE',  ( -0.6834205802178441314, -7.050398998296187436, -0.6963091382628930903 ) ) ;
#3857=CARTESIAN_POINT ( 'NONE',  ( 3.394470486402062281, 108.6891572770382624, 4.119616105806038320 ) ) ;
#3859=CARTESIAN_POINT ( 'NONE',  ( -8.995803412248951858, 123.1852847016406685, 0.4677080646552715382 ) ) ;
#3860=CARTESIAN_POINT ( 'NONE',  ( 1.930977371672661924, -15.05712096081325591, 5.742647184725750087 ) ) ;
#3861=CARTESIAN_POINT ( 'NONE',  ( 0.009513407573606913470, 119.7614543879625586, -0.4760898169610157660 ) ) ;
#3862=CARTESIAN_POINT ( 'NONE',  ( -3.256054338613478816, 118.9727644790723531, -0.9029027703446362851 ) ) ;
#3863=CARTESIAN_POINT ( 'NONE',  ( 3.260699289283686131, 104.6144662015457669, 3.570726652107954813 ) ) ;
#3864=CARTESIAN_POINT ( 'NONE',  ( 3.187143392547471255, -14.52651900126690876, 3.212499789951002604 ) ) ;
#3865=CARTESIAN_POINT ( 'NONE',  ( -6.313817790419506082, 30.81489375714620138, 1.175039937232976062 ) ) ;
#3866=CARTESIAN_POINT ( 'NONE',  ( 15.40211203110474969, 147.8297367799732456, 0.07919316026241145223 ) ) ;
#3867=ORIENTED_EDGE ( 'NONE', *, *, #24853, .T. ) ;
#3868=CARTESIAN_POINT ( 'NONE',  ( -2.633132161630451940, 107.2195770060342284, 4.632131451278267420 ) ) ;
#3873=CIRCLE ( 'NONE', #28321, 5.588000000000006295 ) ;
#3875=CARTESIAN_POINT ( 'NONE',  ( 3.739900805225205183, 116.6566025657135413, -0.03821340562556407167 ) ) ;
#3876=CARTESIAN_POINT ( 'NONE',  ( -5.793465281260614219, 118.4310156723767307, 0.4331262667984490666 ) ) ;
#3877=CARTESIAN_POINT ( 'NONE',  ( -0.01822531903872333034, 118.1564764849152738, 0.9120692297075591037 ) ) ;
#3879=CARTESIAN_POINT ( 'NONE',  ( -4.061900884676539647, 32.22309257017796824, 0.8408443696299722214 ) ) ;
#3880=CARTESIAN_POINT ( 'NONE',  ( 1.134298505455532569, 158.7113841514841681, 1.516915449716996989 ) ) ;
#3881=CARTESIAN_POINT ( 'NONE',  ( 2.838909340336904563, 21.51804255560577772, 3.663749385350952181 ) ) ;
#3882=CARTESIAN_POINT ( 'NONE',  ( 2.985612812371020386, 19.08565862607713370, -7.890306666671915714 ) ) ;
#3883=CARTESIAN_POINT ( 'NONE',  ( 8.618216296094656670, 118.6576028950189823, -0.8123356437107368544 ) ) ;
#3884=CARTESIAN_POINT ( 'NONE',  ( -1.682799138809848882, 120.1914007830323214, -0.5335993566373051777 ) ) ;
#3885=FACE_OUTER_BOUND ( 'NONE', #35928, .T. ) ;
#3886=CARTESIAN_POINT ( 'NONE',  ( -0.9117815773467171647, 106.1653671795302074, -5.214745729516177875 ) ) ;
#3887=CARTESIAN_POINT ( 'NONE',  ( -3.698849545476382783, 105.1233800755782255, 3.857623938754290105 ) ) ;
#3889=CARTESIAN_POINT ( 'NONE',  ( -2.614655561276646889, 23.60746518810343986, 3.812863311767609620 ) ) ;
#3892=CARTESIAN_POINT ( 'NONE',  ( 3.243601939617143159, -13.81697766888033385, 2.329280267808830907 ) ) ;
#3893=CARTESIAN_POINT ( 'NONE',  ( 1.702772465368721511, 120.1914007830323214, -0.4659475787731966467 ) ) ;
#3894=CARTESIAN_POINT ( 'NONE',  ( -1.955870317219649213, 116.9162416783649689, 0.3393494064863860626 ) ) ;
#3895=CARTESIAN_POINT ( 'NONE',  ( 5.008289758173663841, 117.3984635900009295, -0.7758770640922041384 ) ) ;
#3899=VERTEX_POINT ( 'NONE', #37293 ) ;
#3901=CARTESIAN_POINT ( 'NONE',  ( 4.914263517198875775, -15.39432152949170352, 0.3857354017804055513 ) ) ;
#3902=CARTESIAN_POINT ( 'NONE',  ( -20.30545318303849456, 145.4934252350392114, 1.680122328351855820 ) ) ;
#3903=CARTESIAN_POINT ( 'NONE',  ( 14.28818831795921440, 121.8555783441548073, -1.022170725131337665 ) ) ;
#3904=CARTESIAN_POINT ( 'NONE',  ( 0.4343283552818534288, -9.202337043772711667, -4.603842121470758997 ) ) ;
#3905=CARTESIAN_POINT ( 'NONE',  ( 3.174366308151880922, 104.6144662015457243, 0.06343139340882769650 ) ) ;
#3909=CARTESIAN_POINT ( 'NONE',  ( 0.7127221660106257684, 117.6736730875354766, 1.182500608623780813 ) ) ;
#3910=CARTESIAN_POINT ( 'NONE',  ( 4.856046737116808565, 117.4074955614782851, 1.171143430823223808 ) ) ;
#3911=CARTESIAN_POINT ( 'NONE',  ( -16.84814155439281080, 148.3581316477378493, 1.364645798843572955 ) ) ;
#3913=CARTESIAN_POINT ( 'NONE',  ( 18.09605103972940654, 148.5173242358814321, -1.660853775707743285 ) ) ;
#3914=CARTESIAN_POINT ( 'NONE',  ( -7.739031927415108036, 119.2688035297948659, -1.343379870322972236 ) ) ;
#3917=CARTESIAN_POINT ( 'NONE',  ( 4.447414120290241080, 118.1635491156278448, -0.4464743765249865604 ) ) ;
#3918=CARTESIAN_POINT ( 'NONE',  ( 9.519849589794681322, 124.0643708016488063, -0.3285928725474104861 ) ) ;
#3920=CARTESIAN_POINT ( 'NONE',  ( 3.259035188333455846, -14.62011735832338744, 2.262668647611313588 ) ) ;
#3921=DIRECTION ( 'NONE',  ( 0.9998004120163608288, 0.000000000000000000, 0.01997839162482760791 ) ) ;
#3923=DIRECTION ( 'NONE',  ( 0.01997839162482749689, 1.040247600000945640E-18, -0.9998004120163610509 ) ) ;
#3925=CARTESIAN_POINT ( 'NONE',  ( -2.426139246716550346, 10.07336736126799437, 3.943011612146583023 ) ) ;
#3926=CARTESIAN_POINT ( 'NONE',  ( 2.024284171598446314, 156.9412006218898057, 1.489060257140892407 ) ) ;
#3927=CARTESIAN_POINT ( 'NONE',  ( -2.880736501481948153, 31.22451072257329585, 0.7774695130801791976 ) ) ;
#3928=CARTESIAN_POINT ( 'NONE',  ( -0.9211762648548540433, 10.43857344512876040, -4.529598961101950927 ) ) ;
#3929=CARTESIAN_POINT ( 'NONE',  ( 15.74517894787269867, 145.7063497038720925, 0.5455200375299577020 ) ) ;
#3933=CARTESIAN_POINT ( 'NONE',  ( 2.175103472038542929, 116.2667018202340898, -0.1328812213640993556 ) ) ;
#3934=CARTESIAN_POINT ( 'NONE',  ( 10.83330528665002923, 157.8980211815716928, 0.2164752214609689529 ) ) ;
#3943=CARTESIAN_POINT ( 'NONE',  ( -1.881116149107413760, 116.6503132507590124, 0.1904188032791132856 ) ) ;
#3946=CARTESIAN_POINT ( 'NONE',  ( -6.980741664752802222, 121.9496248960778786, -0.1878529747284405360 ) ) ;
#3949=CARTESIAN_POINT ( 'NONE',  ( -3.750075860242207071, 121.0949217282140182, -0.1016972523499029696 ) ) ;
#3950=CARTESIAN_POINT ( 'NONE',  ( 6.004855586296256931, -14.40561964533282335, 2.074926179989267094 ) ) ;
#3951=CARTESIAN_POINT ( 'NONE',  ( -9.525696296010787378, 157.4068808874136209, 1.471446521238429561 ) ) ;
#3952=CARTESIAN_POINT ( 'NONE',  ( 4.496586626007489151, 27.28078351817337222, -1.068494511273165193 ) ) ;
#3953=CARTESIAN_POINT ( 'NONE',  ( 0.9228193675733716850, 116.5712332538976455, 0.1866785551396779874 ) ) ;
#3955=CARTESIAN_POINT ( 'NONE',  ( 2.121138329832424230, -15.54773473020022756, 5.902882008759894106 ) ) ;
#3956=CARTESIAN_POINT ( 'NONE',  ( -0.9950013725589796909, 29.65466048987409309, -4.513790593961638287 ) ) ;
#3957=CARTESIAN_POINT ( 'NONE',  ( -0.006055453635351584415, 1.369653838947524349, -0.9756124606672940125 ) ) ;
#3958=CARTESIAN_POINT ( 'NONE',  ( -23.06561215160527567, 149.8841935741895384, -0.7910477959972078699 ) ) ;
#3959=CARTESIAN_POINT ( 'NONE',  ( -6.654617103318593247E-14, 104.6144662015457243, 1.534725424433578570E-31 ) ) ;
#3960=CARTESIAN_POINT ( 'NONE',  ( 4.962376320764782633, 117.4036719250501335, 1.029954939118661095 ) ) ;
#3962=CARTESIAN_POINT ( 'NONE',  ( -5.552612348590429292, 116.8946703468410675, 0.3109655406019063983 ) ) ;
#3963=CARTESIAN_POINT ( 'NONE',  ( -11.09075344257221474, 123.0430266451958232, 1.157373622111985467 ) ) ;
#3965=CARTESIAN_POINT ( 'NONE',  ( 21.29237892510558439, 148.2102652567764380, 2.313897094871049553 ) ) ;
#3966=CARTESIAN_POINT ( 'NONE',  ( 13.91587783890476793, 154.2684476645699760, -1.737230819368874135 ) ) ;
#3967=CARTESIAN_POINT ( 'NONE',  ( 0.5230511744754561265, -14.76557578359995837, -0.8217837604668620788 ) ) ;
#3968=CARTESIAN_POINT ( 'NONE',  ( -14.13476661394985179, 155.9232964860746620, -1.730687652093988449 ) ) ;
#3969=CARTESIAN_POINT ( 'NONE',  ( 4.725354652796848853, 117.9692588958336046, -0.6261570487145760033 ) ) ;
#3970=CARTESIAN_POINT ( 'NONE',  ( 4.833220906894529101, 105.1215657678094573, 2.265336830653343458 ) ) ;
#3972=CARTESIAN_POINT ( 'NONE',  ( 9.956456675072738349, 154.0333045108203009, -1.106646445589350103 ) ) ;
#3973=CARTESIAN_POINT ( 'NONE',  ( -7.045353508903627215, 122.0728772437221323, -0.1110369332536842307 ) ) ;
#3975=CARTESIAN_POINT ( 'NONE',  ( -5.029336563147013273, 119.5555251685854330, -1.067692183578045073 ) ) ;
#3976=CARTESIAN_POINT ( 'NONE',  ( 4.883858777703569132, -15.45279978240890451, 0.9440085714135780792 ) ) ;
#3978=CARTESIAN_POINT ( 'NONE',  ( -4.695219223534134123, 117.9582964687422617, -0.8613277202148715839 ) ) ;
#3981=B_SPLINE_CURVE_WITH_KNOTS ( 'NONE', 1,
 ( #39860, #10656 ),
 .UNSPECIFIED., .F., .F.,
 ( 2, 2 ),
 ( 0.000000000000000000, 1.000000000000000000 ),
 .UNSPECIFIED. ) ;
#3982=CARTESIAN_POINT ( 'NONE',  ( 4.065926199369043204, 118.2429491485453354, 0.3080910687088499467 ) ) ;
#3983=CARTESIAN_POINT ( 'NONE',  ( 0.8917109795614704959, 157.3234082283764792, 1.558336142952464032 ) ) ;
#3984=CARTESIAN_POINT ( 'NONE',  ( -6.517733866319332394E-14, 78.32546620154573702, 2.848871684924056535E-29 ) ) ;
#3985=CARTESIAN_POINT ( 'NONE',  ( 2.736438259132175865, 116.5290148844309357, 0.04129949523434448683 ) ) ;
#3986=CARTESIAN_POINT ( 'NONE',  ( 7.891363246779867779, 17.78247237326412034, -2.951631208061117562 ) ) ;
#3987=CARTESIAN_POINT ( 'NONE',  ( 0.6142257358152197755, 120.7813932625355307, 0.2072529566615757823 ) ) ;
#3989=CARTESIAN_POINT ( 'NONE',  ( 22.27630879610695658, 150.1947564971097222, -0.7286472789443331211 ) ) ;
#3991=ORIENTED_EDGE ( 'NONE', *, *, #32280, .F. ) ;
#3992=DIRECTION ( 'NONE',  ( -0.9998004120163608288, 0.000000000000000000, -0.01997839162482749342 ) ) ;
#3993=CARTESIAN_POINT ( 'NONE',  ( -22.69744207413532067, 137.3157656003441787, -0.3098006952201957098 ) ) ;
#3996=CARTESIAN_POINT ( 'NONE',  ( -5.716351369186457809, 121.0728109688119787, -0.5777774213903609235 ) ) ;
#3998=CARTESIAN_POINT ( 'NONE',  ( -7.609804580617608671, 122.3831840716419066, -0.4262428003126359499 ) ) ;
#3999=CARTESIAN_POINT ( 'NONE',  ( 3.811713748825880543, -11.77916328849872052, 0.6977653098966205558 ) ) ;
#4000=CARTESIAN_POINT ( 'NONE',  ( -22.14298845881056366, 148.3267584643486146, 1.148356825654135660 ) ) ;
#4002=CARTESIAN_POINT ( 'NONE',  ( 23.33940156856670711, 149.0646716566344026, 0.5435133253920599872 ) ) ;
#4004=CARTESIAN_POINT ( 'NONE',  ( -4.637963820743935983, -6.603494994175692412, 0.1710436084038768345 ) ) ;
#4006=CARTESIAN_POINT ( 'NONE',  ( 1.830559115875370457, 105.1242114329274671, 5.019440104649677714 ) ) ;
#4007=DIRECTION ( 'NONE',  ( -0.9998004120163608288, 0.000000000000000000, -0.01997839162482750383 ) ) ;
#4008=CARTESIAN_POINT ( 'NONE',  ( 3.174366308151880478, 101.6934662015457320, 0.06343139340882768262 ) ) ;
#4009=CARTESIAN_POINT ( 'NONE',  ( 4.462489588987306632, 118.6703996354438289, 1.056833130132613929 ) ) ;
#4010=EDGE_CURVE ( 'NONE', #19701, #34211, #29900, .T. ) ;
#4011=CARTESIAN_POINT ( 'NONE',  ( 3.857898856315107761, -6.768822978661375167, 2.551181839177400601 ) ) ;
#4012=CARTESIAN_POINT ( 'NONE',  ( 22.13959287704968304, 149.5167998366165989, 1.884152790553834889 ) ) ;
#4015=CARTESIAN_POINT ( 'NONE',  ( 20.98992760039521954, 147.8517002469272370, -1.565498118541299055 ) ) ;
#4016=CARTESIAN_POINT ( 'NONE',  ( -4.027482788729651375, -0.2968512080594384317, 2.264360808822050597 ) ) ;
#4017=CARTESIAN_POINT ( 'NONE',  ( -22.70140800483401833, 148.7873826295267747, -1.635989027091524939 ) ) ;
#4020=CARTESIAN_POINT ( 'NONE',  ( -15.72482880707722686, 147.2451778420852406, 0.1375710997406975333 ) ) ;
#4022=CARTESIAN_POINT ( 'NONE',  ( 5.611355841363750763, -14.32207541480874724, 3.167021961541031327 ) ) ;
#4025=CARTESIAN_POINT ( 'NONE',  ( 18.85674122909604833, 149.4003703399637288, 2.492295690319127122 ) ) ;
#4028=CARTESIAN_POINT ( 'NONE',  ( -1.339128788961420069, 159.4185946040361728, 0.8255809207588795662 ) ) ;
#4029=CARTESIAN_POINT ( 'NONE',  ( 4.614102091175348086, 5.327238342305563812, -7.074968232746598140 ) ) ;
#4030=CARTESIAN_POINT ( 'NONE',  ( 16.45678414710221205, 146.8700648836752691, 1.605370559133788122 ) ) ;
#4031=CARTESIAN_POINT ( 'NONE',  ( 5.842267051812621403, 117.1711376449269721, -0.3073735213368161689 ) ) ;
#4032=CARTESIAN_POINT ( 'NONE',  ( 3.009276887026297587, 50.13146620154573441, -1.210121013456480599 ) ) ;
#4035=CARTESIAN_POINT ( 'NONE',  ( 4.755545234561889600, 111.7581959907442268, -2.489084640299535245 ) ) ;
#4038=CARTESIAN_POINT ( 'NONE',  ( -4.515032206727305208, 118.1273750342149640, 0.5013739007068812592 ) ) ;
#4040=EDGE_CURVE ( 'NONE', #34334, #26787, #18292, .T. ) ;
#4041=ORIENTED_EDGE ( 'NONE', *, *, #28465, .F. ) ;
#4044=CARTESIAN_POINT ( 'NONE',  ( -6.117143830817480143, 119.5759206346389334, -1.252900237863971089 ) ) ;
#4046=CARTESIAN_POINT ( 'NONE',  ( -6.914225208283879098, 121.8192184429722005, -0.2944576502256238126 ) ) ;
#4047=CARTESIAN_POINT ( 'NONE',  ( 4.528603410297228571, 118.1085942879815036, 0.6812181296683174070 ) ) ;
#4048=CARTESIAN_POINT ( 'NONE',  ( -9.559621201325507300, 153.9312916436033447, -1.179784447169990758 ) ) ;
#4049=DIRECTION ( 'NONE',  ( -0.9998004120163608288, 0.000000000000000000, -0.01997839162482749342 ) ) ;
#4050=CARTESIAN_POINT ( 'NONE',  ( 1.584774673591883065, 118.1651004081050473, -0.7984633640959337697 ) ) ;
#4051=CARTESIAN_POINT ( 'NONE',  ( 7.694720906311244057, 124.7202454748262710, 0.1538800020430352300 ) ) ;
#4052=CARTESIAN_POINT ( 'NONE',  ( -5.120605266512877840, 120.5246234221128248, -0.8194923670329070653 ) ) ;
#4056=CARTESIAN_POINT ( 'NONE',  ( 8.798071512540863282, 117.6842349196870572, 0.1758064070670784795 ) ) ;
#4057=CARTESIAN_POINT ( 'NONE',  ( -5.939622480684505490, 155.4177107962312903, 0.03793785350558757236 ) ) ;
#4059=CARTESIAN_POINT ( 'NONE',  ( 4.611808778022512989, -11.57686662695173929, 0.3579861242195471194 ) ) ;
#4060=CARTESIAN_POINT ( 'NONE',  ( 3.829241263245279026, 116.9593488885201538, 0.4901781634895739370 ) ) ;
#4062=CARTESIAN_POINT ( 'NONE',  ( 2.709380901426776678, -15.26748983718428931, 4.527680251005613776 ) ) ;
#4063=CARTESIAN_POINT ( 'NONE',  ( -15.01676740740995797, 152.9649416503947634, 1.747251348416148042 ) ) ;
#4064=CARTESIAN_POINT ( 'NONE',  ( -0.2316695588195925026, 0.1309245165040176240, 0.9467938775014126396 ) ) ;
#4065=CARTESIAN_POINT ( 'NONE',  ( -23.06466230714223897, 149.5685596498530288, -1.055262110361126826 ) ) ;
#4067=CARTESIAN_POINT ( 'NONE',  ( 0.4358653558703468045, -2.730035452555519271, 0.8728101606764442355 ) ) ;
#4068=ORIENTED_EDGE ( 'NONE', *, *, #14121, .F. ) ;
#4070=CARTESIAN_POINT ( 'NONE',  ( 4.351830713014955165, 111.2795884869231173, 3.127581853150075197 ) ) ;
#4071=CARTESIAN_POINT ( 'NONE',  ( -9.867693216206411932, 124.1914461168675530, 0.5013480754756758362 ) ) ;
#4072=CARTESIAN_POINT ( 'NONE',  ( 3.920414950246539298, -14.18668476855415506, 4.724392046630619291 ) ) ;
#4073=CARTESIAN_POINT ( 'NONE',  ( 13.59099248324865883, 128.5255724691869830, -1.296117023882648933 ) ) ;
#4074=CARTESIAN_POINT ( 'NONE',  ( -12.00151653869066770, 122.4500365997666336, -1.784698555944021159 ) ) ;
#4076=CARTESIAN_POINT ( 'NONE',  ( 4.076263842723025554, 104.6144662015457527, 2.604289233363719980 ) ) ;
#4077=CARTESIAN_POINT ( 'NONE',  ( 2.660183686505937839, -13.21883649654037640, 0.1900507390742080804 ) ) ;
#4078=CARTESIAN_POINT ( 'NONE',  ( -4.761227440037233194, 117.5395613512557986, -1.175773913404245308 ) ) ;
#4079=B_SPLINE_CURVE_WITH_KNOTS ( 'NONE', 3,
 ( #8429, #21387, #28009, #27593, #5246, #17580, #41018, #11827, #24815, #27181, #24180, #20982, #1634, #34003, #4833, #30784, #40602, #18841, #41446, #31845, #38667, #22437, #28859, #19048, #35467, #31635, #28226, #21813, #34839, #38457, #6492, #41232, #6085, #6290, #22029, #15437, #9474, #19261, #19470, #35058, #15853, #38871, #41658, #5879, #25460, #12035, #32053, #9064, #2685, #12251, #15642, #2891, #28647, #25864, #18630, #22233, #32269, #2262, #12466, #8849, #28440, #12876, #3099, #5673, #2476, #25244, #38247, #9275, #35261, #41872, #42082, #12671, #25660, #16060, #15225, #29062, #9683, #22649, #35683, #25026, #38029, #19676, #9887, #23283, #30119, #13723, #23709, #26717, #32691, #3526, #121, #36320 ),
 .UNSPECIFIED., .F., .F.,
 ( 4, 2, 2, 2, 2, 2, 1, 1, 2, 2, 2, 2, 2, 2, 2, 2, 2, 1, 1, 2, 2, 2, 2, 1, 1, 2, 2, 2, 1, 2, 2, 1, 1, 2, 2, 2, 1, 1, 1, 2, 2, 2, 2, 2, 2, 2, 1, 1, 1, 1, 2, 2, 2, 4 ),
 ( 0.000000000000000000, 0.03124999999996325856, 0.04687499999994489130, 0.06249999999992653099, 0.09374999999988976873, 0.1093749999998713668, 0.1171874999998621797, 0.1210937499998576000, 0.1230468749998553379, 0.1249999999998530897, 0.1406249999998358813, 0.1484374999998272771, 0.1523437499998230027, 0.1562499999998187006, 0.1718749999998016864, 0.1874999999997846722, 0.2187499999997506162, 0.2343749999997334910, 0.2421874999997249422, 0.2460937499997206401, 0.2499999999997163935, 0.3124999999996500577, 0.3437499999996169175, 0.3593749999996002642, 0.3671874999995919375, 0.3710937499995877187, 0.3749999999995834998, 0.4062499999995490829, 0.4140624999995403122, 0.4160156249995382582, 0.4169921874995372035, 0.4179687499995361488, 0.4218749999995391464, 0.4374999999995509148, 0.4687499999995748956, 0.4843749999995868860, 0.4921874999995928257, 0.4960937499995958788, 0.4980468749995973221, 0.4990234374995980993, 0.4999999999995988764, 0.5624999999996533884, 0.5937499999996804778, 0.6093749999996941336, 0.6249999999997076783, 0.6874999999997625233, 0.7187499999997897238, 0.7343749999998032685, 0.7421874999998098188, 0.7460937499998131495, 0.7480468749998148148, 0.7499999999998164801, 0.8749999999999082956, 1.000000000000000000 ),
 .UNSPECIFIED. ) ;
#4080=CARTESIAN_POINT ( 'NONE',  ( 1.594039003485483441, 156.2604006213118453, -0.1692965565027964581 ) ) ;
#4083=CARTESIAN_POINT ( 'NONE',  ( -3.070716065586290622, 107.8343606798839573, 4.352802841326662175 ) ) ;
#4084=CARTESIAN_POINT ( 'NONE',  ( 1.808844889178175208, 106.7498038803831975, 4.947659371736781608 ) ) ;
#4085=CARTESIAN_POINT ( 'NONE',  ( 1.569820930545707149, 117.3993836205989680, 1.461711849568192889 ) ) ;
#4087=CARTESIAN_POINT ( 'NONE',  ( 20.69264154312380555, 152.5691845998198346, 0.2640292844866434230 ) ) ;
#4088=CARTESIAN_POINT ( 'NONE',  ( -1.586608521453102272, 106.2379067940291293, 5.113598281387616851 ) ) ;
#4089=CARTESIAN_POINT ( 'NONE',  ( 1.938612655782578242, -15.67376786758054052, 5.527897971745494132 ) ) ;
#4092=CARTESIAN_POINT ( 'NONE',  ( 20.26628159282160269, 149.4216517587604756, 2.427422966980313568 ) ) ;
#4094=CARTESIAN_POINT ( 'NONE',  ( 6.774419413954826830, 18.20997082500984376, -5.007560425318187569 ) ) ;
#4095=CARTESIAN_POINT ( 'NONE',  ( 2.286771429912684006, 117.0703292719262691, -0.5337017719177589159 ) ) ;
#4096=CARTESIAN_POINT ( 'NONE',  ( -0.02009831008155203366, 106.6745790697264056, -5.014625686322316866 ) ) ;
#4099=CARTESIAN_POINT ( 'NONE',  ( -4.383638697405572771, 105.1218378623483858, 3.059989124871295818 ) ) ;
#4100=CARTESIAN_POINT ( 'NONE',  ( 2.829288187452689396, 6.340478445469713620, 3.655570690059357197 ) ) ;
#4102=CARTESIAN_POINT ( 'NONE',  ( -4.832057687079985620, 118.5264896598256854, 0.7487645382029636254 ) ) ;
#4103=CARTESIAN_POINT ( 'NONE',  ( 1.848046085800040483, -15.12359198595263088, 5.521975501593071378 ) ) ;
#4104=CARTESIAN_POINT ( 'NONE',  ( 4.298926901474557916, 118.7880935209305591, -0.4986311761637901574 ) ) ;
#4105=CARTESIAN_POINT ( 'NONE',  ( -3.184986510633185830, 159.3937097445585778, 0.5650791069852594273 ) ) ;
#4107=CARTESIAN_POINT ( 'NONE',  ( 4.923031700297470614, 117.4076359181580216, -0.9493066511862697787 ) ) ;
#4110=CARTESIAN_POINT ( 'NONE',  ( -2.960856320778833872, 31.17411798999470918, 0.6378382452821288462 ) ) ;
#4111=CARTESIAN_POINT ( 'NONE',  ( 4.858843758304779215, -15.48047902945742749, 1.209346601706016378 ) ) ;
#4112=CARTESIAN_POINT ( 'NONE',  ( -12.87447296688135090, 155.3440856034525837, 1.681555337288024976 ) ) ;
#4114=CARTESIAN_POINT ( 'NONE',  ( -3.974385726840726107, -7.478117039488521023, -2.359557994316856533 ) ) ;
#4117=DIRECTION ( 'NONE',  ( 4.017660918040594346E-17, -1.000000000000000000, -2.376309959284834438E-19 ) ) ;
#4118=CARTESIAN_POINT ( 'NONE',  ( -0.06390210066022013191, 106.1446358501009826, 5.228158908302722452 ) ) ;
#4120=CARTESIAN_POINT ( 'NONE',  ( -5.149255372874281811, 120.5246234221128248, 0.6142761105479900285 ) ) ;
#4122=CARTESIAN_POINT ( 'NONE',  ( 0.03153862713803012863, 157.4657262375360176, -1.578321868909182246 ) ) ;
#4123=CARTESIAN_POINT ( 'NONE',  ( -4.699679879531093007, 158.1906701298835856, -1.765476639684187887 ) ) ;
#4126=CARTESIAN_POINT ( 'NONE',  ( 4.162481684639020685, 118.2393836468389594, -0.2285641109998220177 ) ) ;
#4127=CARTESIAN_POINT ( 'NONE',  ( 7.092669859378088582, 121.9239394581621809, -0.2697480494961534969 ) ) ;
#4129=CARTESIAN_POINT ( 'NONE',  ( 3.231433726605559276, -14.53588044659766254, 1.883291753459793716 ) ) ;
#4131=CARTESIAN_POINT ( 'NONE',  ( -6.507153519498132566E-14, 76.29346620154572634, 3.067795752821199360E-29 ) ) ;
#4133=CARTESIAN_POINT ( 'NONE',  ( 4.506137822554599381, 3.376467715207942533, 1.027655576270160243 ) ) ;
#4134=CARTESIAN_POINT ( 'NONE',  ( 10.79132569999976177, 123.6843197456346672, 1.443847663909934464 ) ) ;
#4135=CARTESIAN_POINT ( 'NONE',  ( -2.677528989280510086, 30.35663814294097307, 0.2735905739161426098 ) ) ;
#4136=CARTESIAN_POINT ( 'NONE',  ( -1.932895124392534303, 20.38400505531995321, -4.219463811995566083 ) ) ;
#4137=CARTESIAN_POINT ( 'NONE',  ( 15.65552799280926699, 147.2250547476223801, 0.5422809309331375616 ) ) ;
#4140=CARTESIAN_POINT ( 'NONE',  ( -8.792159704875166071, 117.7003605453419084, -0.3061736163580975334 ) ) ;
#4141=LINE ( 'NONE', #23480, #39367 ) ;
#4147=DIRECTION ( 'NONE',  ( -0.9998004120163609398, 0.000000000000000000, -0.01997839162482749689 ) ) ;
#4150=CARTESIAN_POINT ( 'NONE',  ( -16.05353943441306441, 121.3766923467913585, 0.004207837007976961835 ) ) ;
#4151=EDGE_LOOP ( 'NONE', ( #15825, #14704, #7546, #13311 ) ) ;
#4153=CARTESIAN_POINT ( 'NONE',  ( -6.060908664785462641, 121.4331619493032832, -0.1231561192607217164 ) ) ;
#4157=CARTESIAN_POINT ( 'NONE',  ( -14.67688973683561571, 148.8424012017631242, -0.4203365054377472543 ) ) ;
#4158=CARTESIAN_POINT ( 'NONE',  ( 3.642312988314884592, -15.20939988557298861, 5.384177138096517545 ) ) ;
#4159=CARTESIAN_POINT ( 'NONE',  ( -16.85638304633373252, 153.6818489539412553, 1.479736204719018122 ) ) ;
#4160=CARTESIAN_POINT ( 'NONE',  ( 0.4746723515649934888, 24.68197512780947278, 4.609222710213416896 ) ) ;
#4161=CARTESIAN_POINT ( 'NONE',  ( 15.47334368943519500, 120.8153160915142337, 0.6283931236857892566 ) ) ;
#4162=CARTESIAN_POINT ( 'NONE',  ( 2.249953683904569957, -15.41150387077881767, 5.858494404600263827 ) ) ;
#4163=CARTESIAN_POINT ( 'NONE',  ( 1.790774717077139089, 25.13178105314743860, 4.274281468382033822 ) ) ;
#4164=CARTESIAN_POINT ( 'NONE',  ( -0.7070771686734943495, -4.675651901196332005, 0.6724949525944122763 ) ) ;
#4165=CARTESIAN_POINT ( 'NONE',  ( -13.39999158873821195, 156.9487217736090940, -0.4592210153261409578 ) ) ;
#4166=DIRECTION ( 'NONE',  ( -5.206863593109713661E-17, 1.000000000000000000, -1.077750396879097183E-30 ) ) ;
#4167=CARTESIAN_POINT ( 'NONE',  ( 4.812227470261317919, 117.4055065471341237, 1.197252064078428990 ) ) ;
#4169=CARTESIAN_POINT ( 'NONE',  ( -8.791734470649634758, 117.7397621763150966, 0.07689045645447853405 ) ) ;
#4170=CARTESIAN_POINT ( 'NONE',  ( -9.495682976374393292, 155.1592096034013366, 1.579384785498887167 ) ) ;
#4172=CARTESIAN_POINT ( 'NONE',  ( 5.844449987888563847, 118.2031694463412634, 1.045635565433329583 ) ) ;
#4173=CARTESIAN_POINT ( 'NONE',  ( 16.79779972313707859, 131.5287050380659082, -1.642352026799754450 ) ) ;
#4174=CARTESIAN_POINT ( 'NONE',  ( -0.9740112296533943725, -11.51769927068266419, -0.01433540041261589619 ) ) ;
#4175=CARTESIAN_POINT ( 'NONE',  ( -3.973247942572257330, 117.7793252414215317, -0.8392447889045229203 ) ) ;
#4177=CARTESIAN_POINT ( 'NONE',  ( 4.832410959468069755, 104.6144662015479412, 2.264944922177924536 ) ) ;
#4178=CARTESIAN_POINT ( 'NONE',  ( 16.50777979357271263, 146.8700648836752691, -0.9466601202970253981 ) ) ;
#4181=CARTESIAN_POINT ( 'NONE',  ( -5.835067757121142229, 120.0568572605186546, -1.100767069290504718 ) ) ;
#4182=CARTESIAN_POINT ( 'NONE',  ( 5.161689517976459030, -15.45231451347503437, 1.550260198497607877 ) ) ;
#4184=CARTESIAN_POINT ( 'NONE',  ( -4.801770124281918406, 117.3993836135855133, 1.016061139389656587 ) ) ;
#4185=CARTESIAN_POINT ( 'NONE',  ( -4.708247763567237953, 117.9524266585390677, -0.8424022261019792346 ) ) ;
#4188=DIRECTION ( 'NONE',  ( -0.9998004120163608288, 0.000000000000000000, -0.01997839162482749342 ) ) ;
#4190=CARTESIAN_POINT ( 'NONE',  ( 13.11083847086517906, 125.9194590699508893, 1.866409529942264944 ) ) ;
#4191=FACE_OUTER_BOUND ( 'NONE', #25863, .T. ) ;
#4192=CIRCLE ( 'NONE', #8264, 0.5080000000000002292 ) ;
#4193=CARTESIAN_POINT ( 'NONE',  ( 16.30362368704338394, 121.4145675751456253, 0.3085868453551565693 ) ) ;
#4194=CARTESIAN_POINT ( 'NONE',  ( -3.339872139798120809, 10.66371166075841437, -7.743087711851694088 ) ) ;
#4195=CARTESIAN_POINT ( 'NONE',  ( 7.064669522240043520, 121.9740017686541194, 0.4795729057185784128 ) ) ;
#4196=CARTESIAN_POINT ( 'NONE',  ( 1.996658253870856381, 117.0827246868714013, -0.4092875891974778746 ) ) ;
#4199=CARTESIAN_POINT ( 'NONE',  ( -15.69674027099064340, 120.8333755831694702, -0.2629491152481263083 ) ) ;
#4201=CARTESIAN_POINT ( 'NONE',  ( -8.075719299406451057, 121.0962356888206983, -1.310857334151179998 ) ) ;
#4203=ORIENTED_EDGE ( 'NONE', *, *, #12647, .F. ) ;
#4204=DIRECTION ( 'NONE',  ( 0.9998004120163608288, 0.000000000000000000, 0.01997839162482749342 ) ) ;
#4205=CARTESIAN_POINT ( 'NONE',  ( -15.32065199451917437, 143.5038931315047535, -0.7650733020788531569 ) ) ;
#4206=CARTESIAN_POINT ( 'NONE',  ( 4.513689648792266418, -13.57929909251434708, 3.776549439516510898 ) ) ;
#4207=CARTESIAN_POINT ( 'NONE',  ( -14.39601482975368008, 155.9958976045614349, 1.017949466214369325 ) ) ;
#4210=CARTESIAN_POINT ( 'NONE',  ( 1.814945173922627442, 116.4909138135563040, 0.1082358691141157847 ) ) ;
#4211=EDGE_CURVE ( 'NONE', #1598, #40883, #9091, .T. ) ;
#4213=CARTESIAN_POINT ( 'NONE',  ( 0.4343283552818534288, -9.202337043772711667, -4.603842121470758997 ) ) ;
#4215=CARTESIAN_POINT ( 'NONE',  ( -23.29064488658028864, 149.3519930085110161, -0.4911336289882582418 ) ) ;
#4219=CARTESIAN_POINT ( 'NONE',  ( 6.579380666976237357, 119.9434534851795462, 1.241007387725648892 ) ) ;
#4220=CARTESIAN_POINT ( 'NONE',  ( -0.4757704999385121702, -3.320450887815510121, -4.596079559024887295 ) ) ;
#4221=CARTESIAN_POINT ( 'NONE',  ( 4.857111322523725683, 117.4312795728108227, 0.7492135168955068592 ) ) ;
#4224=CARTESIAN_POINT ( 'NONE',  ( 20.96550312372659519, 148.3608207065297222, -1.563628808460498565 ) ) ;
#4226=CARTESIAN_POINT ( 'NONE',  ( 0.9983407785579379023, 1.652274601622760741, 4.518288805521794238 ) ) ;
#4227=CARTESIAN_POINT ( 'NONE',  ( -20.32146383345317275, 132.1502320877631007, -1.598207211936853334 ) ) ;
#4229=CARTESIAN_POINT ( 'NONE',  ( -0.6357087519303221690, 120.9405031987692212, 0.07870476970620013391 ) ) ;
#4230=CARTESIAN_POINT ( 'NONE',  ( 3.642312988314884592, -15.20939988557298861, 5.384177138096517545 ) ) ;
#4232=CARTESIAN_POINT ( 'NONE',  ( -4.258558535336168127, 112.0482830817686590, -2.856570678809109864 ) ) ;
#4233=VERTEX_POINT ( 'NONE', #16590 ) ;
#4234=CARTESIAN_POINT ( 'NONE',  ( 4.389113801267265025, 157.7533977378147654, 1.847790720561485633 ) ) ;
#4236=DIRECTION ( 'NONE',  ( 4.017660918040594346E-17, -1.000000000000000000, -2.376309959284834438E-19 ) ) ;
#4238=CARTESIAN_POINT ( 'NONE',  ( -1.044861395164040196, 117.1967307433898640, 0.4172573962433457906 ) ) ;
#4239=CARTESIAN_POINT ( 'NONE',  ( 2.011605530963595623, 11.37297026005182587, 8.215081034461865883 ) ) ;
#4241=CARTESIAN_POINT ( 'NONE',  ( 4.434842451389386930, 120.7762672505206041, 0.5587804529453967994 ) ) ;
#4243=CARTESIAN_POINT ( 'NONE',  ( 16.81386451639889756, 122.6968688451475771, -0.2091777910580984723 ) ) ;
#4247=CARTESIAN_POINT ( 'NONE',  ( 5.211496251797417933, 114.7155965213235334, -1.248716016855044852 ) ) ;
#4250=CARTESIAN_POINT ( 'NONE',  ( -4.525247824673359176, 118.1239580192302157, 0.4884167081844107416 ) ) ;
#4251=CARTESIAN_POINT ( 'NONE',  ( 2.790246638979534843, 107.7056043231319364, -4.425809011598065723 ) ) ;
#4255=CARTESIAN_POINT ( 'NONE',  ( -3.910367129306138168, 119.0646914673601060, -0.9244502089851933668 ) ) ;
#4256=CARTESIAN_POINT ( 'NONE',  ( -5.487604538598444215, 117.4962825466697467, -0.8290304003371101738 ) ) ;
#4257=CARTESIAN_POINT ( 'NONE',  ( 4.563865627759259525, 118.0172877987257891, 0.8781525176551367995 ) ) ;
#4258=CARTESIAN_POINT ( 'NONE',  ( -16.21957319403762554, 147.1082353761072454, -1.436993664011566807 ) ) ;
#4259=CARTESIAN_POINT ( 'NONE',  ( -0.5747239345953479850, 115.7029522507744446, -1.760667902980975086 ) ) ;
#4260=CARTESIAN_POINT ( 'NONE',  ( 0.5167143258659047111, 118.1651003012477048, -0.8730464947480743865 ) ) ;
#4261=CARTESIAN_POINT ( 'NONE',  ( 6.150459292200123329, 119.5049778551863682, -0.2724401547530461709 ) ) ;
#4262=CARTESIAN_POINT ( 'NONE',  ( -1.860601238663146084, 156.5995568990359175, -1.190227115183317474 ) ) ;
#4265=CARTESIAN_POINT ( 'NONE',  ( 8.378245210821091860, 119.8566484287663343, -1.107698278211587617 ) ) ;
#4266=FACE_OUTER_BOUND ( 'NONE', #1434, .T. ) ;
#4267=DIRECTION ( 'NONE',  ( 0.01997839162482749689, 1.040247600000945640E-18, -0.9998004120163610509 ) ) ;
#4268=CARTESIAN_POINT ( 'NONE',  ( 22.87667167544107372, 149.1739538623130272, 1.428090254611251719 ) ) ;
#4270=CARTESIAN_POINT ( 'NONE',  ( 2.484037338616324142, -15.29988040857715959, 4.804498879097399033 ) ) ;
#4271=CARTESIAN_POINT ( 'NONE',  ( -0.03153862713815891450, 157.4657262375360176, 1.578321868909182690 ) ) ;
#4272=CARTESIAN_POINT ( 'NONE',  ( -0.6899137464274212039, -3.097154947502566813, -0.6881565663087282347 ) ) ;
#4273=CARTESIAN_POINT ( 'NONE',  ( -23.25105004451273416, 146.7258352529021863, -1.066525923017375588 ) ) ;
#4275=CARTESIAN_POINT ( 'NONE',  ( -0.6564745402265276253, 25.61689014148909393, -0.7196881648562951650 ) ) ;
#4279=CARTESIAN_POINT ( 'NONE',  ( 5.553235467069344011, 117.9513286348681476, 0.7459228754688892460 ) ) ;
#4280=CARTESIAN_POINT ( 'NONE',  ( -4.488166000884779905, 120.9326014760084007, 0.2785428184686808417 ) ) ;
#4281=CARTESIAN_POINT ( 'NONE',  ( 4.246535372682106235, -13.89508586689386327, 4.277860383763752772 ) ) ;
#4282=CARTESIAN_POINT ( 'NONE',  ( 0.5497817020642016272, 119.7690751942239729, -0.4902208388216631740 ) ) ;
#4283=VERTEX_POINT ( 'NONE', #29598 ) ;
#4284=CARTESIAN_POINT ( 'NONE',  ( -4.155191945500765094, 119.0775769483117870, -1.003333751211267666 ) ) ;
#4285=CARTESIAN_POINT ( 'NONE',  ( 3.782349093391025541, 115.7032132741988590, 1.604868649576247641 ) ) ;
#4286=CARTESIAN_POINT ( 'NONE',  ( 3.187349844189338199, -14.38168857376666310, 3.261415970826748278 ) ) ;
#4287=CARTESIAN_POINT ( 'NONE',  ( -4.973571103949897321, 117.3993852294894822, -0.9750599430652935329 ) ) ;
#4288=CARTESIAN_POINT ( 'NONE',  ( 0.6357087519301933831, 120.9405031987692212, -0.07870476970620002288 ) ) ;
#4292=DIRECTION ( 'NONE',  ( -5.206863593109713661E-17, 1.000000000000000000, -1.077750396879097183E-30 ) ) ;
#4293=CARTESIAN_POINT ( 'NONE',  ( 4.730923123951279230, 114.9758604107125848, 1.767004453122148711 ) ) ;
#4296=CARTESIAN_POINT ( 'NONE',  ( 11.68775717287289773, 118.7263634577040676, 0.08842886322950112288 ) ) ;
#4299=CIRCLE ( 'NONE', #6998, 0.5080000000000002292 ) ;
#4301=CARTESIAN_POINT ( 'NONE',  ( 1.981454933681730202, -15.19403129753971271, 5.950052743700623203 ) ) ;
#4303=CARTESIAN_POINT ( 'NONE',  ( -2.317791448294674428, 31.60761946039689718, 1.124105164688197211 ) ) ;
#4304=CARTESIAN_POINT ( 'NONE',  ( 11.41340492329610434, 156.2473422840488979, 2.091747920666957139 ) ) ;
#4306=CARTESIAN_POINT ( 'NONE',  ( 8.244768260990875675, 16.90678017261275556, 1.796629206788997513 ) ) ;
#4307=CARTESIAN_POINT ( 'NONE',  ( 2.257211396292739369, 116.9995425702703926, -0.5090954389876272135 ) ) ;
#4308=CARTESIAN_POINT ( 'NONE',  ( -0.05023876518796718121, 106.0087397856094356, -5.285590276201098447 ) ) ;
#4310=CARTESIAN_POINT ( 'NONE',  ( -2.116593079194864835, 107.0582647851741882, -4.811305763238920008 ) ) ;
#4311=CARTESIAN_POINT ( 'NONE',  ( -5.284023326239697838, 104.6144662015015143, 0.8090710649176173774 ) ) ;
#4312=CIRCLE ( 'NONE', #28090, 0.5080000000000004512 ) ;
#4313=CARTESIAN_POINT ( 'NONE',  ( -2.406711483539481389, 4.503775517365914638, 3.979180414515509412 ) ) ;
#4315=CARTESIAN_POINT ( 'NONE',  ( -4.402866250424960270, 110.7917892407665050, -3.073120133393222098 ) ) ;
#4316=CARTESIAN_POINT ( 'NONE',  ( 3.089232434235547942, -13.39873834325867819, 1.372807258641574935 ) ) ;
#4317=CARTESIAN_POINT ( 'NONE',  ( 3.258544586981714453, 118.6786177306206014, -0.6136036933997358611 ) ) ;
#4318=CARTESIAN_POINT ( 'NONE',  ( -14.85158921512566721, 156.1223461918646933, 0.5575614454322269653 ) ) ;
#4320=CARTESIAN_POINT ( 'NONE',  ( -3.933769473788126803, 27.98561731294367050, 0.4889718192695882149 ) ) ;
#4322=ORIENTED_EDGE ( 'NONE', *, *, #35707, .F. ) ;
#4323=CARTESIAN_POINT ( 'NONE',  ( -4.779485535544667485, 104.6144662015457811, -0.6866870093448155243 ) ) ;
#4324=CARTESIAN_POINT ( 'NONE',  ( 3.609959606426583978, -15.77075149864894144, 4.467226954163184161 ) ) ;
#4325=CARTESIAN_POINT ( 'NONE',  ( -0.01133701039344079536, 118.4098733054621277, 0.5673503590873754110 ) ) ;
#4326=CARTESIAN_POINT ( 'NONE',  ( -0.4908008364610317309, 30.95719094559541418, -0.8433761395939078920 ) ) ;
#4327=ORIENTED_EDGE ( 'NONE', *, *, #19041, .F. ) ;
#4329=CARTESIAN_POINT ( 'NONE',  ( 0.8061429914041100542, 121.2007779179981384, 0.4207382890248005936 ) ) ;
#4330=CARTESIAN_POINT ( 'NONE',  ( -4.378102236263193170, 120.3584862571861436, 0.5730137456143139518 ) ) ;
#4332=CARTESIAN_POINT ( 'NONE',  ( 13.41341228195535784, 125.8771108566470502, -1.381187796596252459 ) ) ;
#4334=CARTESIAN_POINT ( 'NONE',  ( -5.842949248259256656, 118.5625182843610617, -1.130067629703343624 ) ) ;
#4337=CARTESIAN_POINT ( 'NONE',  ( 4.244956071762963745, 118.2245432729572627, -0.3158671543450045638 ) ) ;
#4340=CARTESIAN_POINT ( 'NONE',  ( 6.495086324197963279, 121.6155390319085683, -0.2579311815284315856 ) ) ;
#4343=CARTESIAN_POINT ( 'NONE',  ( 3.351397644842732948, -15.05179984492975542, 2.935234935891222641 ) ) ;
#4346=DIRECTION ( 'NONE',  ( -0.9998004120163608288, 0.000000000000000000, -0.01997839162482747608 ) ) ;
#4347=CARTESIAN_POINT ( 'NONE',  ( 0.7003524534433175353, 11.14785949628657669, 4.567531960304466843 ) ) ;
#4348=CARTESIAN_POINT ( 'NONE',  ( 11.67499187284218820, 153.3684197651487580, 1.838730530730912083 ) ) ;
#4349=CARTESIAN_POINT ( 'NONE',  ( -2.644846971204092068, 29.87439188816612656, 0.9757876149222759476 ) ) ;
#4351=CARTESIAN_POINT ( 'NONE',  ( -3.854280124997887746, 21.23357344512866973, -2.551540157904111261 ) ) ;
#4352=CARTESIAN_POINT ( 'NONE',  ( 9.006184665392719779, 123.9742709865185191, 0.2138692079817592906 ) ) ;
#4353=CARTESIAN_POINT ( 'NONE',  ( -3.372034046726852807, 108.0377789575252194, 4.123912905361212466 ) ) ;
#4355=CARTESIAN_POINT ( 'NONE',  ( 2.181655109597531617, 116.2239731218073615, -0.08111321244062891234 ) ) ;
#4357=AXIS2_PLACEMENT_3D ( 'NONE', #35062, #29914, #23077 ) ;
#4359=CARTESIAN_POINT ( 'NONE',  ( -0.1065207248106255222, 105.8844037013956125, 5.332933549509750293 ) ) ;
#4361=CARTESIAN_POINT ( 'NONE',  ( 4.698174212119619497, 9.136213905105968536, -7.004248122051734526 ) ) ;
#4366=CARTESIAN_POINT ( 'NONE',  ( -23.22389216488258867, 148.7951734159264561, 0.1326450332456386438 ) ) ;
#4367=EDGE_LOOP ( 'NONE', ( #33395, #40194, #15655, #31299 ) ) ;
#4369=CARTESIAN_POINT ( 'NONE',  ( 7.785084361432049072, 122.6279490200930695, 0.1367715089808400897 ) ) ;
#4372=CARTESIAN_POINT ( 'NONE',  ( -7.787205264484130751, 154.6472212274131550, -0.1983306932048339022 ) ) ;
#4373=CARTESIAN_POINT ( 'NONE',  ( 3.039728791924208195, -15.34324946256290723, 5.681930179901951483 ) ) ;
#4374=CARTESIAN_POINT ( 'NONE',  ( -7.892561109811933484, 118.8455990504009492, 0.9355921144164882630 ) ) ;
#4375=CARTESIAN_POINT ( 'NONE',  ( 2.332027132427558769, 25.33165720878049498, 3.998286310156994983 ) ) ;
#4376=AXIS2_PLACEMENT_3D ( 'NONE', #29722, #16931, #16718 ) ;
#4377=CARTESIAN_POINT ( 'NONE',  ( 6.906622810364680731, 117.2343425291504104, 0.3847307661620061325 ) ) ;
#4378=DIRECTION ( 'NONE',  ( -0.9998004120163609398, 0.000000000000000000, -0.01997839162482749689 ) ) ;
#4380=CARTESIAN_POINT ( 'NONE',  ( -0.09873697212813982438, -3.591044343564580910, 0.9733856795103970061 ) ) ;
#4381=CARTESIAN_POINT ( 'NONE',  ( -17.10498822929456253, 122.7072422303320707, -0.5849822763170866580 ) ) ;
#4384=EDGE_LOOP ( 'NONE', ( #34868, #37574, #30317, #22681 ) ) ;
#4385=CARTESIAN_POINT ( 'NONE',  ( 5.535474336661085459, 116.8955343539433045, 0.5335339445610354225 ) ) ;
#4386=CARTESIAN_POINT ( 'NONE',  ( -11.17823620286587349, 123.1247571232444784, 1.162497134544157928 ) ) ;
#4388=CARTESIAN_POINT ( 'NONE',  ( 5.844153588741368921, 118.3130479344264501, 1.074361049658993927 ) ) ;
#4389=CARTESIAN_POINT ( 'NONE',  ( 6.324931890614029051, 157.3995435888475072, -1.705594245970836420 ) ) ;
#4392=CARTESIAN_POINT ( 'NONE',  ( 0.2395577018624739096, -8.716993574909102094, 0.9436776969787653568 ) ) ;
#4393=CARTESIAN_POINT ( 'NONE',  ( -20.92851329017044293, 150.0074445146613584, -2.223361304733721955 ) ) ;
#4395=CARTESIAN_POINT ( 'NONE',  ( 5.344249437077539966, 105.1225132350959939, -0.1103424742704069983 ) ) ;
#4396=CARTESIAN_POINT ( 'NONE',  ( 5.880513813086725605, 121.0368588677253143, -0.5043468530174898268 ) ) ;
#4397=CARTESIAN_POINT ( 'NONE',  ( -9.104209967888042598, 153.9432936505793066, -0.1819237819739442652 ) ) ;
#4399=CARTESIAN_POINT ( 'NONE',  ( -18.01525633490682665, 148.5173242358814321, -2.382443637188214502 ) ) ;
#4400=CARTESIAN_POINT ( 'NONE',  ( 2.867278011408870064, -15.71882806570827640, 4.918777663456151750 ) ) ;
#4403=CARTESIAN_POINT ( 'NONE',  ( -4.392784016475978603, 118.1805867164427184, -0.5718452568440313133 ) ) ;
#4405=CARTESIAN_POINT ( 'NONE',  ( 4.109713352107567275, 118.2429491485453354, 0.3484632730576381343 ) ) ;
#4406=CARTESIAN_POINT ( 'NONE',  ( 17.50950237657569986, 148.8653046532945723, 2.321071487785774767 ) ) ;
#4408=CARTESIAN_POINT ( 'NONE',  ( 23.45208337669170007, 146.8499405026647651, 0.4686284387228156212 ) ) ;
#4409=CARTESIAN_POINT ( 'NONE',  ( -5.330747076954383878, 11.08732641057851964, -6.519097198751918398 ) ) ;
#4410=CARTESIAN_POINT ( 'NONE',  ( 15.89665129872314431, 146.6311637152522565, 0.9120559015848338502 ) ) ;
#4411=CARTESIAN_POINT ( 'NONE',  ( 0.01443894962456075334, 159.4760848062415732, -0.7225840825867285711 ) ) ;
#4413=CARTESIAN_POINT ( 'NONE',  ( 0.4699976290979421267, 115.6909491485452719, 1.765048339911096553 ) ) ;
#4415=CARTESIAN_POINT ( 'NONE',  ( -3.728135546147876678, 116.6403000632267464, 0.003128093132697681595 ) ) ;
#4418=CARTESIAN_POINT ( 'NONE',  ( -6.784182173561120521, 121.2536750021979799, -0.8970767929546700215 ) ) ;
#4421=CARTESIAN_POINT ( 'NONE',  ( -4.611806494114576438, 117.9324678712513759, -0.9633187536371230486 ) ) ;
#4422=CARTESIAN_POINT ( 'NONE',  ( -7.055095707297289742, 122.0164807696326790, -0.4009610655988181671 ) ) ;
#4423=CARTESIAN_POINT ( 'NONE',  ( 4.673344545167823938, -12.29283961637177214, 1.688191869143181201 ) ) ;
#4424=CARTESIAN_POINT ( 'NONE',  ( -3.058359628041920963, 159.2229145144301867, 0.9584471420995394064 ) ) ;
#4426=CARTESIAN_POINT ( 'NONE',  ( 23.44243449907606092, 146.8400249081559537, 0.5456528120549732908 ) ) ;
#4428=CARTESIAN_POINT ( 'NONE',  ( 4.440276399826426967, -1.430929408009915083, -1.287880193523989636 ) ) ;
#4429=CARTESIAN_POINT ( 'NONE',  ( -1.421603664355800101, 159.6054662015457666, -0.02840702444251828190 ) ) ;
#4431=DIRECTION ( 'NONE',  ( -4.017660918040594346E-17, 1.000000000000000000, 2.376309959284834438E-19 ) ) ;
#4433=CARTESIAN_POINT ( 'NONE',  ( 6.506277007714310834, 119.7857196899097119, 1.251456028858768610 ) ) ;
#4434=CARTESIAN_POINT ( 'NONE',  ( 2.459658384930404118, -7.418532284756778949, 3.912982838641719141 ) ) ;
#4435=CARTESIAN_POINT ( 'NONE',  ( 8.039955067132906308, 118.1206512225135015, 0.9611422114813542583 ) ) ;
#4437=CARTESIAN_POINT ( 'NONE',  ( 2.760819571866365951, 158.5977336698458089, -1.488126253378572184 ) ) ;
#4438=CARTESIAN_POINT ( 'NONE',  ( -1.146732334619779969, -3.095543821355960734, -4.488006035213349953 ) ) ;
#4439=CARTESIAN_POINT ( 'NONE',  ( -9.505306604063539666, 118.4542681464805298, -0.9615324788044602444 ) ) ;
#4441=CARTESIAN_POINT ( 'NONE',  ( -11.88810549871057454, 151.9737369308441544, 0.07145411264644083160 ) ) ;
#4442=CARTESIAN_POINT ( 'NONE',  ( 3.231152580208111580, -15.43077800403741584, 5.551260886339890455 ) ) ;
#4444=B_SPLINE_CURVE_WITH_KNOTS ( 'NONE', 3,
 ( #20833, #33231, #33857, #30644 ),
 .UNSPECIFIED., .F., .F.,
 ( 4, 4 ),
 ( 0.0001481480970339296298, 0.0005781902081302999060 ),
 .UNSPECIFIED. ) ;
#4445=CARTESIAN_POINT ( 'NONE',  ( -0.3864694276889155677, 117.9496048067635456, -1.408072416706073415 ) ) ;
#4446=ORIENTED_EDGE ( 'NONE', *, *, #7122, .T. ) ;
#4447=CARTESIAN_POINT ( 'NONE',  ( 12.16261443152838773, 122.9664497093790629, 1.797897170200384753 ) ) ;
#4450=CARTESIAN_POINT ( 'NONE',  ( -6.890728787288654900, 117.8105958006179890, 0.6119090536800846358 ) ) ;
#4451=CARTESIAN_POINT ( 'NONE',  ( -8.422295717417405569, 8.547183656736235591, -0.3195422701574849311 ) ) ;
#4452=CARTESIAN_POINT ( 'NONE',  ( 10.26858343235344861, 124.8461398015159745, 0.9314245544334066595 ) ) ;
#4455=CARTESIAN_POINT ( 'NONE',  ( 19.95587765737794683, 128.8226523212408949, -0.2284701554834993320 ) ) ;
#4461=CARTESIAN_POINT ( 'NONE',  ( -4.478724048142634473, 118.1112337407861048, 0.5787802498093359560 ) ) ;
#4462=CARTESIAN_POINT ( 'NONE',  ( 2.507403849662985795, 107.3040393085582167, -4.608059665216667433 ) ) ;
#4463=EDGE_LOOP ( 'NONE', ( #4041, #9223, #31844, #1633 ) ) ;
#4465=CARTESIAN_POINT ( 'NONE',  ( 6.052716142014698875, 119.3318794080258129, -1.025634881525736786 ) ) ;
#4466=CARTESIAN_POINT ( 'NONE',  ( -6.308735553862911516, 120.0717973201777511, -0.4535485300176084755 ) ) ;
#4467=CARTESIAN_POINT ( 'NONE',  ( 4.448170622692431131, 118.1283731037481601, 0.7238786398437021541 ) ) ;
#4468=CARTESIAN_POINT ( 'NONE',  ( -16.13275712328133693, 147.4171829256358137, -1.433441054525536051 ) ) ;
#4470=CARTESIAN_POINT ( 'NONE',  ( 2.810880042475876639, 117.3993815990320542, -1.303394573401737810 ) ) ;
#4471=CARTESIAN_POINT ( 'NONE',  ( -4.050807963365556930, 30.95410787014092335, -2.229501126309402448 ) ) ;
#4472=CARTESIAN_POINT ( 'NONE',  ( -9.375340687752244051, 122.9055586947561522, -1.148039706409768490 ) ) ;
#4475=CARTESIAN_POINT ( 'NONE',  ( 7.845668856638584820, 122.3864107020766596, -0.3364293281536828162 ) ) ;
#4476=CARTESIAN_POINT ( 'NONE',  ( -2.867346308344148831, 121.0282051601325577, 0.04542865946695314600 ) ) ;
#4477=CARTESIAN_POINT ( 'NONE',  ( 6.888626713468121388, 117.5201695557886410, 0.7016588733424087287 ) ) ;
#4479=CARTESIAN_POINT ( 'NONE',  ( 3.261251233531137217, -14.70027692227136917, 2.623613175195522285 ) ) ;
#4480=CARTESIAN_POINT ( 'NONE',  ( -11.63135762381498850, 122.7176759045101022, 1.263630383496116005 ) ) ;
#4481=CARTESIAN_POINT ( 'NONE',  ( 0.3740510792576948185, -8.494654975422754717, 0.8997923438783246297 ) ) ;
#4482=CARTESIAN_POINT ( 'NONE',  ( -3.185756255432687922, 159.4163042773305676, -0.6073767776667647889 ) ) ;
#4483=CARTESIAN_POINT ( 'NONE',  ( 0.2014313232957813393, -8.551994341567581870, -0.9548264729560895780 ) ) ;
#4486=CARTESIAN_POINT ( 'NONE',  ( 5.166232791441969674, 115.4535745449993982, 1.513138011745335909 ) ) ;
#4488=CARTESIAN_POINT ( 'NONE',  ( -0.004350076772786141965, 120.7058980590201429, 0.2176956299261768035 ) ) ;
#4489=CARTESIAN_POINT ( 'NONE',  ( 4.598504975971844821, -12.83055836278033901, 2.569316529143384820 ) ) ;
#4490=CARTESIAN_POINT ( 'NONE',  ( 15.09269357795375122, 134.7883251604851580, -1.349233830697067926 ) ) ;
#4491=ORIENTED_EDGE ( 'NONE', *, *, #2459, .F. ) ;
#4492=CARTESIAN_POINT ( 'NONE',  ( -12.25516334840921928, 122.6846661264431191, -1.808440497450061413 ) ) ;
#4494=CARTESIAN_POINT ( 'NONE',  ( 3.259676495098780880, -13.96886708669151034, 2.676229364769742158 ) ) ;
#4495=CARTESIAN_POINT ( 'NONE',  ( -4.830560651430104713, 117.5458123619130646, -1.145125986471454027 ) ) ;
#4496=CARTESIAN_POINT ( 'NONE',  ( 0.001786757842147936167, 120.9379535345006076, -0.08941666878750646752 ) ) ;
#4498=CARTESIAN_POINT ( 'NONE',  ( 12.41171712301729713, 121.5863879130357503, 1.717582910027388721 ) ) ;
#4499=CARTESIAN_POINT ( 'NONE',  ( 2.894556870215603261, 107.8345691432927254, 4.471910717343379638 ) ) ;
#4502=CARTESIAN_POINT ( 'NONE',  ( 17.17894352244471534, 122.7237354506536491, 0.1767255469942458634 ) ) ;
#4504=CARTESIAN_POINT ( 'NONE',  ( 2.153962292805264855, -15.42765719885048981, 5.938214566648465365 ) ) ;
#4508=CARTESIAN_POINT ( 'NONE',  ( -0.01081828485868089468, 118.1092738308834669, 0.5413912121690739321 ) ) ;
#4511=CARTESIAN_POINT ( 'NONE',  ( 7.891363246779867779, 17.78247237326412034, -2.951631208061117562 ) ) ;
#4512=CARTESIAN_POINT ( 'NONE',  ( -2.209815719917325616, 116.9321326171075413, -0.5724128154462628792 ) ) ;
#4513=CARTESIAN_POINT ( 'NONE',  ( -0.007549346801299551199, 106.0530876078258586, -5.266739608401566741 ) ) ;
#4516=CARTESIAN_POINT ( 'NONE',  ( -4.591961393772478139, 104.6144662015457811, 1.495199714113508049 ) ) ;
#4517=CARTESIAN_POINT ( 'NONE',  ( -0.2480930319908794535, 10.21371511114847053, -4.635561276548324727 ) ) ;
#4519=CARTESIAN_POINT ( 'NONE',  ( -2.293106875121391663, 106.8185943591930993, -4.820918091293040497 ) ) ;
#4520=CARTESIAN_POINT ( 'NONE',  ( 3.361318737587208005, -13.21634134694392415, 1.934622048986600840 ) ) ;
#4521=CARTESIAN_POINT ( 'NONE',  ( 3.175984444280615104, 117.6701293611589278, -0.8859276027576483692 ) ) ;
#4522=CARTESIAN_POINT ( 'NONE',  ( -5.005498311287589708, 28.16151697905833373, 1.324705785854183748 ) ) ;
#4525=CARTESIAN_POINT ( 'NONE',  ( -5.339850745321377268, 104.6144662015545066, -0.2412019823091631210 ) ) ;
#4526=CARTESIAN_POINT ( 'NONE',  ( 4.357275237516622823, -15.68314232965556343, 3.240836981083619062 ) ) ;
#4527=CARTESIAN_POINT ( 'NONE',  ( -18.20160870511337592, 135.6759721228443425, 1.705493676697015015 ) ) ;
#4528=CARTESIAN_POINT ( 'NONE',  ( -2.646443841375008432, -8.127818987380491578, -3.789199236247322133 ) ) ;
#4529=EDGE_CURVE ( 'NONE', #37319, #13530, #32097, .T. ) ;
#4533=CARTESIAN_POINT ( 'NONE',  ( 0.5479319383245284669, 107.0594419416054848, 4.854436055212457468 ) ) ;
#4535=CARTESIAN_POINT ( 'NONE',  ( -6.676265340062506048, 155.5185402614932570, 1.076558685701347384 ) ) ;
#4537=ADVANCED_FACE ( 'NONE', ( #1479 ), #22537, .T. ) ;
#4538=CARTESIAN_POINT ( 'NONE',  ( 3.394752741017162290, 119.5845705363850442, -0.6980748167159183115 ) ) ;
#4539=CARTESIAN_POINT ( 'NONE',  ( -13.38228307180527565, 122.0388263298542739, -1.742221313037096264 ) ) ;
#4542=ORIENTED_EDGE ( 'NONE', *, *, #6317, .F. ) ;
#4544=CARTESIAN_POINT ( 'NONE',  ( 4.313720991269348382, 118.2128926607351929, -0.3282634486935400164 ) ) ;
#4545=CARTESIAN_POINT ( 'NONE',  ( 14.56142545302297364, 139.1552669279217298, -0.4455586761712629906 ) ) ;
#4546=CIRCLE ( 'NONE', #29021, 0.5080000000000002292 ) ;
#4548=CARTESIAN_POINT ( 'NONE',  ( 3.235674727752381852, -14.79813088844142399, -0.3705354414145333730 ) ) ;
#4551=CARTESIAN_POINT ( 'NONE',  ( -3.469956624915944587, 9.623539240006554252, 3.074419811715999984 ) ) ;
#4552=CARTESIAN_POINT ( 'NONE',  ( 10.46581596931669722, 123.6668265419868646, 1.337773356492248711 ) ) ;
#4553=CARTESIAN_POINT ( 'NONE',  ( -1.659418339086100591, 31.10872648155390507, 2.656305225562720196 ) ) ;
#4554=CARTESIAN_POINT ( 'NONE',  ( -6.476067766296674577, 120.6581566633936404, 0.1355830077277816459 ) ) ;
#4555=CARTESIAN_POINT ( 'NONE',  ( -3.640175008984333882, 11.51306413504884318, -2.862805987297033727 ) ) ;
#4556=CARTESIAN_POINT ( 'NONE',  ( 9.106973723525536357, 153.9337724597031070, 0.2264262902970469726 ) ) ;
#4559=CARTESIAN_POINT ( 'NONE',  ( 5.556563611783038148, 116.7705472551883901, -0.1784112738407624132 ) ) ;
#4560=AXIS2_PLACEMENT_3D ( 'NONE', #32547, #22517, #9346 ) ;
#4563=CARTESIAN_POINT ( 'NONE',  ( -1.969665360195132608, 106.3924174363482678, 4.957232547992387772 ) ) ;
#4565=CARTESIAN_POINT ( 'NONE',  ( 8.428375251627102216, -1.854023157342211903, -0.5381045032988257537 ) ) ;
#4567=CARTESIAN_POINT ( 'NONE',  ( 3.174366308151881810, 78.32546620154573702, 0.06343139340882768262 ) ) ;
#4569=CARTESIAN_POINT ( 'NONE',  ( 0.002462548248794847305, 123.7646714092002611, -0.1232359841711013482 ) ) ;
#4570=CARTESIAN_POINT ( 'NONE',  ( -17.03046551078694293, 122.6950552906510694, -0.003367075177501115558 ) ) ;
#4574=CARTESIAN_POINT ( 'NONE',  ( 7.788904351887272703, 122.6147082451171713, 0.08148216547788392217 ) ) ;
#4578=CARTESIAN_POINT ( 'NONE',  ( -9.128616289401854544, 124.2274432543504332, -0.1375126816698667986 ) ) ;
#4579=CARTESIAN_POINT ( 'NONE',  ( 5.121635214396401459, -14.94813357331645243, 3.889196783476005059 ) ) ;
#4580=CARTESIAN_POINT ( 'NONE',  ( -4.850700283611360852, 158.3075559295907055, 1.526604748539100997 ) ) ;
#4581=CARTESIAN_POINT ( 'NONE',  ( 23.06197264524083579, 149.2510847660714148, 1.189562549516614665 ) ) ;
#4582=CARTESIAN_POINT ( 'NONE',  ( 1.339128788961291283, 159.4185946040361728, -0.8255809207588793441 ) ) ;
#4583=CARTESIAN_POINT ( 'NONE',  ( 0.9564925537785137211, 29.00497265395555857, -4.523030980006896407 ) ) ;
#4584=CARTESIAN_POINT ( 'NONE',  ( -18.63890302240357144, 125.2334963081946313, -0.6306532867605572079 ) ) ;
#4586=ORIENTED_EDGE ( 'NONE', *, *, #25846, .T. ) ;
#4588=CARTESIAN_POINT ( 'NONE',  ( -8.786270220348933790, 117.7728096769080679, 0.1425748814448410673 ) ) ;
#4589=CARTESIAN_POINT ( 'NONE',  ( -11.48915734413155398, 123.4929228318607386, 1.183242792625787576 ) ) ;
#4591=CARTESIAN_POINT ( 'NONE',  ( 9.920314382278954568, 120.7895603300898699, -1.200622369358214758 ) ) ;
#4592=CARTESIAN_POINT ( 'NONE',  ( -0.9396370176409497565, -11.09013235204027659, 0.2555656002325920051 ) ) ;
#4593=CARTESIAN_POINT ( 'NONE',  ( -2.121516847112316917, 117.7847241295267651, -0.6923378844829269907 ) ) ;
#4597=CARTESIAN_POINT ( 'NONE',  ( 5.339689988358259143, 105.1224923508004707, 0.2456598103791063359 ) ) ;
#4598=CARTESIAN_POINT ( 'NONE',  ( 0.006810764310266656518, 120.3493709785083183, -0.3408384964863780398 ) ) ;
#4599=CARTESIAN_POINT ( 'NONE',  ( -4.883848590450072358, 117.7607009110569862, 0.7127853619805604168 ) ) ;
#4601=CARTESIAN_POINT ( 'NONE',  ( -12.17039870458273043, 124.2599011343719155, -1.750469281869918792 ) ) ;
#4602=CARTESIAN_POINT ( 'NONE',  ( 2.341541575351651083, -15.74615379138004378, 5.495207524874286875 ) ) ;
#4604=DIRECTION ( 'NONE',  ( -4.017660918040594346E-17, 1.000000000000000000, 2.376309959284834438E-19 ) ) ;
#4605=CARTESIAN_POINT ( 'NONE',  ( -4.301501440665757237, 118.2120994191875099, -0.4958915692504695105 ) ) ;
#4608=CARTESIAN_POINT ( 'NONE',  ( 4.151427346349458425, 118.2394115087963371, 0.3932352160703678767 ) ) ;
#4609=CARTESIAN_POINT ( 'NONE',  ( 7.499533598998342043, 156.0351187175861867, 1.911400249181836264 ) ) ;
#4611=CARTESIAN_POINT ( 'NONE',  ( 16.18905205736044906, 121.2598130428683447, 0.3234957879086920451 ) ) ;
#4612=CARTESIAN_POINT ( 'NONE',  ( 8.244768260990875675, 16.90678017261275556, 1.796629206788997513 ) ) ;
#4613=CARTESIAN_POINT ( 'NONE',  ( 15.86281397719557162, 145.7686330500600036, 0.9137093302325698385 ) ) ;
#4614=CARTESIAN_POINT ( 'NONE',  ( 22.74864191258929935, 148.7873826295267747, -0.7277888646341178491 ) ) ;
#4616=CARTESIAN_POINT ( 'NONE',  ( 1.984410438080367767, 115.6909491485452719, 1.718756010027771230 ) ) ;
#4619=CARTESIAN_POINT ( 'NONE',  ( -22.73457742531305925, 137.3553536570635742, -0.3842032436244983695 ) ) ;
#4622=CARTESIAN_POINT ( 'NONE',  ( 7.870661077993043264, 122.2665614860925416, -0.4372302326949743523 ) ) ;
#4624=EDGE_LOOP ( 'NONE', ( #40451, #32785, #13588, #1752 ) ) ;
#4626=CARTESIAN_POINT ( 'NONE',  ( -15.32629999177647662, 148.0267799683202554, -0.7554886701871539323 ) ) ;
#4627=CARTESIAN_POINT ( 'NONE',  ( 3.665585082022325025, -14.37195162699216056, 4.995470683262428935 ) ) ;
#4628=CARTESIAN_POINT ( 'NONE',  ( -18.33177592110340370, 128.6097515361309149, 1.108544906447614720 ) ) ;
#4630=CARTESIAN_POINT ( 'NONE',  ( 18.61947985292891872, 154.1412379532633850, 0.5163013828871976241 ) ) ;
#4632=CARTESIAN_POINT ( 'NONE',  ( 1.968029828064305153, -3.592386099649644837, 4.203610184747879508 ) ) ;
#4633=CARTESIAN_POINT ( 'NONE',  ( -23.41829197008364360, 142.8308675865925181, -0.4933589455792335432 ) ) ;
#4637=CARTESIAN_POINT ( 'NONE',  ( -8.259150402946779934, 120.4370358907085716, 1.103988885813925958 ) ) ;
#4638=CARTESIAN_POINT ( 'NONE',  ( -0.6580430243309095539, -8.493043821084315326, 4.585212396833119541 ) ) ;
#4639=CARTESIAN_POINT ( 'NONE',  ( 7.493104803958843263, 158.4854300789945398, 1.293057490532128373 ) ) ;
#4641=CARTESIAN_POINT ( 'NONE',  ( 20.61281631175392093, 145.6130255286810495, -1.629730044589046578 ) ) ;
#4642=CARTESIAN_POINT ( 'NONE',  ( -4.227217475240903077, -11.31673468295422147, -1.889206449475258509 ) ) ;
#4643=CARTESIAN_POINT ( 'NONE',  ( -14.55652921886118811, 120.9595740141730289, -1.205336527378881195 ) ) ;
#4645=ORIENTED_EDGE ( 'NONE', *, *, #41983, .F. ) ;
#4647=CARTESIAN_POINT ( 'NONE',  ( -14.72002613302119656, 148.8393470518043955, 0.03138755845351943324 ) ) ;
#4648=CARTESIAN_POINT ( 'NONE',  ( 3.844517683078125803, -15.15487594273597161, 5.256808347261554104 ) ) ;
#4651=CARTESIAN_POINT ( 'NONE',  ( -5.167152973807009886, 114.8006916078235378, -1.419485145312306962 ) ) ;
#4653=CARTESIAN_POINT ( 'NONE',  ( 18.41451321397395802, 140.7300538122508726, 2.503121031321716483 ) ) ;
#4657=CARTESIAN_POINT ( 'NONE',  ( -16.19941014871838547, 155.1612327564137388, 0.8792224148362003389 ) ) ;
#4658=CARTESIAN_POINT ( 'NONE',  ( -1.148743315670426535, 1.199490873200159013, 8.378133985588048560 ) ) ;
#4659=CARTESIAN_POINT ( 'NONE',  ( 9.839787852217051878, 124.1914461168675530, 0.8951504484210820456 ) ) ;
#4661=CARTESIAN_POINT ( 'NONE',  ( 3.828842504638720445, 116.8938343318378088, -0.2916468201809273020 ) ) ;
#4664=CYLINDRICAL_SURFACE ( 'NONE', #23469, 5.588000000000006295 ) ;
#4667=CARTESIAN_POINT ( 'NONE',  ( -4.261598188410213872, 118.2248179704908182, 0.2974968183558716062 ) ) ;
#4668=CARTESIAN_POINT ( 'NONE',  ( 0.4041248631678749925, 105.7854974534225221, -5.326937287149722700 ) ) ;
#4669=ORIENTED_EDGE ( 'NONE', *, *, #32717, .T. ) ;
#4671=( BOUNDED_CURVE ( )  B_SPLINE_CURVE ( 3, ( #10896, #21100, #11739, #14292 ),
 .UNSPECIFIED., .F., .F. ) 
 B_SPLINE_CURVE_WITH_KNOTS ( ( 4, 4 ),
 ( 0.4253411113690419576, 0.4854033284062813647 ),
 .UNSPECIFIED. ) 
 CURVE ( )  GEOMETRIC_REPRESENTATION_ITEM ( )  RATIONAL_B_SPLINE_CURVE ( ( 0.7459560426888018903, 0.8021233807506140678, 0.8679106385868964324, 0.9433178161976487619 ) ) 
 REPRESENTATION_ITEM ( '' )  );
#4672=CARTESIAN_POINT ( 'NONE',  ( 6.222678124517797116, 119.6959855836942523, -0.9950030739501369847 ) ) ;
#4673=CARTESIAN_POINT ( 'NONE',  ( -5.045732318125732085, 114.3381464724725447, -1.964647476694348027 ) ) ;
#4674=CARTESIAN_POINT ( 'NONE',  ( 4.444225408500467545, 118.1580887933540254, 0.6034175566067268015 ) ) ;
#4675=CARTESIAN_POINT ( 'NONE',  ( -10.26858343235357829, 124.8461398015159745, -0.9314245544334064375 ) ) ;
#4677=CARTESIAN_POINT ( 'NONE',  ( 2.017207601148263141, 117.3993839199529390, -1.370552602517844276 ) ) ;
#4678=ORIENTED_EDGE ( 'NONE', *, *, #38324, .F. ) ;
#4679=CARTESIAN_POINT ( 'NONE',  ( 7.694663930960251363, 124.9344662015457317, 0.1537576976229973746 ) ) ;
#4680=CARTESIAN_POINT ( 'NONE',  ( -16.72040787068460332, 146.6545634508490821, -1.779279871595183637 ) ) ;
#4681=CARTESIAN_POINT ( 'NONE',  ( 5.336610043934060243, 104.6144662015457527, -0.07732958313162717479 ) ) ;
#4684=CARTESIAN_POINT ( 'NONE',  ( -6.518479118499084457, 121.7796321915099469, -0.01654800507752220151 ) ) ;
#4687=CARTESIAN_POINT ( 'NONE',  ( 3.843811238687773191, 117.0275016673472663, 0.5328274117395520593 ) ) ;
#4689=CARTESIAN_POINT ( 'NONE',  ( 3.205191379615736746, -14.47393913169138102, 3.051678166811226500 ) ) ;
#4690=CARTESIAN_POINT ( 'NONE',  ( 21.77700140173205057, 149.0176745010074342, -1.274060564799276651 ) ) ;
#4691=CARTESIAN_POINT ( 'NONE',  ( -4.236690124160904070, 119.4047208153655646, 0.8054972593864423436 ) ) ;
#4692=CIRCLE ( 'NONE', #7415, 3.175000000000001155 ) ;
#4693=CARTESIAN_POINT ( 'NONE',  ( -0.9740112296533943725, -11.51769927068266419, -0.01433540041261589619 ) ) ;
#4694=CARTESIAN_POINT ( 'NONE',  ( -22.53452490051039803, 150.3096427868838987, -1.298398843693310045 ) ) ;
#4695=CARTESIAN_POINT ( 'NONE',  ( 0.8462494346447723137, 11.68649857616015275, 0.4938625092760188795 ) ) ;
#4699=SHAPE_DEFINITION_REPRESENTATION ( #16363, #19076 ) ;
#4700=CARTESIAN_POINT ( 'NONE',  ( -3.658657848224285747, 120.8687762150871379, 0.2216941123881817910 ) ) ;
#4701=CARTESIAN_POINT ( 'NONE',  ( 4.980517673276738222, -11.70649569897110709, 0.6972323075040541829 ) ) ;
#4702=CARTESIAN_POINT ( 'NONE',  ( 0.008308630153144203057, 120.0570981805881559, -0.4157978282972240591 ) ) ;
#4706=CARTESIAN_POINT ( 'NONE',  ( 3.402052537932679588, -13.50846463298115196, 2.481730329246660371 ) ) ;
#4707=CARTESIAN_POINT ( 'NONE',  ( -4.881263862402589027, 117.4111615705287477, -1.144645852924967455 ) ) ;
#4708=CARTESIAN_POINT ( 'NONE',  ( 2.899431565053843141, 156.0891579660883508, -0.02704053119243710751 ) ) ;
#4710=CARTESIAN_POINT ( 'NONE',  ( -0.01111639779270567722, 118.2594330468507593, 0.5563100024230162033 ) ) ;
#4711=CARTESIAN_POINT ( 'NONE',  ( 4.304948217593230098, 111.0465000999332830, 3.212748056633830895 ) ) ;
#4714=CARTESIAN_POINT ( 'NONE',  ( 15.38960455597340626, 120.6961994932685798, 0.07768288530491213040 ) ) ;
#4718=CARTESIAN_POINT ( 'NONE',  ( 1.705331049022388745, -15.56171815815048021, 5.564216269553816652 ) ) ;
#4720=CARTESIAN_POINT ( 'NONE',  ( -4.881326591836633533, 117.7576924424856486, -0.7323402894751116499 ) ) ;
#4721=CARTESIAN_POINT ( 'NONE',  ( 2.184917017309174536, 118.1205262787358663, 0.7523320384000313776 ) ) ;
#4722=ORIENTED_EDGE ( 'NONE', *, *, #18578, .F. ) ;
#4723=CARTESIAN_POINT ( 'NONE',  ( 4.095665791538102063, 15.60827804425945331, 7.401523448874606892 ) ) ;
#4724=ADVANCED_FACE ( 'NONE', ( #34893 ), #31665, .F. ) ;
#4725=CARTESIAN_POINT ( 'NONE',  ( -5.507127385143735232, 117.8102281818942458, -1.047516571110145511 ) ) ;
#4726=CARTESIAN_POINT ( 'NONE',  ( -4.014846287426898641, 122.0441497943765370, -0.2789485273175660307 ) ) ;
#4727=CARTESIAN_POINT ( 'NONE',  ( 4.844604166567388681, 117.7309004960029171, 0.9915350356305726587 ) ) ;
#4729=CARTESIAN_POINT ( 'NONE',  ( -4.780815387031786656, 104.6144662015457527, 0.7323460767296593454 ) ) ;
#4730=CARTESIAN_POINT ( 'NONE',  ( -4.274281473441157608, 3.541781053574249327, 1.790774723582081451 ) ) ;
#4732=CARTESIAN_POINT ( 'NONE',  ( -2.928647764479141102, 107.6119852313951526, -4.449003297184745520 ) ) ;
#4733=CARTESIAN_POINT ( 'NONE',  ( 3.297440819997984107, -14.19009280176566890, 4.446257544676719853 ) ) ;
#4734=CARTESIAN_POINT ( 'NONE',  ( 3.145827930497913538, 117.0475107411037641, -1.097865318250619726 ) ) ;
#4735=CARTESIAN_POINT ( 'NONE',  ( 0.9281906404964566093, 34.59732502943162302, 2.863135987906454183 ) ) ;
#4736=CARTESIAN_POINT ( 'NONE',  ( -2.052054811892178421, 115.7029480924404226, 1.635839580152672390 ) ) ;
#4738=CARTESIAN_POINT ( 'NONE',  ( -4.506737449472459467, 104.6144662015545350, -2.874441546340825049 ) ) ;
#4739=CARTESIAN_POINT ( 'NONE',  ( 2.422525963563016749, -15.70080278133445617, 5.253054914258033392 ) ) ;
#4740=CARTESIAN_POINT ( 'NONE',  ( -10.86053312202636079, 155.9024031350590462, 1.736732359437422879 ) ) ;
#4741=CARTESIAN_POINT ( 'NONE',  ( 0.1338929724787690234, 25.55936205620983515, 0.9658879472844225100 ) ) ;
#4746=CARTESIAN_POINT ( 'NONE',  ( 4.584725329087942391, 124.7699485019152945, 0.09621079440654298209 ) ) ;
#4747=CARTESIAN_POINT ( 'NONE',  ( -14.42666092703575664, 134.5679602169015254, 1.107736707283931032 ) ) ;
#4750=CARTESIAN_POINT ( 'NONE',  ( 4.541578696478873134, 118.0696556320928181, -0.6340941426453600149 ) ) ;
#4751=CARTESIAN_POINT ( 'NONE',  ( 11.32523555543259697, 123.0403929720162495, -1.197004354367267931 ) ) ;
#4753=CARTESIAN_POINT ( 'NONE',  ( -14.56794066961899148, 154.5799843816573684, -2.217559120334770650 ) ) ;
#4756=CARTESIAN_POINT ( 'NONE',  ( 4.316099701937201161, 118.2124166868408111, -0.3255499669043997457 ) ) ;
#4757=ADVANCED_FACE ( 'NONE', ( #9407 ), #32017, .T. ) ;
#4758=CARTESIAN_POINT ( 'NONE',  ( 14.45325548908953728, 139.0941462050048187, -0.3122831254358888198 ) ) ;
#4760=CARTESIAN_POINT ( 'NONE',  ( 3.092642723064080279, -14.67800799544728285, 3.675123631970977911 ) ) ;
#4763=CARTESIAN_POINT ( 'NONE',  ( -0.7749869142727341398, -12.81603963768374044, -4.556214072895795830 ) ) ;
#4764=CARTESIAN_POINT ( 'NONE',  ( 10.50156301541547244, 123.3532649940754027, 1.413946074136436692 ) ) ;
#4765=CARTESIAN_POINT ( 'NONE',  ( -2.808975559516362797, 29.02362447754844865, 0.3931306422602618977 ) ) ;
#4766=CARTESIAN_POINT ( 'NONE',  ( -4.883585300477498947, 117.2937442104795593, 0.7242188414070882541 ) ) ;
#4767=CARTESIAN_POINT ( 'NONE',  ( 3.102408547967445696, -0.5812848888516047863, -3.453265078539196509 ) ) ;
#4768=CARTESIAN_POINT ( 'NONE',  ( -0.0005023639978857188547, 120.9974662015457056, 0.02514034870427548501 ) ) ;
#4774=CARTESIAN_POINT ( 'NONE',  ( 8.794618831136583381, 117.7206556621920299, -0.02516188889388990338 ) ) ;
#4775=CARTESIAN_POINT ( 'NONE',  ( 0.004379098345483538150, 122.8649044353672934, -0.2191479880733794572 ) ) ;
#4777=FACE_OUTER_BOUND ( 'NONE', #41919, .T. ) ;
#4779=CARTESIAN_POINT ( 'NONE',  ( -2.166771814436331045, 10.43868160547798674, -8.139002505017437272 ) ) ;
#4780=ADVANCED_FACE ( 'NONE', ( #33684 ), #34100, .T. ) ;
#4782=DIRECTION ( 'NONE',  ( -0.9998004120163608288, 0.000000000000000000, -0.01997839162482747608 ) ) ;
#4784=CARTESIAN_POINT ( 'NONE',  ( 0.01386859376319274882, 119.8383472832138779, -0.6940411431075989013 ) ) ;
#4785=CARTESIAN_POINT ( 'NONE',  ( -22.77159426375468243, 150.3871190066015799, -0.004147128915567659807 ) ) ;
#4786=ORIENTED_EDGE ( 'NONE', *, *, #4211, .F. ) ;
#4790=CARTESIAN_POINT ( 'NONE',  ( -14.16569067496518564, 138.8670163227233161, -0.2830642121559646673 ) ) ;
#4791=CARTESIAN_POINT ( 'NONE',  ( 3.639791848495840476, -15.36872039720094207, 5.326864320309495859 ) ) ;
#4792=CARTESIAN_POINT ( 'NONE',  ( -20.46179744412678758, 141.4490678312372722, 1.579512522682919418 ) ) ;
#4793=CARTESIAN_POINT ( 'NONE',  ( 14.96856157597580150, 121.5307057168427605, -0.7335553340177136672 ) ) ;
#4794=CARTESIAN_POINT ( 'NONE',  ( 1.111903444298625754, 15.29877551736591812, 4.515507465039587665 ) ) ;
#4795=CARTESIAN_POINT ( 'NONE',  ( -10.79372094067549526, 157.9251727141802633, -0.3940533352873706874 ) ) ;
#4798=CARTESIAN_POINT ( 'NONE',  ( 8.793348182195531493, 117.6962994879057334, 0.2883727696902242954 ) ) ;
#4799=CARTESIAN_POINT ( 'NONE',  ( -11.03120429849349193, 123.2082810311540300, 1.124825114493487543 ) ) ;
#4801=CARTESIAN_POINT ( 'NONE',  ( 18.78250995143891089, 149.1225091032880528, -1.736135053443003784 ) ) ;
#4802=CARTESIAN_POINT ( 'NONE',  ( -20.19347568108163671, 136.2683111393718320, -2.155148867324337303 ) ) ;
#4805=CARTESIAN_POINT ( 'NONE',  ( 9.788763933236980463, 123.8372022493589100, -0.5907035020478675902 ) ) ;
#4808=CARTESIAN_POINT ( 'NONE',  ( -0.8917109795615992818, 157.3234082283764792, -1.558336142952463810 ) ) ;
#4809=CARTESIAN_POINT ( 'NONE',  ( 4.514867502249738429, -15.46117574218924773, 1.158286244139274279 ) ) ;
#4810=CARTESIAN_POINT ( 'NONE',  ( -4.491279449957480630, 118.0838085148757841, -0.7971429151108968547 ) ) ;
#4813=CARTESIAN_POINT ( 'NONE',  ( 5.835695000730356519, 120.1673030736515955, 1.074193948046630709 ) ) ;
#4814=ADVANCED_FACE ( 'NONE', ( #8101 ), #32652, .T. ) ;
#4816=CARTESIAN_POINT ( 'NONE',  ( 20.69815783549627497, 152.5608647341385335, 0.3383848979192933260 ) ) ;
#4818=CARTESIAN_POINT ( 'NONE',  ( -6.605212570472872358, 13.46189590645272460, 5.224192399652773489 ) ) ;
#4819=CARTESIAN_POINT ( 'NONE',  ( 2.769557799161845857, 120.9068798055765370, 0.2367794989410801354 ) ) ;
#4820=CARTESIAN_POINT ( 'NONE',  ( 4.801338745261147345, 117.3993836135855275, -1.016148444996444189 ) ) ;
#4825=EDGE_CURVE ( 'NONE', #4233, #5241, #11691, .T. ) ;
#4827=CARTESIAN_POINT ( 'NONE',  ( -21.64725176087522840, 132.7051459832101443, -0.3678724904816468300 ) ) ;
#4830=CARTESIAN_POINT ( 'NONE',  ( -6.848981279076908457, 121.5714736848644861, -0.7266479796884791620 ) ) ;
#4831=DIRECTION ( 'NONE',  ( 0.9998004120163609398, 0.000000000000000000, 0.01997839162482749689 ) ) ;
#4833=CARTESIAN_POINT ( 'NONE',  ( 0.6269658669242333948, 115.7029626408947536, -1.737418004581801290 ) ) ;
#4834=CARTESIAN_POINT ( 'NONE',  ( -15.80138807371441523, 145.9351319680867221, -0.6472794460535241656 ) ) ;
#4835=CARTESIAN_POINT ( 'NONE',  ( 3.288375567735513094, -14.78372392556953585, 5.458595067156710279 ) ) ;
#4836=CARTESIAN_POINT ( 'NONE',  ( -0.3953301572312742929, 117.5049145548240972, 0.4632619789290193246 ) ) ;
#4838=CARTESIAN_POINT ( 'NONE',  ( 8.055701656131518007, 158.6724238832827609, 0.2706798611393589904 ) ) ;
#4839=CARTESIAN_POINT ( 'NONE',  ( 8.901366582544378403, 123.9008345302928120, 0.2219616208084491948 ) ) ;
#4841=CARTESIAN_POINT ( 'NONE',  ( 0.9475510003767251277, 17.78785052102138664, 0.2306771022979090535 ) ) ;
#4842=CARTESIAN_POINT ( 'NONE',  ( -5.755000932441543426, 159.1151184437813981, -0.1316611545253205395 ) ) ;
#4846=CARTESIAN_POINT ( 'NONE',  ( 3.037128892075650288, 117.4034716445605540, 0.7578594852576387986 ) ) ;
#4847=CARTESIAN_POINT ( 'NONE',  ( 3.440871586586784492, -6.993729544307833557, 3.087053954803492317 ) ) ;
#4848=CARTESIAN_POINT ( 'NONE',  ( 3.949038439882183837, 117.6225627337916393, 0.7921763187007300200 ) ) ;
#4850=CARTESIAN_POINT ( 'NONE',  ( 4.664640489119654454, 158.0471523224993859, -1.621167461353164585 ) ) ;
#4851=CARTESIAN_POINT ( 'NONE',  ( -3.263082884110522386, 19.99377609092593389, 7.766292582686701529 ) ) ;
#4852=CARTESIAN_POINT ( 'NONE',  ( -22.54389841724633570, 148.7221180073953235, -1.757920738659724647 ) ) ;
#4853=CARTESIAN_POINT ( 'NONE',  ( 4.945934694223368844, 117.6258612243657637, -0.7624269308906101994 ) ) ;
#4856=CARTESIAN_POINT ( 'NONE',  ( -9.310784039460543227, 124.2035065715909496, 0.04725383350292546719 ) ) ;
#4857=CARTESIAN_POINT ( 'NONE',  ( 2.079616623477898329, -15.54617723206731839, 5.925385729176050553 ) ) ;
#4861=CARTESIAN_POINT ( 'NONE',  ( -3.610648906290234716, 109.1680670511277498, -3.931663264847707673 ) ) ;
#4863=CARTESIAN_POINT ( 'NONE',  ( 12.10717961583465652, 122.5392882283422864, 1.794329550371804194 ) ) ;
#4866=CARTESIAN_POINT ( 'NONE',  ( -2.437154581274205256, 119.8248006784163380, 0.4733635836876309289 ) ) ;
#4867=CARTESIAN_POINT ( 'NONE',  ( 8.368836169178564433, 3.587476746713724740, 1.217019533931793074 ) ) ;
#4868=CARTESIAN_POINT ( 'NONE',  ( 11.15578272721372421, 126.1638007343821641, 1.112962985253807657 ) ) ;
#4870=CARTESIAN_POINT ( 'NONE',  ( 0.3352962839983787968, 116.7787044104018861, -0.2500268678974714720 ) ) ;
#4871=CARTESIAN_POINT ( 'NONE',  ( -5.332935397695336199, 105.1224662015457199, -0.1065647409268299373 ) ) ;
#4879=CARTESIAN_POINT ( 'NONE',  ( -4.316210094789089347, 118.2124209707147742, 0.3254998515997128417 ) ) ;
#4880=CARTESIAN_POINT ( 'NONE',  ( 4.077454352797809989, 109.5187069194699632, -3.449181840922602049 ) ) ;
#4883=CARTESIAN_POINT ( 'NONE',  ( -8.274239857666382036, 120.1145857019959209, -1.449899955590871592 ) ) ;
#4884=CARTESIAN_POINT ( 'NONE',  ( -1.980401745281053172, 106.6864334246082961, -4.967395836420048560 ) ) ;
#4886=CARTESIAN_POINT ( 'NONE',  ( 4.255616016246193567, 118.2236154135255930, 0.4577608436404123071 ) ) ;
#4887=CARTESIAN_POINT ( 'NONE',  ( 0.01133107913638299775, 156.3792106723807649, -0.5670535347366656431 ) ) ;
#4888=CARTESIAN_POINT ( 'NONE',  ( 0.02983097934372052479, 117.3993836135855418, -1.492864285909942579 ) ) ;
#4890=CARTESIAN_POINT ( 'NONE',  ( 1.893578447776079754, 19.08455809737888487, -4.224370802633358402 ) ) ;
#4891=CARTESIAN_POINT ( 'NONE',  ( -7.898163624196860688, 121.8456834504061845, -1.011533665549599004 ) ) ;
#4895=CARTESIAN_POINT ( 'NONE',  ( -9.014953340893313793, 124.1466903544668838, -0.04592658822908208399 ) ) ;
#4896=CARTESIAN_POINT ( 'NONE',  ( 4.941652259254307289, 117.6448581155076880, -0.7476730690041486493 ) ) ;
#4897=CARTESIAN_POINT ( 'NONE',  ( 10.42794149288025984, 157.8855781193960297, 1.079236549925195465 ) ) ;
#4899=CARTESIAN_POINT ( 'NONE',  ( 2.994295736468014280, -14.77441112906794984, 3.968895097548184037 ) ) ;
#4900=CARTESIAN_POINT ( 'NONE',  ( 21.83857928711794116, 148.7205309135917730, -1.274413580488712006 ) ) ;
#4901=CARTESIAN_POINT ( 'NONE',  ( -5.067974813687988522, 119.5555251685854330, 0.8659238720033423098 ) ) ;
#4902=CIRCLE ( 'NONE', #25273, 0.5080000000000002292 ) ;
#4903=CARTESIAN_POINT ( 'NONE',  ( -0.6538259107469485132, -10.21753563294075384, 0.7251761174241220242 ) ) ;
#4904=CARTESIAN_POINT ( 'NONE',  ( -22.97411545401789468, 149.2143936249396461, -1.313106760764511050 ) ) ;
#4905=CARTESIAN_POINT ( 'NONE',  ( 0.1179719058304127544, 10.27755972103446958, 0.9685762618712100425 ) ) ;
#4906=EDGE_LOOP ( 'NONE', ( #26892, #32231, #22425, #41155 ) ) ;
#4908=CARTESIAN_POINT ( 'NONE',  ( -9.648208730819588297, 124.2480737032941533, 0.3321887029122945756 ) ) ;
#4909=CARTESIAN_POINT ( 'NONE',  ( 3.665585082022325025, -14.37195162699216056, 4.995470683262428935 ) ) ;
#4910=CARTESIAN_POINT ( 'NONE',  ( 10.84039127762408228, 123.6843197456346672, -1.011594478071749625 ) ) ;
#4911=ORIENTED_EDGE ( 'NONE', *, *, #32619, .F. ) ;
#4912=CIRCLE ( 'NONE', #19167, 3.175000000000001155 ) ;
#4913=CARTESIAN_POINT ( 'NONE',  ( 0.5786556323373592825, 115.7029630015946111, 1.760570191192437628 ) ) ;
#4915=CARTESIAN_POINT ( 'NONE',  ( 3.387566103704702236, -13.77904243453481570, 2.987699908524332759 ) ) ;
#4916=CARTESIAN_POINT ( 'NONE',  ( -4.940781816828488715, 117.5342059363709950, -0.9902978256015019243 ) ) ;
#4917=CARTESIAN_POINT ( 'NONE',  ( 4.236260012103334915, 155.8470599587123502, -0.007037385900262056911 ) ) ;
#4918=ORIENTED_EDGE ( 'NONE', *, *, #26356, .F. ) ;
#4919=CARTESIAN_POINT ( 'NONE',  ( 3.146714701748970278, 118.3302933575512412, 0.8734028913305708075 ) ) ;
#4920=CARTESIAN_POINT ( 'NONE',  ( 5.183445353050514015, 115.9099169135977974, 1.326074002626195680 ) ) ;
#4921=CARTESIAN_POINT ( 'NONE',  ( -6.604303299200508256E-14, 94.83546620154572793, -1.207165459215201580E-19 ) ) ;
#4922=CARTESIAN_POINT ( 'NONE',  ( 0.03212618750946916180, 158.2819368290249713, -1.607725792532325393 ) ) ;
#4923=CARTESIAN_POINT ( 'NONE',  ( 8.215251585939698842, 117.5146787832509858, 0.03113046551775530690 ) ) ;
#4925=CARTESIAN_POINT ( 'NONE',  ( 1.920772546426502192, -15.19580626328599671, 5.957450100407664983 ) ) ;
#4926=CARTESIAN_POINT ( 'NONE',  ( -4.645572480595541620, 117.9340260526530813, 0.7769932229682322555 ) ) ;
#4927=DIRECTION ( 'NONE',  ( -0.9998004120163608288, 0.000000000000000000, -0.01997839162482749342 ) ) ;
#4928=CARTESIAN_POINT ( 'NONE',  ( -4.633588795532518567, 117.9522783733740567, 0.7617726623130426367 ) ) ;
#4930=CARTESIAN_POINT ( 'NONE',  ( 5.204330674627346554, 115.7029491485453150, -1.024362258486631649 ) ) ;
#4931=CARTESIAN_POINT ( 'NONE',  ( 3.328596738436636393, 118.4670010328146503, -0.7846298696386536653 ) ) ;
#4932=CARTESIAN_POINT ( 'NONE',  ( 0.1065646865915094166, 105.8844662015457061, -5.332932678536314697 ) ) ;
#4933=CARTESIAN_POINT ( 'NONE',  ( 4.748484029138242413, 117.5371517732831421, 1.178549711470926020 ) ) ;
#4934=CARTESIAN_POINT ( 'NONE',  ( -1.058771226886514372, 124.8229041592835387, -0.01153269281271720494 ) ) ;
#4935=AXIS2_PLACEMENT_3D ( 'NONE', #41822, #18995, #38193 ) ;
#4936=CARTESIAN_POINT ( 'NONE',  ( 1.398650104629075797, 0.06838872207683838189, -4.420329592304430122 ) ) ;
#4939=CARTESIAN_POINT ( 'NONE',  ( 3.022112892507086812, -12.39725416092116106, 0.4273193741429963666 ) ) ;
#4940=CARTESIAN_POINT ( 'NONE',  ( 3.998592866256202694, 116.4303826247378026, -1.177299868075282641 ) ) ;
#4941=CARTESIAN_POINT ( 'NONE',  ( 0.1238897909883466403, 36.81462384746927086, 2.295035569577275059 ) ) ;
#4942=CARTESIAN_POINT ( 'NONE',  ( -2.044842387155601848, 115.7029490949802266, 1.636383577350578156 ) ) ;
#4944=CARTESIAN_POINT ( 'NONE',  ( -4.979428488236589345, 104.6144662015479412, -1.943962536390259954 ) ) ;
#4945=CARTESIAN_POINT ( 'NONE',  ( 1.868457900240735103, -15.55086107261449690, 5.421086310357067894 ) ) ;
#4946=CARTESIAN_POINT ( 'NONE',  ( -0.03245814172817860360, 158.1186941186938952, 1.624338139048501661 ) ) ;
#4947=CARTESIAN_POINT ( 'NONE',  ( 0.6255416438669687551, 26.40915095058528905, 0.7518939258676016202 ) ) ;
#4951=FACE_OUTER_BOUND ( 'NONE', #13212, .T. ) ;
#4952=CARTESIAN_POINT ( 'NONE',  ( 4.364892838101803285, 123.4689364668338385, 0.1663115080531035461 ) ) ;
#4953=CARTESIAN_POINT ( 'NONE',  ( -7.221579903134116130, 121.4526873951801633, 0.6561908252823553944 ) ) ;
#4955=CARTESIAN_POINT ( 'NONE',  ( 4.584778834665758751, 118.0135720478281485, -0.7024323280929735125 ) ) ;
#4956=CARTESIAN_POINT ( 'NONE',  ( 5.099922610523941024, 119.9665122172617231, -0.7872683264543846038 ) ) ;
#4957=CARTESIAN_POINT ( 'NONE',  ( -4.088037439073751500, 118.5849532427036905, -0.9900007573961080443 ) ) ;
#4959=ORIENTED_EDGE ( 'NONE', *, *, #15150, .T. ) ;
#4960=CARTESIAN_POINT ( 'NONE',  ( 4.257727891021212407, 118.2250048574998829, -0.3017987544622640628 ) ) ;
#4961=CARTESIAN_POINT ( 'NONE',  ( 2.758537940428885005, 120.8469057251343060, -0.1732774955029139363 ) ) ;
#4963=CARTESIAN_POINT ( 'NONE',  ( 2.908198840139253338, -13.99431844974620454, 0.6722015529863232253 ) ) ;
#4966=B_SPLINE_CURVE_WITH_KNOTS ( 'NONE', 3,
 ( #27806, #40814, #8433, #12040, #18635, #20986, #11615, #28444, #5251, #37194 ),
 .UNSPECIFIED., .F., .F.,
 ( 4, 2, 2, 2, 4 ),
 ( -5.999999999942070351E-08, 0.0005999509680439210927, 0.001199961936087841612, 0.002399983872175682868, 0.004800027744351364513 ),
 .UNSPECIFIED. ) ;
#4968=CARTESIAN_POINT ( 'NONE',  ( 2.459658384930404118, -7.418532284756778949, 3.912982838641719141 ) ) ;
#4969=CARTESIAN_POINT ( 'NONE',  ( 14.69551782889044489, 134.6798445586954927, 1.826766161810339462 ) ) ;
#4970=CARTESIAN_POINT ( 'NONE',  ( 2.878515509655334093, 37.92758169195481344, 1.187197144508459701 ) ) ;
#4971=CARTESIAN_POINT ( 'NONE',  ( -6.983131083342716927, 124.7321584522365896, -0.1385298619991067737 ) ) ;
#4973=CARTESIAN_POINT ( 'NONE',  ( 1.961646697876492373, -0.1315482170498871728, -4.191205975169975950 ) ) ;
#4974=CARTESIAN_POINT ( 'NONE',  ( 15.76280660274394663, 145.9085485750152316, 0.3664889719343316088 ) ) ;
#4975=CARTESIAN_POINT ( 'NONE',  ( 5.239248437989107998, 115.6909491485453145, 1.024417804751308614 ) ) ;
#4979=CARTESIAN_POINT ( 'NONE',  ( 8.784622439875429123, 117.7823766468853250, -0.1582906694335896591 ) ) ;
#4980=CARTESIAN_POINT ( 'NONE',  ( 0.008700780993235806074, 121.2597428844645293, -0.4354226598341944809 ) ) ;
#4983=CARTESIAN_POINT ( 'NONE',  ( -3.044072069279135651, 34.44269722464345307, 3.574075509920750626 ) ) ;
#4984=CARTESIAN_POINT ( 'NONE',  ( 0.8402904295469701967, 0.2923264105788614398, -8.379105243356319122 ) ) ;
#4985=FACE_OUTER_BOUND ( 'NONE', #30038, .T. ) ;
#4988=CARTESIAN_POINT ( 'NONE',  ( 0.09221630143774380006, 107.6766875080336376, -4.614880812453306724 ) ) ;
#4989=CARTESIAN_POINT ( 'NONE',  ( -20.57623859521469001, 152.5775223076369400, 0.1637982859500254906 ) ) ;
#4990=VERTEX_POINT ( 'NONE', #18089 ) ;
#4995=CARTESIAN_POINT ( 'NONE',  ( -4.218275339060285845, 155.8585684991085714, -0.08429118021179402009 ) ) ;
#4996=CARTESIAN_POINT ( 'NONE',  ( 3.586901592285024698, -15.56753269123677086, 5.192771612050266050 ) ) ;
#4997=CARTESIAN_POINT ( 'NONE',  ( -1.193991991012630205, 158.7113841514841681, 1.470390664574136252 ) ) ;
#4999=CARTESIAN_POINT ( 'NONE',  ( 16.19941014871825402, 155.1612327564137388, -0.8792224148362001168 ) ) ;
#5000=CARTESIAN_POINT ( 'NONE',  ( -0.8080508600641240768, 24.25718022715097888, 4.550674767031389401 ) ) ;
#5001=CARTESIAN_POINT ( 'NONE',  ( -16.04055624107204636, 121.3766923467913585, -0.6455242483069041359 ) ) ;
#5003=CARTESIAN_POINT ( 'NONE',  ( 8.792199711666244255, 117.7001252806687148, 0.3065861086990905870 ) ) ;
#5005=CARTESIAN_POINT ( 'NONE',  ( -2.509025565091423715, 119.7126118883416410, 0.5998098196673843363 ) ) ;
#5007=CARTESIAN_POINT ( 'NONE',  ( 0.5002616235672558975, 119.0154928070276412, -0.5875571981567377922 ) ) ;
#5008=CARTESIAN_POINT ( 'NONE',  ( 0.02399864187730229442, 159.1630378086529731, -1.200990174154242141 ) ) ;
#5012=CARTESIAN_POINT ( 'NONE',  ( 0.5989337510911817430, 120.4790399057546182, -0.3068722873270139928 ) ) ;
#5013=ORIENTED_EDGE ( 'NONE', *, *, #29167, .F. ) ;
#5014=CARTESIAN_POINT ( 'NONE',  ( -18.14277298170013708, 148.2327041560005512, -2.387153687107330224 ) ) ;
#5015=CARTESIAN_POINT ( 'NONE',  ( 4.191701569836151720, -15.46661069841161229, 1.593937231346424843 ) ) ;
#5016=CARTESIAN_POINT ( 'NONE',  ( -4.486916041353520512, 118.0822494517943966, -0.8002166990800740898 ) ) ;
#5018=CARTESIAN_POINT ( 'NONE',  ( -4.852412226131026962, 117.4768382700202238, 0.9922438998348902528 ) ) ;
#5019=CARTESIAN_POINT ( 'NONE',  ( 11.12287255170432232, 123.1247571232444784, 1.608126361149619044 ) ) ;
#5020=DIRECTION ( 'NONE',  ( -0.9998004120163610509, -5.205824365704083805E-17, -0.01997839162482749689 ) ) ;
#5022=CARTESIAN_POINT ( 'NONE',  ( 0.8920107295035074602, 116.4394364983335493, -0.02072182073814201816 ) ) ;
#5024=CARTESIAN_POINT ( 'NONE',  ( 8.391957350906555035, -2.082342975431243026, 0.7039615705134369961 ) ) ;
#5025=CARTESIAN_POINT ( 'NONE',  ( 10.48728279712171663, 126.1106773019354819, 0.5683957799248651188 ) ) ;
#5029=CARTESIAN_POINT ( 'NONE',  ( -2.601682421829722980, 117.9394517735116210, 1.236607248841048667 ) ) ;
#5030=CARTESIAN_POINT ( 'NONE',  ( -7.931483696868459887, 121.8266375666164834, -1.035712634723692682 ) ) ;
#5033=EDGE_CURVE ( 'NONE', #20535, #40413, #13020, .T. ) ;
#5034=CARTESIAN_POINT ( 'NONE',  ( -2.769246990705085398, 116.5678055239024644, 0.05256187475617120353 ) ) ;
#5037=CARTESIAN_POINT ( 'NONE',  ( -7.892965638028277553, 122.0249252363302332, -0.9262618160925026878 ) ) ;
#5038=CARTESIAN_POINT ( 'NONE',  ( -8.026787933082857762, 121.5445110286360801, 0.8405406253987726117 ) ) ;
#5039=AXIS2_PLACEMENT_3D ( 'NONE', #13503, #36306, #16259 ) ;
#5041=CARTESIAN_POINT ( 'NONE',  ( 4.060319184079548727, 115.6909491485452435, -1.425993417255509987 ) ) ;
#5042=CARTESIAN_POINT ( 'NONE',  ( -9.229262982541685645, 124.0999252189730697, -0.4162339757116149674 ) ) ;
#5043=CARTESIAN_POINT ( 'NONE',  ( 4.908419482240064191, -12.74103600948764381, 2.406175225133469819 ) ) ;
#5044=CARTESIAN_POINT ( 'NONE',  ( -2.090077592200571655, 117.5043770775735510, 0.5427014567576284865 ) ) ;
#5045=DIRECTION ( 'NONE',  ( -4.017660918040594346E-17, 1.000000000000000000, 2.376309959284834438E-19 ) ) ;
#5046=CARTESIAN_POINT ( 'NONE',  ( 17.17229002331729859, 122.7237354506536491, 0.5096938506424069093 ) ) ;
#5047=CARTESIAN_POINT ( 'NONE',  ( -6.439798515484507670E-14, 156.3034662015457172, 9.575285601066443938E-17 ) ) ;
#5049=CARTESIAN_POINT ( 'NONE',  ( -0.5455758836206960893, 21.45819190514113117, -0.8097498057291211415 ) ) ;
#5050=CARTESIAN_POINT ( 'NONE',  ( -23.21373371908098449, 149.6306211361744829, -0.4638656453230912136 ) ) ;
#5055=CARTESIAN_POINT ( 'NONE',  ( -8.380759076080833481, 119.8444141578249287, 1.108220873400043383 ) ) ;
#5057=CARTESIAN_POINT ( 'NONE',  ( 21.06903215802083906, 150.2702755442954583, 2.120733010085479986 ) ) ;
#5059=CARTESIAN_POINT ( 'NONE',  ( 20.48420673234485534, 149.1468970683199586, -1.615293151967227558 ) ) ;
#5061=CARTESIAN_POINT ( 'NONE',  ( 2.913282581332740762, -14.11548038430587937, -3.586046950971230274 ) ) ;
#5062=CARTESIAN_POINT ( 'NONE',  ( -22.34249146463940860, 149.5981344557702641, -1.749037778780574204 ) ) ;
#5063=CARTESIAN_POINT ( 'NONE',  ( 4.794168055694363773, 117.6364379244655680, -0.9473893282713367059 ) ) ;
#5065=VERTEX_POINT ( 'NONE', #27895 ) ;
#5066=CARTESIAN_POINT ( 'NONE',  ( -9.238523569214027731, 124.0999252189730697, 0.04720364951821285487 ) ) ;
#5068=CARTESIAN_POINT ( 'NONE',  ( 6.397261194921658678, -14.09295207620744961, -0.07176229933514734205 ) ) ;
#5071=EDGE_CURVE ( 'NONE', #24980, #17493, #4912, .T. ) ;
#5074=CARTESIAN_POINT ( 'NONE',  ( 5.016192601342504886, 119.3892302351119810, 1.087184205914811574 ) ) ;
#5076=TOROIDAL_SURFACE ( 'NONE', #31569, 5.080000000000005400, 0.5080000000000000071 ) ;
#5077=CARTESIAN_POINT ( 'NONE',  ( 5.078986093043054595, 72.48346620154573827, 0.1014902294541243782 ) ) ;
#5078=CARTESIAN_POINT ( 'NONE',  ( -2.387353046264593548, 119.4803856251332945, 0.5366433100809054890 ) ) ;
#5079=CARTESIAN_POINT ( 'NONE',  ( 0.8732425085435751022, -3.549726780817298977, -8.398906084147368389 ) ) ;
#5080=CARTESIAN_POINT ( 'NONE',  ( 9.787166303541834367, 124.1138826855306831, 0.8907577946409742653 ) ) ;
#5081=CARTESIAN_POINT ( 'NONE',  ( -4.726681166799090228, 118.5930653697794384, -1.020516978120344476 ) ) ;
#5082=CARTESIAN_POINT ( 'NONE',  ( 2.881812722985360953, 116.8851979753409580, -0.3221759108904497793 ) ) ;
#5087=CARTESIAN_POINT ( 'NONE',  ( 1.858891552337616826, -15.10179129218686711, 5.555419934288657657 ) ) ;
#5088=CARTESIAN_POINT ( 'NONE',  ( -4.266030196957218301, 118.2243171346437407, 0.2924649446876417258 ) ) ;
#5090=EDGE_LOOP ( 'NONE', ( #3682, #11368, #8634, #15558, #23099, #490, #37101, #24090, #37153, #22767, #31433 ) ) ;
#5092=CARTESIAN_POINT ( 'NONE',  ( 4.269537782945402427, 119.3621508961521442, -0.7584028417339077066 ) ) ;
#5094=CARTESIAN_POINT ( 'NONE',  ( 4.291477964748057872, 118.2137869882025001, 0.5063463920358112214 ) ) ;
#5095=CARTESIAN_POINT ( 'NONE',  ( -7.076231864619286327, 121.9239394581621809, -0.5528764260536546127 ) ) ;
#5097=CARTESIAN_POINT ( 'NONE',  ( 14.91134437181069927, 120.3281135998953459, 0.2979641475761143354 ) ) ;
#5098=VERTEX_POINT ( 'NONE', #31094 ) ;
#5099=CARTESIAN_POINT ( 'NONE',  ( 4.496586626007489151, 27.28078351817337222, -1.068494511273165193 ) ) ;
#5100=CARTESIAN_POINT ( 'NONE',  ( -11.65596162629437593, 126.1299551460304542, -1.384704262848757583 ) ) ;
#5105=CARTESIAN_POINT ( 'NONE',  ( 6.996049371394188476, 121.9530687059719583, 0.1976249421933106154 ) ) ;
#5106=CARTESIAN_POINT ( 'NONE',  ( -4.024516124431025688, 26.91537645720152128, -2.298571904627217499 ) ) ;
#5107=CARTESIAN_POINT ( 'NONE',  ( 20.68355264112275904, 132.2482564273973935, 1.400420337322433983 ) ) ;
#5109=CARTESIAN_POINT ( 'NONE',  ( 3.213008622916347701, -14.43860267280072662, 2.307402664594705222 ) ) ;
#5110=CARTESIAN_POINT ( 'NONE',  ( 13.60293432442217210, 121.5020190402118203, -1.066732574264078526 ) ) ;
#5111=CARTESIAN_POINT ( 'NONE',  ( -16.36721571005508835, 151.0861551944122141, 1.708847769304776110 ) ) ;
#5112=CARTESIAN_POINT ( 'NONE',  ( -1.535301415185580609, 19.99377045568717293, 4.360315235486975638 ) ) ;
#5113=CARTESIAN_POINT ( 'NONE',  ( -3.210256534570933962, 159.4348965051207756, -0.5208765431038285820 ) ) ;
#5114=CARTESIAN_POINT ( 'NONE',  ( 0.2465545558977290663, 24.09562519341298170, -0.9435640554424079562 ) ) ;
#5115=ORIENTED_EDGE ( 'NONE', *, *, #7621, .F. ) ;
#5117=B_SPLINE_CURVE_WITH_KNOTS ( 'NONE', 3,
 ( #19722, #380, #35729, #32741, #26129, #35515, #6133, #22907, #10147, #28900, #29324, #6540, #6336, #29108, #39131, #41915, #32105, #9937, #12715, #35941, #25705, #3574, #16535, #6970, #22487, #29545, #41703, #19306, #13346, #26335, #36153, #19941, #12511, #10776, #13562 ),
 .UNSPECIFIED., .F., .F.,
 ( 4, 1, 1, 1, 1, 1, 1, 1, 1, 1, 1, 1, 1, 1, 1, 1, 1, 1, 1, 1, 1, 1, 1, 1, 1, 1, 1, 1, 1, 1, 1, 1, 4 ),
 ( 0.000000000000000000, 0.02711375962671787321, 0.05385523109991235263, 0.08027126036152537614, 0.1064096946071439176, 0.1323192412471900226, 0.1580495177521483718, 0.1882118685537063907, 0.2182788543618764954, 0.2483346178351386324, 0.2784631806910429774, 0.3054937156393619513, 0.3327069032348308197, 0.3601597580799023035, 0.3879077415152338837, 0.4160045136367338525, 0.4445017332217630623, 0.4734489055539064517, 0.5028932750457014711, 0.5328797594123376724, 0.5634509204570880003, 0.5946469669818265080, 0.6265057848166851739, 0.6590629893014032792, 0.6923519956652609553, 0.7264041031822485728, 0.7612485893105871426, 0.7986318966073006065, 0.8369441774603861850, 0.8762126957585177900, 0.9164627945539034481, 0.9577180065289634392, 1.000000000000000000 ),
 .UNSPECIFIED. ) ;
#5118=CARTESIAN_POINT ( 'NONE',  ( -0.6165924928998587351, 120.7136710450757988, 0.2143668442300581123 ) ) ;
#5119=CARTESIAN_POINT ( 'NONE',  ( 2.450443274655972559, -15.26395620497007855, 5.889056594049635329 ) ) ;
#5120=CARTESIAN_POINT ( 'NONE',  ( 7.262759831279620215, 121.2980461901665308, -0.7361999724971874937 ) ) ;
#5121=ORIENTED_EDGE ( 'NONE', *, *, #37079, .T. ) ;
#5122=CARTESIAN_POINT ( 'NONE',  ( 1.405512873546346686, 115.7027606773773130, 1.735607224157626360 ) ) ;
#5125=CARTESIAN_POINT ( 'NONE',  ( 3.089232434235547942, -13.39873834325867819, 1.372807258641574935 ) ) ;
#5126=CARTESIAN_POINT ( 'NONE',  ( -4.784569842647550253, 117.8429238250669329, -0.9400432804894900407 ) ) ;
#5127=CARTESIAN_POINT ( 'NONE',  ( 8.054407255016364786, 122.8529229587361442, 0.1293742239074502920 ) ) ;
#5128=ADVANCED_FACE ( 'NONE', ( #38338 ), #17788, .T. ) ;
#5130=CARTESIAN_POINT ( 'NONE',  ( 5.840405771877526853, 118.8996324090661147, 1.179527747254400349 ) ) ;
#5131=CARTESIAN_POINT ( 'NONE',  ( -3.682264917456322895, 65.62546620154573418, -0.07358041635423968885 ) ) ;
#5132=DIRECTION ( 'NONE',  ( 4.017660918040594346E-17, -1.000000000000000000, -2.376309959284834438E-19 ) ) ;
#5133=CARTESIAN_POINT ( 'NONE',  ( 0.03067001211929198945, 158.6015251912307633, -1.534852821454057770 ) ) ;
#5134=CARTESIAN_POINT ( 'NONE',  ( 6.912985389844387818, 117.2044255678715814, -0.04371034868568298565 ) ) ;
#5136=CARTESIAN_POINT ( 'NONE',  ( 1.939574901179839994, -15.09955500034904041, 5.855824770328826645 ) ) ;
#5139=CARTESIAN_POINT ( 'NONE',  ( -4.713257660251447767, 117.8947922744557815, 0.7957716318157286306 ) ) ;
#5142=CARTESIAN_POINT ( 'NONE',  ( -4.908310932783608749, 117.4079579380719736, 0.9676122992747743234 ) ) ;
#5143=CARTESIAN_POINT ( 'NONE',  ( 8.499044578041351272, 119.2581920680855774, -1.011821766694761981 ) ) ;
#5144=CARTESIAN_POINT ( 'NONE',  ( -4.571503503190820439, 114.7252160460498516, -1.874454982749236276 ) ) ;
#5145=CARTESIAN_POINT ( 'NONE',  ( 4.862967985527940407, 117.6413485483879953, 1.052801483323805298 ) ) ;
#5146=CARTESIAN_POINT ( 'NONE',  ( -6.517733866319332394E-14, 78.32546620154573702, 2.848871684924056535E-29 ) ) ;
#5147=CARTESIAN_POINT ( 'NONE',  ( -0.7689147969093301782, 119.5055576915191580, 0.7020325503247997201 ) ) ;
#5148=CARTESIAN_POINT ( 'NONE',  ( 4.900892916173488878, 117.4105777512120596, -0.9669312268769758578 ) ) ;
#5149=FACE_OUTER_BOUND ( 'NONE', #4624, .T. ) ;
#5150=CARTESIAN_POINT ( 'NONE',  ( 3.456814872816273088, -13.76118077623555891, 3.223863823609153023 ) ) ;
#5151=CARTESIAN_POINT ( 'NONE',  ( 2.817215192600937446, 108.0685014782224442, -4.280041469292686251 ) ) ;
#5152=CARTESIAN_POINT ( 'NONE',  ( -4.381111989981776311, 28.12932232230255281, 1.300020847918438527 ) ) ;
#5153=CIRCLE ( 'NONE', #28924, 5.588000000000006295 ) ;
#5154=CARTESIAN_POINT ( 'NONE',  ( -0.6390711918370651778, 115.7029491485453292, 1.736656509918723668 ) ) ;
#5155=CARTESIAN_POINT ( 'NONE',  ( -4.247245584637960647, 22.75789413176893206, 1.861891798430825862 ) ) ;
#5157=CARTESIAN_POINT ( 'NONE',  ( -3.490548159187448096, 104.6144662015455253, -3.347245557147066286 ) ) ;
#5158=CARTESIAN_POINT ( 'NONE',  ( 4.167245103190982292, -15.48560191675932352, 1.819225864046467356 ) ) ;
#5159=CARTESIAN_POINT ( 'NONE',  ( -19.82182223277795075, 148.2167131080949787, 1.724547319354139630 ) ) ;
#5160=CARTESIAN_POINT ( 'NONE',  ( -0.9201843903949125103, 16.76996313919548598, -0.3265437062991076722 ) ) ;
#5161=CARTESIAN_POINT ( 'NONE',  ( -0.09387087892865565719, 20.69761720779959902, -0.9769954323643923466 ) ) ;
#5164=DIRECTION ( 'NONE',  ( -0.9998004120163608288, 0.000000000000000000, -0.01997839162482749342 ) ) ;
#5165=CARTESIAN_POINT ( 'NONE',  ( 2.231675704589601850, 117.6064948828932444, 1.117935386608752024 ) ) ;
#5166=CARTESIAN_POINT ( 'NONE',  ( -7.857169925943728650, 121.9903164032602518, 0.5981771023335126225 ) ) ;
#5169=CARTESIAN_POINT ( 'NONE',  ( 4.535580177108445632, 118.0878415417625433, -0.6032448829988410477 ) ) ;
#5170=CARTESIAN_POINT ( 'NONE',  ( 18.18950303832456328, 147.2296321676236062, -1.619102437044615206 ) ) ;
#5171=CARTESIAN_POINT ( 'NONE',  ( -20.02396230387753917, 148.3334041379468715, -2.502640320863741330 ) ) ;
#5172=CARTESIAN_POINT ( 'NONE',  ( 4.801216665947148243, 117.4032681888235459, -1.015537427445656782 ) ) ;
#5174=CARTESIAN_POINT ( 'NONE',  ( -6.398136396394987102, 30.40553754182522539, 1.409394703459281084 ) ) ;
#5175=CARTESIAN_POINT ( 'NONE',  ( 0.006534791579796636780, 156.3267223255430167, -0.3270276925529294054 ) ) ;
#5177=CARTESIAN_POINT ( 'NONE',  ( 3.221942100833175893, -14.53498920702628361, 2.661941298785070575 ) ) ;
#5178=( BOUNDED_CURVE ( )  B_SPLINE_CURVE ( 3, ( #31995, #22797, #12409, #28591 ),
 .UNSPECIFIED., .F., .T. ) 
 B_SPLINE_CURVE_WITH_KNOTS ( ( 4, 4 ),
 ( 0.5001855759278981406, 0.7498838476046071344 ),
 .UNSPECIFIED. ) 
 CURVE ( )  GEOMETRIC_REPRESENTATION_ITEM ( )  RATIONAL_B_SPLINE_CURVE ( ( 1.000000000000000000, 0.6670689721821350116, 0.5004025482900600341, 0.5000007283237750677 ) ) 
 REPRESENTATION_ITEM ( '' )  );
#5181=CIRCLE ( 'NONE', #3134, 0.5080000000000002292 ) ;
#5182=CARTESIAN_POINT ( 'NONE',  ( -2.587970193024280441, -12.16632112844677494, -3.833404006186521773 ) ) ;
#5183=CARTESIAN_POINT ( 'NONE',  ( 15.47075146591460104, 139.6011575924185877, 1.761802977227842737 ) ) ;
#5184=FACE_OUTER_BOUND ( 'NONE', #21824, .T. ) ;
#5185=CARTESIAN_POINT ( 'NONE',  ( -2.433495328593940243, 107.4436264546101967, 4.557236999380250175 ) ) ;
#5186=CARTESIAN_POINT ( 'NONE',  ( 2.267534764145236803, 6.115564135048844108, 4.037922524061999141 ) ) ;
#5187=CARTESIAN_POINT ( 'NONE',  ( 8.770618086120967050, 123.6813396614493712, 0.1752578222716852652 ) ) ;
#5188=CARTESIAN_POINT ( 'NONE',  ( 8.137580693842743074, 4.222088520697473868, -2.276242723817686997 ) ) ;
#5190=CARTESIAN_POINT ( 'NONE',  ( -2.146602167848374432, 116.4048268131027868, -0.3314024647271391899 ) ) ;
#5194=CARTESIAN_POINT ( 'NONE',  ( -5.224212249200172131, -8.128124378088662283, -6.605211778952579493 ) ) ;
#5195=CARTESIAN_POINT ( 'NONE',  ( 3.904803215525951554, 118.1588881757245986, 0.7354103002220402363 ) ) ;
#5198=CARTESIAN_POINT ( 'NONE',  ( 0.3199181899538769414, 107.4969721965504021, -4.676354563382915330 ) ) ;
#5199=CARTESIAN_POINT ( 'NONE',  ( -16.72896750809251998, 155.2649736186859570, 0.2017331744915137337 ) ) ;
#5204=CARTESIAN_POINT ( 'NONE',  ( -2.884051542275779756, 156.0957788938021054, -0.05763021347587621995 ) ) ;
#5205=CARTESIAN_POINT ( 'NONE',  ( 5.510877305967752271, -15.11690630435501248, 2.581843384194929758 ) ) ;
#5206=CARTESIAN_POINT ( 'NONE',  ( -13.31748376333910322, 121.6721647909590303, 1.150164054616430676 ) ) ;
#5207=CARTESIAN_POINT ( 'NONE',  ( 21.76596270643820219, 150.3096123636779566, -1.000581967439477138 ) ) ;
#5208=CARTESIAN_POINT ( 'NONE',  ( -3.789191232057584902, 13.46218022696137773, 2.646434746401360893 ) ) ;
#5209=CARTESIAN_POINT ( 'NONE',  ( -23.32660363739045906, 146.7646281656787437, -0.9249455126139313199 ) ) ;
#5213=CARTESIAN_POINT ( 'NONE',  ( -2.183349241107786387, 116.1870506606769311, -0.03693642060881925648 ) ) ;
#5215=CARTESIAN_POINT ( 'NONE',  ( -10.94646760555361276, 123.1276765127550021, 1.119819633367153289 ) ) ;
#5217=CARTESIAN_POINT ( 'NONE',  ( 4.191956958763752183, 119.0775769483117870, -0.8365378509937176910 ) ) ;
#5218=CARTESIAN_POINT ( 'NONE',  ( -13.51395941584921268, 155.6725583577350278, -2.021746995258101975 ) ) ;
#5220=EDGE_CURVE ( 'NONE', #12023, #39424, #37016, .T. ) ;
#5221=CARTESIAN_POINT ( 'NONE',  ( 3.160209531530921545, 156.1781389015385457, -0.7303267873898456886 ) ) ;
#5223=CARTESIAN_POINT ( 'NONE',  ( -5.349253755625555939, 156.5090806470891209, -1.752114854137454492 ) ) ;
#5224=CARTESIAN_POINT ( 'NONE',  ( 3.048550003781630213, -15.65190959513015834, 4.520219006486421165 ) ) ;
#5225=CARTESIAN_POINT ( 'NONE',  ( -4.452087279397210828, 118.1112359772488105, -0.7572249732135748479 ) ) ;
#5227=CARTESIAN_POINT ( 'NONE',  ( -4.890164892654324191, 117.4101971730238461, 0.9753743779596022456 ) ) ;
#5228=CARTESIAN_POINT ( 'NONE',  ( 12.25802010074268722, 153.5964916033214820, 2.078998712700113938 ) ) ;
#5229=CARTESIAN_POINT ( 'NONE',  ( 5.332935397695207413, 50.63946620154572997, 0.1065647409268298818 ) ) ;
#5230=CARTESIAN_POINT ( 'NONE',  ( -8.364652471777612064, 2.666895906452835252, -0.9765287277423425616 ) ) ;
#5231=CARTESIAN_POINT ( 'NONE',  ( 15.79012389680288564, 146.9282941555416073, 0.7681517710631365903 ) ) ;
#5236=CARTESIAN_POINT ( 'NONE',  ( -1.144332903081027197, 117.3993836041148597, 1.432019610544279509 ) ) ;
#5240=CARTESIAN_POINT ( 'NONE',  ( -23.33610279681233379, 149.0590277239482475, -0.3121099645145853363 ) ) ;
#5241=VERTEX_POINT ( 'NONE', #23158 ) ;
#5243=CARTESIAN_POINT ( 'NONE',  ( -6.895199152412361698, 121.8168396766305079, -0.5159271962741722728 ) ) ;
#5246=CARTESIAN_POINT ( 'NONE',  ( 0.2391656075941314130, 115.7030485030756637, -1.756104538880229438 ) ) ;
#5247=CARTESIAN_POINT ( 'NONE',  ( -4.547323659248203143, 121.1438296405421937, -0.2486498796252667176 ) ) ;
#5248=CARTESIAN_POINT ( 'NONE',  ( 4.521557965551993519, -14.38033123432501448, 4.565926699156682922 ) ) ;
#5249=CARTESIAN_POINT ( 'NONE',  ( -15.47853073355919840, 123.0316835747794642, 0.9738675477772638089 ) ) ;
#5250=AXIS2_PLACEMENT_3D ( 'NONE', #29878, #716, #26681 ) ;
#5251=CARTESIAN_POINT ( 'NONE',  ( 4.016744494447205049, 117.3993836135117732, -1.174929138160409448 ) ) ;
#5252=CARTESIAN_POINT ( 'NONE',  ( 23.34743456777619386, 142.7586093370927074, 0.6964168797349272744 ) ) ;
#5253=CARTESIAN_POINT ( 'NONE',  ( 6.506917054590420690, 121.7798191776175685, 0.1679176037484078621 ) ) ;
#5254=CARTESIAN_POINT ( 'NONE',  ( -4.977848145772336252, 117.5941869881971655, 0.7723625501233751800 ) ) ;
#5255=CARTESIAN_POINT ( 'NONE',  ( -0.09387087892865565719, 20.69761720779959902, -0.9769954323643923466 ) ) ;
#5256=CARTESIAN_POINT ( 'NONE',  ( -5.779653879267294236, 116.9360814311326777, -0.1581498910197087771 ) ) ;
#5258=EDGE_CURVE ( 'NONE', #41397, #9260, #16575, .T. ) ;
#5261=CARTESIAN_POINT ( 'NONE',  ( 3.533749852891390208, 117.8629878115362715, 0.8862737175697782410 ) ) ;
#5263=CARTESIAN_POINT ( 'NONE',  ( 9.950292893259801374, 157.6892375622926181, 1.550998551202242615 ) ) ;
#5265=CIRCLE ( 'NONE', #24969, 0.5080000000000002292 ) ;
#5266=CARTESIAN_POINT ( 'NONE',  ( 18.00466200016590435, 151.7072807693909340, -1.676127293294198628 ) ) ;
#5267=CARTESIAN_POINT ( 'NONE',  ( -7.601118931484537100, 27.11072341857771306, -3.643763446188946542 ) ) ;
#5268=CARTESIAN_POINT ( 'NONE',  ( -22.03343284943311176, 146.2042277794223537, -2.039575571141828192 ) ) ;
#5269=CARTESIAN_POINT ( 'NONE',  ( 4.810014216029472323, 117.7355684663886137, -0.8789097560846608204 ) ) ;
#5271=CARTESIAN_POINT ( 'NONE',  ( 1.375939976466430181, 106.2431249238853894, 5.170880015306797084 ) ) ;
#5274=CARTESIAN_POINT ( 'NONE',  ( -13.61628268276122178, 150.2179846313823930, -0.04905232040057764392 ) ) ;
#5275=CARTESIAN_POINT ( 'NONE',  ( -19.45004534592214185, 148.0998626603252148, -2.515250464377976947 ) ) ;
#5276=CARTESIAN_POINT ( 'NONE',  ( 6.296695397805594396, -14.23921929796089003, 0.5540845800015932188 ) ) ;
#5277=CARTESIAN_POINT ( 'NONE',  ( -3.361735136380934019, 117.3993835122084590, -1.373601552275676596 ) ) ;
#5280=CARTESIAN_POINT ( 'NONE',  ( 8.582646176847930519, 120.3810071108087243, 1.481269161951472624 ) ) ;
#5281=CARTESIAN_POINT ( 'NONE',  ( -3.174366308152013261, 91.02546620154572565, -0.06343139340882732180 ) ) ;
#5282=CARTESIAN_POINT ( 'NONE',  ( -5.341065829615910587, 115.6909491485453003, 0.1995911688841381648 ) ) ;
#5283=TOROIDAL_SURFACE ( 'NONE', #29068, 5.080000000000005400, 0.5080000000000000071 ) ;
#5284=CARTESIAN_POINT ( 'NONE',  ( -2.312669815851230659, 124.5312663981120380, -0.02133033151766248331 ) ) ;
#5285=CARTESIAN_POINT ( 'NONE',  ( -7.766292583485225443, -1.596223907437250844, -3.263082884517814364 ) ) ;
#5286=CARTESIAN_POINT ( 'NONE',  ( 3.609032566395310671, 120.7384399880717467, 0.4518473439704071004 ) ) ;
#5287=DIRECTION ( 'NONE',  ( -4.017660918040594346E-17, 1.000000000000000000, 2.376309959284834438E-19 ) ) ;
#5288=CARTESIAN_POINT ( 'NONE',  ( 5.848384816632722583, 117.2350771734024164, -0.3616545339607747933 ) ) ;
#5293=CARTESIAN_POINT ( 'NONE',  ( 1.826496821415122707, -15.21410320048187970, 5.439012564009858330 ) ) ;
#5294=CARTESIAN_POINT ( 'NONE',  ( -4.166291299642304047, 118.2394655740918097, 0.2241564256093856733 ) ) ;
#5299=CARTESIAN_POINT ( 'NONE',  ( 4.179037867723048194, 119.2769959767378651, -0.7610518346563297509 ) ) ;
#5300=CARTESIAN_POINT ( 'NONE',  ( -4.705839724742440389, 116.0444662015457595, 3.565396701626624143 ) ) ;
#5301=CARTESIAN_POINT ( 'NONE',  ( 4.237069621333032110, 118.2250994327943943, 0.4770513927000196164 ) ) ;
#5302=CARTESIAN_POINT ( 'NONE',  ( -15.52857178871880883, 148.0963874134046705, -1.155438959258076936 ) ) ;
#5304=CARTESIAN_POINT ( 'NONE',  ( 3.703049682113265018, 116.6240124373522065, 0.07399574541707873432 ) ) ;
#5305=ADVANCED_FACE ( 'NONE', ( #19549, #3180 ), #38542, .F. ) ;
#5306=ORIENTED_EDGE ( 'NONE', *, *, #30088, .F. ) ;
#5307=CARTESIAN_POINT ( 'NONE',  ( 2.889066315880882030, 25.55657059589919911, 3.609430016826872478 ) ) ;
#5311=CARTESIAN_POINT ( 'NONE',  ( 6.079341768894599873, 121.3741006014788724, 0.4360735354898734317 ) ) ;
#5312=CARTESIAN_POINT ( 'NONE',  ( 2.838909340336904563, 21.51804255560577772, 3.663749385350952181 ) ) ;
#5313=CARTESIAN_POINT ( 'NONE',  ( 15.38106892591210872, 121.3506620944898060, 1.079669858139658434 ) ) ;
#5314=CARTESIAN_POINT ( 'NONE',  ( 3.570581317670051380, 104.6144662015457243, -3.261568590886288810 ) ) ;
#5315=CARTESIAN_POINT ( 'NONE',  ( 2.971193505762239617, -14.05637172046637851, 0.8995351626913862253 ) ) ;
#5316=CARTESIAN_POINT ( 'NONE',  ( 3.087569247026485275, 117.8293475852256904, -0.6612947004247918814 ) ) ;
#5317=CARTESIAN_POINT ( 'NONE',  ( -1.363824289596636374, 119.4570717772418220, 0.5813626927913073672 ) ) ;
#5318=CARTESIAN_POINT ( 'NONE',  ( -2.394960105286914942, 16.54535949628658997, -3.951836011466995036 ) ) ;
#5319=CARTESIAN_POINT ( 'NONE',  ( -1.907136510351378655, 116.7789519286944966, -0.3469662120689607776 ) ) ;
#5320=CARTESIAN_POINT ( 'NONE',  ( -0.6881565663083963891, 18.49284505249605459, 0.6899137464212180548 ) ) ;
#5321=ORIENTED_EDGE ( 'NONE', *, *, #29282, .F. ) ;
#5323=CARTESIAN_POINT ( 'NONE',  ( -3.061305989504190972, 156.1243923452879017, 0.5262318146843659727 ) ) ;
#5324=CARTESIAN_POINT ( 'NONE',  ( 5.272318886577700425, -12.73938755324596706, 2.198237985477529577 ) ) ;
#5325=CARTESIAN_POINT ( 'NONE',  ( 0.5597765207467094717, 119.9180165495073283, -0.4599786748625143695 ) ) ;
#5326=VERTEX_POINT ( 'NONE', #3612 ) ;
#5327=CARTESIAN_POINT ( 'NONE',  ( 0.9215934890950072678, 115.7029463657684829, 1.750466622602536493 ) ) ;
#5328=CARTESIAN_POINT ( 'NONE',  ( -4.777110523374184403, 117.8777403950456062, -0.8659071637066898530 ) ) ;
#5329=CARTESIAN_POINT ( 'NONE',  ( 0.0005023639977465172704, 120.9974662015457056, -0.02514034870427557522 ) ) ;
#5331=CARTESIAN_POINT ( 'NONE',  ( 16.68944084648531501, 128.5636217276695561, 2.149857652400631203 ) ) ;
#5334=CARTESIAN_POINT ( 'NONE',  ( 0.03212616895145502249, 157.6269964811067155, -1.607724863813388971 ) ) ;
#5336=CARTESIAN_POINT ( 'NONE',  ( 23.25176476241877310, 142.6711341654318801, 0.007203867522444172208 ) ) ;
#5339=CARTESIAN_POINT ( 'NONE',  ( 1.868973561629162061, -15.15741002263305859, 5.907646661756425388 ) ) ;
#5340=CARTESIAN_POINT ( 'NONE',  ( -5.332935397695334423, 51.14746620154573264, -0.1065647409268298818 ) ) ;
#5342=CARTESIAN_POINT ( 'NONE',  ( -4.646523143152131219, 117.9818477556987943, 0.7218086234193739070 ) ) ;
#5345=CARTESIAN_POINT ( 'NONE',  ( -0.2209998912935267623, 118.7629491485454025, 1.272056456734703245 ) ) ;
#5346=ADVANCED_FACE ( 'NONE', ( #19598 ), #32353, .T. ) ;
#5347=CARTESIAN_POINT ( 'NONE',  ( -5.811960698193874286, 118.8837068780349142, -1.247592088532381460 ) ) ;
#5348=CARTESIAN_POINT ( 'NONE',  ( -6.804471202056847190, 123.7298400107579255, -0.1732695889264300182 ) ) ;
#5349=CARTESIAN_POINT ( 'NONE',  ( 4.730984371466873561, 117.6315449097853048, 1.144802877355001192 ) ) ;
#5351=CARTESIAN_POINT ( 'NONE',  ( -0.7718547489771787617, 119.9044272045951374, 0.6164056859965566515 ) ) ;
#5352=CARTESIAN_POINT ( 'NONE',  ( 2.294499597581835193, -9.852027417895397932, -4.012603411698490774 ) ) ;
#5356=CARTESIAN_POINT ( 'NONE',  ( 3.206936388013850614, -12.21552616865279006, 0.5380348851386724807 ) ) ;
#5357=CARTESIAN_POINT ( 'NONE',  ( 1.980640663884704722, 106.8720524443079967, -4.823141945187445323 ) ) ;
#5359=CARTESIAN_POINT ( 'NONE',  ( -6.441001096823943506, 29.32969738650800551, -0.01017983961634277151 ) ) ;
#5360=DIRECTION ( 'NONE',  ( -4.017660918040594346E-17, 1.000000000000000000, 2.376309959284834438E-19 ) ) ;
#5361=CARTESIAN_POINT ( 'NONE',  ( -0.2084201458593382406, 5.265951782950084592, 4.622859108429906883 ) ) ;
#5362=CARTESIAN_POINT ( 'NONE',  ( 5.654702199549676678, 159.1134716836843381, 0.5125381600378310365 ) ) ;
#5363=EDGE_LOOP ( 'NONE', ( #4322, #31448, #25073, #34490 ) ) ;
#5364=CARTESIAN_POINT ( 'NONE',  ( 1.753713527278395468, 104.6144662015458096, -4.497131813391320954 ) ) ;
#5365=CARTESIAN_POINT ( 'NONE',  ( 2.557542807212066283, -15.51814986354871451, 4.851437248720891660 ) ) ;
#5366=CARTESIAN_POINT ( 'NONE',  ( -19.22350799451007575, 148.9694856701144090, 1.735702374547824389 ) ) ;
#5368=CARTESIAN_POINT ( 'NONE',  ( -0.9749442489646007459, 26.91501818708639249, 0.01812370653153724809 ) ) ;
#5369=CARTESIAN_POINT ( 'NONE',  ( 0.6724949529566155437, 16.91434809748496804, 0.7070771739444717818 ) ) ;
#5373=CARTESIAN_POINT ( 'NONE',  ( 3.315449255180855204, 124.9344662015457743, 0.06625056644921942239 ) ) ;
#5374=CARTESIAN_POINT ( 'NONE',  ( -5.877307974080659747, 120.8872308857076519, 0.5842564153471766497 ) ) ;
#5376=CARTESIAN_POINT ( 'NONE',  ( 1.928300050954173450, -15.05328954375542772, 5.649432967411273765 ) ) ;
#5377=CARTESIAN_POINT ( 'NONE',  ( 5.091199858995886451, 119.8577235299091228, -0.8121313320900890309 ) ) ;
#5378=CARTESIAN_POINT ( 'NONE',  ( -13.90099558903415478, 123.5874490550988014, -1.899532866591826519 ) ) ;
#5380=CARTESIAN_POINT ( 'NONE',  ( -0.02896191955447584981, 39.05846921699762220, 0.8727513426688231490 ) ) ;
#5381=CARTESIAN_POINT ( 'NONE',  ( 9.439772580079011988, 124.2753396726362780, -0.1368060863603346999 ) ) ;
#5382=VERTEX_POINT ( 'NONE', #19760 ) ;
#5383=CARTESIAN_POINT ( 'NONE',  ( 3.220686968960577712, -14.48737495597347902, 2.486805533510040078 ) ) ;
#5387=CARTESIAN_POINT ( 'NONE',  ( 4.999358879416575974, 117.3993846089301911, 0.8254721163526904659 ) ) ;
#5389=CARTESIAN_POINT ( 'NONE',  ( -3.339653329301207840, -2.245917679271888900, -3.199182135983138053 ) ) ;
#5390=CARTESIAN_POINT ( 'NONE',  ( 10.39772550536720885, 123.9810924921358151, 1.245468829273463474 ) ) ;
#5391=CARTESIAN_POINT ( 'NONE',  ( -3.312261290190312568, 29.35545767321095667, 2.878016369877077985 ) ) ;
#5392=CARTESIAN_POINT ( 'NONE',  ( -5.205184729905311336, 115.4673366222922368, 1.303740999714490201 ) ) ;
#5393=CARTESIAN_POINT ( 'NONE',  ( 0.09481320634720795393, -4.229605868409334057, 4.636458411128852930 ) ) ;
#5394=CARTESIAN_POINT ( 'NONE',  ( 8.487687333566158898, 123.3253871723413368, 0.1696041924978713422 ) ) ;
#5395=CARTESIAN_POINT ( 'NONE',  ( 3.645047284007026267, 5.522537913078280347, -7.602695550683356451 ) ) ;
#5397=CARTESIAN_POINT ( 'NONE',  ( -2.141217111143084217, 116.5628937121521176, -0.4137402603370525234 ) ) ;
#5398=CARTESIAN_POINT ( 'NONE',  ( -0.1292312685654156412, 109.4728569552520554, -3.923176234211465552 ) ) ;
#5400=CARTESIAN_POINT ( 'NONE',  ( -7.992722778381481596, -7.251515252772184894, -2.728257467986670903 ) ) ;
#5402=CARTESIAN_POINT ( 'NONE',  ( 1.957861286920753674, 117.9394489915384270, 1.364553959153947282 ) ) ;
#5405=CARTESIAN_POINT ( 'NONE',  ( 0.4040709798585657153, 123.7646714092001190, -0.1152108919326050862 ) ) ;
#5406=CARTESIAN_POINT ( 'NONE',  ( -23.05883864707335817, 142.5499849734818838, 0.2756568390806650726 ) ) ;
#5407=ORIENTED_EDGE ( 'NONE', *, *, #15141, .F. ) ;
#5411=DIRECTION ( 'NONE',  ( -0.01997839162482737546, -1.040247600000940825E-18, 0.9998004120163610509 ) ) ;
#5412=CARTESIAN_POINT ( 'NONE',  ( -8.741281759966728515, 123.6764614546807621, -0.1311366048815914842 ) ) ;
#5413=CARTESIAN_POINT ( 'NONE',  ( 6.479796796485603139, -13.80134569450770776, 0.08439370571411514144 ) ) ;
#5414=CARTESIAN_POINT ( 'NONE',  ( -15.00359386227412273, 154.7288491705591866, 1.534247969496847386 ) ) ;
#5415=CARTESIAN_POINT ( 'NONE',  ( 17.95360460524294410, 154.0540368679750998, -0.8775891217286382329 ) ) ;
#5416=CARTESIAN_POINT ( 'NONE',  ( 3.874746376330849618, 18.20996518813934628, -2.522041008920607563 ) ) ;
#5417=CARTESIAN_POINT ( 'NONE',  ( -0.3142790036447159485, 116.6413645472259617, -0.2007485675953368798 ) ) ;
#5420=CARTESIAN_POINT ( 'NONE',  ( 5.560951712478671816, 116.7029514248484929, 0.1869645659760804934 ) ) ;
#5422=CARTESIAN_POINT ( 'NONE',  ( -17.22187362939842359, 148.7218176724978775, 1.531815132551777259 ) ) ;
#5424=CARTESIAN_POINT ( 'NONE',  ( 19.29290905409789758, 147.1635184732690220, -1.739861672056419506 ) ) ;
#5425=CARTESIAN_POINT ( 'NONE',  ( -21.10215338253927797, 147.9292434580435724, -2.361242315759020993 ) ) ;
#5427=CARTESIAN_POINT ( 'NONE',  ( 15.90968206782430983, 148.0001117310855250, -0.7891277450764202506 ) ) ;
#5429=CARTESIAN_POINT ( 'NONE',  ( -8.234130529647242014, 121.1361926620737393, -1.330377128061139835 ) ) ;
#5430=CARTESIAN_POINT ( 'NONE',  ( 1.868457900240735103, -15.55086107261449690, 5.421086310357067894 ) ) ;
#5431=CARTESIAN_POINT ( 'NONE',  ( -4.065972646788793554, 118.2429491485453070, -0.3080848862740693250 ) ) ;
#5433=CIRCLE ( 'NONE', #29220, 0.5080000000000002292 ) ;
#5434=CARTESIAN_POINT ( 'NONE',  ( -4.792200577477630397, 117.5371802918334225, 0.9878184568134641408 ) ) ;
#5435=CARTESIAN_POINT ( 'NONE',  ( 5.074328365123657925, 120.0747842884402132, 0.9638994778299828647 ) ) ;
#5436=PLANE ( 'NONE',  #21230 ) ;
#5438=CARTESIAN_POINT ( 'NONE',  ( -5.377075248297400911, 4.191758615746518757, 6.528609652590111168 ) ) ;
#5439=CARTESIAN_POINT ( 'NONE',  ( 5.911602206138902638, 121.5031286879076902, 0.2921876764073587651 ) ) ;
#5447=CARTESIAN_POINT ( 'NONE',  ( -0.001838942458917565501, 116.4858755864912183, 0.09202820039585841994 ) ) ;
#5448=ORIENTED_EDGE ( 'NONE', *, *, #10739, .F. ) ;
#5450=CARTESIAN_POINT ( 'NONE',  ( -6.877540358266958975, 121.7309737470392434, -0.6052161323226827871 ) ) ;
#5451=CARTESIAN_POINT ( 'NONE',  ( -7.794969618782333853, 122.5994144667442498, -0.004875387122262515339 ) ) ;
#5453=CARTESIAN_POINT ( 'NONE',  ( 0.03523692298162432734, 115.6909491485452719, -1.763399716048400734 ) ) ;
#5454=CARTESIAN_POINT ( 'NONE',  ( -9.153275543502907396, 153.8946005065304803, -0.4698995960908562419 ) ) ;
#5455=CARTESIAN_POINT ( 'NONE',  ( 5.856266048228023990, -12.49204451700697227, 1.108958003446382845 ) ) ;
#5456=CARTESIAN_POINT ( 'NONE',  ( -21.26362230212582816, 150.1117090729339623, 1.276404781699089996 ) ) ;
#5458=CARTESIAN_POINT ( 'NONE',  ( 15.84538651563799050, 121.0146182718019645, 0.4760991727851862088 ) ) ;
#5459=CARTESIAN_POINT ( 'NONE',  ( 15.76023951477780294, 145.9043208129480433, 0.3821549961928484840 ) ) ;
#5461=CARTESIAN_POINT ( 'NONE',  ( -0.009113691291695666039, 25.33460033795575583, 0.9756159547818916700 ) ) ;
#5462=CARTESIAN_POINT ( 'NONE',  ( -4.723387343850809827, 116.7592613395855352, -0.1361797943638454467 ) ) ;
#5464=TOROIDAL_SURFACE ( 'NONE', #14946, 3.683000000000000718, 0.5080000000000000071 ) ;
#5467=CARTESIAN_POINT ( 'NONE',  ( -6.079585152903477230, 118.8420829952417535, 0.9834774059785402756 ) ) ;
#5468=CARTESIAN_POINT ( 'NONE',  ( -3.942997264624582776, -11.51663297089948479, -2.426127359622226809 ) ) ;
#5469=CARTESIAN_POINT ( 'NONE',  ( 20.86915823776852008, 136.4823663107028722, 1.950121757083878249 ) ) ;
#5470=CARTESIAN_POINT ( 'NONE',  ( 20.39294766749429755, 148.4497675966422889, -1.664483663417329673 ) ) ;
#5471=CARTESIAN_POINT ( 'NONE',  ( -8.001679540263406665, 18.69059125004590172, 2.668541714186715819 ) ) ;
#5472=CARTESIAN_POINT ( 'NONE',  ( -1.281755300609965120, 159.3505072347868747, -0.9987438389826045482 ) ) ;
#5473=CARTESIAN_POINT ( 'NONE',  ( 4.932541054738843300, 117.5465815472490192, -0.8858376886457886012 ) ) ;
#5474=CARTESIAN_POINT ( 'NONE',  ( 7.474242191267162383, 123.6620266863018855, 0.1838331482465498379 ) ) ;
#5476=CARTESIAN_POINT ( 'NONE',  ( -6.497458072406325336, 121.7745328324513139, -0.05723077286956937404 ) ) ;
#5477=CARTESIAN_POINT ( 'NONE',  ( -18.98749958112902902, 148.5750135429820205, -2.495758040776018927 ) ) ;
#5478=CARTESIAN_POINT ( 'NONE',  ( 5.316001070410483642, -15.20466279102368468, 3.045604417706107458 ) ) ;
#5480=AXIS2_PLACEMENT_3D ( 'NONE', #19956, #36168, #15913 ) ;
#5483=CARTESIAN_POINT ( 'NONE',  ( 11.65353862096119641, 154.7938929448963279, 2.201148936174281534 ) ) ;
#5486=DIRECTION ( 'NONE',  ( 4.017660918040594346E-17, -1.000000000000000000, -2.376309959284834438E-19 ) ) ;
#5487=CARTESIAN_POINT ( 'NONE',  ( -2.102284131448474369, 122.9394440205640961, 0.1126375150955782195 ) ) ;
#5488=CARTESIAN_POINT ( 'NONE',  ( -0.5966991250155297966, -8.296908750894687046, 8.413794654835093922 ) ) ;
#5489=CARTESIAN_POINT ( 'NONE',  ( 0.6895396258585522187, 156.3865044363621450, 0.6062415235663760615 ) ) ;
#5490=CARTESIAN_POINT ( 'NONE',  ( -5.219367156868218061, 115.6909491485453003, -1.134611224921844963 ) ) ;
#5491=CARTESIAN_POINT ( 'NONE',  ( 3.184986510633057488, 159.3937097445585778, -0.5650791069852592052 ) ) ;
#5494=CARTESIAN_POINT ( 'NONE',  ( 8.798408771645801707, 117.6899328986124402, 0.1004551508774383928 ) ) ;
#5498=CARTESIAN_POINT ( 'NONE',  ( 2.083301838685657881, -15.46665383083971790, 5.961979448439958418 ) ) ;
#5499=CARTESIAN_POINT ( 'NONE',  ( -4.239777078203335492, 118.2238256456127061, 0.3214240529150897974 ) ) ;
#5500=CARTESIAN_POINT ( 'NONE',  ( -15.73471677569744287, 120.8416612192341972, -0.3144170877231853845 ) ) ;
#5503=CARTESIAN_POINT ( 'NONE',  ( -4.317885076038099790, 119.4472151493546761, -0.9270640149902646954 ) ) ;
#5505=CARTESIAN_POINT ( 'NONE',  ( -10.15204665306235476, 124.8647468421599598, -0.8418846390287857417 ) ) ;
#5508=CARTESIAN_POINT ( 'NONE',  ( 0.2378307671391127198, 117.3993841993812453, -1.487622118729645893 ) ) ;
#5509=ORIENTED_EDGE ( 'NONE', *, *, #9443, .T. ) ;
#5510=CARTESIAN_POINT ( 'NONE',  ( -3.130497002865707312, 23.39511390029671745, 3.426874451367011520 ) ) ;
#5515=CARTESIAN_POINT ( 'NONE',  ( -7.786259069948810563, 122.6240336826886050, -0.1181640060794083291 ) ) ;
#5517=CARTESIAN_POINT ( 'NONE',  ( 20.20545065706713572, 152.4988772720997190, 1.451042778694937585 ) ) ;
#5518=CARTESIAN_POINT ( 'NONE',  ( 4.722155446386091526, 104.6144662015456817, -1.045890991608505960 ) ) ;
#5519=CARTESIAN_POINT ( 'NONE',  ( 3.221942100833175893, -14.53498920702628361, 2.661941298785070575 ) ) ;
#5520=CARTESIAN_POINT ( 'NONE',  ( 18.85936551755639101, 131.8417273817641444, -1.350502370828212229 ) ) ;
#5522=CARTESIAN_POINT ( 'NONE',  ( -0.5282936316508035635, 119.4440140289964774, 0.5434071943388012471 ) ) ;
#5523=CARTESIAN_POINT ( 'NONE',  ( 3.724956840101937505, 21.94285949141939440, 2.734508905299370518 ) ) ;
#5524=CARTESIAN_POINT ( 'NONE',  ( -18.24338043389154507, 154.1370782493726210, -1.275500441016771402 ) ) ;
#5525=CARTESIAN_POINT ( 'NONE',  ( -0.8533247626149625953, -2.668348290978065140, -0.4694259674561338525 ) ) ;
#5526=ORIENTED_EDGE ( 'NONE', *, *, #16135, .T. ) ;
#5528=CARTESIAN_POINT ( 'NONE',  ( -15.50313878892752939, 143.5853813351167219, 0.4270882868188066173 ) ) ;
#5529=CARTESIAN_POINT ( 'NONE',  ( 5.396235140300779776, -11.83248475511457976, 0.6634469457710948648 ) ) ;
#5530=CARTESIAN_POINT ( 'NONE',  ( 12.65121035427608298, 128.4643691153342218, -0.9906145297030367614 ) ) ;
#5532=CARTESIAN_POINT ( 'NONE',  ( 0.5744245648901143975, 115.7029491485453718, 1.760676250340797777 ) ) ;
#5533=CARTESIAN_POINT ( 'NONE',  ( -4.860056194691428466, 117.7242711327382239, -0.9629742322061086712 ) ) ;
#5534=EDGE_CURVE ( 'NONE', #32767, #27965, #19456, .T. ) ;
#5535=CARTESIAN_POINT ( 'NONE',  ( 7.788912029362537126, 154.6472212274131550, 0.1129171994251849803 ) ) ;
#5537=CARTESIAN_POINT ( 'NONE',  ( 19.91185195753428516, 145.3736917597469471, 2.515063280254572042 ) ) ;
#5539=FACE_OUTER_BOUND ( 'NONE', #28619, .T. ) ;
#5542=CARTESIAN_POINT ( 'NONE',  ( 22.80463473692766740, 150.3987591554885626, 0.1267456695372862208 ) ) ;
#5544=CIRCLE ( 'NONE', #24577, 5.588000000000006295 ) ;
#5546=CARTESIAN_POINT ( 'NONE',  ( 1.717835917352494635, -15.15497214477301569, 5.627788587114283203 ) ) ;
#5547=CYLINDRICAL_SURFACE ( 'NONE', #26967, 3.175000000000001155 ) ;
#5550=CARTESIAN_POINT ( 'NONE',  ( -4.706501277415600981, 117.8934301135909095, 0.8007959269290801929 ) ) ;
#5553=DIRECTION ( 'NONE',  ( -0.9998004120163608288, -4.016384292689131511E-17, -0.01997839162482749342 ) ) ;
#5554=CARTESIAN_POINT ( 'NONE',  ( 5.779644130035700655, 118.6808122264324084, -0.9965243451110286088 ) ) ;
#5555=CARTESIAN_POINT ( 'NONE',  ( 0.1065646865915093333, 105.8844662015456777, -5.332932678536312032 ) ) ;
#5556=CARTESIAN_POINT ( 'NONE',  ( 4.842532773218567677, 117.4782487948497902, 1.162086725208648863 ) ) ;
#5559=CARTESIAN_POINT ( 'NONE',  ( -0.3839444928497607878, 119.8383472832136931, 0.6866461459122013000 ) ) ;
#5560=CARTESIAN_POINT ( 'NONE',  ( 4.560200836559435977, -11.68919918208664122, 0.6963878748952898601 ) ) ;
#5561=CARTESIAN_POINT ( 'NONE',  ( 3.682264917456191888, 97.37546620154573418, 0.07358041635424013294 ) ) ;
#5562=CARTESIAN_POINT ( 'NONE',  ( 0.1116392523994730462, 39.20946620154573736, -5.586884702347429510 ) ) ;
#5563=CARTESIAN_POINT ( 'NONE',  ( 1.897380780832740532, -15.05783359004129984, 5.662421594695133287 ) ) ;
#5564=CARTESIAN_POINT ( 'NONE',  ( 5.756868464772053606, 120.3160329940760818, -0.2053529492706007153 ) ) ;
#5565=CARTESIAN_POINT ( 'NONE',  ( -5.103418814394366620, 120.3680889145531552, -0.8767301089910150003 ) ) ;
#5567=CARTESIAN_POINT ( 'NONE',  ( -6.067023846813282439, 121.4357121891808191, -0.1206843736590161587 ) ) ;
#5568=DIRECTION ( 'NONE',  ( 4.017660918040594346E-17, -1.000000000000000000, -2.376309959284834438E-19 ) ) ;
#5569=CARTESIAN_POINT ( 'NONE',  ( 2.003160574663116034, 15.61121511114846960, 4.187759092076685619 ) ) ;
#5570=CARTESIAN_POINT ( 'NONE',  ( 22.96526709448173165, 149.8455236008688303, 1.052246632350672950 ) ) ;
#5572=CARTESIAN_POINT ( 'NONE',  ( -0.8085285286411788563, 104.6144662015543361, -5.283841362478505665 ) ) ;
#5573=CARTESIAN_POINT ( 'NONE',  ( 2.429471885602138670, -15.51652123318236676, 4.968198114871331228 ) ) ;
#5574=CARTESIAN_POINT ( 'NONE',  ( -11.67114148714794730, 122.1450671466348439, 1.284540048876763096 ) ) ;
#5575=AXIS2_PLACEMENT_3D ( 'NONE', #8731, #21693, #25336 ) ;
#5576=CARTESIAN_POINT ( 'NONE',  ( -0.3022039251088723399, 24.96921649940425425, -0.9259629999792299282 ) ) ;
#5578=CARTESIAN_POINT ( 'NONE',  ( -0.6941440390767986690, 12.16465383894776409, -0.6855803344193639459 ) ) ;
#5582=CARTESIAN_POINT ( 'NONE',  ( 5.854942301702412699, 124.9344662015456890, 0.1169956811762814242 ) ) ;
#5584=CARTESIAN_POINT ( 'NONE',  ( -16.26403174311784028, 147.1082353761072454, 0.7878939306839422008 ) ) ;
#5585=ADVANCED_FACE ( 'NONE', ( #16474, #39495 ), #32678, .F. ) ;
#5587=CARTESIAN_POINT ( 'NONE',  ( 3.722123463297008605, -13.62806973238828157, 3.608531954378976891 ) ) ;
#5588=CARTESIAN_POINT ( 'NONE',  ( 15.69153790699141027, 150.8349565870724120, -1.587821608835076503 ) ) ;
#5590=CARTESIAN_POINT ( 'NONE',  ( -16.68944084648544646, 128.5636217276695561, -2.149857652400630759 ) ) ;
#5592=CARTESIAN_POINT ( 'NONE',  ( -12.85860202769644545, 133.7716054015561156, -0.2569454702854385153 ) ) ;
#5593=CARTESIAN_POINT ( 'NONE',  ( 4.074910602682932925, 118.2429491485453354, -0.1454311599470142491 ) ) ;
#5594=CARTESIAN_POINT ( 'NONE',  ( 9.317815699932298301, 124.0984330410602183, -0.1356161447201455761 ) ) ;
#5596=CARTESIAN_POINT ( 'NONE',  ( 2.459637058406862309, -15.11974833578012856, 4.824092508607692231 ) ) ;
#5602=CARTESIAN_POINT ( 'NONE',  ( 0.2036312542886812293, -3.545347522689146214, -4.628372119175537591 ) ) ;
#5603=CARTESIAN_POINT ( 'NONE',  ( 16.42797441217041765, 147.8801373804967341, 1.766026403434534098 ) ) ;
#5605=CARTESIAN_POINT ( 'NONE',  ( -2.668012146925317740, 107.2306503360107541, 4.624472725681509466 ) ) ;
#5607=CARTESIAN_POINT ( 'NONE',  ( -4.550674770548566173, 2.667180226961371137, -0.8080508602523945871 ) ) ;
#5608=CARTESIAN_POINT ( 'NONE',  ( 5.308493528853203358, 121.3525139070573147, 0.1060763342189516983 ) ) ;
#5609=ADVANCED_FACE ( 'NONE', ( #39282 ), #39057, .T. ) ;
#5610=CARTESIAN_POINT ( 'NONE',  ( -7.571256676022106724, -0.2985773316772562525, 3.683590697331973196 ) ) ;
#5612=CARTESIAN_POINT ( 'NONE',  ( -2.148791889500600405, 116.6464491036702640, -0.4521275957688462022 ) ) ;
#5613=CARTESIAN_POINT ( 'NONE',  ( -1.058122102717379942, 124.9344662015457459, -0.02114379780294260366 ) ) ;
#5614=LINE ( 'NONE', #24534, #15098 ) ;
#5616=CARTESIAN_POINT ( 'NONE',  ( -8.268995186617910775, -7.056286353048313309, -1.660136952399225319 ) ) ;
#5617=CARTESIAN_POINT ( 'NONE',  ( 0.3344074102203439813, 117.9394486947857814, 1.410084100385009531 ) ) ;
#5620=CARTESIAN_POINT ( 'NONE',  ( 0.3781434503561393878, 120.9711055683163323, -0.4753422346318206815 ) ) ;
#5621=CARTESIAN_POINT ( 'NONE',  ( -16.81386451639902901, 122.6968688451475771, 0.2091777910580985833 ) ) ;
#5625=DIRECTION ( 'NONE',  ( 0.9998004120163608288, 4.016384292689131511E-17, 0.01997839162482749342 ) ) ;
#5626=CARTESIAN_POINT ( 'NONE',  ( -15.72656178636810331, 146.8976252942685505, -0.1802331088929658987 ) ) ;
#5627=CARTESIAN_POINT ( 'NONE',  ( 2.659284927817582744, -15.52939239755456136, 5.761088356787748666 ) ) ;
#5628=CARTESIAN_POINT ( 'NONE',  ( -3.179094171403719304, 118.3302933575512412, 0.7469981754565537813 ) ) ;
#5629=CARTESIAN_POINT ( 'NONE',  ( 1.068372181839128965, 117.3444111807523882, -0.4585463030235086834 ) ) ;
#5630=CARTESIAN_POINT ( 'NONE',  ( -2.359559261509405204, 14.11188314818778267, 3.974389579228013503 ) ) ;
#5631=CARTESIAN_POINT ( 'NONE',  ( -15.37635245578029419, 120.8297411738997624, -0.7275678838439406659 ) ) ;
#5635=CARTESIAN_POINT ( 'NONE',  ( -2.182332153758789417, 116.1897970675078255, -0.04360822100441016230 ) ) ;
#5637=CARTESIAN_POINT ( 'NONE',  ( -16.62515567699083618, 149.4842840675632658, 1.536177446654198198 ) ) ;
#5639=CARTESIAN_POINT ( 'NONE',  ( 0.03245814172805025488, 157.7902383798253538, -1.624338139048501439 ) ) ;
#5640=CARTESIAN_POINT ( 'NONE',  ( -12.91357091396832146, 121.2479969211051127, -1.612259173617573094 ) ) ;
#5643=CARTESIAN_POINT ( 'NONE',  ( 16.17714305270723685, 147.4171829256358137, -0.7878123557203797755 ) ) ;
#5646=CARTESIAN_POINT ( 'NONE',  ( -2.462641994822475144, 119.6096776070104681, -0.7191205607878169426 ) ) ;
#5647=CARTESIAN_POINT ( 'NONE',  ( 2.631420558634286255, -15.64638348417481062, 4.926794133592228064 ) ) ;
#5648=CARTESIAN_POINT ( 'NONE',  ( -4.113113975211506457, 118.2429491485453070, -0.3449889555224052717 ) ) ;
#5649=ADVANCED_FACE ( 'NONE', ( #29687 ), #15892, .F. ) ;
#5653=CARTESIAN_POINT ( 'NONE',  ( -5.008553330431526618, 117.3993852298624745, 0.7755932876167446199 ) ) ;
#5654=CARTESIAN_POINT ( 'NONE',  ( 17.44789039799410446, 148.6234142586927476, 2.276312578826294786 ) ) ;
#5656=CARTESIAN_POINT ( 'NONE',  ( -0.5673920217975719771, -4.456920702667952483, 8.403146712094516246 ) ) ;
#5657=CARTESIAN_POINT ( 'NONE',  ( 2.942445288855353169, 156.0884104482065595, 0.3607664148606970489 ) ) ;
#5660=ORIENTED_EDGE ( 'NONE', *, *, #22168, .F. ) ;
#5661=CARTESIAN_POINT ( 'NONE',  ( -1.006826980415389095, 118.1588900228295387, 0.8541050747360177109 ) ) ;
#5667=CARTESIAN_POINT ( 'NONE',  ( -8.215251585939828516, 117.5146787832509858, -0.03113046551775517159 ) ) ;
#5668=ORIENTED_EDGE ( 'NONE', *, *, #37538, .F. ) ;
#5670=CARTESIAN_POINT ( 'NONE',  ( 7.858252769910347268, 122.3222094090309326, -0.3873341666547952533 ) ) ;
#5673=CARTESIAN_POINT ( 'NONE',  ( 2.370544184569783219, 115.7028721635570747, -1.611047144755549887 ) ) ;
#5674=CARTESIAN_POINT ( 'NONE',  ( -9.185235947232945009, 124.1858035287836231, -0.2689572614166575448 ) ) ;
#5675=CARTESIAN_POINT ( 'NONE',  ( 2.642260502442670855, -15.21879886190521880, 5.833332612881661383 ) ) ;
#5676=CARTESIAN_POINT ( 'NONE',  ( -21.00062727315632927, 150.0074445146613584, 1.385517290469731266 ) ) ;
#5678=CARTESIAN_POINT ( 'NONE',  ( 22.94033276177397340, 150.1476136049543868, 0.7879714733284358674 ) ) ;
#5679=CARTESIAN_POINT ( 'NONE',  ( 14.67388681441289933, 148.8571912859537179, 0.3592780155011008336 ) ) ;
#5680=CARTESIAN_POINT ( 'NONE',  ( -4.896144065122994604, 117.7626873562327603, 0.6092677679091855758 ) ) ;
#5681=CARTESIAN_POINT ( 'NONE',  ( -0.5268263777171366957, 24.48095756788062261, 0.8226642508852344271 ) ) ;
#5682=CARTESIAN_POINT ( 'NONE',  ( -13.42863190281036800, 156.9273374874128137, -0.3327859972200287175 ) ) ;
#5686=CARTESIAN_POINT ( 'NONE',  ( 6.113542531766674948, 119.0002034676630416, 1.241036244702666380 ) ) ;
#5688=CARTESIAN_POINT ( 'NONE',  ( 5.210988722241143734, 158.8115599018184412, 1.325654878232527700 ) ) ;
#5689=CARTESIAN_POINT ( 'NONE',  ( 0.03067001211929459153, 158.6015251912307633, -1.534852821454057548 ) ) ;
#5690=CARTESIAN_POINT ( 'NONE',  ( 0.2322036383927537639, 20.64316925235604216, 8.417729739967510838 ) ) ;
#5691=CARTESIAN_POINT ( 'NONE',  ( -9.366440581936362975, 118.7255599110314961, -1.127239873969282602 ) ) ;
#5692=CARTESIAN_POINT ( 'NONE',  ( 4.755450631031003184, 117.7575004727687400, -0.8921683121825315643 ) ) ;
#5693=CARTESIAN_POINT ( 'NONE',  ( 4.366878780879478228, 111.2667756541687538, 3.131538613950388239 ) ) ;
#5694=CARTESIAN_POINT ( 'NONE',  ( -0.001255909994593423394, 120.9722815239556439, 0.06285087176068931969 ) ) ;
#5695=CARTESIAN_POINT ( 'NONE',  ( -5.971676678096491386, 157.1185343457808301, -1.951309749225692336 ) ) ;
#5696=CARTESIAN_POINT ( 'NONE',  ( 2.449088499779481953, -15.60605025760848719, 5.768239595176595458 ) ) ;
#5701=ORIENTED_EDGE ( 'NONE', *, *, #33419, .F. ) ;
#5702=CARTESIAN_POINT ( 'NONE',  ( 18.35995883219814928, 144.7751241387205425, 2.452750363274776912 ) ) ;
#5704=CARTESIAN_POINT ( 'NONE',  ( 5.008145224984434485, 117.3993836135855418, -0.7758584094373792706 ) ) ;
#5706=CARTESIAN_POINT ( 'NONE',  ( -1.751097875589126440, 120.5851793143259130, 0.4017021596164531139 ) ) ;
#5707=CARTESIAN_POINT ( 'NONE',  ( -7.571256676022106724, -0.2985773316772562525, 3.683590697331973196 ) ) ;
#5708=CARTESIAN_POINT ( 'NONE',  ( 7.694217360203059464, 122.2455405838764335, 0.6631844599531894202 ) ) ;
#5710=CARTESIAN_POINT ( 'NONE',  ( 16.58356254348269587, 122.7279807066903032, -0.3948093068319185606 ) ) ;
#5716=CARTESIAN_POINT ( 'NONE',  ( -6.439570805302779653E-14, 116.4254662015457313, -3.894619736530179447E-17 ) ) ;
#5719=CARTESIAN_POINT ( 'NONE',  ( -8.090109699362759699, 121.0242191076253988, -1.329746640891595888 ) ) ;
#5720=CARTESIAN_POINT ( 'NONE',  ( -5.247413993112555630, 104.6144662015457385, -1.481417380683311968 ) ) ;
#5722=CARTESIAN_POINT ( 'NONE',  ( 0.009747742627749139341, 156.3581291470199233, -0.4878169013068171522 ) ) ;
#5726=CARTESIAN_POINT ( 'NONE',  ( 4.585487687326599726, 17.13547844546973309, 0.5842699607688729424 ) ) ;
#5732=CARTESIAN_POINT ( 'NONE',  ( -6.992768045718048775, 121.9460250970137594, -0.06266173978408597078 ) ) ;
#5733=CARTESIAN_POINT ( 'NONE',  ( 5.332935392244917416, 115.7029491189645825, 0.1065647408284378928 ) ) ;
#5734=CARTESIAN_POINT ( 'NONE',  ( 21.67644226493397142, 136.7703657609320658, 1.576579429902728036 ) ) ;
#5737=CARTESIAN_POINT ( 'NONE',  ( 20.25200034474471522, 150.8812763393641490, -1.391365372170581649 ) ) ;
#5738=CARTESIAN_POINT ( 'NONE',  ( -8.333011053690857040, 121.0263440914440736, 1.031464938890432226 ) ) ;
#5739=CARTESIAN_POINT ( 'NONE',  ( -4.024516124431025688, 26.91537645720152128, -2.298571904627217499 ) ) ;
#5740=CARTESIAN_POINT ( 'NONE',  ( -14.30760545270006290, 120.4308286971427862, -0.9551244717093422265 ) ) ;
#5742=CARTESIAN_POINT ( 'NONE',  ( -0.5387148418522960114, 9.198764818822382949, 0.8109227438555447476 ) ) ;
#5745=CARTESIAN_POINT ( 'NONE',  ( -10.62272853480731172, 153.0636280899912549, 0.4455235322555911037 ) ) ;
#5746=CARTESIAN_POINT ( 'NONE',  ( 5.123467091704872800, -13.13098499675426112, 2.859697440480786668 ) ) ;
#5747=CARTESIAN_POINT ( 'NONE',  ( 16.77814054344316474, 146.6545634508490821, -1.109899152166417213 ) ) ;
#5749=CARTESIAN_POINT ( 'NONE',  ( 3.234322848356350644, 115.7029687383090675, 1.652822622332805969 ) ) ;
#5750=CARTESIAN_POINT ( 'NONE',  ( -4.745068207385612524, 117.6672791227833414, -1.125171127401668469 ) ) ;
#5751=CARTESIAN_POINT ( 'NONE',  ( 0.6418402141071639644, 156.3034662015456888, -0.01455126635812856346 ) ) ;
#5752=ORIENTED_EDGE ( 'NONE', *, *, #38896, .T. ) ;
#5753=CARTESIAN_POINT ( 'NONE',  ( 12.56843540011181304, 155.2353133052689032, 2.219430909113760730 ) ) ;
#5756=CARTESIAN_POINT ( 'NONE',  ( 15.21351360038763012, 143.4186079242255119, 0.3040022078858786170 ) ) ;
#5757=CARTESIAN_POINT ( 'NONE',  ( 4.958342374402591624, 117.4102150217221237, -0.9055978162701078249 ) ) ;
#5758=CARTESIAN_POINT ( 'NONE',  ( 23.17968947452040851, 149.6103952014060212, 0.1325215592567121625 ) ) ;
#5759=CARTESIAN_POINT ( 'NONE',  ( 0.08519874065564590759, 108.5751225745497948, -4.263693374914214296 ) ) ;
#5762=CARTESIAN_POINT ( 'NONE',  ( 1.647208221611285328, -15.32968734497926278, 5.596083536306344364 ) ) ;
#5764=DIRECTION ( 'NONE',  ( 0.9998004120163609398, 0.000000000000000000, 0.01997839162482749689 ) ) ;
#5765=CARTESIAN_POINT ( 'NONE',  ( -4.663774143481600021, 117.9610258373863019, 0.7407624695946702920 ) ) ;
#5768=CARTESIAN_POINT ( 'NONE',  ( -8.436567987665011259, 119.3310770286054492, -1.366807089744759285 ) ) ;
#5769=CARTESIAN_POINT ( 'NONE',  ( -3.617430929662352135, 113.7286232773062125, -2.299356966923025158 ) ) ;
#5770=CARTESIAN_POINT ( 'NONE',  ( 4.663391270879224670, 118.0052440920974277, 0.7715685123608813090 ) ) ;
#5772=CARTESIAN_POINT ( 'NONE',  ( -0.3819982885359083369, 122.2435587914033022, 0.2867773152523558911 ) ) ;
#5773=CARTESIAN_POINT ( 'NONE',  ( -4.288638401707804526, -7.253218809911426312, -1.756103832032595680 ) ) ;
#5774=CARTESIAN_POINT ( 'NONE',  ( 4.931598085382976393, 117.4109156735239452, -0.9380226465277491377 ) ) ;
#5776=CARTESIAN_POINT ( 'NONE',  ( 5.416028590487108829, 119.2618716387835747, -0.3471801096392532759 ) ) ;
#5777=CARTESIAN_POINT ( 'NONE',  ( -4.324763564747823530, 120.2039194668847699, -0.7996884002708144479 ) ) ;
#5779=CARTESIAN_POINT ( 'NONE',  ( -6.016145911062735330, 28.73530235815178102, 1.153596677464569398 ) ) ;
#5780=CARTESIAN_POINT ( 'NONE',  ( -2.146936912001416342, 115.7025561470850192, 1.628770542867131743 ) ) ;
#5781=CARTESIAN_POINT ( 'NONE',  ( 4.458631606973747274, 16.91056413504885825, 1.251853190366734259 ) ) ;
#5782=CARTESIAN_POINT ( 'NONE',  ( 8.168866085573474933, 117.6493956690293317, 0.5746791023534236764 ) ) ;
#5784=CARTESIAN_POINT ( 'NONE',  ( 4.895073708310537342, 104.6144662015544640, -2.147637011550606267 ) ) ;
#5785=CARTESIAN_POINT ( 'NONE',  ( 3.893829680932177517, -15.58178733528788129, 3.041689768969074503 ) ) ;
#5786=CARTESIAN_POINT ( 'NONE',  ( -14.27152401005736415, 125.7140216354555804, 1.459898031787023598 ) ) ;
#5787=CARTESIAN_POINT ( 'NONE',  ( -0.5888577047260095121, 18.69815917492401880, 0.7773729966010974879 ) ) ;
#5788=CARTESIAN_POINT ( 'NONE',  ( 0.3244192847266222923, 10.43846528477952340, -0.9201954171864650256 ) ) ;
#5792=CARTESIAN_POINT ( 'NONE',  ( 0.3635706870683514946, 106.2969274751293938, 5.168771910137537340 ) ) ;
#5794=CARTESIAN_POINT ( 'NONE',  ( -9.788763933237108361, 123.8372022493589100, 0.5907035020478677012 ) ) ;
#5796=CARTESIAN_POINT ( 'NONE',  ( 3.015147157152042290, -12.41699557045261670, 0.4662733852003331791 ) ) ;
#5797=CARTESIAN_POINT ( 'NONE',  ( 11.09075344257208684, 123.0430266451958232, -1.157373622111985467 ) ) ;
#5798=CARTESIAN_POINT ( 'NONE',  ( -17.72814975036780183, 131.6735282812448986, -2.269257323068798460 ) ) ;
#5799=CARTESIAN_POINT ( 'NONE',  ( 3.174366308151880922, 104.6144662015457243, 0.06343139340882769650 ) ) ;
#5801=CARTESIAN_POINT ( 'NONE',  ( 7.963027852037909859, 121.6653397483754020, 1.110511108043854778 ) ) ;
#5802=CARTESIAN_POINT ( 'NONE',  ( -0.01691503824241830795, 39.20946620154573026, 0.8464976821738520174 ) ) ;
#5803=CARTESIAN_POINT ( 'NONE',  ( 9.357997026032778720, 124.2740283646700306, -0.04730198213477312952 ) ) ;
#5804=VERTEX_POINT ( 'NONE', #40755 ) ;
#5805=CARTESIAN_POINT ( 'NONE',  ( -2.372405652431340606, 106.9230564690743819, -4.772463516138556905 ) ) ;
#5810=CARTESIAN_POINT ( 'NONE',  ( 1.466575460758787530, 20.86946789039323491, 8.308456332865098659 ) ) ;
#5811=CARTESIAN_POINT ( 'NONE',  ( 10.07755082079036235, 123.5826510519420509, 1.213607387526569381 ) ) ;
#5812=DIRECTION ( 'NONE',  ( -4.017660918040594346E-17, 1.000000000000000000, 2.376309959284834438E-19 ) ) ;
#5813=CARTESIAN_POINT ( 'NONE',  ( 21.90617686096470251, 151.4314113202728436, 0.4124301881307766982 ) ) ;
#5814=CARTESIAN_POINT ( 'NONE',  ( -0.3637657132513893443, 105.8833743670705445, 5.328194401858565854 ) ) ;
#5815=CARTESIAN_POINT ( 'NONE',  ( 4.349802767100347189, -10.92635770930747796, -1.576909098649299512 ) ) ;
#5816=CARTESIAN_POINT ( 'NONE',  ( 4.218275339060157059, 155.8585684991085714, 0.08429118021179421438 ) ) ;
#5818=CARTESIAN_POINT ( 'NONE',  ( 4.267473507877284078, -4.198009126799147062, -7.300781474974544771 ) ) ;
#5819=CARTESIAN_POINT ( 'NONE',  ( 5.516891121731406500, 117.1192735582419004, -0.5335394950436042061 ) ) ;
#5820=CARTESIAN_POINT ( 'NONE',  ( -0.4232488410869896800, 124.9344662015457317, -0.008457519121176893320 ) ) ;
#5821=CARTESIAN_POINT ( 'NONE',  ( 4.854633716284418199, 115.7029491485453150, -1.279498648767042557 ) ) ;
#5822=CARTESIAN_POINT ( 'NONE',  ( -6.573280687130626123E-14, 88.99346620154574339, 1.699031322814114629E-29 ) ) ;
#5823=CARTESIAN_POINT ( 'NONE',  ( 7.741462187161934239, -10.92447321953606654, -3.338652055795839679 ) ) ;
#5824=CARTESIAN_POINT ( 'NONE',  ( 0.3314860322431096296, 118.1588881126417050, 0.9092559162175757326 ) ) ;
#5828=CARTESIAN_POINT ( 'NONE',  ( 0.6471768874970514895, 112.6282971158091470, -2.732684515117583590 ) ) ;
#5829=CARTESIAN_POINT ( 'NONE',  ( -22.91960207526971871, 149.8162411397050278, 0.2683370967508547644 ) ) ;
#5832=EDGE_CURVE ( 'NONE', #3703, #276, #32095, .T. ) ;
#5833=ORIENTED_EDGE ( 'NONE', *, *, #13123, .F. ) ;
#5835=CARTESIAN_POINT ( 'NONE',  ( -15.77337136323457578, 146.5674407247335864, -0.1809852566079092895 ) ) ;
#5836=CARTESIAN_POINT ( 'NONE',  ( 4.513795256570364067, -15.26848473984131260, 4.551867270201407578 ) ) ;
#5837=CARTESIAN_POINT ( 'NONE',  ( -5.883382875664681322, 118.7305451321402501, 0.9239882381799517930 ) ) ;
#5839=CARTESIAN_POINT ( 'NONE',  ( 14.39601482975355040, 155.9958976045614349, -1.017949466214369325 ) ) ;
#5840=CARTESIAN_POINT ( 'NONE',  ( 3.345514242732226418, 6.565394131763864216, 3.211428121085859733 ) ) ;
#5841=CARTESIAN_POINT ( 'NONE',  ( -1.872007501980990085, 116.6503132507590124, -0.2654151457657343283 ) ) ;
#5844=CARTESIAN_POINT ( 'NONE',  ( -0.01046636459302786523, 120.7331730230139755, 0.5237796829255390030 ) ) ;
#5845=DIRECTION ( 'NONE',  ( 4.017660918040594346E-17, -1.000000000000000000, -2.376309959284834438E-19 ) ) ;
#5846=CARTESIAN_POINT ( 'NONE',  ( -0.008945177888008831735, 119.9096241394016715, 0.4476532798976762817 ) ) ;
#5848=CARTESIAN_POINT ( 'NONE',  ( 11.27019207447471416, 122.4230570912197038, -1.244363564371071540 ) ) ;
#5849=CARTESIAN_POINT ( 'NONE',  ( -21.29267830536757700, 148.0064520001644723, -2.314741142932118301 ) ) ;
#5851=CARTESIAN_POINT ( 'NONE',  ( 9.279111390949699611, 123.6186430441458981, -0.4039598099628549099 ) ) ;
#5852=CIRCLE ( 'NONE', #39957, 3.683000000000001162 ) ;
#5854=CARTESIAN_POINT ( 'NONE',  ( -11.03566430468816328, 123.0430266451958232, -1.599512106649902288 ) ) ;
#5855=CARTESIAN_POINT ( 'NONE',  ( 2.813987013336220144, -15.51818976969260255, 4.585835125202748053 ) ) ;
#5856=CARTESIAN_POINT ( 'NONE',  ( -4.106443892462531942, 118.2429491485453070, -0.3519330368941736564 ) ) ;
#5858=CARTESIAN_POINT ( 'NONE',  ( -4.887531664472737347, 117.7483860691352646, 0.7386977146963198404 ) ) ;
#5859=CARTESIAN_POINT ( 'NONE',  ( 17.73873607445671041, 146.7645792007554633, 2.242890973037755753 ) ) ;
#5861=CARTESIAN_POINT ( 'NONE',  ( -7.781828003681788175, 2.241565531857627303, -3.240848859074576094 ) ) ;
#5862=CARTESIAN_POINT ( 'NONE',  ( 13.02783148976608807, 133.9378623523624299, 0.5757418746946232346 ) ) ;
#5866=CARTESIAN_POINT ( 'NONE',  ( -0.8541570955536235132, 117.3993835805775490, 1.452923500009727809 ) ) ;
#5872=CARTESIAN_POINT ( 'NONE',  ( -23.34154082800050745, 148.8574307740229585, -0.2355990431193896728 ) ) ;
#5875=CARTESIAN_POINT ( 'NONE',  ( -7.802523906719404323, 122.5105737818149407, -0.4685457770883232897 ) ) ;
#5876=ADVANCED_FACE ( 'NONE', ( #4777 ), #12497, .T. ) ;
#5877=CARTESIAN_POINT ( 'NONE',  ( 5.008145594203718076, 117.3993868333640478, -0.7758522469519856246 ) ) ;
#5878=ORIENTED_EDGE ( 'NONE', *, *, #36551, .F. ) ;
#5879=CARTESIAN_POINT ( 'NONE',  ( 1.799517872912148819, 115.7029357459833818, -1.654564060799146752 ) ) ;
#5880=CARTESIAN_POINT ( 'NONE',  ( -15.78121303607992942, 145.9231181611787918, -0.5460855120906793481 ) ) ;
#5881=CARTESIAN_POINT ( 'NONE',  ( 5.728675787863017455, -12.92793046001887447, 1.911514839944304045 ) ) ;
#5882=CARTESIAN_POINT ( 'NONE',  ( -0.009931510163747995362, 117.7854482299006378, 0.4970133802592051064 ) ) ;
#5883=CARTESIAN_POINT ( 'NONE',  ( -5.151949832170181764, 116.8361703259256217, -0.1799158315879852421 ) ) ;
#5884=CARTESIAN_POINT ( 'NONE',  ( 22.51303867192105912, 150.7865899205276321, 0.6781733187083919256 ) ) ;
#5886=CARTESIAN_POINT ( 'NONE',  ( 5.942184298922027708, 155.4082271737278234, 0.2231331471019911694 ) ) ;
#5888=CARTESIAN_POINT ( 'NONE',  ( -0.9756160567605162148, 3.744600508531710226, -0.009113680661486545098 ) ) ;
#5889=CARTESIAN_POINT ( 'NONE',  ( -15.18737561846517892, 156.0999766016731769, -0.3708822620858232555 ) ) ;
#5890=FACE_OUTER_BOUND ( 'NONE', #28904, .T. ) ;
#5891=CARTESIAN_POINT ( 'NONE',  ( -3.682264917456322895, 66.13346620154572975, -0.07358041635423968885 ) ) ;
#5892=ORIENTED_EDGE ( 'NONE', *, *, #10812, .F. ) ;
#5893=CARTESIAN_POINT ( 'NONE',  ( 5.529506464480028249, 117.0650090453692798, 0.6737858539469722130 ) ) ;
#5895=CARTESIAN_POINT ( 'NONE',  ( 21.09420047167885315, 149.7512365312068709, 2.228874019815534346 ) ) ;
#5896=CARTESIAN_POINT ( 'NONE',  ( 7.699499347746429301, 119.6133147451300971, -1.075113282820071570 ) ) ;
#5897=CARTESIAN_POINT ( 'NONE',  ( 1.285294229880325600, 5.975470260049262627, -8.359553334813638159 ) ) ;
#5898=EDGE_CURVE ( 'NONE', #28135, #8589, #36447, .T. ) ;
#5899=CARTESIAN_POINT ( 'NONE',  ( -21.19929070476258204, 136.5942649496780632, -1.819607900871525574 ) ) ;
#5900=CARTESIAN_POINT ( 'NONE',  ( 4.712039816507104462, 117.8377826564535980, -0.8492390109202567761 ) ) ;
#5901=CARTESIAN_POINT ( 'NONE',  ( 6.914225208283751201, 121.8192184429722005, 0.2944576502256240347 ) ) ;
#5902=CARTESIAN_POINT ( 'NONE',  ( -7.800806202325043515, 154.6345575486818404, -0.04849676858278722386 ) ) ;
#5903=CARTESIAN_POINT ( 'NONE',  ( -18.80567741551218930, 148.1672603684278329, -2.476295349149460367 ) ) ;
#5904=CARTESIAN_POINT ( 'NONE',  ( 3.388119949408427978, -15.58183483456807039, 5.324763925812813881 ) ) ;
#5905=CARTESIAN_POINT ( 'NONE',  ( 4.726842832297071695, 118.5931160184169073, 1.020482801973786380 ) ) ;
#5907=CARTESIAN_POINT ( 'NONE',  ( -1.960935811749206170, 117.3993839180219254, -1.450040409155178622 ) ) ;
#5908=AXIS2_PLACEMENT_3D ( 'NONE', #22731, #28933, #13386 ) ;
#5910=CARTESIAN_POINT ( 'NONE',  ( 9.495519422240706220, 121.2752502669211339, 1.536911970732435684 ) ) ;
#5913=CARTESIAN_POINT ( 'NONE',  ( -1.341555883842942887, 107.4826764677166864, 4.621745984720207368 ) ) ;
#5914=CARTESIAN_POINT ( 'NONE',  ( -8.308456333890557488, -0.7205321100333081930, 1.466575456822119206 ) ) ;
#5915=CARTESIAN_POINT ( 'NONE',  ( 9.680894551640095713, 124.1466939447965814, 0.8054060769509039375 ) ) ;
#5916=CARTESIAN_POINT ( 'NONE',  ( 10.53014098995821435, 157.9057380314836223, -0.5653498989572928179 ) ) ;
#5920=CARTESIAN_POINT ( 'NONE',  ( -6.552838421881942555E-14, 85.18346620154574111, 1.207165459533130484E-19 ) ) ;
#5922=CARTESIAN_POINT ( 'NONE',  ( -22.53527615164633602, 150.7831677823008363, -0.4503084484864735004 ) ) ;
#5923=ORIENTED_EDGE ( 'NONE', *, *, #8940, .T. ) ;
#5924=CARTESIAN_POINT ( 'NONE',  ( -8.204323950348388905, 120.4574377990110463, -1.430383891062076085 ) ) ;
#5927=CARTESIAN_POINT ( 'NONE',  ( -7.064669522240172306, 121.9740017686541194, -0.4795729057185782462 ) ) ;
#5929=CARTESIAN_POINT ( 'NONE',  ( 11.73662545640870114, 118.7267541726749869, 0.2503127652027327121 ) ) ;
#5932=CARTESIAN_POINT ( 'NONE',  ( 3.121479725567877228, 16.06095178295013071, 3.416230322513892137 ) ) ;
#5933=CARTESIAN_POINT ( 'NONE',  ( -5.041288869262119832, 105.1216794573741282, 1.777295568394765546 ) ) ;
#5934=CARTESIAN_POINT ( 'NONE',  ( -6.426369768295692736E-14, 159.6054662015457382, 1.032716915552223178E-16 ) ) ;
#5935=LINE ( 'NONE', #8906, #34673 ) ;
#5938=CARTESIAN_POINT ( 'NONE',  ( -6.068594780648083997, 121.4118082408263746, 0.08813677267068076304 ) ) ;
#5940=CARTESIAN_POINT ( 'NONE',  ( -2.131885088311801901, 26.04095958170969638, -4.099730575217565232 ) ) ;
#5941=CARTESIAN_POINT ( 'NONE',  ( 21.30289582938779702, 151.2846570542378117, 1.588627997894106247 ) ) ;
#5942=CARTESIAN_POINT ( 'NONE',  ( 2.602530512026160370, 104.6144662015457243, -4.073939027099183541 ) ) ;
#5943=CARTESIAN_POINT ( 'NONE',  ( -0.1058213901579529159, 105.9761915687834914, 5.295735085524055030 ) ) ;
#5944=CARTESIAN_POINT ( 'NONE',  ( 7.150008447151647850, 158.1912585135832785, -1.373277972272069380 ) ) ;
#5945=CARTESIAN_POINT ( 'NONE',  ( -9.808453647370097173, 155.3230018269108825, 1.667681936676748133 ) ) ;
#5946=CARTESIAN_POINT ( 'NONE',  ( 0.7725151586569730666, -15.29989167607388900, -0.5872501270430795506 ) ) ;
#5947=CARTESIAN_POINT ( 'NONE',  ( -16.43260349481045424, 122.7513851185756693, -1.135385547233646042 ) ) ;
#5948=EDGE_LOOP ( 'NONE', ( #15129, #15605, #31191, #32905 ) ) ;
#5950=CARTESIAN_POINT ( 'NONE',  ( -12.26386414673838843, 130.6044139104978115, 0.2969705276545481776 ) ) ;
#5951=CARTESIAN_POINT ( 'NONE',  ( 3.928490385995774936, -14.72231570353084429, 5.141255514400237203 ) ) ;
#5952=CARTESIAN_POINT ( 'NONE',  ( 10.67172107669495418, 123.8807653058400575, -0.9292482510779808136 ) ) ;
#5953=DIRECTION ( 'NONE',  ( -5.206863593109713661E-17, 1.000000000000000000, -1.077750396879097183E-30 ) ) ;
#5955=CARTESIAN_POINT ( 'NONE',  ( -4.676071978438741894, 117.9791466300892750, -0.8444188316661053184 ) ) ;
#5956=CARTESIAN_POINT ( 'NONE',  ( 15.21929369751753924, 143.4245298570049840, 0.2523546585945008469 ) ) ;
#5958=CARTESIAN_POINT ( 'NONE',  ( 20.02396230387740772, 148.3334041379468715, 2.502640320863741774 ) ) ;
#5961=CARTESIAN_POINT ( 'NONE',  ( 5.002599301907898699, 117.4023545182666055, -0.8031422281648238348 ) ) ;
#5962=AXIS2_PLACEMENT_3D ( 'NONE', #8377, #21342, #6242 ) ;
#5963=CARTESIAN_POINT ( 'NONE',  ( 0.3151558924358287550, 116.5752054743899038, -0.1523977429619429169 ) ) ;
#5967=CARTESIAN_POINT ( 'NONE',  ( 1.694057231424134446, -15.22899506564825955, 5.771026123934793972 ) ) ;
#5969=CARTESIAN_POINT ( 'NONE',  ( -4.665613787933919454, 118.0266005560186358, 0.5747475622275362017 ) ) ;
#5973=CARTESIAN_POINT ( 'NONE',  ( -5.958530970433706386, 119.2302670178880817, -1.266206984860304585 ) ) ;
#5974=CARTESIAN_POINT ( 'NONE',  ( -3.948369173669738608, 116.4303826247378026, -1.336099082351541956 ) ) ;
#5975=CARTESIAN_POINT ( 'NONE',  ( 4.772709941698821901, 117.8804716543160112, 0.8736280956481000670 ) ) ;
#5976=CARTESIAN_POINT ( 'NONE',  ( 3.205191379615736746, -14.47393913169138102, 3.051678166811226500 ) ) ;
#5977=CARTESIAN_POINT ( 'NONE',  ( -10.42685857375371050, 124.8149993102252182, -1.042337215157124186 ) ) ;
#5978=CIRCLE ( 'NONE', #22269, 0.5079999999999997851 ) ;
#5979=CARTESIAN_POINT ( 'NONE',  ( -2.983771112188844832, -5.329111280313512999, 3.548611825089460048 ) ) ;
#5980=CARTESIAN_POINT ( 'NONE',  ( -1.958751975754273289, 106.7073577057565643, 4.892300404344175568 ) ) ;
#5982=CARTESIAN_POINT ( 'NONE',  ( 5.578601203221819738, 117.9513286348681476, -0.5234822864975615664 ) ) ;
#5983=CARTESIAN_POINT ( 'NONE',  ( -10.91091678335021342, 123.4376579628654014, -1.516229561143084492 ) ) ;
#5984=CARTESIAN_POINT ( 'NONE',  ( 16.31694223957253698, 121.4173703750124531, 0.3260513381110077824 ) ) ;
#5985=CARTESIAN_POINT ( 'NONE',  ( -3.991072007095600949, 33.40439263831326855, 3.842775004540742501 ) ) ;
#5986=CARTESIAN_POINT ( 'NONE',  ( -4.589169710308834915, 115.7029491485453434, 1.333228958008984888 ) ) ;
#5987=CARTESIAN_POINT ( 'NONE',  ( -1.178223178616622402, 14.53665720681882689, 4.476207649055042204 ) ) ;
#5988=CARTESIAN_POINT ( 'NONE',  ( 23.25105004451259916, 146.7258352529021863, 1.066525923017375810 ) ) ;
#5990=CARTESIAN_POINT ( 'NONE',  ( 2.045048008636439540, 104.6144662015458096, -4.372098095898148351 ) ) ;
#5991=CARTESIAN_POINT ( 'NONE',  ( 3.879565938682602244, -15.27118588775909558, 0.8622231344456012803 ) ) ;
#5992=CARTESIAN_POINT ( 'NONE',  ( -3.289525010481907596, 118.9727644790723531, 0.7721065173366226109 ) ) ;
#5993=CARTESIAN_POINT ( 'NONE',  ( -0.5956917769015268593, 15.89737491555829685, -0.7703063551142234067 ) ) ;
#5994=B_SPLINE_CURVE_WITH_KNOTS ( 'NONE', 3,
 ( #6052, #32650, #18802, #19014, #38633, #35645, #291, #22822, #19434, #6255 ),
 .UNSPECIFIED., .F., .F.,
 ( 4, 2, 2, 2, 4 ),
 ( 0.000000000000000000, 0.0001138296224026695075, 0.0002276592448053389066, 0.0004553184896106773254, 0.0009106369792213540003 ),
 .UNSPECIFIED. ) ;
#5995=CARTESIAN_POINT ( 'NONE',  ( 0.5139362334885246852, 0.5165572279304807557, -0.8313783143454911428 ) ) ;
#5999=CARTESIAN_POINT ( 'NONE',  ( 1.025137579952656308, 106.6134986179334589, 5.027802332087124348 ) ) ;
#6001=CARTESIAN_POINT ( 'NONE',  ( -9.877746432283343481, 123.9483309312939099, 0.5948279539607077560 ) ) ;
#6002=CARTESIAN_POINT ( 'NONE',  ( -9.538359384048678891, 124.8019839352694476, -0.1905991205270209377 ) ) ;
#6003=CARTESIAN_POINT ( 'NONE',  ( 2.740927916200229131, -14.67636064986481337, 4.771625012207401539 ) ) ;
#6004=CARTESIAN_POINT ( 'NONE',  ( 17.52489820599659254, 148.6234142586927476, -1.577473031907404621 ) ) ;
#6005=CARTESIAN_POINT ( 'NONE',  ( -17.05522983032417628, 131.5760549582342094, -2.311017189013932160 ) ) ;
#6006=DIRECTION ( 'NONE',  ( 0.9998004120163610509, 4.016384292689131511E-17, 0.01997839162482749689 ) ) ;
#6007=CARTESIAN_POINT ( 'NONE',  ( 8.788213500272473055, 117.7098710386940894, 0.3783554591865261885 ) ) ;
#6008=CARTESIAN_POINT ( 'NONE',  ( 4.074910602682932925, 118.2429491485453354, -0.1454311599470142491 ) ) ;
#6009=CARTESIAN_POINT ( 'NONE',  ( 15.68661553393314456, 147.2319784351455780, -0.01612984191841659518 ) ) ;
#6011=CARTESIAN_POINT ( 'NONE',  ( 2.666490510518176649, -13.49855353256042889, 0.05227394649444832425 ) ) ;
#6012=CARTESIAN_POINT ( 'NONE',  ( 5.586884702347362897, 123.6644662015457214, 0.1116392523995368424 ) ) ;
#6013=CARTESIAN_POINT ( 'NONE',  ( 2.928799644063047936, 38.81416391459460158, 1.351591292951386469 ) ) ;
#6015=FACE_OUTER_BOUND ( 'NONE', #12670, .T. ) ;
#6016=CARTESIAN_POINT ( 'NONE',  ( -6.293633234193186432, 17.08131519529194975, -5.670988759835773330 ) ) ;
#6017=CARTESIAN_POINT ( 'NONE',  ( 14.37089176232986354, 134.5679602169015254, 1.683180344383908400 ) ) ;
#6019=CARTESIAN_POINT ( 'NONE',  ( 5.781358041568656070, 116.9360814311326777, 0.07286664083783171708 ) ) ;
#6021=CARTESIAN_POINT ( 'NONE',  ( -4.473299935328737931, 111.2795884869231173, 2.951234740152492986 ) ) ;
#6022=CARTESIAN_POINT ( 'NONE',  ( -0.2095918955067871126, -8.989892990265463624, -4.636818132431064221 ) ) ;
#6023=CARTESIAN_POINT ( 'NONE',  ( 1.561582345843624431, 156.2588034088681184, 0.03120413162939523685 ) ) ;
#6024=B_SPLINE_CURVE_WITH_KNOTS ( 'NONE', 3,
 ( #41497, #8485, #37866, #21652, #15274, #25078 ),
 .UNSPECIFIED., .F., .F.,
 ( 4, 2, 4 ),
 ( 0.000000000000000000, 0.5000000000000000000, 1.000000000000000000 ),
 .UNSPECIFIED. ) ;
#6025=CARTESIAN_POINT ( 'NONE',  ( 15.86975487621997871, 125.3951846505478329, 1.921535798876653711 ) ) ;
#6026=CARTESIAN_POINT ( 'NONE',  ( 4.673167956146812685, 25.32871407960522347, 7.020956665532097851 ) ) ;
#6027=CARTESIAN_POINT ( 'NONE',  ( -5.476986130384075224, 117.4239406935068786, -0.9134031189204426804 ) ) ;
#6028=CARTESIAN_POINT ( 'NONE',  ( -0.2094794444023877211, 111.5577547982948801, -3.149697633913104422 ) ) ;
#6029=CARTESIAN_POINT ( 'NONE',  ( -22.98488057257204886, 150.1591296352320910, -0.4592926148156235011 ) ) ;
#6031=CARTESIAN_POINT ( 'NONE',  ( -2.768688662514669385, 30.30441277318858795, -3.700580903672975541 ) ) ;
#6032=CARTESIAN_POINT ( 'NONE',  ( 3.117173950248831815, 118.1588878836352166, 0.8040983753412327406 ) ) ;
#6034=CARTESIAN_POINT ( 'NONE',  ( 2.234143439902941175, -15.10063862499563747, 5.099642030148213934 ) ) ;
#6036=CARTESIAN_POINT ( 'NONE',  ( 0.7761819157717084749, 120.0979018405971175, -0.5779541898223675700 ) ) ;
#6037=CARTESIAN_POINT ( 'NONE',  ( -22.39781672572324567, 150.5530013069706285, 0.3987920954333213919 ) ) ;
#6038=VERTEX_POINT ( 'NONE', #7727 ) ;
#6039=CARTESIAN_POINT ( 'NONE',  ( -3.682264917456323339, 78.83346620154574680, -0.07358041635423968885 ) ) ;
#6040=ORIENTED_EDGE ( 'NONE', *, *, #20631, .T. ) ;
#6042=CARTESIAN_POINT ( 'NONE',  ( 4.894061823620152296, -15.42295773938226411, 3.608731902971048733 ) ) ;
#6043=CARTESIAN_POINT ( 'NONE',  ( -1.172281656590623111, 158.5855360310326319, 1.517099175104413833 ) ) ;
#6044=CARTESIAN_POINT ( 'NONE',  ( 12.65084386183212040, 120.1953580586475567, -0.8051295378619940379 ) ) ;
#6045=CARTESIAN_POINT ( 'NONE',  ( -3.812863311134618183, 2.017465188139291765, -2.614655560905410958 ) ) ;
#6049=CARTESIAN_POINT ( 'NONE',  ( 0.4232488410868608941, 124.9344662015457317, 0.008457519121177021690 ) ) ;
#6050=CARTESIAN_POINT ( 'NONE',  ( -6.654617103318593247E-14, 104.6144662015457243, 1.534725424433578570E-31 ) ) ;
#6051=CARTESIAN_POINT ( 'NONE',  ( -14.11650378654216631, 131.1061190467503934, 1.279305142450560151 ) ) ;
#6052=CARTESIAN_POINT ( 'NONE',  ( 5.152689472752729039, 116.8412042436348912, 0.1029629964107459106 ) ) ;
#6054=CARTESIAN_POINT ( 'NONE',  ( 5.877700541659331535, 119.5807162246413498, -0.9453723347071265604 ) ) ;
#6056=CARTESIAN_POINT ( 'NONE',  ( -18.56731909478085996, 131.8045874826418071, -2.147352672676718033 ) ) ;
#6058=CARTESIAN_POINT ( 'NONE',  ( 4.498274173885895344, 155.8822484669112214, -0.6329996689149901545 ) ) ;
#6060=CARTESIAN_POINT ( 'NONE',  ( -0.5133504486497384445, 119.5442839488369628, -0.5494766105906193632 ) ) ;
#6061=CARTESIAN_POINT ( 'NONE',  ( 3.555255404795384599, -15.46298345743583802, 3.323699395844104565 ) ) ;
#6062=CARTESIAN_POINT ( 'NONE',  ( -4.149547856688258207, 118.2393522679058009, -0.3953376121465850823 ) ) ;
#6065=CARTESIAN_POINT ( 'NONE',  ( -4.902692966696466925, 117.7192222769238441, 0.7484533029765950696 ) ) ;
#6066=CARTESIAN_POINT ( 'NONE',  ( 11.83432680469861431, 124.3826620800890339, 1.661842703385269848 ) ) ;
#6068=CARTESIAN_POINT ( 'NONE',  ( 2.332027132427558769, 25.33165720878049498, 3.998286310156994983 ) ) ;
#6069=CARTESIAN_POINT ( 'NONE',  ( 14.27613791431590151, 138.9852717218771261, 0.6171993629658321101 ) ) ;
#6071=TOROIDAL_SURFACE ( 'NONE', #30567, 3.683000000000000718, 0.5080000000000000071 ) ;
#6073=CARTESIAN_POINT ( 'NONE',  ( -0.2378499585937704497, 117.3993841996711041, 1.487621480530184614 ) ) ;
#6079=CARTESIAN_POINT ( 'NONE',  ( -22.50450395291955275, 150.7830971219523519, -0.1219060866366470514 ) ) ;
#6082=CARTESIAN_POINT ( 'NONE',  ( 6.957078529942896772, 121.9380298548064445, -0.02067918444371699693 ) ) ;
#6083=CARTESIAN_POINT ( 'NONE',  ( 4.854575378875618519, 117.4045355995268096, -0.9984935320486798549 ) ) ;
#6085=CARTESIAN_POINT ( 'NONE',  ( 1.153264477914338615, 115.7029425313346280, -1.700750124145387732 ) ) ;
#6086=CARTESIAN_POINT ( 'NONE',  ( -15.76687399610644391, 145.9134097338176730, -0.4436328104633034397 ) ) ;
#6087=CARTESIAN_POINT ( 'NONE',  ( 2.458590490134419770, -15.31022926314896893, 5.890968354261565842 ) ) ;
#6088=CARTESIAN_POINT ( 'NONE',  ( -17.06313393459315719, 153.7580772870718988, 1.402989014430432668 ) ) ;
#6089=CARTESIAN_POINT ( 'NONE',  ( -5.010144981628188887, 117.3993855238222608, -0.7522679339500687457 ) ) ;
#6090=CARTESIAN_POINT ( 'NONE',  ( 23.33231982438472940, 148.8574307740229585, 0.6970557703302366903 ) ) ;
#6091=CARTESIAN_POINT ( 'NONE',  ( 8.410838065576685452, 123.3149317519321784, 0.2957792723555629499 ) ) ;
#6093=CARTESIAN_POINT ( 'NONE',  ( 0.7153056356866435150, 7.414959551268969662, 0.6636563042211964802 ) ) ;
#6094=CARTESIAN_POINT ( 'NONE',  ( -6.901437262003314643, 117.1762911274595496, -0.2238905109288658601 ) ) ;
#6098=EDGE_LOOP ( 'NONE', ( #278, #12115, #24384, #26357 ) ) ;
#6099=CARTESIAN_POINT ( 'NONE',  ( -5.697209421088824222, 117.9270612091053891, 0.8225170165645491194 ) ) ;
#6100=ORIENTED_EDGE ( 'NONE', *, *, #19550, .F. ) ;
#6102=CARTESIAN_POINT ( 'NONE',  ( 12.03559625110886522, 156.5645100661158153, 1.882936990620205808 ) ) ;
#6103=CARTESIAN_POINT ( 'NONE',  ( 12.82775609536331807, 122.1393999080170971, -1.276540306405074876 ) ) ;
#6104=CARTESIAN_POINT ( 'NONE',  ( -8.197529660144020625, 8.984976746712527884, 2.078235512056660017 ) ) ;
#6105=CARTESIAN_POINT ( 'NONE',  ( -11.09758427587551743, 119.2389763063149388, -1.130321237809625234 ) ) ;
#6106=CARTESIAN_POINT ( 'NONE',  ( 4.657610911615179816, 117.9597807199399000, -0.7455203706293841437 ) ) ;
#6107=CARTESIAN_POINT ( 'NONE',  ( 8.798071512540863282, 117.6842349196870572, 0.1758064070670784795 ) ) ;
#6108=CARTESIAN_POINT ( 'NONE',  ( -10.43234786055289653, 153.0845720789597522, -0.001036074960336963707 ) ) ;
#6110=CARTESIAN_POINT ( 'NONE',  ( -10.72551448100101901, 121.7859837122882283, -1.665033671525604220 ) ) ;
#6112=CARTESIAN_POINT ( 'NONE',  ( 2.008732664060286055, -15.70244684250787870, 5.701976698490775597 ) ) ;
#6114=CARTESIAN_POINT ( 'NONE',  ( -6.376221727585796537E-14, 51.14746620154573264, 5.777789833161707559E-29 ) ) ;
#6117=CARTESIAN_POINT ( 'NONE',  ( 14.67610382776214628, 152.8628051715174365, 2.323547792494559339 ) ) ;
#6118=DIRECTION ( 'NONE',  ( -0.9998004120163608288, 0.000000000000000000, -0.01997839162482747608 ) ) ;
#6121=CARTESIAN_POINT ( 'NONE',  ( -3.145827930498041880, 117.0475107411037641, 1.097865318250619948 ) ) ;
#6123=CARTESIAN_POINT ( 'NONE',  ( 8.391225363336687337, -15.30560670943152957, -0.4339906691978474562 ) ) ;
#6124=CARTESIAN_POINT ( 'NONE',  ( 15.79391552826336209, 147.6293441119438512, 1.163731531224506899 ) ) ;
#6125=CARTESIAN_POINT ( 'NONE',  ( 0.01133159106138621405, 159.5297144918048673, -0.5670791535570575137 ) ) ;
#6128=CIRCLE ( 'NONE', #28560, 1.000000000000000888 ) ;
#6129=CARTESIAN_POINT ( 'NONE',  ( -15.19604463793445959, 156.0859089222169587, -0.3036531364422413448 ) ) ;
#6130=ADVANCED_FACE ( 'NONE', ( #14511, #37113 ), #20267, .F. ) ;
#6132=CARTESIAN_POINT ( 'NONE',  ( -8.200576496910658264, 120.4759052327119235, -1.428406516435469342 ) ) ;
#6133=CARTESIAN_POINT ( 'NONE',  ( 3.038459613674064919, -15.39881274666275779, 5.660802783634620639 ) ) ;
#6134=CARTESIAN_POINT ( 'NONE',  ( -15.96686920080710870, 146.6619865182943272, -1.046663894505766468 ) ) ;
#6136=CARTESIAN_POINT ( 'NONE',  ( 23.34372044207203700, 149.0681261006882039, 0.4664630893996631333 ) ) ;
#6137=VERTEX_POINT ( 'NONE', #40531 ) ;
#6138=CARTESIAN_POINT ( 'NONE',  ( -4.012847786888796620, 11.73797844546971270, -2.294585225469591983 ) ) ;
#6141=DIRECTION ( 'NONE',  ( -5.206863593109713661E-17, 1.000000000000000000, -1.077750396879097183E-30 ) ) ;
#6143=CARTESIAN_POINT ( 'NONE',  ( 6.049108887567863135, 120.6719078856681193, 0.9521718272089157997 ) ) ;
#6144=CARTESIAN_POINT ( 'NONE',  ( 4.531904421025400254, 4.026177021345840323, -0.9239884639389631671 ) ) ;
#6145=CARTESIAN_POINT ( 'NONE',  ( -0.007599820978813201684, 117.2191897141855179, 0.3803261187632672735 ) ) ;
#6146=CARTESIAN_POINT ( 'NONE',  ( 15.78437780952694069, 146.2378312303354448, 0.3154094333657936899 ) ) ;
#6147=CARTESIAN_POINT ( 'NONE',  ( 2.666490510518176649, -13.49855353256042889, 0.05227394649444832425 ) ) ;
#6148=CARTESIAN_POINT ( 'NONE',  ( 1.211137314531071985, 158.8088198215516229, -1.425359051240900232 ) ) ;
#6149=CARTESIAN_POINT ( 'NONE',  ( -1.441504266290200897, 6.599927940091079748, -4.410093354674724964 ) ) ;
#6150=CARTESIAN_POINT ( 'NONE',  ( -14.90772019895849709, 120.8072429308574414, -0.9794594453158805836 ) ) ;
#6151=ORIENTED_EDGE ( 'NONE', *, *, #38941, .T. ) ;
#6153=CARTESIAN_POINT ( 'NONE',  ( -3.022581645176320553, 156.1079525116674631, 0.4343475099915219961 ) ) ;
#6154=CARTESIAN_POINT ( 'NONE',  ( 5.218988718559132600, -14.41095047787725747, 3.833162268628383718 ) ) ;
#6155=CARTESIAN_POINT ( 'NONE',  ( -5.008987216574991130, 117.3966124399498199, 0.7756614662348499944 ) ) ;
#6156=CARTESIAN_POINT ( 'NONE',  ( -4.635334609548626084, 118.0286145527519039, -0.7659634255356302379 ) ) ;
#6157=CARTESIAN_POINT ( 'NONE',  ( 15.64289809528657926, 147.2198192248932571, 0.2613308799247722747 ) ) ;
#6158=B_SPLINE_CURVE_WITH_KNOTS ( 'NONE', 3,
 ( #16161, #19364, #16378, #3843, #30014, #29809, #12771, #35786, #649, #10420, #25761, #38768, #26396, #35996, #22548, #436, #19570, #13198, #22754, #39185, #13406, #9579, #23391, #36208, #22966, #6394, #32369, #38978, #3410, #23174, #11, #6599, #7030, #3199, #12977, #9786, #29383, #223, #9994, #36423, #25970, #6809, #29602, #10204, #33015, #13617, #16593, #19778, #32798 ),
 .UNSPECIFIED., .F., .F.,
 ( 4, 1, 1, 1, 1, 1, 1, 1, 1, 1, 1, 1, 1, 1, 1, 1, 1, 1, 1, 1, 1, 1, 1, 1, 1, 1, 1, 1, 1, 1, 1, 1, 1, 1, 1, 1, 1, 1, 1, 1, 1, 1, 1, 1, 1, 1, 4 ),
 ( 0.000000000000000000, 0.007812500000000000000, 0.01562500000000000000, 0.02343750000000000000, 0.03125000000000000000, 0.04687500000000000000, 0.06250000000000000000, 0.07812500000000000000, 0.09375000000000000000, 0.1093750000000000000, 0.1250000000000000000, 0.1406250000000000000, 0.1562500000000000000, 0.1875000000000000000, 0.2187500000000000000, 0.2500000000000000000, 0.2812500000000000000, 0.3125000000000000000, 0.3281250000000000000, 0.3437500000000000000, 0.3750000000000000000, 0.4062500000000000000, 0.4375000000000000000, 0.4687500000000000000, 0.5000000000000000000, 0.5312500000000000000, 0.5625000000000000000, 0.5937500000000000000, 0.6250000000000000000, 0.6562500000000000000, 0.6718750000000000000, 0.6875000000000000000, 0.7187500000000000000, 0.7500000000000000000, 0.7812500000000000000, 0.8125000000000000000, 0.8437500000000000000, 0.8750000000000000000, 0.8906250000000000000, 0.9062500000000000000, 0.9218750000000000000, 0.9375000000000000000, 0.9531250000000000000, 0.9687500000000000000, 0.9765625000000000000, 0.9843750000000000000, 1.000000000000000000 ),
 .UNSPECIFIED. ) ;
#6160=CARTESIAN_POINT ( 'NONE',  ( 13.64693284513001004, 123.6869008171703541, 1.914747182567867023 ) ) ;
#6161=CARTESIAN_POINT ( 'NONE',  ( 3.174366308151881810, 76.29346620154572634, 0.06343139340882768262 ) ) ;
#6162=CARTESIAN_POINT ( 'NONE',  ( 9.538359384048550993, 124.8019839352694476, 0.1905991205270211042 ) ) ;
#6163=CARTESIAN_POINT ( 'NONE',  ( -2.917496378899196774, 117.0242007548465608, 0.3950530357975751139 ) ) ;
#6166=CARTESIAN_POINT ( 'NONE',  ( 21.39485547647971586, 132.5159896776619917, 0.01683271311856786301 ) ) ;
#6173=CARTESIAN_POINT ( 'NONE',  ( -6.654617103318593247E-14, 104.6144662015457243, 1.534725424433578570E-31 ) ) ;
#6174=CARTESIAN_POINT ( 'NONE',  ( -4.600121016240784400, 118.0774895349771327, 0.5278871946396123116 ) ) ;
#6177=CARTESIAN_POINT ( 'NONE',  ( -5.008987216574991130, 117.3966124399498199, 0.7756614662348499944 ) ) ;
#6178=CARTESIAN_POINT ( 'NONE',  ( 3.500270007598507149, 118.6368327427319400, -0.7934551251016943585 ) ) ;
#6179=CARTESIAN_POINT ( 'NONE',  ( -7.643894675291609708, 124.7210964017841377, -0.1527028184316445991 ) ) ;
#6181=CARTESIAN_POINT ( 'NONE',  ( 4.720176955733354163, 117.9455280608507337, 0.8233293243692888508 ) ) ;
#6182=CARTESIAN_POINT ( 'NONE',  ( 3.216700609619024931, -14.42020774479446921, 2.887214088933996337 ) ) ;
#6183=CARTESIAN_POINT ( 'NONE',  ( -11.02756477914281419, 153.1537610418535849, -1.395931567138233076 ) ) ;
#6184=CARTESIAN_POINT ( 'NONE',  ( -1.783861003286922209, 115.7029489855490851, -1.723409893597471543 ) ) ;
#6187=CARTESIAN_POINT ( 'NONE',  ( 6.130181428581209069, 119.5149100643186983, -0.2724793030934817839 ) ) ;
#6188=CARTESIAN_POINT ( 'NONE',  ( -3.575075884023375394, 156.6183338678525558, -1.521800568792661013 ) ) ;
#6190=CARTESIAN_POINT ( 'NONE',  ( 5.078986093043053707, 82.13546620154573930, 0.1014902294541238092 ) ) ;
#6191=CARTESIAN_POINT ( 'NONE',  ( -4.358130382724847429, 115.7036741551124663, 1.373039722754557657 ) ) ;
#6192=CARTESIAN_POINT ( 'NONE',  ( 2.584458374606236841, 15.83607344512877368, 3.832284875798456447 ) ) ;
#6193=CARTESIAN_POINT ( 'NONE',  ( 3.185756255432559580, 159.4163042773305676, 0.6073767776667650109 ) ) ;
#6195=CARTESIAN_POINT ( 'NONE',  ( 0.8444020299261373319, 104.6144662015456674, -4.761538540800747121 ) ) ;
#6196=CARTESIAN_POINT ( 'NONE',  ( 3.394867371861720606, -15.19666007832035071, 3.108802900814295000 ) ) ;
#6197=CARTESIAN_POINT ( 'NONE',  ( -7.611130975157204048, 119.9600249249614592, 1.076879093209133664 ) ) ;
#6198=CARTESIAN_POINT ( 'NONE',  ( 0.9581548452940278349, 12.22225311242794099, 0.1719060106794997322 ) ) ;
#6199=CARTESIAN_POINT ( 'NONE',  ( 0.9340445150430609633, -0.5783478219614121008, -0.2901879621234355056 ) ) ;
#6200=ORIENTED_EDGE ( 'NONE', *, *, #29018, .T. ) ;
#6201=ORIENTED_EDGE ( 'NONE', *, *, #20106, .F. ) ;
#6203=CARTESIAN_POINT ( 'NONE',  ( 5.854120942168423269, 124.7508695889173111, 0.1197652058513697382 ) ) ;
#6205=CARTESIAN_POINT ( 'NONE',  ( -9.963230294258281106, 124.0638329749226330, 0.5989708749582572933 ) ) ;
#6206=DIRECTION ( 'NONE',  ( 0.01997839162482793751, 0.000000000000000000, -0.9998004120163608288 ) ) ;
#6207=CARTESIAN_POINT ( 'NONE',  ( 2.073997095138572000, -14.95492255878227894, 5.604884748988061105 ) ) ;
#6208=CARTESIAN_POINT ( 'NONE',  ( 18.00062125403720970, 147.1528319293316542, -1.577578161537398271 ) ) ;
#6209=CARTESIAN_POINT ( 'NONE',  ( -14.08011273344106939, 154.3735777161816429, -2.279704494881448884 ) ) ;
#6212=DIRECTION ( 'NONE',  ( -0.9998004120163608288, -5.205824365704082573E-17, -0.01997839162482763914 ) ) ;
#6213=CARTESIAN_POINT ( 'NONE',  ( -2.613675400483765010, 35.04346971370642905, 1.554312572134140424 ) ) ;
#6214=CARTESIAN_POINT ( 'NONE',  ( 11.35800195117471745, 128.2076764602477681, -0.1601657033123584928 ) ) ;
#6215=ORIENTED_EDGE ( 'NONE', *, *, #40126, .T. ) ;
#6218=CARTESIAN_POINT ( 'NONE',  ( -3.216045294022573664, 29.79186273158684983, 3.430717191674401700 ) ) ;
#6219=CARTESIAN_POINT ( 'NONE',  ( 4.977872327462655733, 117.5914563484107447, -0.7726522923643426299 ) ) ;
#6220=CARTESIAN_POINT ( 'NONE',  ( 9.472608709197571031, 123.5188755717998816, 0.9573233835003832626 ) ) ;
#6221=DIRECTION ( 'NONE',  ( 0.9998004120163609398, 0.000000000000000000, 0.01997839162482749689 ) ) ;
#6222=CARTESIAN_POINT ( 'NONE',  ( 8.217303172778491316, 117.5015518944296247, 0.1195796404652191836 ) ) ;
#6223=CARTESIAN_POINT ( 'NONE',  ( -5.257173101726059450, 116.1034411669277375, 1.028648520082846574 ) ) ;
#6226=CARTESIAN_POINT ( 'NONE',  ( -3.391986336308672634, 31.79029220026756519, 0.7414760692215754956 ) ) ;
#6227=CARTESIAN_POINT ( 'NONE',  ( 20.88630183647680028, 148.3608207065297222, 2.399927473325583094 ) ) ;
#6228=CARTESIAN_POINT ( 'NONE',  ( 5.478597439045088890, 28.15663318097115209, -6.435035585623773535 ) ) ;
#6229=CARTESIAN_POINT ( 'NONE',  ( 2.190996476981287966, 116.7774030019725444, -0.4241678434939673004 ) ) ;
#6230=CARTESIAN_POINT ( 'NONE',  ( -0.08587196332417050548, 108.5751225745497806, -4.267111774705384164 ) ) ;
#6231=CARTESIAN_POINT ( 'NONE',  ( -22.66375647020940320, 150.6386093215953679, -0.4528757910175281731 ) ) ;
#6232=CARTESIAN_POINT ( 'NONE',  ( 4.854633716284414646, 115.7029491485453292, -1.279498648767039448 ) ) ;
#6233=CARTESIAN_POINT ( 'NONE',  ( 1.821748264913740423, 104.6144662015434932, 5.025386274610280424 ) ) ;
#6235=CARTESIAN_POINT ( 'NONE',  ( -4.151662239014343392, 13.23730288530712862, 2.070234887608822572 ) ) ;
#6238=CARTESIAN_POINT ( 'NONE',  ( 3.131463087139035206, -14.49961247625831895, 3.567833873788547550 ) ) ;
#6239=CARTESIAN_POINT ( 'NONE',  ( 1.803835135052165084, 120.9773948236336878, -0.3431470217397347144 ) ) ;
#6240=CARTESIAN_POINT ( 'NONE',  ( -8.157450159232212172, 117.7673425867732249, 0.3794901880580580644 ) ) ;
#6242=DIRECTION ( 'NONE',  ( 0.9998004120163608288, 0.000000000000000000, 0.01997839162482749342 ) ) ;
#6246=CARTESIAN_POINT ( 'NONE',  ( 2.438853454531733966, -15.63545089637397112, 5.735818209389550226 ) ) ;
#6247=CARTESIAN_POINT ( 'NONE',  ( -12.92430874792265350, 121.9120276846612256, 1.237792553996327261 ) ) ;
#6248=CARTESIAN_POINT ( 'NONE',  ( 14.74288075364456674, 121.6338672040446767, -0.8423781477486336211 ) ) ;
#6249=CARTESIAN_POINT ( 'NONE',  ( 4.440276399826426967, -1.430929408009915083, -1.287880193523989636 ) ) ;
#6253=CARTESIAN_POINT ( 'NONE',  ( -0.06282972276541670675, 111.5577547982949227, 3.144256248693278355 ) ) ;
#6254=CARTESIAN_POINT ( 'NONE',  ( -17.21539028065174293, 147.4900653055648547, 1.363477025422525024 ) ) ;
#6255=CARTESIAN_POINT ( 'NONE',  ( 5.010184479710102501, 117.3993854065330851, 0.7504461923096029663 ) ) ;
#6256=CARTESIAN_POINT ( 'NONE',  ( 3.316780243214140889, 119.1333808041459577, -0.7607270569537704086 ) ) ;
#6257=CARTESIAN_POINT ( 'NONE',  ( -2.699166815671299346, 158.5977336698458089, -1.597229775447004396 ) ) ;
#6260=CARTESIAN_POINT ( 'NONE',  ( 4.380560454800319192, 118.1845274366070129, -0.4312657318652557970 ) ) ;
#6261=CARTESIAN_POINT ( 'NONE',  ( 9.625125523471051991, 124.0356975489027036, -0.4152212053287653304 ) ) ;
#6262=ORIENTED_EDGE ( 'NONE', *, *, #11061, .T. ) ;
#6263=CARTESIAN_POINT ( 'NONE',  ( -2.024284171598574655, 156.9412006218898057, -1.489060257140892407 ) ) ;
#6264=CARTESIAN_POINT ( 'NONE',  ( 2.120377039319510715, -15.39027815159008128, 5.169171589912422426 ) ) ;
#6266=CARTESIAN_POINT ( 'NONE',  ( -4.111767271380013078, 118.2429491485453070, -0.3463599732680077148 ) ) ;
#6269=CARTESIAN_POINT ( 'NONE',  ( -4.825021315912614739, 117.6416127849941802, 0.9313223449158248846 ) ) ;
#6270=CARTESIAN_POINT ( 'NONE',  ( 7.307041242074578058, 120.9764928074160082, 1.161154363956387492 ) ) ;
#6272=CARTESIAN_POINT ( 'NONE',  ( 1.580769961479467911, 28.79261460129497863, -4.363931058323818668 ) ) ;
#6273=CARTESIAN_POINT ( 'NONE',  ( 7.868938471672396240, 154.6027768716304820, 0.5345728592648683053 ) ) ;
#6280=DIRECTION ( 'NONE',  ( -4.017660918040594346E-17, 1.000000000000000000, 2.376309959284834438E-19 ) ) ;
#6284=CARTESIAN_POINT ( 'NONE',  ( -0.9295402922912642252, 116.5712332538976455, 0.1496640007645970161 ) ) ;
#6288=CARTESIAN_POINT ( 'NONE',  ( -7.813505862531938462, 122.4480138429351683, -0.5609622212283363885 ) ) ;
#6289=ORIENTED_EDGE ( 'NONE', *, *, #32124, .F. ) ;
#6290=CARTESIAN_POINT ( 'NONE',  ( 1.199038730579973677, 115.7029469957295191, -1.697507966841996563 ) ) ;
#6291=CARTESIAN_POINT ( 'NONE',  ( -9.611064403080925800, 124.8310256250372277, -0.2802631513932193896 ) ) ;
#6292=CARTESIAN_POINT ( 'NONE',  ( 2.083301838685661878, -15.46665383083971257, 5.961979448439955753 ) ) ;
#6293=CARTESIAN_POINT ( 'NONE',  ( -12.31483450803191104, 120.4651188882986759, 0.9715887866197354672 ) ) ;
#6295=CIRCLE ( 'NONE', #30093, 0.5080000000000002292 ) ;
#6296=CARTESIAN_POINT ( 'NONE',  ( 23.16647984970247620, 149.6103952014060212, 0.7935852015942148618 ) ) ;
#6297=CARTESIAN_POINT ( 'NONE',  ( 7.537398615003564117, 122.4256905169532388, 0.2304582891925715249 ) ) ;
#6299=CARTESIAN_POINT ( 'NONE',  ( -0.08934464221186895483, 15.61415217803747169, 0.9739947352787643453 ) ) ;
#6300=CARTESIAN_POINT ( 'NONE',  ( -17.17229002331743004, 122.7237354506536491, -0.5096938506424069093 ) ) ;
#6303=CARTESIAN_POINT ( 'NONE',  ( -8.715372737337569120, 118.1578756808219168, 0.5461737873414159727 ) ) ;
#6306=CARTESIAN_POINT ( 'NONE',  ( 5.844526503020529340, 118.0670013439590491, 1.005764768584936686 ) ) ;
#6307=CARTESIAN_POINT ( 'NONE',  ( 3.207104841129760242, 118.4902560533893592, -0.7629184910595987468 ) ) ;
#6308=CARTESIAN_POINT ( 'NONE',  ( -6.647063868753328997, 9.619588520696709111, 5.217091374630535405 ) ) ;
#6309=CARTESIAN_POINT ( 'NONE',  ( -21.32959265000934579, 150.3702682424204511, -2.003547396033109163 ) ) ;
#6310=CARTESIAN_POINT ( 'NONE',  ( 4.646224276046603485, 117.9817966608726323, -0.7219288950694058293 ) ) ;
#6311=CARTESIAN_POINT ( 'NONE',  ( 6.937169949972861183, 121.8132169909553966, 0.2949249740950675158 ) ) ;
#6313=CARTESIAN_POINT ( 'NONE',  ( -9.568355480995553108, 124.8108731098830049, -0.1557749891131962605 ) ) ;
#6314=CARTESIAN_POINT ( 'NONE',  ( -0.4763900686813665741, 119.0154928070276412, -0.6070730232697146844 ) ) ;
#6315=CARTESIAN_POINT ( 'NONE',  ( 3.081975983035755373, -15.74694164559999088, 5.217090789712465870 ) ) ;
#6317=EDGE_CURVE ( 'NONE', #5065, #14379, #10490, .T. ) ;
#6320=CARTESIAN_POINT ( 'NONE',  ( 18.42282194684149133, 148.3462492009778373, 2.436111078577046118 ) ) ;
#6321=DIRECTION ( 'NONE',  ( 0.9998004120163608288, 0.000000000000000000, 0.01997839162482749342 ) ) ;
#6324=CARTESIAN_POINT ( 'NONE',  ( -2.721163413801487518, 112.7379566594982663, 2.570110030560514680 ) ) ;
#6325=CARTESIAN_POINT ( 'NONE',  ( -7.524129562762011503, 22.75916136179084859, 3.848622047589015160 ) ) ;
#6326=CARTESIAN_POINT ( 'NONE',  ( 3.037839899925966147, 156.1243923452879017, 0.6481072647156853606 ) ) ;
#6328=CARTESIAN_POINT ( 'NONE',  ( 15.53115535783863699, 121.4967652112180048, -0.4657050394012308692 ) ) ;
#6329=DIRECTION ( 'NONE',  ( -0.01997839162482761832, -1.040247600000950455E-18, 0.9998004120163610509 ) ) ;
#6332=AXIS2_PLACEMENT_3D ( 'NONE', #39010, #36607, #10604 ) ;
#6333=CARTESIAN_POINT ( 'NONE',  ( -23.41930689910524421, 142.8308675865925181, -0.4425677471174259137 ) ) ;
#6335=CARTESIAN_POINT ( 'NONE',  ( 4.871727757954943172, 119.9531087571945136, -0.7028895344987076133 ) ) ;
#6336=CARTESIAN_POINT ( 'NONE',  ( 4.210393360348192004, -15.14515747025066084, 4.947006310901637782 ) ) ;
#6337=CARTESIAN_POINT ( 'NONE',  ( -15.96902210417531620, 146.0164801329953548, -1.048924711619906969 ) ) ;
#6338=CARTESIAN_POINT ( 'NONE',  ( 4.295506980234458538, -13.52603301450379369, 3.694598940018447575 ) ) ;
#6340=CARTESIAN_POINT ( 'NONE',  ( 9.819578298035914088, 117.9942579372833933, 0.2115136170467759036 ) ) ;
#6341=ORIENTED_EDGE ( 'NONE', *, *, #25441, .T. ) ;
#6342=CARTESIAN_POINT ( 'NONE',  ( 3.263621351691376571, 8.939281053574255509, -3.290156819607050753 ) ) ;
#6343=ADVANCED_FACE ( 'NONE', ( #16877, #33505 ), #20694, .F. ) ;
#6344=CARTESIAN_POINT ( 'NONE',  ( -2.123093575600416560, 105.1241855340452247, 4.902909873598239265 ) ) ;
#6345=CARTESIAN_POINT ( 'NONE',  ( -4.976634676106532318, 117.4097617497457975, 0.8837896011837403920 ) ) ;
#6347=CARTESIAN_POINT ( 'NONE',  ( -5.036351857865265735, 117.3993844875897139, 0.5494637324817667201 ) ) ;
#6348=CARTESIAN_POINT ( 'NONE',  ( -7.902730875908052788, 122.1217003200704028, 0.5555494452425332463 ) ) ;
#6350=CARTESIAN_POINT ( 'NONE',  ( -4.422273941422524501, 8.986318502778324557, 1.404945367500548548 ) ) ;
#6351=CARTESIAN_POINT ( 'NONE',  ( 7.681555067352521249, 158.5863655655865330, 1.054772010160867080 ) ) ;
#6352=CARTESIAN_POINT ( 'NONE',  ( -0.03519895178523997636, 115.7029491485446613, 1.761499482104069703 ) ) ;
#6353=CARTESIAN_POINT ( 'NONE',  ( 4.967439785005383968, 118.2512723699127832, -0.8146033317824222797 ) ) ;
#6354=CARTESIAN_POINT ( 'NONE',  ( -4.468841950160419962, 8.124252568732815760, -1.173904233648782158 ) ) ;
#6355=CARTESIAN_POINT ( 'NONE',  ( -15.49230080900824369, 121.3130774642648220, -1.004719031932798767 ) ) ;
#6357=ORIENTED_EDGE ( 'NONE', *, *, #2992, .F. ) ;
#6358=CARTESIAN_POINT ( 'NONE',  ( -6.164480127824659483, 155.3548635187015350, 0.4492659787150439232 ) ) ;
#6359=CARTESIAN_POINT ( 'NONE',  ( 2.081461833008368512, -15.42522581128935499, 5.972092850182497692 ) ) ;
#6361=CARTESIAN_POINT ( 'NONE',  ( 15.77260762454789322, 146.5697412905949477, 0.2637713227210860545 ) ) ;
#6362=ORIENTED_EDGE ( 'NONE', *, *, #14169, .F. ) ;
#6363=CARTESIAN_POINT ( 'NONE',  ( 13.08242246048928514, 122.4605402651681487, 1.816276721775475611 ) ) ;
#6365=CARTESIAN_POINT ( 'NONE',  ( 8.112862105095262066, 122.9271997657419604, 0.1621142923985558204 ) ) ;
#6366=CARTESIAN_POINT ( 'NONE',  ( -14.73113557689553588, 120.8948172685174001, 0.5329945393104404960 ) ) ;
#6367=FACE_OUTER_BOUND ( 'NONE', #2092, .T. ) ;
#6368=CARTESIAN_POINT ( 'NONE',  ( 6.918545264603641165, 117.3320596397172721, -0.2494728033470789974 ) ) ;
#6369=CARTESIAN_POINT ( 'NONE',  ( -4.800085724567980883, 115.7029491485352537, -1.472342921364584889 ) ) ;
#6373=CARTESIAN_POINT ( 'NONE',  ( -4.937504354476867086, 117.4086944262769237, -1.082066183473587850 ) ) ;
#6377=CARTESIAN_POINT ( 'NONE',  ( -4.579105009936609960, 118.0741109548545467, 0.5987129210286493697 ) ) ;
#6378=LINE ( 'NONE', #10406, #10431 ) ;
#6382=CARTESIAN_POINT ( 'NONE',  ( -4.800388046789877627, 115.6909491485452719, -1.474219336061443952 ) ) ;
#6383=CARTESIAN_POINT ( 'NONE',  ( 5.961890394766238721, 119.1281689002219082, -1.026328349456139488 ) ) ;
#6384=CARTESIAN_POINT ( 'NONE',  ( -7.065765265293135755, 122.4340714744230496, -0.2508917249367680902 ) ) ;
#6385=CARTESIAN_POINT ( 'NONE',  ( 4.707952333973207892, 117.9523840734817810, 0.8425572090526738389 ) ) ;
#6387=CARTESIAN_POINT ( 'NONE',  ( -9.210551279805695657, 123.0263237342149978, -1.033454686166954017 ) ) ;
#6390=CARTESIAN_POINT ( 'NONE',  ( -0.4328386126936296097, 105.9953805924852333, 5.278113798800131207 ) ) ;
#6392=CARTESIAN_POINT ( 'NONE',  ( 4.047044637104031395, 109.8183322527596602, -3.518666775989008677 ) ) ;
#6393=CARTESIAN_POINT ( 'NONE',  ( -15.77815547270824936, 139.7295799824062499, -1.909820663798255103 ) ) ;
#6394=CARTESIAN_POINT ( 'NONE',  ( -0.03256023585726924852, 157.9544661776888290, 1.629447346748784664 ) ) ;
#6396=CARTESIAN_POINT ( 'NONE',  ( -3.594857975007920814, -7.703025367003809798, -2.923569511714296798 ) ) ;
#6397=CARTESIAN_POINT ( 'NONE',  ( 0.9591953284561349768, 116.7682604261274264, 0.2970936445032630879 ) ) ;
#6400=CARTESIAN_POINT ( 'NONE',  ( 2.813987013336220144, -15.51818976969260255, 4.585835125202748053 ) ) ;
#6402=CARTESIAN_POINT ( 'NONE',  ( -17.77426102521102536, 149.9241642446907292, 1.728420094174573318 ) ) ;
#6403=CARTESIAN_POINT ( 'NONE',  ( -0.9660709935815289251, 7.903159174923253261, 0.1333004412508401459 ) ) ;
#6405=CARTESIAN_POINT ( 'NONE',  ( -0.08510646190747463147, 11.08924109716144280, -0.9717149503703566005 ) ) ;
#6409=CARTESIAN_POINT ( 'NONE',  ( 4.819599041176311438, 120.7138498849978987, 0.4051376471031730708 ) ) ;
#6410=CARTESIAN_POINT ( 'NONE',  ( -0.01596947694136538129, 156.4635559983122448, 0.7991779281049289363 ) ) ;
#6411=CARTESIAN_POINT ( 'NONE',  ( 3.231995002093183800, -14.34039573884512997, 4.866605245980782257 ) ) ;
#6412=CARTESIAN_POINT ( 'NONE',  ( 7.412650754288764077, 120.7277362223577768, -0.9451843054385554721 ) ) ;
#6413=AXIS2_PLACEMENT_3D ( 'NONE', #9612, #22581, #9822 ) ;
#6414=CARTESIAN_POINT ( 'NONE',  ( -19.09066119453658317, 140.9752145814059645, -2.516632075137498870 ) ) ;
#6416=CARTESIAN_POINT ( 'NONE',  ( 8.212088287371502204, 120.4194928741279256, 1.432818887811018405 ) ) ;
#6417=CARTESIAN_POINT ( 'NONE',  ( -1.123920628080118167, 36.51502492732748095, 0.1267022063819566724 ) ) ;
#6418=CARTESIAN_POINT ( 'NONE',  ( 9.747124062405188027, 124.8671652961716489, -0.04776528062357090348 ) ) ;
#6422=CARTESIAN_POINT ( 'NONE',  ( 4.988558773217932618, 117.5914558864278519, -0.6981965400864760252 ) ) ;
#6423=CARTESIAN_POINT ( 'NONE',  ( 12.48065534322204151, 152.0704867801853766, 1.458211671286262057 ) ) ;
#6425=CARTESIAN_POINT ( 'NONE',  ( 10.82496502431732210, 157.9086237439880733, 0.1564342443379709291 ) ) ;
#6426=CARTESIAN_POINT ( 'NONE',  ( -0.8805184999823391090, 105.9455060897651748, 5.280965183963572507 ) ) ;
#6429=CARTESIAN_POINT ( 'NONE',  ( -4.273992351614648300, 31.99305554651359174, 0.5394102745547180167 ) ) ;
#6430=CARTESIAN_POINT ( 'NONE',  ( 13.36424875645652932, 155.6061939908119882, 2.069718186823302108 ) ) ;
#6431=CARTESIAN_POINT ( 'NONE',  ( 0.1277143096572389558, 15.67076514537015974, -4.628409624684062251 ) ) ;
#6432=CARTESIAN_POINT ( 'NONE',  ( -2.078203845413400863, -12.60517393744602721, -8.197436486331740824 ) ) ;
#6433=CARTESIAN_POINT ( 'NONE',  ( 8.743324216112098313, 118.0100196136648236, -0.4276613644598801223 ) ) ;
#6434=CARTESIAN_POINT ( 'NONE',  ( -0.7422006451358510448, 119.7070660435176279, -0.6877902101425065196 ) ) ;
#6436=CARTESIAN_POINT ( 'NONE',  ( 0.6265181353984804469, 106.0244491581631223, -5.258298658868172382 ) ) ;
#6437=CARTESIAN_POINT ( 'NONE',  ( -1.776898248692639903, 105.1238429332592688, 5.030869823623774550 ) ) ;
#6438=CARTESIAN_POINT ( 'NONE',  ( -3.562413952978887632, 23.18266144714348798, 2.948169924785601470 ) ) ;
#6441=CARTESIAN_POINT ( 'NONE',  ( 2.994295736468014280, -14.77441112906794984, 3.968895097548184037 ) ) ;
#6442=CARTESIAN_POINT ( 'NONE',  ( 1.600813358578667245, 118.7759820277219944, -0.7642889039740424773 ) ) ;
#6443=CARTESIAN_POINT ( 'NONE',  ( -3.828842504638848787, 116.8938343318378088, 0.2916468201809274130 ) ) ;
#6444=ORIENTED_EDGE ( 'NONE', *, *, #25155, .T. ) ;
#6449=CARTESIAN_POINT ( 'NONE',  ( 4.647714231081432779, -15.48178215826023774, 3.998406189266252131 ) ) ;
#6450=CARTESIAN_POINT ( 'NONE',  ( -12.47042458399958953, 121.5863879130357503, 1.220378502515000019 ) ) ;
#6451=CARTESIAN_POINT ( 'NONE',  ( 21.51971352461169573, 150.2128557559047692, -1.148904605754655250 ) ) ;
#6453=CARTESIAN_POINT ( 'NONE',  ( 1.968029828064305153, -3.592386099649644837, 4.203610184747879508 ) ) ;
#6457=CARTESIAN_POINT ( 'NONE',  ( -0.08519874065850288614, 108.5751225745497948, 4.263693374914160117 ) ) ;
#6458=CARTESIAN_POINT ( 'NONE',  ( 4.756911902486301358, 117.3993836135862949, 1.207145067066230038 ) ) ;
#6459=CARTESIAN_POINT ( 'NONE',  ( -10.84737219364650329, 123.3109526380878833, 1.071866780254096208 ) ) ;
#6461=CARTESIAN_POINT ( 'NONE',  ( 18.75354316333441673, 144.8948545501563103, -1.742436930347202040 ) ) ;
#6462=CARTESIAN_POINT ( 'NONE',  ( -20.49864673575787677, 149.5144255282053223, -2.384675166241297273 ) ) ;
#6465=CARTESIAN_POINT ( 'NONE',  ( 4.569713780653100521, 118.0880689344100034, -0.5677796928598370929 ) ) ;
#6466=CARTESIAN_POINT ( 'NONE',  ( 7.714568708787782114, 122.2455405838764335, -0.3552802434219701211 ) ) ;
#6467=VERTEX_POINT ( 'NONE', #41578 ) ;
#6468=CARTESIAN_POINT ( 'NONE',  ( -13.78929608597947620, 128.5353789189983900, -1.909663635655581393 ) ) ;
#6469=CARTESIAN_POINT ( 'NONE',  ( 3.885732391871624447, -15.29168275415018741, 1.106840230638412192 ) ) ;
#6470=DIRECTION ( 'NONE',  ( 4.017660918040594346E-17, -1.000000000000000000, -2.376309959284834438E-19 ) ) ;
#6472=CARTESIAN_POINT ( 'NONE',  ( -4.805526376074356953, 117.7656062655381675, 0.8575794806940943982 ) ) ;
#6473=CARTESIAN_POINT ( 'NONE',  ( -0.008945177888024442511, 119.9096241394016715, 0.4476532798976759486 ) ) ;
#6475=CARTESIAN_POINT ( 'NONE',  ( -2.201963191602333225, 30.07953629247752758, -4.075912811544394998 ) ) ;
#6476=CARTESIAN_POINT ( 'NONE',  ( 14.23422759389726977, 138.9464670490549452, 0.5149110934774582260 ) ) ;
#6480=LINE ( 'NONE', #17102, #25058 ) ;
#6482=DIRECTION ( 'NONE',  ( 4.017660918040594346E-17, -1.000000000000000000, -2.376309959284834438E-19 ) ) ;
#6487=CARTESIAN_POINT ( 'NONE',  ( -23.39020171064290210, 146.7932648766621639, -0.1331748977937666500 ) ) ;
#6490=CARTESIAN_POINT ( 'NONE',  ( -6.948590427472591813, 121.9371117883950006, -0.2862137248287923152 ) ) ;
#6491=ORIENTED_EDGE ( 'NONE', *, *, #28031, .T. ) ;
#6492=CARTESIAN_POINT ( 'NONE',  ( 1.039317103187317404, 115.7029401488263147, -1.708817239941311295 ) ) ;
#6493=CARTESIAN_POINT ( 'NONE',  ( -15.73804366022566548, 146.9052959264698757, -0.5443085878246288756 ) ) ;
#6494=CARTESIAN_POINT ( 'NONE',  ( 5.936869294410564990, -12.97241973064336484, 1.608696005067407953 ) ) ;
#6495=CARTESIAN_POINT ( 'NONE',  ( -7.954494586186919847, 118.5968412048868288, 0.8561882949445159818 ) ) ;
#6496=CARTESIAN_POINT ( 'NONE',  ( -5.152689475313444234, 116.8412042432202185, -0.1029630068797482562 ) ) ;
#6497=CARTESIAN_POINT ( 'NONE',  ( 22.62002883431060596, 150.6357905964555925, 0.7802727354960533601 ) ) ;
#6498=CARTESIAN_POINT ( 'NONE',  ( 9.460061892327653155, 124.7787809139916106, 0.2814990181333890118 ) ) ;
#6499=CARTESIAN_POINT ( 'NONE',  ( 4.765531619307481925, 118.5266822147775940, -0.8412287920200557378 ) ) ;
#6500=CARTESIAN_POINT ( 'NONE',  ( 0.05603342037570913786, 10.86776798020533086, -0.9749832093204870986 ) ) ;
#6501=CARTESIAN_POINT ( 'NONE',  ( -21.54627550604365638, 132.6250929350426020, -0.6335863061179134448 ) ) ;
#6503=EDGE_CURVE ( 'NONE', #40008, #34211, #3667, .T. ) ;
#6507=CARTESIAN_POINT ( 'NONE',  ( 8.685978770867098575, 118.1606796386214455, 0.8960457658865661479 ) ) ;
#6510=CARTESIAN_POINT ( 'NONE',  ( 9.779442063456341927, 157.5983698538113629, 1.672576317993901496 ) ) ;
#6511=CARTESIAN_POINT ( 'NONE',  ( 11.29660330931799450, 121.3367100885591015, -1.243740200939188911 ) ) ;
#6512=CARTESIAN_POINT ( 'NONE',  ( 0.9749890475506259868, 2.950361319068162569, -0.03356295239053608964 ) ) ;
#6513=CARTESIAN_POINT ( 'NONE',  ( -2.748994976520039213, 10.49642266832308124, 7.958378898918418543 ) ) ;
#6514=CARTESIAN_POINT ( 'NONE',  ( -15.42726980375961965, 123.0316835747794642, -1.591438994230370829 ) ) ;
#6515=CARTESIAN_POINT ( 'NONE',  ( 4.662377642780485942, 117.9838022724669457, -0.7074655422033281349 ) ) ;
#6516=CARTESIAN_POINT ( 'NONE',  ( 1.987587706212191385, 106.6795586461009009, 4.969950645211479667 ) ) ;
#6517=CARTESIAN_POINT ( 'NONE',  ( -4.599243292695419427, 121.2024757821991159, -0.09190382657876447481 ) ) ;
#6519=CARTESIAN_POINT ( 'NONE',  ( -18.35995883219828073, 144.7751241387205425, -2.452750363274776468 ) ) ;
#6520=CARTESIAN_POINT ( 'NONE',  ( 5.215289103204772125, -15.32183344268082870, 2.967178555186370303 ) ) ;
#6524=CARTESIAN_POINT ( 'NONE',  ( 5.554730375462953340, 156.7050554705274408, 1.852363956736410744 ) ) ;
#6527=CARTESIAN_POINT ( 'NONE',  ( -4.418733742721505209, 119.2572634999566930, 0.4175613206465203509 ) ) ;
#6528=CARTESIAN_POINT ( 'NONE',  ( -8.293629857537270667, 31.38027257336059250, -1.381021427861755635 ) ) ;
#6529=CARTESIAN_POINT ( 'NONE',  ( 15.96686920080697725, 146.6619865182943272, 1.046663894505766912 ) ) ;
#6531=CARTESIAN_POINT ( 'NONE',  ( 3.161282452094233975, 159.3671203531505114, -0.6484678655804383407 ) ) ;
#6533=CARTESIAN_POINT ( 'NONE',  ( 5.317570146058844038, 115.7029491485453150, -0.5111954518035258799 ) ) ;
#6535=PRODUCT_DEFINITION_CONTEXT ( 'detailed design', #25946, 'design' ) ;
#6537=CARTESIAN_POINT ( 'NONE',  ( -22.53594553814350832, 150.7843406352268687, -0.4248312833800680921 ) ) ;
#6538=ORIENTED_EDGE ( 'NONE', *, *, #7707, .T. ) ;
#6539=CARTESIAN_POINT ( 'NONE',  ( 5.026392434963103284, 120.1182786053553002, -0.6754308463122872253 ) ) ;
#6540=CARTESIAN_POINT ( 'NONE',  ( 4.032974650908811576, -15.19488190071041345, 5.088841723123956662 ) ) ;
#6541=CARTESIAN_POINT ( 'NONE',  ( -12.24221062544605942, 130.6044139104978115, -0.7866602228194182755 ) ) ;
#6542=CARTESIAN_POINT ( 'NONE',  ( 2.527534073033691708, -14.76126024938119485, 5.399385249886175409 ) ) ;
#6544=CARTESIAN_POINT ( 'NONE',  ( -0.0002511744761471925336, 116.4254662015457171, 0.01256979787922185565 ) ) ;
#6547=CARTESIAN_POINT ( 'NONE',  ( 1.719524320724281852, 5.915668354077112667, 4.300554535892874064 ) ) ;
#6548=CARTESIAN_POINT ( 'NONE',  ( 5.140088096925614636, 105.1220910292376800, 1.436521125592880255 ) ) ;
#6549=CARTESIAN_POINT ( 'NONE',  ( -4.976778051443659479, 117.4086891970763560, 0.8838977329282806661 ) ) ;
#6551=CARTESIAN_POINT ( 'NONE',  ( -6.107213356235562607, 121.2381221225252830, 0.3743496410843655808 ) ) ;
#6552=CARTESIAN_POINT ( 'NONE',  ( 4.233688895176465294, 13.94658232072815807, -1.861163356065342001 ) ) ;
#6553=CARTESIAN_POINT ( 'NONE',  ( 22.22261828963529595, 149.8733841865972920, 1.744734864234219085 ) ) ;
#6555=CARTESIAN_POINT ( 'NONE',  ( 3.369285701246146569, 109.1383298698278566, 3.951686121084368342 ) ) ;
#6556=CARTESIAN_POINT ( 'NONE',  ( 7.892561109811804698, 118.8455990504009492, -0.9355921144164880410 ) ) ;
#6557=CARTESIAN_POINT ( 'NONE',  ( 4.099978103716023448, 4.450953565018914482, -2.131961072590273343 ) ) ;
#6558=CARTESIAN_POINT ( 'NONE',  ( -15.38653228232040782, 121.5363848317736739, -1.155577132538254448 ) ) ;
#6561=B_SPLINE_CURVE_WITH_KNOTS ( 'NONE', 3,
 ( #6369, #15936, #12953, #32141, #28932, #41950 ),
 .UNSPECIFIED., .F., .F.,
 ( 4, 2, 4 ),
 ( 0.000000000000000000, 0.5000000000000000000, 1.000000000000000000 ),
 .UNSPECIFIED. ) ;
#6564=CARTESIAN_POINT ( 'NONE',  ( -3.712124141557985979, 121.0264708767875561, 0.07522066808841054719 ) ) ;
#6565=VECTOR ( 'NONE', #2140, 1000.000000000000227 ) ;
#6566=CARTESIAN_POINT ( 'NONE',  ( 4.852936394019410571, -14.31369683153947747, 4.236952399839363892 ) ) ;
#6569=EDGE_CURVE ( 'NONE', #39307, #38156, #9192, .T. ) ;
#6570=CARTESIAN_POINT ( 'NONE',  ( 10.57181108402524039, 155.7851685111067184, 2.170362527570921962 ) ) ;
#6573=CARTESIAN_POINT ( 'NONE',  ( -11.30743779403340277, 119.0414093155750379, 0.5171725168954618423 ) ) ;
#6575=CARTESIAN_POINT ( 'NONE',  ( 6.918378865934368349, 117.2797055272990292, -0.1815168674402108384 ) ) ;
#6580=CARTESIAN_POINT ( 'NONE',  ( 2.164775582100227247, -15.10189236760869846, 5.710855967119448096 ) ) ;
#6581=EDGE_CURVE ( 'NONE', #39868, #22781, #3208, .T. ) ;
#6584=CARTESIAN_POINT ( 'NONE',  ( -4.531800530025674512, 118.0871158275990069, 0.6067528179264731758 ) ) ;
#6588=FACE_OUTER_BOUND ( 'NONE', #31664, .T. ) ;
#6589=CARTESIAN_POINT ( 'NONE',  ( -8.337209054434152833, 119.8086030055221869, -1.438699114785731537 ) ) ;
#6590=CARTESIAN_POINT ( 'NONE',  ( -5.571761382372367066, 117.9391977826196296, -0.7470240521525300936 ) ) ;
#6591=CARTESIAN_POINT ( 'NONE',  ( 4.675781884360660001, 117.9791009951701000, 0.8445612169912808387 ) ) ;
#6592=CARTESIAN_POINT ( 'NONE',  ( 3.047145566129288330, -14.72663143740328806, 3.823360744794035870 ) ) ;
#6593=CARTESIAN_POINT ( 'NONE',  ( -8.534279067096813165, 122.4751019636825049, -0.9739960529120706978 ) ) ;
#6594=CARTESIAN_POINT ( 'NONE',  ( -4.800085724567980883, 115.7029491485352537, -1.472342921364584889 ) ) ;
#6595=CARTESIAN_POINT ( 'NONE',  ( -1.351554245314562586, 106.2775040229277153, 5.112464471456568127 ) ) ;
#6596=CARTESIAN_POINT ( 'NONE',  ( -4.711190372662979797, 117.8992862897405871, -0.9551895239324142972 ) ) ;
#6597=CARTESIAN_POINT ( 'NONE',  ( 4.488494058616853799, 111.2667756541687538, -2.954587190001159325 ) ) ;
#6598=CARTESIAN_POINT ( 'NONE',  ( -11.67499187284231610, 153.3684197651487580, -1.838730530730911861 ) ) ;
#6599=CARTESIAN_POINT ( 'NONE',  ( -0.02874415600673332558, 157.0795416643300939, 1.438475106415294302 ) ) ;
#6600=CARTESIAN_POINT ( 'NONE',  ( -3.658134704041837271, 115.7029491485453434, 1.477887315928634759 ) ) ;
#6601=CARTESIAN_POINT ( 'NONE',  ( -3.781325196301324354, 121.0927823605408662, -0.005689350045973306028 ) ) ;
#6602=CARTESIAN_POINT ( 'NONE',  ( 0.05711764529616595448, 0.5181683540770933849, -4.631227783250111862 ) ) ;
#6603=CARTESIAN_POINT ( 'NONE',  ( 22.11976774214178931, 136.9573810088325843, 1.270382039940954222 ) ) ;
#6605=DIRECTION ( 'NONE',  ( 0.9998004120163609398, 0.000000000000000000, 0.01997839162482749689 ) ) ;
#6606=CARTESIAN_POINT ( 'NONE',  ( 3.431757876926103012, -15.17734022545018391, 2.935651181724953318 ) ) ;
#6607=CARTESIAN_POINT ( 'NONE',  ( -11.47069961394323201, 122.2847249198043471, 1.269327653809199985 ) ) ;
#6608=CARTESIAN_POINT ( 'NONE',  ( 0.3177745610913299545, 14.38516025884261929, -0.9235644396001725376 ) ) ;
#6610=CARTESIAN_POINT ( 'NONE',  ( -23.16247218334359559, 146.6831645211815101, -1.199661776592803264 ) ) ;
#6611=AXIS2_PLACEMENT_3D ( 'NONE', #39520, #3747, #13526 ) ;
#6612=CARTESIAN_POINT ( 'NONE',  ( -0.7366970693195243891, 2.667464547469879488, -0.6395729927624468347 ) ) ;
#6614=ORIENTED_EDGE ( 'NONE', *, *, #37079, .F. ) ;
#6616=CARTESIAN_POINT ( 'NONE',  ( 1.966029823418392608, 106.7001829816230725, 4.962286218837188123 ) ) ;
#6618=CARTESIAN_POINT ( 'NONE',  ( -15.06908741399251817, 148.9283877096812034, 0.6536164350837786463 ) ) ;
#6619=CARTESIAN_POINT ( 'NONE',  ( 3.464659682708206123, -14.15734315221130224, 4.609430909834149048 ) ) ;
#6620=CARTESIAN_POINT ( 'NONE',  ( 17.55799248491146614, 146.4615580561186050, -1.465990265564338646 ) ) ;
#6622=CARTESIAN_POINT ( 'NONE',  ( -4.132678194918598003, 118.9132445967212419, -1.007338114003851315 ) ) ;
#6624=CARTESIAN_POINT ( 'NONE',  ( 8.261346106638972842, 120.1775813921023399, 1.448714831781537260 ) ) ;
#6625=CARTESIAN_POINT ( 'NONE',  ( -5.231323785280036276, 32.40695963756544273, 1.837218211224142861 ) ) ;
#6626=B_SPLINE_CURVE_WITH_KNOTS ( 'NONE', 3,
 ( #4421, #35573, #6596, #219, #26976, #38974 ),
 .UNSPECIFIED., .F., .F.,
 ( 4, 2, 4 ),
 ( 0.000000000000000000, 0.0001566688501089290775, 0.0003133377002178581549 ),
 .UNSPECIFIED. ) ;
#6627=CARTESIAN_POINT ( 'NONE',  ( 2.792630161979468006, 120.9517662584847102, -0.08501465617163896094 ) ) ;
#6631=CARTESIAN_POINT ( 'NONE',  ( -0.1064799869811820787, 105.7853621660184444, 5.332934571178567396 ) ) ;
#6635=CARTESIAN_POINT ( 'NONE',  ( 18.62524206359421086, 154.1412379532633850, 0.2279367985168735955 ) ) ;
#6637=CARTESIAN_POINT ( 'NONE',  ( -6.519249125050614602, 120.6419738463991536, 0.1350556763279783523 ) ) ;
#6638=CIRCLE ( 'NONE', #12072, 3.175000000000001155 ) ;
#6640=CARTESIAN_POINT ( 'NONE',  ( -3.259680568650582977, 115.6909491485508852, 1.531580627320187293 ) ) ;
#6641=CARTESIAN_POINT ( 'NONE',  ( 2.862861873098513588, -10.07698056833738320, -3.640125809621840069 ) ) ;
#6642=CARTESIAN_POINT ( 'NONE',  ( -5.212520885064538589, 31.45212241211192605, -0.4657032193360505778 ) ) ;
#6643=CARTESIAN_POINT ( 'NONE',  ( 6.769736154946609297, 118.6475953829349379, 1.187203428762516388 ) ) ;
#6644=CARTESIAN_POINT ( 'NONE',  ( 2.551181839206869917, 14.82117702134586779, -3.857898856385788999 ) ) ;
#6645=CARTESIAN_POINT ( 'NONE',  ( 6.556273983038449771, -14.34328088419217728, -5.323198733142235461 ) ) ;
#6646=CARTESIAN_POINT ( 'NONE',  ( -8.731353435635694993, 117.9558915041894522, -0.7268751822057367695 ) ) ;
#6647=CARTESIAN_POINT ( 'NONE',  ( -0.2286055872010028245, 108.3383513567250986, -4.353007566726654787 ) ) ;
#6648=CARTESIAN_POINT ( 'NONE',  ( -23.36121599383904623, 148.8756354987168606, -0.4668126921610641911 ) ) ;
#6649=CARTESIAN_POINT ( 'NONE',  ( 3.222817655156935412, 108.4800784852299955, -4.089130794945939229 ) ) ;
#6650=CARTESIAN_POINT ( 'NONE',  ( -2.420033166307097972, 104.6144662015456959, 4.756650020785883726 ) ) ;
#6651=CARTESIAN_POINT ( 'NONE',  ( -4.460028654926622593, 22.53297844546955631, 1.214995109042491528 ) ) ;
#6652=FACE_OUTER_BOUND ( 'NONE', #30275, .T. ) ;
#6654=CARTESIAN_POINT ( 'NONE',  ( 3.162791966164926638, -14.44121541014482801, 3.416220915275241854 ) ) ;
#6655=CARTESIAN_POINT ( 'NONE',  ( 2.219425127536471809, 123.7320667226965867, -0.04105829392232412944 ) ) ;
#6656=CARTESIAN_POINT ( 'NONE',  ( -16.70010949199491179, 122.7093839631038463, 0.3053630257279365545 ) ) ;
#6660=VERTEX_POINT ( 'NONE', #15354 ) ;
#6661=CARTESIAN_POINT ( 'NONE',  ( -0.7387659178326329013, 32.94979111317254450, 0.8178967711910589689 ) ) ;
#6662=CARTESIAN_POINT ( 'NONE',  ( 6.000997576644805598, -14.76005184138509740, 0.6970346396957283197 ) ) ;
#6663=CARTESIAN_POINT ( 'NONE',  ( -11.27973791692654260, 156.1341193432522800, 1.681596738997434892 ) ) ;
#6664=CARTESIAN_POINT ( 'NONE',  ( 14.51588022701130676, 121.7426775721902175, -0.9381456983900905433 ) ) ;
#6665=CARTESIAN_POINT ( 'NONE',  ( 3.746277899330032302, -0.8937244826341392834, -2.755274729908455900 ) ) ;
#6667=ORIENTED_EDGE ( 'NONE', *, *, #2714, .F. ) ;
#6668=CARTESIAN_POINT ( 'NONE',  ( 5.078986093043053707, 85.18346620154574111, 0.1014902294541244060 ) ) ;
#6669=CARTESIAN_POINT ( 'NONE',  ( 0.3746108773302438966, 122.5569158606515003, 0.2627672029693577382 ) ) ;
#6670=CARTESIAN_POINT ( 'NONE',  ( 0.000000000000000000, 0.000000000000000000, 0.000000000000000000 ) ) ;
#6671=CARTESIAN_POINT ( 'NONE',  ( -9.584070499013474631, 122.7780075402122151, 0.8664194973949997935 ) ) ;
#6673=CARTESIAN_POINT ( 'NONE',  ( 5.067974813687860625, 119.5555251685854330, -0.8659238720033421988 ) ) ;
#6674=CARTESIAN_POINT ( 'NONE',  ( -19.44881300980853922, 136.0480396440595996, -2.307899331309747559 ) ) ;
#6676=ORIENTED_EDGE ( 'NONE', *, *, #2235, .F. ) ;
#6677=CARTESIAN_POINT ( 'NONE',  ( 4.496309931980947638, 118.1299276439104631, -0.5226211628217811711 ) ) ;
#6678=CARTESIAN_POINT ( 'NONE',  ( 15.94526953466029973, 147.3275361421020193, -0.5311500221062649407 ) ) ;
#6679=ORIENTED_EDGE ( 'NONE', *, *, #22807, .T. ) ;
#6680=CARTESIAN_POINT ( 'NONE',  ( -17.64033768477188246, 147.6919162452172145, -2.236185705752640196 ) ) ;
#6681=CARTESIAN_POINT ( 'NONE',  ( 2.294714809908028119, -15.51018114022951977, 5.078884642465592236 ) ) ;
#6682=CARTESIAN_POINT ( 'NONE',  ( 3.682264917456193665, 66.13346620154572975, 0.07358041635424013294 ) ) ;
#6684=CARTESIAN_POINT ( 'NONE',  ( -4.746868605287419385, 117.7551308511543198, 0.8963948101134247004 ) ) ;
#6685=CARTESIAN_POINT ( 'NONE',  ( 13.52836484031751496, 128.5255724691869830, 1.838026323690954422 ) ) ;
#6686=CARTESIAN_POINT ( 'NONE',  ( -2.190119082386309035, 30.63587144615187086, 1.931548619664235522 ) ) ;
#6688=CARTESIAN_POINT ( 'NONE',  ( 2.598967704003971146, -9.625211180298204994, -8.041545772114961466 ) ) ;
#6689=CARTESIAN_POINT ( 'NONE',  ( 0.6475778113725148000, 156.3069099058775748, 0.1429049811405687098 ) ) ;
#6692=CARTESIAN_POINT ( 'NONE',  ( 2.185739921021631726, 116.1876150569675730, -0.001408202639197844719 ) ) ;
#6693=CARTESIAN_POINT ( 'NONE',  ( -4.017108196799733300, 117.3993836135118158, 1.174877857344739596 ) ) ;
#6695=CARTESIAN_POINT ( 'NONE',  ( 3.174366308151880922, 104.6144662015457243, 0.06343139340882769650 ) ) ;
#6696=DIRECTION ( 'NONE',  ( 0.9998004120163608288, 0.000000000000000000, 0.01997839162482760791 ) ) ;
#6698=CARTESIAN_POINT ( 'NONE',  ( 5.078986093043053707, 87.97746620154572383, 0.1014902294541237954 ) ) ;
#6702=CARTESIAN_POINT ( 'NONE',  ( -17.11470313646614727, 122.7072422303320707, -0.09880859551014491149 ) ) ;
#6703=ORIENTED_EDGE ( 'NONE', *, *, #36211, .T. ) ;
#6705=CARTESIAN_POINT ( 'NONE',  ( -6.048481876759730369, 121.4346570564865857, -0.1338841272842773988 ) ) ;
#6706=AXIS2_PLACEMENT_3D ( 'NONE', #13070, #39920, #26060 ) ;
#6709=CARTESIAN_POINT ( 'NONE',  ( -7.044165191775566548, 122.0728772437221323, -0.1705051815768210965 ) ) ;
#6710=CARTESIAN_POINT ( 'NONE',  ( 3.428369065731536658, -15.18705194980916851, 5.515041984116586526 ) ) ;
#6711=CARTESIAN_POINT ( 'NONE',  ( -21.08161885447505313, 149.3892802667211868, 1.460526482899864531 ) ) ;
#6712=CARTESIAN_POINT ( 'NONE',  ( 8.196043946343802844, 117.5568930537867800, 0.4237257472399769131 ) ) ;
#6713=CARTESIAN_POINT ( 'NONE',  ( 0.6484723942714255562, 120.9972571750055579, 0.07908818383241446315 ) ) ;
#6714=FACE_OUTER_BOUND ( 'NONE', #18886, .T. ) ;
#6715=CARTESIAN_POINT ( 'NONE',  ( -0.7518944845272079736, 4.819152178039351142, 0.6255420797857809134 ) ) ;
#6716=CARTESIAN_POINT ( 'NONE',  ( -22.81319227411009365, 150.4043717142618277, -0.6849243123989297022 ) ) ;
#6720=CARTESIAN_POINT ( 'NONE',  ( 8.600551643892799802, 118.5561038629244592, 1.113272402564501995 ) ) ;
#6722=CARTESIAN_POINT ( 'NONE',  ( -16.17691485933977091, 135.1141785778430346, 1.596016904437364881 ) ) ;
#6724=CARTESIAN_POINT ( 'NONE',  ( 10.72975491961945593, 119.6772744462923157, 1.366487948980413369 ) ) ;
#6725=CARTESIAN_POINT ( 'NONE',  ( 12.99265913520512683, 122.2940260782629451, -1.284300974089672920 ) ) ;
#6726=CARTESIAN_POINT ( 'NONE',  ( 0.5559618826558695437, 1.427253112428326753, 0.7990736944121461516 ) ) ;
#6728=CARTESIAN_POINT ( 'NONE',  ( -19.51124600060716929, 152.2820370773569323, -1.942483913431541920 ) ) ;
#6729=CARTESIAN_POINT ( 'NONE',  ( 4.807494110098772921, 117.8776439329783017, -0.6745073813406683438 ) ) ;
#6730=CARTESIAN_POINT ( 'NONE',  ( 6.733859895263996975, 121.2177056076135528, 0.3428974583126989661 ) ) ;
#6731=CARTESIAN_POINT ( 'NONE',  ( 9.413719431533399629, 122.9055586947561522, -0.7725895697485186675 ) ) ;
#6732=CARTESIAN_POINT ( 'NONE',  ( -15.64289809528671071, 147.2198192248932571, -0.2613308799247720526 ) ) ;
#6734=CARTESIAN_POINT ( 'NONE',  ( -2.214684683099673812, 157.4004113605966211, -1.675081295071568110 ) ) ;
#6735=CARTESIAN_POINT ( 'NONE',  ( 4.376329468599289285, -15.53264713215277126, 4.356271056886698467 ) ) ;
#6739=CARTESIAN_POINT ( 'NONE',  ( 7.432183457866615051, 120.4750020944285609, 1.305203700904508546 ) ) ;
#6744=CARTESIAN_POINT ( 'NONE',  ( -1.593197492609443433, 110.3135721340718334, 3.506749948187484645 ) ) ;
#6745=CARTESIAN_POINT ( 'NONE',  ( 7.636339006008190822, 27.50728337528610012, -3.595707551023701765 ) ) ;
#6746=CARTESIAN_POINT ( 'NONE',  ( 11.59282501421104783, 128.2970750771678752, 0.8590849294959500559 ) ) ;
#6747=CARTESIAN_POINT ( 'NONE',  ( 22.86776170061652280, 148.6346580502994073, -0.6251136566479097434 ) ) ;
#6750=CARTESIAN_POINT ( 'NONE',  ( -15.72215902125780751, 120.8394623874526275, -0.2972128523334375272 ) ) ;
#6752=CARTESIAN_POINT ( 'NONE',  ( -7.950921552827399985, 121.7269089819065329, -1.084193410159759452 ) ) ;
#6753=CARTESIAN_POINT ( 'NONE',  ( 22.66375647020927531, 150.6386093215953395, 0.4528757910175285062 ) ) ;
#6754=CARTESIAN_POINT ( 'NONE',  ( -13.78138926674715314, 150.2278160098252329, -0.9796190600867306086 ) ) ;
#6755=CARTESIAN_POINT ( 'NONE',  ( 3.821280252649200460, -11.76149679029331274, 0.6556923638117722053 ) ) ;
#6757=CARTESIAN_POINT ( 'NONE',  ( 23.41829197008351215, 142.8308675865925181, 0.4933589455792337652 ) ) ;
#6759=CARTESIAN_POINT ( 'NONE',  ( -4.636761822055341042, 12.60011390031314349, 0.2095705037016724059 ) ) ;
#6760=CARTESIAN_POINT ( 'NONE',  ( -4.612917339777265369, 105.1215402076766878, 2.701253017043198312 ) ) ;
#6761=CARTESIAN_POINT ( 'NONE',  ( -4.855027809809237205, 117.4045417072194226, 0.9983932867329968763 ) ) ;
#6763=CARTESIAN_POINT ( 'NONE',  ( -7.930528998391228157, 121.9940456953541741, 0.6366723744063579327 ) ) ;
#6765=CARTESIAN_POINT ( 'NONE',  ( -2.065029617914060367, 6.824861272777455135, -4.134893973632223663 ) ) ;
#6766=CARTESIAN_POINT ( 'NONE',  ( 15.11776246977249905, 121.4505734225448066, 1.235019191190165344 ) ) ;
#6767=CARTESIAN_POINT ( 'NONE',  ( 15.19943428492308080, 148.1072807477730748, 0.3037208696559882681 ) ) ;
#6770=CARTESIAN_POINT ( 'NONE',  ( 5.882407806703735531, 118.3130479344264501, -0.8400364453129069986 ) ) ;
#6771=CARTESIAN_POINT ( 'NONE',  ( 4.577905313181523717, 13.52175256873284326, -0.6256056815880789435 ) ) ;
#6772=CARTESIAN_POINT ( 'NONE',  ( -8.098994982418762589, 117.9016134627522945, -0.8176261169560977704 ) ) ;
#6774=CARTESIAN_POINT ( 'NONE',  ( -6.491509040565048849, 121.7133186976561205, 0.1169240713195678211 ) ) ;
#6775=CARTESIAN_POINT ( 'NONE',  ( 3.596007053926196573, -14.96754207850672991, 5.407624617413868684 ) ) ;
#6777=CARTESIAN_POINT ( 'NONE',  ( 3.026662605148213725, -13.87242449132548217, 1.205013440933411228 ) ) ;
#6779=CARTESIAN_POINT ( 'NONE',  ( -0.01152893261320977157, 118.7114655739656257, 0.5769549317675699562 ) ) ;
#6781=CARTESIAN_POINT ( 'NONE',  ( 3.174366308151880922, 95.34346620154573770, 0.06343139340882768262 ) ) ;
#6782=CARTESIAN_POINT ( 'NONE',  ( -10.46273137052137336, 157.8855781193960297, 0.6617911890761500882 ) ) ;
#6784=CARTESIAN_POINT ( 'NONE',  ( -0.5057995593169576365, 15.89392266832286182, -8.404578209849391968 ) ) ;
#6785=ADVANCED_FACE ( 'NONE', ( #13431 ), #35870, .F. ) ;
#6786=CARTESIAN_POINT ( 'NONE',  ( 23.22389216488245722, 148.7951734159264561, -0.1326450332456384218 ) ) ;
#6791=CARTESIAN_POINT ( 'NONE',  ( -4.812686597042231895, 117.4055138428619784, -1.197175370899103752 ) ) ;
#6793=DIRECTION ( 'NONE',  ( 0.9998004120163608288, 4.016384292689131511E-17, 0.01997839162482749342 ) ) ;
#6794=CARTESIAN_POINT ( 'NONE',  ( -4.527558639897409698, 118.1161936615429084, 0.5308642384113577695 ) ) ;
#6798=CARTESIAN_POINT ( 'NONE',  ( -1.075895380385707201, 115.6909491485452577, -1.747627985865146227 ) ) ;
#6799=CARTESIAN_POINT ( 'NONE',  ( 4.019189700197100201, 119.1285266303971753, -0.7637224803080886470 ) ) ;
#6800=CARTESIAN_POINT ( 'NONE',  ( -7.618479139564731106, 124.7215218652630710, -0.1522353441811850894 ) ) ;
#6801=CARTESIAN_POINT ( 'NONE',  ( 4.603208726993124777, 118.0397272544194180, 0.8064533428228448653 ) ) ;
#6803=CARTESIAN_POINT ( 'NONE',  ( -14.24959175664888633, 150.3563008155378213, -1.527850727897531291 ) ) ;
#6806=CARTESIAN_POINT ( 'NONE',  ( 7.475619626241481797, 123.6620266863018855, 0.1149006695610369777 ) ) ;
#6807=CARTESIAN_POINT ( 'NONE',  ( -16.40533521683946816, 148.4304801786341272, -1.905158959863711088 ) ) ;
#6809=CARTESIAN_POINT ( 'NONE',  ( -0.008148072696648066618, 156.3406798448389168, 0.4077628766201955579 ) ) ;
#6810=CARTESIAN_POINT ( 'NONE',  ( 8.635102817405984510, 118.5712416014077206, -0.7746300195078601458 ) ) ;
#6811=CARTESIAN_POINT ( 'NONE',  ( -10.39718957393781551, 153.1349757784973349, -0.1475885461366300277 ) ) ;
#6812=CARTESIAN_POINT ( 'NONE',  ( 0.09481320634720795393, -4.229605868409334057, 4.636458411128852930 ) ) ;
#6813=CARTESIAN_POINT ( 'NONE',  ( 20.39753840605626678, 152.5480347002736607, 1.233721349276552637 ) ) ;
#6815=CARTESIAN_POINT ( 'NONE',  ( 3.239928030326187258, -14.81799142783181367, -0.3301716407829758948 ) ) ;
#6816=CARTESIAN_POINT ( 'NONE',  ( -19.29290905409802903, 147.1635184732690220, 1.739861672056419728 ) ) ;
#6817=CARTESIAN_POINT ( 'NONE',  ( -0.9360807938713975318, 7.254031735439380846, -0.2770855581244007215 ) ) ;
#6818=CARTESIAN_POINT ( 'NONE',  ( -23.18613385382707648, 148.9919839608952827, -1.059503902452021418 ) ) ;
#6819=CARTESIAN_POINT ( 'NONE',  ( 0.9751244372034794106, -10.72340290332181567, 0.05698045496536860433 ) ) ;
#6822=AXIS2_PLACEMENT_3D ( 'NONE', #5131, #34927, #11483 ) ;
#6824=CARTESIAN_POINT ( 'NONE',  ( 4.699507673534768948, 115.8251506319059843, 1.445723734630264046 ) ) ;
#6826=CARTESIAN_POINT ( 'NONE',  ( -16.18586682243777020, 146.0959698922748942, 0.6488728679227169227 ) ) ;
#6827=CARTESIAN_POINT ( 'NONE',  ( 3.811713748825880543, -11.77916328849872052, 0.6977653098966205558 ) ) ;
#6828=CARTESIAN_POINT ( 'NONE',  ( 14.44833386134782316, 131.1674235819977241, -1.369607862251506436 ) ) ;
#6829=CARTESIAN_POINT ( 'NONE',  ( -7.650403556475662725, 119.6133147451300971, -1.381840873585064688 ) ) ;
#6831=CARTESIAN_POINT ( 'NONE',  ( 2.969447359227861405, -13.80100253337253946, 0.9847735008004718793 ) ) ;
#6832=CARTESIAN_POINT ( 'NONE',  ( -3.999880774356848523, 33.21692059697370070, 1.336717509662867620 ) ) ;
#6833=CARTESIAN_POINT ( 'NONE',  ( 14.24343488940565194, 138.9464670490549452, 0.05414037600900938746 ) ) ;
#6835=CARTESIAN_POINT ( 'NONE',  ( -5.024436415346294815, 113.9634239268893339, 1.916893372365422454 ) ) ;
#6838=TOROIDAL_SURFACE ( 'NONE', #25284, 5.080000000000005400, 0.5080000000000000071 ) ;
#6841=CARTESIAN_POINT ( 'NONE',  ( 11.70725067560570309, 118.7242475115495495, 0.1376448473428155683 ) ) ;
#6842=CARTESIAN_POINT ( 'NONE',  ( -2.184544675938124403, 106.6795586461009009, 4.886581511092879637 ) ) ;
#6843=TOROIDAL_SURFACE ( 'NONE', #23828, 3.683000000000000718, 0.5080000000000000071 ) ;
#6844=CARTESIAN_POINT ( 'NONE',  ( -0.03523692298175334220, 115.6909491485452435, 1.763399716048406285 ) ) ;
#6845=B_SPLINE_CURVE_WITH_KNOTS ( 'NONE', 3,
 ( #39253, #10060, #710, #13681, #19848, #501, #26462, #39466, #10269, #26673, #39681, #23453 ),
 .UNSPECIFIED., .F., .F.,
 ( 4, 2, 1, 2, 1, 2, 4 ),
 ( 0.000000000000000000, 0.1250000000000000000, 0.2500000000000000000, 0.5000000000000000000, 0.7500000000000000000, 0.8750000000000000000, 1.000000000000000000 ),
 .UNSPECIFIED. ) ;
#6847=CARTESIAN_POINT ( 'NONE',  ( -3.633364037744279074, 31.58192510899068850, 0.2531645344678472020 ) ) ;
#6849=CARTESIAN_POINT ( 'NONE',  ( 13.53750608930579169, 121.6867650304669013, 1.656372850109685269 ) ) ;
#6850=CARTESIAN_POINT ( 'NONE',  ( -0.2796867633624597893, 20.41853924017881283, 4.627572958784220702 ) ) ;
#6851=CARTESIAN_POINT ( 'NONE',  ( -1.087716277807347254, 29.42523365726748708, -8.383486966309323662 ) ) ;
#6852=CARTESIAN_POINT ( 'NONE',  ( -2.169812748839434313, 116.7701370764819586, -0.5085666708809641889 ) ) ;
#6853=CARTESIAN_POINT ( 'NONE',  ( 0.02647280040252846661, 106.0860833631645193, -5.252669131072539521 ) ) ;
#6856=CARTESIAN_POINT ( 'NONE',  ( 2.891928348976603225, 104.6144662015456959, 3.864987668791159070 ) ) ;
#6857=CARTESIAN_POINT ( 'NONE',  ( 1.111903444298625754, 15.29877551736591812, 4.515507465039587665 ) ) ;
#6860=CARTESIAN_POINT ( 'NONE',  ( 2.104008947125556528, -15.14483647969354330, 5.217645225406672971 ) ) ;
#6861=CARTESIAN_POINT ( 'NONE',  ( 2.298002300860023439, 118.5759350612125900, -0.7369678581462181244 ) ) ;
#6862=CARTESIAN_POINT ( 'NONE',  ( -22.93637923037195137, 149.5023856264156450, 0.3943874666890925806 ) ) ;
#6863=CARTESIAN_POINT ( 'NONE',  ( 7.383526128983457504, 117.2783386326274524, 0.1475404238727041073 ) ) ;
#6868=CARTESIAN_POINT ( 'NONE',  ( 4.276943344491330734, -15.69687736684960377, 3.951204673509490117 ) ) ;
#6869=CARTESIAN_POINT ( 'NONE',  ( -20.15738656758755099, 148.0303212619860744, 1.701566911850819208 ) ) ;
#6871=CARTESIAN_POINT ( 'NONE',  ( 1.273577801943096999, 159.1407128229522527, -1.197834500974594096 ) ) ;
#6872=CARTESIAN_POINT ( 'NONE',  ( 0.7580923926444932404, 28.79380631387826028, -0.6184068814828035388 ) ) ;
#6877=CARTESIAN_POINT ( 'NONE',  ( -0.02887436318431864379, 106.7790779034713324, 4.972892908546473478 ) ) ;
#6878=SURFACE_STYLE_USAGE ( .BOTH. , #36064 ) ;
#6880=CARTESIAN_POINT ( 'NONE',  ( -16.46834812293206340, 148.4304801786341272, 1.248264531716813508 ) ) ;
#6881=CARTESIAN_POINT ( 'NONE',  ( -5.946078212987909062, 28.42590610009758478, 0.3016625663984517924 ) ) ;
#6883=CARTESIAN_POINT ( 'NONE',  ( 11.50890483677792453, 122.9335272575421669, -1.234163556480095014 ) ) ;
#6885=CARTESIAN_POINT ( 'NONE',  ( -13.83539046132058203, 122.2371923977168109, -1.727333621972642064 ) ) ;
#6889=CARTESIAN_POINT ( 'NONE',  ( 4.404749925360578189, 118.1622680122423077, -0.4911679557709572874 ) ) ;
#6890=CARTESIAN_POINT ( 'NONE',  ( 15.47786622725289973, 148.0679034673509875, -0.4116497765502034611 ) ) ;
#6891=VERTEX_POINT ( 'NONE', #33 ) ;
#6892=CARTESIAN_POINT ( 'NONE',  ( -10.89299388415068037, 123.1276765127550021, -1.556224048961160733 ) ) ;
#6893=CARTESIAN_POINT ( 'NONE',  ( 3.043194142253923928, -14.61827878651010515, -0.2680077959190000358 ) ) ;
#6894=CARTESIAN_POINT ( 'NONE',  ( -3.156656716243205096, 105.1239622688229645, -4.301121616660518399 ) ) ;
#6896=CARTESIAN_POINT ( 'NONE',  ( -2.734508853367146219, 0.3528594962865297391, 3.724956791467788353 ) ) ;
#6897=CARTESIAN_POINT ( 'NONE',  ( 0.5409540667463921260, 119.9180165495073283, 0.4819738915938378554 ) ) ;
#6898=CARTESIAN_POINT ( 'NONE',  ( 1.544194705859216921, 35.01746917326339315, 0.8070499108633334417 ) ) ;
#6900=CARTESIAN_POINT ( 'NONE',  ( 7.741462187161934239, -10.92447321953606654, -3.338652055795839679 ) ) ;
#6901=CARTESIAN_POINT ( 'NONE',  ( 10.25892126925246295, 126.0184183664171655, 0.2980827979995014365 ) ) ;
#6905=CARTESIAN_POINT ( 'NONE',  ( 3.174366308151881366, 82.64346620154573486, 0.06343139340882768262 ) ) ;
#6906=VECTOR ( 'NONE', #20175, 1000.000000000000000 ) ;
#6907=DIRECTION ( 'NONE',  ( 4.017660918040594346E-17, -1.000000000000000000, -2.376309959284834438E-19 ) ) ;
#6909=CARTESIAN_POINT ( 'NONE',  ( -8.133186750442957802, 120.8103564082440613, -1.375394817141416981 ) ) ;
#6910=CARTESIAN_POINT ( 'NONE',  ( 3.164706401634689303, 50.63946620154572997, 1.543954388298181213 ) ) ;
#6912=DIRECTION ( 'NONE',  ( -0.9998004120163610509, -4.016384292689131511E-17, -0.01997839162482749689 ) ) ;
#6915=CARTESIAN_POINT ( 'NONE',  ( -8.212232005054575623, 117.5299140688306352, 0.02651185805045446278 ) ) ;
#6919=CARTESIAN_POINT ( 'NONE',  ( -6.056369948572695172, 121.4335403551348804, -0.1264477557253972650 ) ) ;
#6921=DIRECTION ( 'NONE',  ( 0.01997839162482749689, 1.040247600000945640E-18, -0.9998004120163610509 ) ) ;
#6922=CARTESIAN_POINT ( 'NONE',  ( -11.83578944268997724, 152.0103986367769551, -0.2843524715992693519 ) ) ;
#6923=CARTESIAN_POINT ( 'NONE',  ( 6.383535934857802907, -12.90002020050165576, 0.3830569482466484321 ) ) ;
#6924=CARTESIAN_POINT ( 'NONE',  ( -14.04756362465215247, 122.1591959312462592, 1.132115996748545239 ) ) ;
#6925=CARTESIAN_POINT ( 'NONE',  ( 3.043391175932955495, 18.63480288530714191, -3.501419995799015528 ) ) ;
#6926=CARTESIAN_POINT ( 'NONE',  ( 23.32660363739032761, 146.7646281656787437, 0.9249455126139315420 ) ) ;
#6927=CARTESIAN_POINT ( 'NONE',  ( 15.71643150686912627, 145.6795463615453059, 0.5158341164768996956 ) ) ;
#6929=CARTESIAN_POINT ( 'NONE',  ( 0.9169382621377788478, -11.15192339915171793, 0.3232733857163304081 ) ) ;
#6930=CARTESIAN_POINT ( 'NONE',  ( -22.64824804725711971, 137.2763855621842026, -0.6699328029008018159 ) ) ;
#6931=CARTESIAN_POINT ( 'NONE',  ( -6.651972016613293606E-14, 104.1064662015457287, 7.011588703784780528E-31 ) ) ;
#6933=EDGE_LOOP ( 'NONE', ( #25025, #23634, #38060, #5306 ) ) ;
#6934=CARTESIAN_POINT ( 'NONE',  ( -2.190925350822380047, 116.2108782439287467, -0.0004523116112769919148 ) ) ;
#6936=CARTESIAN_POINT ( 'NONE',  ( -18.08730999440964027, 147.8422069945528108, 1.617706263729447924 ) ) ;
#6938=CARTESIAN_POINT ( 'NONE',  ( 12.00897459848969007, 120.6765805525287334, 1.550193712165491178 ) ) ;
#6939=CARTESIAN_POINT ( 'NONE',  ( 19.17595810167853898, 140.9752145814059645, -1.751973952106583576 ) ) ;
#6940=CARTESIAN_POINT ( 'NONE',  ( -0.2928493810785644524, 9.627489959316354984, 0.9317482488014678932 ) ) ;
#6942=CARTESIAN_POINT ( 'NONE',  ( -21.45663756426511526, 150.2128557559047692, -2.007674378541678628 ) ) ;
#6943=CARTESIAN_POINT ( 'NONE',  ( 4.572607118633827739, 118.0342741157669053, -0.6784189215572231646 ) ) ;
#6946=CARTESIAN_POINT ( 'NONE',  ( 6.134665891606675636, 119.5049778551863682, 0.5179261928985369190 ) ) ;
#6948=CARTESIAN_POINT ( 'NONE',  ( 5.877307974080531849, 120.8872308857076519, -0.5842564153471765387 ) ) ;
#6949=CARTESIAN_POINT ( 'NONE',  ( -15.76486438913732613, 145.9085485750152316, -0.2635089261703655317 ) ) ;
#6950=ORIENTED_EDGE ( 'NONE', *, *, #9615, .F. ) ;
#6951=CARTESIAN_POINT ( 'NONE',  ( -5.042934966769651695, 119.7208665877771665, -1.041708725922360523 ) ) ;
#6952=CARTESIAN_POINT ( 'NONE',  ( 4.389818247250405037, -15.68135102926887470, 3.766867903159812681 ) ) ;
#6953=CARTESIAN_POINT ( 'NONE',  ( -4.590154465017951324, 118.0230796030913893, -0.8584153040694411096 ) ) ;
#6956=CARTESIAN_POINT ( 'NONE',  ( 11.42611330002548087, 154.6851215890897038, 2.167138196937119066 ) ) ;
#6957=CARTESIAN_POINT ( 'NONE',  ( -0.5321123018419734452, 37.22158963861809156, -0.7300149017649124605 ) ) ;
#6958=DIRECTION ( 'NONE',  ( -0.9998004120163608288, 0.000000000000000000, -0.01997839162482749342 ) ) ;
#6959=CARTESIAN_POINT ( 'NONE',  ( -4.802295984089328229, 116.4582014290525507, 0.9960034115346418915 ) ) ;
#6960=CARTESIAN_POINT ( 'NONE',  ( -0.9765287272027848298, 24.25689591457997452, 8.364652468500624494 ) ) ;
#6961=CARTESIAN_POINT ( 'NONE',  ( 10.72508252498916725, 126.1521286088116369, 0.7954780730053834237 ) ) ;
#6962=CARTESIAN_POINT ( 'NONE',  ( 22.81445126409626667, 149.1304179266472261, -0.6239350898115070265 ) ) ;
#6965=B_SPLINE_CURVE_WITH_KNOTS ( 'NONE', 3,
 ( #8112, #40710, #21086, #7497, #4315, #17062, #40304, #17897, #30899, #4732, #17684, #4519, #17279, #1739, #30268, #14698, #27703, #13876 ),
 .UNSPECIFIED., .F., .F.,
 ( 4, 2, 2, 2, 2, 2, 2, 2, 4 ),
 ( 0.0003740348303357290786, 0.003617653094789048760, 0.006861271359242368875, 0.008483080491469027415, 0.009293985057582358419, 0.01010488962369568942, 0.01172669875592231847, 0.01253760332203563213, 0.01334850788814894752 ),
 .UNSPECIFIED. ) ;
#6967=CARTESIAN_POINT ( 'NONE',  ( -9.820189317990269728, 117.9942579372833933, -0.1809356799706721142 ) ) ;
#6969=CARTESIAN_POINT ( 'NONE',  ( -6.748423061888915164, 121.1153472631275179, -0.9535781417299137308 ) ) ;
#6970=CARTESIAN_POINT ( 'NONE',  ( 5.718778735283957637, -14.43046299137125388, 2.876564826015278520 ) ) ;
#6971=CARTESIAN_POINT ( 'NONE',  ( -14.74011517316811215, 148.8440819608433969, -0.7404754567584957980 ) ) ;
#6972=CARTESIAN_POINT ( 'NONE',  ( 3.826441825042426359, -13.78667705120290066, 4.058770776067232688 ) ) ;
#6973=CARTESIAN_POINT ( 'NONE',  ( -13.66011217756167184, 120.8017016962898396, 0.8211468655896804192 ) ) ;
#6974=CARTESIAN_POINT ( 'NONE',  ( -15.19943428492320869, 148.1072807477730748, -0.3037208696559880461 ) ) ;
#6975=CARTESIAN_POINT ( 'NONE',  ( 8.075047650969494839, 158.6620026115301698, 0.1796671307923023986 ) ) ;
#6976=ORIENTED_EDGE ( 'NONE', *, *, #35539, .F. ) ;
#6977=CARTESIAN_POINT ( 'NONE',  ( -1.504723661876595786, -8.552649586842417051, -4.374500482163298898 ) ) ;
#6978=CARTESIAN_POINT ( 'NONE',  ( -6.894732321505390615, 117.1676844715483270, -0.1377731603346601386 ) ) ;
#6980=VECTOR ( 'NONE', #41214, 1000.000000000000000 ) ;
#6982=CARTESIAN_POINT ( 'NONE',  ( 6.614212317611555925, 120.0220961648606561, 1.233748940741835609 ) ) ;
#6983=ADVANCED_FACE ( 'NONE', ( #9810 ), #14560, .T. ) ;
#6984=CARTESIAN_POINT ( 'NONE',  ( 3.019445949670579665, 11.99742794009110014, 3.522755186455234000 ) ) ;
#6985=CARTESIAN_POINT ( 'NONE',  ( 14.16249321059112809, 121.1589565784038456, 1.397539518993202723 ) ) ;
#6986=CARTESIAN_POINT ( 'NONE',  ( -0.03707542933699707610, 115.3931862868688398, 1.855406091731380824 ) ) ;
#6988=CARTESIAN_POINT ( 'NONE',  ( 6.823161219633183450, 118.5360090424673274, -0.8871979454111537100 ) ) ;
#6989=CARTESIAN_POINT ( 'NONE',  ( 2.298459491326434900, 5.325542553220859787, -4.024866414273244430 ) ) ;
#6990=CARTESIAN_POINT ( 'NONE',  ( -6.882329627759522062, 117.5897289630162987, -0.7523600398187278993 ) ) ;
#6994=EDGE_LOOP ( 'NONE', ( #345, #8187, #28575 ) ) ;
#6995=CARTESIAN_POINT ( 'NONE',  ( -5.257554009420361218, 121.2670714900434206, 0.1164621724739934722 ) ) ;
#6996=CARTESIAN_POINT ( 'NONE',  ( 5.987854329437395151, -12.83555092537783082, 1.339350064115379935 ) ) ;
#6998=AXIS2_PLACEMENT_3D ( 'NONE', #26504, #6921, #39508 ) ;
#7001=CARTESIAN_POINT ( 'NONE',  ( 12.70837813489428569, 122.8260676081006153, 1.843161107213562966 ) ) ;
#7003=CARTESIAN_POINT ( 'NONE',  ( 12.85860202769631755, 133.7716054015561156, 0.2569454702854388484 ) ) ;
#7005=CARTESIAN_POINT ( 'NONE',  ( -18.09030135340804435, 154.0913862843578670, 0.7524810965364959747 ) ) ;
#7006=CARTESIAN_POINT ( 'NONE',  ( 3.518211725887771202, 24.73955407011506935, -7.658871095584262711 ) ) ;
#7008=CARTESIAN_POINT ( 'NONE',  ( 5.670663496353971489, 159.1134716836843381, -0.2862304005612824054 ) ) ;
#7009=DIRECTION ( 'NONE',  ( 5.206863593109713661E-17, -1.000000000000000000, 1.077750396879097183E-30 ) ) ;
#7012=CARTESIAN_POINT ( 'NONE',  ( 2.097955312704908870, -15.07800414366253250, 5.719157372618502322 ) ) ;
#7013=B_SPLINE_CURVE_WITH_KNOTS ( 'NONE', 3,
 ( #24294, #37928, #37501, #18526, #40716, #8751, #8327, #34325, #1950, #18315, #40920, #1743, #37300, #21297, #34534, #21713, #5154, #1538, #25143, #18108, #34737, #40515, #8542, #41349, #21091, #31531, #8117, #38147, #21501, #30688, #2161, #12151, #30904, #14910, #15120, #2375, #31113, #28123, #27506, #27914, #15335, #11726, #24714, #41133, #11939, #24930, #34115, #28340, #8960, #11307, #33908, #4942, #14702, #17901, #27707, #4736, #17689, #14493, #9173, #5780, #41558, #35788, #41973, #35361, #41769, #28550, #25557, #12978, #39187, #38561, #25971, #224, #35159, #12, #16379, #19160, #9374, #2999, #31745, #9580, #28756, #2588, #18949, #22338, #19365, #26183, #6600, #3200, #38358, #6191, #5986, #18735 ),
 .UNSPECIFIED., .F., .F.,
 ( 4, 2, 2, 2, 2, 2, 1, 1, 2, 2, 2, 2, 2, 2, 2, 2, 2, 1, 1, 2, 2, 2, 2, 1, 1, 2, 2, 2, 1, 2, 2, 1, 1, 2, 2, 2, 1, 1, 1, 2, 2, 2, 2, 2, 2, 2, 1, 1, 1, 1, 2, 2, 2, 4 ),
 ( 0.000000000000000000, 0.03125000000000136002, 0.04687500000000204003, 0.06250000000000273392, 0.09375000000000413558, 0.1093750000000048711, 0.1171875000000052458, 0.1210937500000054123, 0.1230468750000054678, 0.1250000000000055234, 0.1406250000000056899, 0.1484375000000058009, 0.1523437500000058287, 0.1562500000000058564, 0.1718750000000059119, 0.1875000000000059952, 0.2187500000000059952, 0.2343750000000059674, 0.2421875000000059119, 0.2460937500000058842, 0.2500000000000058287, 0.3125000000000036637, 0.3437500000000024980, 0.3593750000000018874, 0.3671875000000014988, 0.3710937500000013323, 0.3750000000000011657, 0.4062499999999998890, 0.4140624999999997224, 0.4160156249999996114, 0.4169921874999994449, 0.4179687499999992784, 0.4218749999999984457, 0.4374999999999966693, 0.4687499999999931166, 0.4843749999999915068, 0.4921874999999907296, 0.4960937499999902855, 0.4980468749999899525, 0.4990234374999898415, 0.4999999999999897304, 0.5624999999999931166, 0.5937499999999948930, 0.6093749999999957812, 0.6249999999999966693, 0.6875000000000003331, 0.7187500000000024425, 0.7343750000000034417, 0.7421875000000041078, 0.7460937500000043299, 0.7480468750000043299, 0.7500000000000043299, 0.8750000000000022204, 1.000000000000000000 ),
 .UNSPECIFIED. ) ;
#7016=CARTESIAN_POINT ( 'NONE',  ( -4.517639745569246301, 118.1171028094802011, 0.5418958579287725952 ) ) ;
#7020=CARTESIAN_POINT ( 'NONE',  ( -3.773169269958028149, 118.9364908861665242, -0.9318311032467860855 ) ) ;
#7021=CARTESIAN_POINT ( 'NONE',  ( -7.449435858333571581, 123.6645382909113664, -0.1834419053087674445 ) ) ;
#7022=CARTESIAN_POINT ( 'NONE',  ( 4.564985497539753467, 118.0819797128260404, 0.7245633110350869766 ) ) ;
#7023=CARTESIAN_POINT ( 'NONE',  ( -15.73537819279964900, 147.9505201145231865, -1.277015258756127647 ) ) ;
#7025=CARTESIAN_POINT ( 'NONE',  ( -1.784412496506031065, 115.7029491485453434, -1.723391489024520107 ) ) ;
#7027=CARTESIAN_POINT ( 'NONE',  ( 5.416379098809391834, 117.1811293437636721, -0.6832607176795200132 ) ) ;
#7028=CARTESIAN_POINT ( 'NONE',  ( -9.541807374902315786, 122.7780075402122151, -1.248600054375463397 ) ) ;
#7029=CARTESIAN_POINT ( 'NONE',  ( -5.332935397695336199, 116.0444662015457311, -0.1065647409268299234 ) ) ;
#7030=CARTESIAN_POINT ( 'NONE',  ( -0.02768739821015298377, 156.9833357668885014, 1.385590625008459087 ) ) ;
#7032=CARTESIAN_POINT ( 'NONE',  ( -15.64366209671519670, 147.2213131111883513, -0.2456931987577644916 ) ) ;
#7033=CARTESIAN_POINT ( 'NONE',  ( -0.5842699607273857954, -4.454521554441356557, 4.585487691134133570 ) ) ;
#7034=CARTESIAN_POINT ( 'NONE',  ( 22.53452490051026658, 150.3096427868838987, 1.298398843693310267 ) ) ;
#7036=CARTESIAN_POINT ( 'NONE',  ( 3.228916932056940858, -14.69740968606676823, 0.4668019137946345376 ) ) ;
#7037=CARTESIAN_POINT ( 'NONE',  ( -19.00246547725227231, 147.5601278813269914, 1.724645192979526565 ) ) ;
#7038=CARTESIAN_POINT ( 'NONE',  ( -0.2870776928289196506, 5.753151106566044781, -0.9307745581249481370 ) ) ;
#7039=CARTESIAN_POINT ( 'NONE',  ( -15.27623507474957876, 120.8527393138689376, -0.8201955439070724996 ) ) ;
#7041=CARTESIAN_POINT ( 'NONE',  ( 0.1071387893147941056, 24.31912984647217968, -0.9680276682219529638 ) ) ;
#7044=CARTESIAN_POINT ( 'NONE',  ( 5.237871118309306517, 118.7524313932052991, 0.6368175916084592991 ) ) ;
#7046=CARTESIAN_POINT ( 'NONE',  ( -10.78632646169022280, 153.0872561326487187, 0.6669751843662028445 ) ) ;
#7047=CARTESIAN_POINT ( 'NONE',  ( 3.889980283446199838, -12.05568003970028457, 1.127423567058935205 ) ) ;
#7048=CARTESIAN_POINT ( 'NONE',  ( 11.13866856781917392, 123.6647009725989648, -1.091370626813936706 ) ) ;
#7049=CARTESIAN_POINT ( 'NONE',  ( -19.49537437117590599, 147.7952244890416296, -2.518105945687704406 ) ) ;
#7050=CARTESIAN_POINT ( 'NONE',  ( 3.486869749213982406, 104.6144662015456959, 3.351517259169598528 ) ) ;
#7051=CARTESIAN_POINT ( 'NONE',  ( 3.116451998213339625, -14.00698646007624149, 1.619014592372306716 ) ) ;
#7052=CARTESIAN_POINT ( 'NONE',  ( -5.656553017150170781, 31.30584249932583774, -0.4062832063744321043 ) ) ;
#7053=CARTESIAN_POINT ( 'NONE',  ( 5.292481242635903804, 121.3432423864224177, 0.03610140192510987583 ) ) ;
#7054=ORIENTED_EDGE ( 'NONE', *, *, #5258, .F. ) ;
#7055=CARTESIAN_POINT ( 'NONE',  ( -2.507392566506281728, 107.3035951680821967, 4.608238627831032552 ) ) ;
#7056=DIRECTION ( 'NONE',  ( -0.9998004120163610509, -4.016384292689131511E-17, -0.01997839162482749689 ) ) ;
#7059=DIRECTION ( 'NONE',  ( -4.017660918040594346E-17, 1.000000000000000000, 2.376309959284834438E-19 ) ) ;
#7061=CARTESIAN_POINT ( 'NONE',  ( 1.829002187088338838, 116.5125207362610951, -0.06620492630546132018 ) ) ;
#7062=CARTESIAN_POINT ( 'NONE',  ( -7.639359131133931946, 124.2918010433613745, -0.1437932647211236370 ) ) ;
#7064=CARTESIAN_POINT ( 'NONE',  ( -0.4392745730724126330, 115.6909491485452435, 1.750092874769185070 ) ) ;
#7066=CARTESIAN_POINT ( 'NONE',  ( -3.884074962540208897, 32.38989619462120828, 0.9675453285884029198 ) ) ;
#7067=CARTESIAN_POINT ( 'NONE',  ( 6.788760123629391074, 157.9234729166680040, 1.828055096104673760 ) ) ;
#7068=CARTESIAN_POINT ( 'NONE',  ( 4.466176584706416541, 22.48015689762229030, 1.290832665783417488 ) ) ;
#7069=CARTESIAN_POINT ( 'NONE',  ( 7.942258639034435852, 16.71227948022357523, 2.857158061122382353 ) ) ;
#7070=CARTESIAN_POINT ( 'NONE',  ( 8.664868210595660258, 118.4192301925127566, -0.7007756955166910551 ) ) ;
#7071=CARTESIAN_POINT ( 'NONE',  ( 0.1065646865915094443, 105.8844662015457203, -5.332932678536313809 ) ) ;
#7075=CARTESIAN_POINT ( 'NONE',  ( 1.151590580803910635, 105.1234912291904209, 5.218814051747787452 ) ) ;
#7076=CARTESIAN_POINT ( 'NONE',  ( -2.359559261509405204, 14.11188314818778267, 3.974389579228013503 ) ) ;
#7079=CARTESIAN_POINT ( 'NONE',  ( 3.387566103704702236, -13.77904243453481570, 2.987699908524332759 ) ) ;
#7080=CARTESIAN_POINT ( 'NONE',  ( 1.795323270064338006, 111.6436615656963909, -3.008962535700986152 ) ) ;
#7081=CARTESIAN_POINT ( 'NONE',  ( -10.53014098995834225, 157.9057380314836223, 0.5653498989572930400 ) ) ;
#7083=CARTESIAN_POINT ( 'NONE',  ( 4.999405081406732343, 117.4046814563082819, -0.8308242854346027384 ) ) ;
#7084=VERTEX_POINT ( 'NONE', #16398 ) ;
#7087=CARTESIAN_POINT ( 'NONE',  ( -2.317791448294674428, 31.60761946039689718, 1.124105164688197211 ) ) ;
#7089=CARTESIAN_POINT ( 'NONE',  ( 3.016856305723133236, -15.72087675955979869, 4.784217253217923016 ) ) ;
#7090=CARTESIAN_POINT ( 'NONE',  ( -17.73303733098149593, 151.6044147853587845, 1.711203799303050888 ) ) ;
#7091=CARTESIAN_POINT ( 'NONE',  ( 21.57210427006330278, 149.5883454796168621, -1.274511887596344817 ) ) ;
#7092=CARTESIAN_POINT ( 'NONE',  ( 4.560281875334545099, -11.68902278883368595, 0.6958564903332965512 ) ) ;
#7097=CARTESIAN_POINT ( 'NONE',  ( 0.1328480158795370403, 107.4969721965504021, 4.685401909699153045 ) ) ;
#7098=CARTESIAN_POINT ( 'NONE',  ( -5.070296302330613791, 156.2174774745075183, 1.306674740328298334 ) ) ;
#7099=DIRECTION ( 'NONE',  ( 0.9998004120163608288, 0.000000000000000000, 0.01997839162482736852 ) ) ;
#7100=CARTESIAN_POINT ( 'NONE',  ( 11.76378629788668384, 123.2143981803894093, -1.250304744737055218 ) ) ;
#7101=CARTESIAN_POINT ( 'NONE',  ( -20.68324476251077115, 149.5879773183856685, -2.343194491808722191 ) ) ;
#7105=CARTESIAN_POINT ( 'NONE',  ( 4.413039900744538890, 118.1641392279842364, -0.4832662010003311859 ) ) ;
#7107=CARTESIAN_POINT ( 'NONE',  ( 8.835859712557383006, 123.2701452714374568, -0.3110363621490745967 ) ) ;
#7109=CARTESIAN_POINT ( 'NONE',  ( 3.118150858982619233, -14.63350761981947734, -0.02509704758125085033 ) ) ;
#7110=CIRCLE ( 'NONE', #28160, 5.588000000000006295 ) ;
#7113=CARTESIAN_POINT ( 'NONE',  ( 4.585212383536918956, 13.09695617864405470, 0.6580430208065696229 ) ) ;
#7114=CARTESIAN_POINT ( 'NONE',  ( 3.428210029137735759, 119.9243055703230851, 0.7605957222121786376 ) ) ;
#7115=EDGE_CURVE ( 'NONE', #20737, #35057, #7110, .T. ) ;
#7116=CARTESIAN_POINT ( 'NONE',  ( -2.443897349042808642, 30.72383818298906988, 1.256468113927755148 ) ) ;
#7118=CARTESIAN_POINT ( 'NONE',  ( -1.178223178616622402, 14.53665720681882689, 4.476207649055042204 ) ) ;
#7119=CARTESIAN_POINT ( 'NONE',  ( 8.876935545690592733, 123.7004864364556909, 0.3337242414277969971 ) ) ;
#7120=DIRECTION ( 'NONE',  ( -0.5064479475276348897, 0.8622111466057285067, -0.01012003527073121814 ) ) ;
#7122=EDGE_CURVE ( 'NONE', #38903, #30579, #11799, .T. ) ;
#7124=CARTESIAN_POINT ( 'NONE',  ( 5.552440004966861409, 116.7968546181220120, -0.2240355716773803907 ) ) ;
#7125=DIRECTION ( 'NONE',  ( -0.9998004120163608288, 0.000000000000000000, -0.01997839162482747608 ) ) ;
#7133=CARTESIAN_POINT ( 'NONE',  ( -16.92419414914125753, 122.6916909566506320, 0.1062714098145889491 ) ) ;
#7136=CARTESIAN_POINT ( 'NONE',  ( -6.974621529130486053, 121.9482818037246972, -0.2056693399646919718 ) ) ;
#7139=CARTESIAN_POINT ( 'NONE',  ( -1.569753016146457014, 156.2570369995211479, -0.1094014671735938637 ) ) ;
#7140=CARTESIAN_POINT ( 'NONE',  ( 6.030629465787032295, -12.69248357272054228, 1.053518048143269548 ) ) ;
#7141=CARTESIAN_POINT ( 'NONE',  ( -19.98084523315773353, 136.1824594150436383, 1.423751267309647739 ) ) ;
#7142=CARTESIAN_POINT ( 'NONE',  ( 2.739727753987758252, 28.35525327666260864, -3.728201022356329553 ) ) ;
#7143=CARTESIAN_POINT ( 'NONE',  ( 9.754222058523195571, 118.0373187826741486, 0.4689489433136689311 ) ) ;
#7144=CARTESIAN_POINT ( 'NONE',  ( 1.999148240431267487, -15.70856037145330930, 5.662001806903932177 ) ) ;
#7145=CARTESIAN_POINT ( 'NONE',  ( -2.768688662514669385, 30.30441277318858795, -3.700580903672975541 ) ) ;
#7146=CARTESIAN_POINT ( 'NONE',  ( -0.9222101193809760789, -5.324732007522724686, 0.3213417913276819249 ) ) ;
#7147=CARTESIAN_POINT ( 'NONE',  ( -15.38042280020276387, 120.6961994932685798, -0.5371754898667547851 ) ) ;
#7148=FACE_OUTER_BOUND ( 'NONE', #16218, .T. ) ;
#7149=CYLINDRICAL_SURFACE ( 'NONE', #30908, 3.175000000000001155 ) ;
#7150=CARTESIAN_POINT ( 'NONE',  ( 8.764204663043864585, 117.8121725143452778, 0.5577289095695550092 ) ) ;
#7151=ORIENTED_EDGE ( 'NONE', *, *, #26356, .T. ) ;
#7152=CARTESIAN_POINT ( 'NONE',  ( -12.49185498700849806, 153.6617311634574037, 1.629683330142263520 ) ) ;
#7154=CARTESIAN_POINT ( 'NONE',  ( 13.51395941584908478, 155.6725583577350278, 2.021746995258101975 ) ) ;
#7155=CARTESIAN_POINT ( 'NONE',  ( 19.86924145434953815, 147.9128418260961837, -1.725515945229960213 ) ) ;
#7156=CARTESIAN_POINT ( 'NONE',  ( 0.9053751552131774627, -6.120233167431497812, -0.3594991891349857416 ) ) ;
#7157=CARTESIAN_POINT ( 'NONE',  ( -21.19565729220489203, 150.1117090729339623, -2.124842235463313855 ) ) ;
#7158=CARTESIAN_POINT ( 'NONE',  ( 4.566904246663979983, 118.0741002040653171, -0.6113164951592977570 ) ) ;
#7159=CARTESIAN_POINT ( 'NONE',  ( 4.973583767373020770, 117.3966162183443203, 0.9753880922370259388 ) ) ;
#7160=CARTESIAN_POINT ( 'NONE',  ( 14.10444703556369817, 134.4521314832425389, -0.9547003412267361933 ) ) ;
#7161=CARTESIAN_POINT ( 'NONE',  ( -2.836071964827412639, 121.0300505300837415, -0.05667146733340970577 ) ) ;
#7163=CARTESIAN_POINT ( 'NONE',  ( -16.73131056987035237, 135.2943057719725459, -2.348795921478700421 ) ) ;
#7164=CARTESIAN_POINT ( 'NONE',  ( 1.975136073220363553, -15.70315947173593685, 5.621751108460156132 ) ) ;
#7167=CARTESIAN_POINT ( 'NONE',  ( -4.636526327029984351, 118.0184740840416282, -0.8096187216592474201 ) ) ;
#7169=EDGE_CURVE ( 'NONE', #20726, #27974, #26519, .T. ) ;
#7170=CARTESIAN_POINT ( 'NONE',  ( 4.105025596253708997, 118.2429491485453354, 0.3532957070722724802 ) ) ;
#7171=CARTESIAN_POINT ( 'NONE',  ( 18.14277298170000563, 148.2327041560005512, 2.387153687107330668 ) ) ;
#7173=EDGE_CURVE ( 'NONE', #37741, #35331, #11829, .T. ) ;
#7174=CARTESIAN_POINT ( 'NONE',  ( 23.29144772315967771, 149.3526176766912101, 0.4654185560736371352 ) ) ;
#7175=CARTESIAN_POINT ( 'NONE',  ( -0.5381045032992836097, 19.73597684265961050, -8.428375251626778919 ) ) ;
#7176=CARTESIAN_POINT ( 'NONE',  ( 3.646880827531659985, 120.8687762150871379, 0.3676761613455565847 ) ) ;
#7177=CARTESIAN_POINT ( 'NONE',  ( 22.55548643167949052, 142.2972183020237367, -0.7396483830486684230 ) ) ;
#7180=B_SPLINE_CURVE_WITH_KNOTS ( 'NONE', 3,
 ( #29530, #26323, #368, #35931, #25491, #12498 ),
 .UNSPECIFIED., .F., .F.,
 ( 4, 2, 4 ),
 ( 0.000000000000000000, 0.5000000000000000000, 1.000000000000000000 ),
 .UNSPECIFIED. ) ;
#7181=ORIENTED_EDGE ( 'NONE', *, *, #29229, .T. ) ;
#7184=CARTESIAN_POINT ( 'NONE',  ( -20.69815783549640642, 152.5608647341385335, -0.3383848979192931039 ) ) ;
#7186=CARTESIAN_POINT ( 'NONE',  ( 8.076851222567801969, 121.3085770623402624, -0.9248642372525653910 ) ) ;
#7188=CARTESIAN_POINT ( 'NONE',  ( -11.90976107009722362, 151.9662372315928280, -0.6611612027286482007 ) ) ;
#7189=CARTESIAN_POINT ( 'NONE',  ( 4.284293204009990141, -11.98693494109343050, 1.176118521537933725 ) ) ;
#7191=CARTESIAN_POINT ( 'NONE',  ( -21.81261666999477100, 141.9756885651356413, 1.158660305423542924 ) ) ;
#7192=DIRECTION ( 'NONE',  ( 0.9998004120163608288, 0.000000000000000000, 0.01997839162482749342 ) ) ;
#7193=CARTESIAN_POINT ( 'NONE',  ( -0.0008202526018423079166, 159.6052337359418800, 0.04104879434819973250 ) ) ;
#7195=CARTESIAN_POINT ( 'NONE',  ( 0.05711764529616595448, 0.5181683540770932739, -4.631227783250111862 ) ) ;
#7196=CARTESIAN_POINT ( 'NONE',  ( 2.745104810890289126, 105.1243892088056100, 4.583589704686842126 ) ) ;
#7198=CARTESIAN_POINT ( 'NONE',  ( -6.484670282503085616E-14, 71.97546620154574271, 3.533028205012241021E-29 ) ) ;
#7199=CARTESIAN_POINT ( 'NONE',  ( -8.289732393230972107, 120.2889636526078903, 1.114899670313132862 ) ) ;
#7200=CARTESIAN_POINT ( 'NONE',  ( -4.598078022480850180, -10.86695742004451404, -0.5832510952623800593 ) ) ;
#7201=CARTESIAN_POINT ( 'NONE',  ( 15.04114430247500245, 121.6710330000183546, 1.338242383117114853 ) ) ;
#7204=CARTESIAN_POINT ( 'NONE',  ( 4.077592138694859258, 118.2594131075661608, -0.7845094026950484301 ) ) ;
#7205=CARTESIAN_POINT ( 'NONE',  ( -3.538659794179211726, -11.74154716455626257, -2.972011832598964176 ) ) ;
#7206=CARTESIAN_POINT ( 'NONE',  ( -7.741078003750668124, 158.6130819278358501, -0.9685178112996217781 ) ) ;
#7208=CARTESIAN_POINT ( 'NONE',  ( -6.107944937931588214, 155.3491548655973133, 0.3423801154807231684 ) ) ;
#7209=CARTESIAN_POINT ( 'NONE',  ( 2.853125897180512460, -15.37704012655945185, 5.752692477956393269 ) ) ;
#7214=CARTESIAN_POINT ( 'NONE',  ( 18.97962326299249014, 149.2349160008635351, 2.496544457321506094 ) ) ;
#7217=CARTESIAN_POINT ( 'NONE',  ( -19.19817178191696172, 128.6826163344482268, 0.7403421610261617936 ) ) ;
#7218=CARTESIAN_POINT ( 'NONE',  ( -7.074087999897446188, 26.91573472731666783, -4.615267515785972385 ) ) ;
#7219=CARTESIAN_POINT ( 'NONE',  ( 15.17477609654683590, 139.4722935914273307, 1.590378199732649822 ) ) ;
#7220=CARTESIAN_POINT ( 'NONE',  ( 14.60357043488709650, 120.3300541288867862, -0.1192926189779471569 ) ) ;
#7224=CARTESIAN_POINT ( 'NONE',  ( 3.372434712493016296, 108.0380779545110812, -4.123874089241533980 ) ) ;
#7225=ADVANCED_FACE ( 'NONE', ( #35541 ), #5076, .T. ) ;
#7228=CARTESIAN_POINT ( 'NONE',  ( -4.486143021922693208, 118.1136361874718688, 0.5725959421912928393 ) ) ;
#7230=ORIENTED_EDGE ( 'NONE', *, *, #17045, .F. ) ;
#7232=CARTESIAN_POINT ( 'NONE',  ( 3.927402275990105718, 119.0434425390719326, -0.7708394141866733440 ) ) ;
#7233=CARTESIAN_POINT ( 'NONE',  ( -0.6688473404179187121, 105.9455060897651748, -5.311925200740537534 ) ) ;
#7234=CARTESIAN_POINT ( 'NONE',  ( 4.642283747215392609, 118.0244654425472959, 0.7555977772639859147 ) ) ;
#7235=CARTESIAN_POINT ( 'NONE',  ( -16.27374876192092401, 146.7930872653447523, -1.439762483169732432 ) ) ;
#7236=CARTESIAN_POINT ( 'NONE',  ( -0.6864567890905972636, 115.7029491485453718, -1.757685328908172195 ) ) ;
#7237=CARTESIAN_POINT ( 'NONE',  ( 2.010775290776205981, 117.9496054473550402, -1.283640624249119622 ) ) ;
#7238=CARTESIAN_POINT ( 'NONE',  ( 5.239928853181306856, 115.4398124677065596, -1.307349544149847720 ) ) ;
#7239=CARTESIAN_POINT ( 'NONE',  ( -0.5523667267585495866, 120.0661220204379305, -0.4484973920728141938 ) ) ;
#7240=CARTESIAN_POINT ( 'NONE',  ( -0.1506890447697080415, 104.6144662015457527, 6.108955356427616223 ) ) ;
#7243=CARTESIAN_POINT ( 'NONE',  ( 7.895606690698700802, 122.1535174891448321, -0.5249436039529056242 ) ) ;
#7244=CARTESIAN_POINT ( 'NONE',  ( -10.91351724380642096, 127.9361551302125832, -0.05936199999560100304 ) ) ;
#7245=DIRECTION ( 'NONE',  ( 0.9998004120163610509, 4.016384292689131511E-17, 0.01997839162482749689 ) ) ;
#7246=CARTESIAN_POINT ( 'NONE',  ( 16.55455218413301210, 122.7279807066903032, 1.056987703419675961 ) ) ;
#7247=CARTESIAN_POINT ( 'NONE',  ( 5.284239755522298410, 105.1224178746987121, -0.8069738050709613919 ) ) ;
#7248=CARTESIAN_POINT ( 'NONE',  ( 3.238076882636043763, -14.77659300283332122, 2.967476587227507956 ) ) ;
#7249=CARTESIAN_POINT ( 'NONE',  ( -10.78346871132534979, 121.7859837122882283, 1.235232998807844096 ) ) ;
#7250=CARTESIAN_POINT ( 'NONE',  ( -0.8533247626149625953, -2.668348290978065140, -0.4694259674561338525 ) ) ;
#7251=CARTESIAN_POINT ( 'NONE',  ( -9.693497654998228796, 118.1218853900603136, -0.6301662642801911796 ) ) ;
#7252=CARTESIAN_POINT ( 'NONE',  ( -0.9742996550080020857, -5.754034560434002188, 0.05241923913101136784 ) ) ;
#7255=CARTESIAN_POINT ( 'NONE',  ( 5.090087584496979289, 118.2545999410811106, 0.7183934583778605054 ) ) ;
#7256=CARTESIAN_POINT ( 'NONE',  ( -8.258026456251933212, 154.6505398758502849, 0.7900859392159014227 ) ) ;
#7257=CARTESIAN_POINT ( 'NONE',  ( 4.342152980699533593, -13.79257992285246104, 4.116713196511041950 ) ) ;
#7258=CARTESIAN_POINT ( 'NONE',  ( 6.588241325444229801, 120.6599796251122427, -0.8186057014055779790 ) ) ;
#7259=CARTESIAN_POINT ( 'NONE',  ( -1.258058525836236230, 118.8689652838214244, -0.6902481975293248695 ) ) ;
#7260=CARTESIAN_POINT ( 'NONE',  ( -0.8468149500740962399, 104.6144662015457243, 4.761320282458491704 ) ) ;
#7261=CARTESIAN_POINT ( 'NONE',  ( 3.221735024265227398, -14.36526069886394730, 2.718910799868354378 ) ) ;
#7262=CARTESIAN_POINT ( 'NONE',  ( -4.771056762337200219, 117.4047813638584188, -1.203986021773440385 ) ) ;
#7263=CARTESIAN_POINT ( 'NONE',  ( 10.33307603652738038, 126.0505730134521230, 0.02860894079130328269 ) ) ;
#7265=CARTESIAN_POINT ( 'NONE',  ( -3.324521368350398909, 108.2676741415845640, 4.163358009128126369 ) ) ;
#7266=CARTESIAN_POINT ( 'NONE',  ( 2.372169177973964871, 106.9236017804880134, 4.772346225205962966 ) ) ;
#7267=DIRECTION ( 'NONE',  ( 0.9998004120163609398, 0.000000000000000000, 0.01997839162482749689 ) ) ;
#7270=CARTESIAN_POINT ( 'NONE',  ( 6.904872195170157489, 117.1762911274595496, 0.05199240921585736308 ) ) ;
#7271=CARTESIAN_POINT ( 'NONE',  ( -5.239928853181434754, 115.4398124677065596, 1.307349544149847942 ) ) ;
#7272=CARTESIAN_POINT ( 'NONE',  ( 1.847049442607983316, -15.63718699515584376, 5.492472997249506328 ) ) ;
#7274=CARTESIAN_POINT ( 'NONE',  ( -3.137464277621155873, 31.48680077624217688, 0.6829839861511678434 ) ) ;
#7275=CARTESIAN_POINT ( 'NONE',  ( 12.61233984701546440, 121.4495935343099688, 1.683034450629873779 ) ) ;
#7276=CARTESIAN_POINT ( 'NONE',  ( -4.556403025205056245, 17.84477460162305107, -0.8067276567318153457 ) ) ;
#7277=CARTESIAN_POINT ( 'NONE',  ( -8.190863557275731566, 21.65400946394957060, -2.068261358883292989 ) ) ;
#7278=CARTESIAN_POINT ( 'NONE',  ( 2.507300275874562168, 117.4827359074439670, -0.6436947651051395658 ) ) ;
#7279=CARTESIAN_POINT ( 'NONE',  ( -2.311675797007805677, 124.5312663981120380, -0.07107509915817145085 ) ) ;
#7280=CARTESIAN_POINT ( 'NONE',  ( 4.880791232649782430, 117.4111470503218584, 1.144768225355988545 ) ) ;
#7282=CARTESIAN_POINT ( 'NONE',  ( -0.008700780990417026142, 121.2597428844645293, 0.4354226598342535448 ) ) ;
#7284=CARTESIAN_POINT ( 'NONE',  ( 3.263621351691376571, 8.939281053574255509, -3.290156819607050753 ) ) ;
#7286=CARTESIAN_POINT ( 'NONE',  ( 2.120958618816386920, -15.04726689571640819, 5.287964242625700528 ) ) ;
#7287=CARTESIAN_POINT ( 'NONE',  ( 0.5697667371461264674, 106.2969274751293938, -5.150121607182108541 ) ) ;
#7288=CARTESIAN_POINT ( 'NONE',  ( -15.21238092238761297, 121.1469641333237917, 0.4626880538419669842 ) ) ;
#7293=CARTESIAN_POINT ( 'NONE',  ( -5.266611731650901795, 115.7029491485453434, 0.8691344147197622716 ) ) ;
#7294=CARTESIAN_POINT ( 'NONE',  ( 2.197863461560763287, -15.74995721546218519, 5.600911867769769792 ) ) ;
#7295=CARTESIAN_POINT ( 'NONE',  ( -19.99643065938096598, 145.3736917597469471, 1.717600817134501856 ) ) ;
#7296=CARTESIAN_POINT ( 'NONE',  ( 20.26345141861404642, 136.2683111393718320, -1.346723181737012442 ) ) ;
#7297=CARTESIAN_POINT ( 'NONE',  ( 0.9303216910925710126, 27.28174836166085981, 0.2932329443217298603 ) ) ;
#7302=CARTESIAN_POINT ( 'NONE',  ( 0.2537530607703858410, 113.0327356262573915, 2.627782494400416002 ) ) ;
#7304=CARTESIAN_POINT ( 'NONE',  ( -16.73823235880720617, 147.9788754379930822, 1.246688593732825812 ) ) ;
#7305=CARTESIAN_POINT ( 'NONE',  ( 0.7543369490868296889, 118.1473330535139041, 0.9261446413320308935 ) ) ;
#7306=CARTESIAN_POINT ( 'NONE',  ( 17.49586834669421620, 149.8167423968465073, -1.704004628023328083 ) ) ;
#7307=CARTESIAN_POINT ( 'NONE',  ( -20.51324802173768802, 148.8605967840894095, -2.436527653975322227 ) ) ;
#7309=CARTESIAN_POINT ( 'NONE',  ( 4.284053485260008287, 118.2131419831110577, -0.3606587761694292071 ) ) ;
#7310=CARTESIAN_POINT ( 'NONE',  ( 3.061305989504062630, 156.1243923452879017, -0.5262318146843658617 ) ) ;
#7312=CARTESIAN_POINT ( 'NONE',  ( 2.944601773672358203, -15.01875103642165499, 4.065120351795452613 ) ) ;
#7313=CARTESIAN_POINT ( 'NONE',  ( 5.223521521431373493, 105.1221584262004143, -1.132698478535189901 ) ) ;
#7314=CIRCLE ( 'NONE', #6611, 5.080000000000006288 ) ;
#7316=CARTESIAN_POINT ( 'NONE',  ( -2.168033660621066172, 0.5777166996233511487, 4.103230905123370853 ) ) ;
#7317=CARTESIAN_POINT ( 'NONE',  ( 14.96631152213282689, 150.5987129668814077, 1.974168424754894957 ) ) ;
#7318=CARTESIAN_POINT ( 'NONE',  ( -1.750334050913927353, 31.14778888712128690, 2.093020893977926900 ) ) ;
#7319=EDGE_CURVE ( 'NONE', #1073, #6137, #14271, .T. ) ;
#7320=CARTESIAN_POINT ( 'NONE',  ( -2.136650056307613621, 10.86338872207680950, -4.114640003288728920 ) ) ;
#7321=CARTESIAN_POINT ( 'NONE',  ( 7.577119205441340988, 122.4179301937671767, 0.2905534069474317582 ) ) ;
#7322=CARTESIAN_POINT ( 'NONE',  ( -4.755271767586297216, 111.7583057171730729, 2.489475493475922452 ) ) ;
#7325=CARTESIAN_POINT ( 'NONE',  ( -8.790230331137980357, 117.7071499903595821, -0.3330531770478057929 ) ) ;
#7330=CARTESIAN_POINT ( 'NONE',  ( 2.958531772299235918, 50.13146620154573441, 1.329372033065076453 ) ) ;
#7334=CARTESIAN_POINT ( 'NONE',  ( 0.08519874065564590759, 108.5751225745497948, -4.263693374914214296 ) ) ;
#7335=CARTESIAN_POINT ( 'NONE',  ( -15.11282490002057877, 156.1437908837410191, 0.09152821140687306123 ) ) ;
#7336=ORIENTED_EDGE ( 'NONE', *, *, #17814, .T. ) ;
#7338=CARTESIAN_POINT ( 'NONE',  ( 6.980895880038317181, 121.9518852483956124, 0.06772288494938194514 ) ) ;
#7341=CARTESIAN_POINT ( 'NONE',  ( -0.6411011158480280914, 120.9975462804897433, -0.03814546805551050079 ) ) ;
#7342=CARTESIAN_POINT ( 'NONE',  ( 3.842082824490853810, -15.33115451161810938, 5.194229279690915746 ) ) ;
#7343=CARTESIAN_POINT ( 'NONE',  ( -10.59408866556495532, 119.9085704333771787, 1.028430606607102948 ) ) ;
#7344=CARTESIAN_POINT ( 'NONE',  ( -2.614655561276646889, 23.60746518810343630, 3.812863311767609620 ) ) ;
#7345=CARTESIAN_POINT ( 'NONE',  ( 1.853717367163155050, 116.5907236856068181, 0.2192087907590279383 ) ) ;
#7347=CARTESIAN_POINT ( 'NONE',  ( 11.82635486671713743, 152.0554279321345064, 0.4236511662767659669 ) ) ;
#7349=CARTESIAN_POINT ( 'NONE',  ( 0.2615529312792121419, 0.9453775857588032627, -0.9394305312888860948 ) ) ;
#7350=CARTESIAN_POINT ( 'NONE',  ( -15.78464309758879835, 121.0087326939336378, -0.5477818752361016674 ) ) ;
#7353=CARTESIAN_POINT ( 'NONE',  ( -2.238353053745737231, 116.2832059125415896, 0.1037362710514463521 ) ) ;
#7354=CARTESIAN_POINT ( 'NONE',  ( -15.94706863659619778, 135.0473088626721392, 1.554726643320765378 ) ) ;
#7356=CARTESIAN_POINT ( 'NONE',  ( 1.172210521474222666, 158.9035955689636523, 1.423060353815112311 ) ) ;
#7357=CARTESIAN_POINT ( 'NONE',  ( 19.22223103763152352, 149.5120288530235655, -1.725574580128898639 ) ) ;
#7358=CARTESIAN_POINT ( 'NONE',  ( -0.8332992110815757858, -10.66407516643697306, 0.5056687530665907593 ) ) ;
#7359=CARTESIAN_POINT ( 'NONE',  ( -13.04750228320310157, 121.1598417376693533, -1.575122625318853053 ) ) ;
#7360=CARTESIAN_POINT ( 'NONE',  ( 4.532710609442922589, 118.0666091547772396, -0.6408898899164870988 ) ) ;
#7362=CARTESIAN_POINT ( 'NONE',  ( 5.032731182891235555, 105.1218460117307387, 1.777745822249493957 ) ) ;
#7364=CARTESIAN_POINT ( 'NONE',  ( 9.666892607209371491, 123.4354624054469980, -0.6853163995640744188 ) ) ;
#7365=CARTESIAN_POINT ( 'NONE',  ( 7.805882608899723962, 122.5029464779834427, 0.4967789704017860908 ) ) ;
#7366=ORIENTED_EDGE ( 'NONE', *, *, #27896, .F. ) ;
#7367=CARTESIAN_POINT ( 'NONE',  ( -3.311752042447871691, 119.2933411826354728, -0.8767012952321083796 ) ) ;
#7368=CARTESIAN_POINT ( 'NONE',  ( 4.076841989731768479, -15.73006006892005360, 3.802225825406736259 ) ) ;
#7370=CARTESIAN_POINT ( 'NONE',  ( -4.572062116902815276, 118.0791223117457207, -0.7157013623424338666 ) ) ;
#7372=CARTESIAN_POINT ( 'NONE',  ( 4.110706825855569235, 118.2429491485453497, 0.3474105799464941580 ) ) ;
#7373=CARTESIAN_POINT ( 'NONE',  ( 14.16178827078151237, 152.6618899727951089, 2.241469232429742942 ) ) ;
#7375=CARTESIAN_POINT ( 'NONE',  ( 15.96050253218456838, 121.0385544001969436, 0.3018840724360823957 ) ) ;
#7376=CARTESIAN_POINT ( 'NONE',  ( 7.419718609332475623, 16.48482641057854892, 3.982871883899435250 ) ) ;
#7377=CARTESIAN_POINT ( 'NONE',  ( 6.141611553833064896, 155.3548635187015350, 0.6951709773850852647 ) ) ;
#7378=CARTESIAN_POINT ( 'NONE',  ( 0.006942562093227406909, 117.0978366787122127, -0.3474341964894883672 ) ) ;
#7380=CARTESIAN_POINT ( 'NONE',  ( 0.6719655926374001886, 115.6909491485452719, 1.760269452045342131 ) ) ;
#7383=CARTESIAN_POINT ( 'NONE',  ( -16.85745507829919276, 155.2173118157008673, -0.2667832593600951707 ) ) ;
#7385=CARTESIAN_POINT ( 'NONE',  ( 8.106904764074545966, 121.1661902519200282, -0.9676739013972032177 ) ) ;
#7388=CARTESIAN_POINT ( 'NONE',  ( -5.901573779631426042, 121.4708175001875077, -0.3521552259516173566 ) ) ;
#7389=CARTESIAN_POINT ( 'NONE',  ( 4.362034286260056071, -13.41731938665795276, 3.520857194803681534 ) ) ;
#7390=CARTESIAN_POINT ( 'NONE',  ( -12.68208805480606394, 156.8164516032445306, 1.015108139269342624 ) ) ;
#7392=CARTESIAN_POINT ( 'NONE',  ( 22.66113959641428366, 150.6410255081855212, 0.5295512721432398262 ) ) ;
#7393=ORIENTED_EDGE ( 'NONE', *, *, #730, .F. ) ;
#7394=CARTESIAN_POINT ( 'NONE',  ( -1.825063964020108065, -4.879331645356781877, 4.256838567046823840 ) ) ;
#7395=CARTESIAN_POINT ( 'NONE',  ( -22.53492722140454774, 150.7843406352268687, -0.4757920170715050912 ) ) ;
#7398=ORIENTED_EDGE ( 'NONE', *, *, #20106, .T. ) ;
#7399=CARTESIAN_POINT ( 'NONE',  ( -6.473090125947880580, 119.6242553686945058, 1.000010245827238409 ) ) ;
#7401=( BOUNDED_SURFACE ( )  B_SPLINE_SURFACE ( 3, 2, ( 
 ( #1767, #14728, #24521 ),
 ( #25384, #28152, #21741 ),
 ( #5387, #8989, #38387 ),
 ( #41375, #37743, #41587 ) ),
 .UNSPECIFIED., .F., .F., .T. ) 
 B_SPLINE_SURFACE_WITH_KNOTS ( ( 4, 4 ),
 ( 3, 3 ),
 ( -1.135597912584696071E-06, 0.0001904019166766824050 ),
 ( 0.000000000000000000, 0.2833440467634030790 ),
 .UNSPECIFIED. ) 
 GEOMETRIC_REPRESENTATION_ITEM ( )  RATIONAL_B_SPLINE_SURFACE ( (
 ( 1.000000000000000000, 0.9321124567126647387, 0.9026959759050480203),
 ( 1.000000000000000000, 0.9321124565380634053, 0.9026959756547898728),
 ( 1.000000000000000000, 0.9321125502981708610, 0.9026961100422681294),
 ( 1.000000000000000000, 0.9321126250856475171, 0.9026962172360489811) ) ) 
 REPRESENTATION_ITEM ( '' )  SURFACE ( )  );
#7402=CARTESIAN_POINT ( 'NONE',  ( -1.722957355399680202, -2.895624787512894649, -4.295268622497145472 ) ) ;
#7403=CARTESIAN_POINT ( 'NONE',  ( 21.70861548485252968, 150.3096123636779566, 1.869307503447338537 ) ) ;
#7406=CARTESIAN_POINT ( 'NONE',  ( 20.75082247216783671, 147.7542213611591535, -1.617965925928341875 ) ) ;
#7407=CARTESIAN_POINT ( 'NONE',  ( 2.459658384930404118, -7.418532284756778949, 3.912982838641719141 ) ) ;
#7408=CARTESIAN_POINT ( 'NONE',  ( -10.42794149288038952, 157.8855781193960297, -1.079236549925195465 ) ) ;
#7409=ORIENTED_EDGE ( 'NONE', *, *, #26494, .T. ) ;
#7411=CARTESIAN_POINT ( 'NONE',  ( -7.598614292646969304, 122.4062900713904440, 0.04802449110505829788 ) ) ;
#7413=CIRCLE ( 'NONE', #6706, 0.5080000000000002292 ) ;
#7414=CARTESIAN_POINT ( 'NONE',  ( 5.253792623460133981, -14.56763799980149976, 3.797339299194151696 ) ) ;
#7415=AXIS2_PLACEMENT_3D ( 'NONE', #9823, #22789, #18771 ) ;
#7417=ADVANCED_FACE ( 'NONE', ( #26153 ), #29350, .T. ) ;
#7420=CARTESIAN_POINT ( 'NONE',  ( 8.661198069469437044, 120.2102557752085232, 1.489220423754913369 ) ) ;
#7421=CARTESIAN_POINT ( 'NONE',  ( 4.902823790339319032, 117.6536153060737320, 0.9411696025594519233 ) ) ;
#7422=CARTESIAN_POINT ( 'NONE',  ( -6.564189886853176475E-14, 81.62746620154572952, -5.847435218134868453E-18 ) ) ;
#7423=CARTESIAN_POINT ( 'NONE',  ( -22.59612908711474688, 148.7221180073953235, 0.8559155618276412802 ) ) ;
#7424=CARTESIAN_POINT ( 'NONE',  ( 5.986726992493722754, 14.59627609256335923, -5.926391003037220884 ) ) ;
#7425=CARTESIAN_POINT ( 'NONE',  ( 2.668671847104294947, 120.5579296053302727, 0.4429723278990745916 ) ) ;
#7428=CARTESIAN_POINT ( 'NONE',  ( 14.42641459765130030, 120.3907653763288579, -0.3011401359519874088 ) ) ;
#7432=CARTESIAN_POINT ( 'NONE',  ( -4.006527145856388472, 117.9394519250054998, 1.074047527556786008 ) ) ;
#7435=CARTESIAN_POINT ( 'NONE',  ( -4.371358227350733650, 118.1836130580517477, 0.4407715912306871542 ) ) ;
#7436=CARTESIAN_POINT ( 'NONE',  ( 2.633027443571791970, 107.2200259174091315, -4.631959221834722307 ) ) ;
#7437=ORIENTED_EDGE ( 'NONE', *, *, #20613, .T. ) ;
#7439=CARTESIAN_POINT ( 'NONE',  ( -3.887428295838784464, 119.0433692556534737, -0.9258068317460230734 ) ) ;
#7441=CARTESIAN_POINT ( 'NONE',  ( -2.923657115617448454, 107.8178375082508609, -4.476818208047827596 ) ) ;
#7442=CARTESIAN_POINT ( 'NONE',  ( 4.509504427301486373, 118.1210246048803754, 0.6598204393874429474 ) ) ;
#7443=CARTESIAN_POINT ( 'NONE',  ( -9.704918697729887356, 124.0009531390599591, -0.8840593909831663266 ) ) ;
#7444=CARTESIAN_POINT ( 'NONE',  ( -1.183497919878635729, 115.7029491485453292, -1.742415236764897957 ) ) ;
#7445=CARTESIAN_POINT ( 'NONE',  ( 3.928887737881764153, 118.1651004245801460, -0.5645064089330636969 ) ) ;
#7446=CARTESIAN_POINT ( 'NONE',  ( 7.500421786656795042, 123.6595150816924047, 0.1155007223820210815 ) ) ;
#7448=CARTESIAN_POINT ( 'NONE',  ( -16.42797441217054910, 147.8801373804967341, -1.766026403434533876 ) ) ;
#7449=CARTESIAN_POINT ( 'NONE',  ( -5.336420303164543633, 104.6144662015457101, 0.06783417913549341649 ) ) ;
#7452=CARTESIAN_POINT ( 'NONE',  ( -5.586884702347495235, 75.27746620154573520, -0.1116392523995361763 ) ) ;
#7453=CARTESIAN_POINT ( 'NONE',  ( -14.67956819919654343, 148.8681330163217922, -0.09511266571365764588 ) ) ;
#7455=CARTESIAN_POINT ( 'NONE',  ( 8.135778112230736880, 117.7673425867732249, 0.7050676646501273792 ) ) ;
#7457=CARTESIAN_POINT ( 'NONE',  ( 2.112177293979604187, -15.34403890755049815, 5.167321579062071457 ) ) ;
#7458=CARTESIAN_POINT ( 'NONE',  ( -1.346530140709126133, 119.3298839580929638, 0.5995503221117501891 ) ) ;
#7459=CARTESIAN_POINT ( 'NONE',  ( 0.1022289226565744474, -8.938468249466058779, 0.9708619238636220228 ) ) ;
#7460=CARTESIAN_POINT ( 'NONE',  ( -22.76704383476090143, 150.0845277111093310, -1.179919005961814094 ) ) ;
#7461=CARTESIAN_POINT ( 'NONE',  ( -0.8274880129334906131, 26.04165684986237039, -0.5117960016238547460 ) ) ;
#7462=EDGE_LOOP ( 'NONE', ( #33089, #27813, #3991, #5407, #16878 ) ) ;
#7464=CARTESIAN_POINT ( 'NONE',  ( 0.1497278248015747881, 105.8844662015457629, 5.338012126719978490 ) ) ;
#7465=CARTESIAN_POINT ( 'NONE',  ( -7.125763582822579600, 121.8059686962219672, 0.4001172506815712793 ) ) ;
#7466=CARTESIAN_POINT ( 'NONE',  ( 4.648743876849892764, -12.57259931633604388, 2.147031799546866182 ) ) ;
#7467=CARTESIAN_POINT ( 'NONE',  ( 10.78650420462566828, 154.3566586077636487, -1.536168652981084293 ) ) ;
#7468=ORIENTED_EDGE ( 'NONE', *, *, #31016, .F. ) ;
#7469=CARTESIAN_POINT ( 'NONE',  ( -12.21694169560774768, 122.3148578561100948, -1.796258641216138541 ) ) ;
#7470=CARTESIAN_POINT ( 'NONE',  ( 2.769004702249832750, 104.6144662015457811, 3.963074674433550992 ) ) ;
#7472=CARTESIAN_POINT ( 'NONE',  ( 2.672745566561993247, -14.90124427853171873, 4.600530618394071070 ) ) ;
#7474=CARTESIAN_POINT ( 'NONE',  ( 4.275377040554418251, 155.8374496918941077, -0.1508172661092591071 ) ) ;
#7477=CARTESIAN_POINT ( 'NONE',  ( -3.264132200829606312, 108.5668320698289477, 4.052510953551484718 ) ) ;
#7478=CARTESIAN_POINT ( 'NONE',  ( 4.605371197558832286, 113.9923204192811994, 2.135305188882721694 ) ) ;
#7479=VECTOR ( 'NONE', #18471, 1000.000000000000000 ) ;
#7480=CARTESIAN_POINT ( 'NONE',  ( 4.756911902486301358, 117.3993836135862949, 1.207145067066230038 ) ) ;
#7482=CARTESIAN_POINT ( 'NONE',  ( 16.00576599164899605, 121.2237126890796191, 0.08595866332889597061 ) ) ;
#7484=CARTESIAN_POINT ( 'NONE',  ( 2.001812122746663647, -15.27695281082187861, 5.988856565476218918 ) ) ;
#7486=DIRECTION ( 'NONE',  ( -4.017660918040594346E-17, 1.000000000000000000, 2.376309959284834438E-19 ) ) ;
#7487=CARTESIAN_POINT ( 'NONE',  ( 14.56794066961886358, 154.5799843816573684, 2.217559120334770650 ) ) ;
#7489=CARTESIAN_POINT ( 'NONE',  ( 7.433834689873759061, 17.99627214424885580, -4.034796628604029323 ) ) ;
#7490=CARTESIAN_POINT ( 'NONE',  ( -2.328736857929224691, 117.2194318322477642, -0.6714296531164799520 ) ) ;
#7491=CARTESIAN_POINT ( 'NONE',  ( -2.840201032364617184, 114.3344743418335128, -2.128718819835312637 ) ) ;
#7493=CARTESIAN_POINT ( 'NONE',  ( -4.576084639598200887, 113.7931665046256029, -2.209524532645662731 ) ) ;
#7495=CARTESIAN_POINT ( 'NONE',  ( 4.087030650986479330, 6.990161447142720696, 2.163025551504125232 ) ) ;
#7497=CARTESIAN_POINT ( 'NONE',  ( -4.651991910126532126, 111.7581736691619341, -2.677509894684430680 ) ) ;
#7498=CARTESIAN_POINT ( 'NONE',  ( 3.258219809910011033, -14.04213616937880005, 2.843395319141139410 ) ) ;
#7499=CARTESIAN_POINT ( 'NONE',  ( 2.174325380064840996, 109.8863472468248119, -3.630110603364346211 ) ) ;
#7500=CARTESIAN_POINT ( 'NONE',  ( -2.899870334229920132, 116.9538966677400254, 0.3598414239652115709 ) ) ;
#7501=AXIS2_PLACEMENT_3D ( 'NONE', #34300, #18286, #37900 ) ;
#7502=CARTESIAN_POINT ( 'NONE',  ( -1.381525208824001538, 34.89533589863157204, 3.514877943587163767 ) ) ;
#7505=CARTESIAN_POINT ( 'NONE',  ( -2.498980821681361153, 104.6144662015457243, -4.129459300827505785 ) ) ;
#7506=CARTESIAN_POINT ( 'NONE',  ( 5.113606203424133412, -15.47995924129362599, 1.801594979316981204 ) ) ;
#7507=CARTESIAN_POINT ( 'NONE',  ( -16.76200238010698129, 128.5636217276695561, 1.481418206722939335 ) ) ;
#7508=CARTESIAN_POINT ( 'NONE',  ( 0.8793282038724897776, 27.06027571872007442, 0.4248793764785103177 ) ) ;
#7511=CARTESIAN_POINT ( 'NONE',  ( 0.8524833535542716278, 121.9014879524050343, 0.3240522193994319067 ) ) ;
#7513=CARTESIAN_POINT ( 'NONE',  ( -16.95093959817323181, 147.3835828867039766, 1.246432153888628935 ) ) ;
#7515=CARTESIAN_POINT ( 'NONE',  ( 17.82416131750959210, 140.4837523222294351, -1.726486987461785860 ) ) ;
#7516=CARTESIAN_POINT ( 'NONE',  ( -20.53125589898989389, 145.6130255286810495, -2.451886524809591350 ) ) ;
#7518=CARTESIAN_POINT ( 'NONE',  ( 4.308178849057600956, 118.2138035341862405, -0.3345321977047149842 ) ) ;
#7519=CARTESIAN_POINT ( 'NONE',  ( 10.70072142757958922, 153.0728289088170300, -0.5595718250706015473 ) ) ;
#7521=CARTESIAN_POINT ( 'NONE',  ( 3.238076882636043763, -14.77659300283332122, 2.967476587227507956 ) ) ;
#7523=CARTESIAN_POINT ( 'NONE',  ( -4.854232772743657165, 117.4081466956269395, 0.9971777887500445914 ) ) ;
#7525=CARTESIAN_POINT ( 'NONE',  ( -1.246715508051662535, 10.49814879194060069, 4.449005273994115939 ) ) ;
#7526=CARTESIAN_POINT ( 'NONE',  ( 7.227551859934576939, 121.2980461901665308, 1.025750885112893807 ) ) ;
#7527=CARTESIAN_POINT ( 'NONE',  ( -2.647869110835376016, 30.13907626823893082, -0.2047939377594477361 ) ) ;
#7529=CARTESIAN_POINT ( 'NONE',  ( 4.636458409304901274, 17.36039413176390411, -0.09481320587925551324 ) ) ;
#7530=CARTESIAN_POINT ( 'NONE',  ( 15.26129097679449131, 148.0152273645666980, 0.3559380457717283841 ) ) ;
#7533=CARTESIAN_POINT ( 'NONE',  ( 2.173876196063857513, 116.2747682467607575, -0.1408475702141917807 ) ) ;
#7539=AXIS2_PLACEMENT_3D ( 'NONE', #29452, #31813, #19225 ) ;
#7540=CARTESIAN_POINT ( 'NONE',  ( 7.890306666665830804, -2.504341373917490898, 2.985612812370990632 ) ) ;
#7544=CARTESIAN_POINT ( 'NONE',  ( 0.001862839608491519139, 124.0591982226671490, -0.09322411149287214427 ) ) ;
#7545=CARTESIAN_POINT ( 'NONE',  ( -23.16157447928876323, 142.6111785389246336, 0.1383437888640693669 ) ) ;
#7546=ORIENTED_EDGE ( 'NONE', *, *, #10977, .T. ) ;
#7552=CARTESIAN_POINT ( 'NONE',  ( -4.590565121197838216, 121.2030596905490540, -0.1190299148670778545 ) ) ;
#7553=CARTESIAN_POINT ( 'NONE',  ( 3.435007001638270996, -15.26001923902611779, 5.499761658607620340 ) ) ;
#7554=CARTESIAN_POINT ( 'NONE',  ( -20.68240061501462534, 141.5323519391372997, 1.529040698034871859 ) ) ;
#7555=CARTESIAN_POINT ( 'NONE',  ( 0.2838385327444274964, 29.22985346960623332, -4.617364983570896086 ) ) ;
#7556=CARTESIAN_POINT ( 'NONE',  ( 18.54318072098650561, 125.2038358216989735, 0.7288164436403702373 ) ) ;
#7557=CARTESIAN_POINT ( 'NONE',  ( 4.192904522445743964, 155.8780965706680774, 0.2271539898920573453 ) ) ;
#7559=CARTESIAN_POINT ( 'NONE',  ( -0.8651787172165069650, -5.103258934911358402, 0.4504873164067982327 ) ) ;
#7560=CARTESIAN_POINT ( 'NONE',  ( -5.727173706516765606, 159.1225378944267845, -0.2665985390141680789 ) ) ;
#7562=CARTESIAN_POINT ( 'NONE',  ( 4.756911902506432810, 117.3993836136063607, 1.207145067191207621 ) ) ;
#7563=CARTESIAN_POINT ( 'NONE',  ( -8.753730273135673201, 117.9543236253998799, 0.3768632908176075547 ) ) ;
#7564=CARTESIAN_POINT ( 'NONE',  ( -10.93624696698920751, 154.4230204216147513, 1.584134132468239420 ) ) ;
#7566=CARTESIAN_POINT ( 'NONE',  ( 0.4013927055962251411, 117.8786474493541050, 0.5472391114537521473 ) ) ;
#7567=CARTESIAN_POINT ( 'NONE',  ( 12.41883037655676247, 155.1253022143813496, -1.737092194502518394 ) ) ;
#7568=CARTESIAN_POINT ( 'NONE',  ( -0.001188813386588473625, -13.89074316258246000, -0.9734844304884215926 ) ) ;
#7569=CARTESIAN_POINT ( 'NONE',  ( -17.95761459997887144, 128.5942011134444272, -1.926528613670785095 ) ) ;
#7571=CARTESIAN_POINT ( 'NONE',  ( 4.808131379913066716, 104.6144662015456959, -0.4149153342096277841 ) ) ;
#7572=CARTESIAN_POINT ( 'NONE',  ( 16.36402192804832012, 147.4903123243063590, -0.9458667783343724933 ) ) ;
#7573=CARTESIAN_POINT ( 'NONE',  ( 7.844435714580729524, 122.2806349566659065, 0.7396647843393954203 ) ) ;
#7575=CARTESIAN_POINT ( 'NONE',  ( -3.364155546990544199, 119.5845705363850442, -0.8331338896180614517 ) ) ;
#7576=CARTESIAN_POINT ( 'NONE',  ( 4.918985584458519966, -15.36470173770705649, 0.08744857223284302483 ) ) ;
#7577=DIRECTION ( 'NONE',  ( -0.01997839162482737546, -1.040247600000940825E-18, 0.9998004120163610509 ) ) ;
#7578=CARTESIAN_POINT ( 'NONE',  ( -4.395042894517541043, 118.1799360432506347, -0.5693510968962494090 ) ) ;
#7582=CARTESIAN_POINT ( 'NONE',  ( 11.26837603645361341, 123.0403929720162495, 1.648478483780370540 ) ) ;
#7583=CARTESIAN_POINT ( 'NONE',  ( 3.019425909971710009, 50.13146620154573441, -1.718019622760792009 ) ) ;
#7584=CARTESIAN_POINT ( 'NONE',  ( 1.421603664355671315, 159.6054662015457666, 0.02840702444251847966 ) ) ;
#7585=CARTESIAN_POINT ( 'NONE',  ( 8.101632580580826470, 8.064395906452419993, -2.298819013970823999 ) ) ;
#7586=CARTESIAN_POINT ( 'NONE',  ( 15.91353055065138022, 146.3070982487133165, 0.9133378546330941372 ) ) ;
#7587=CARTESIAN_POINT ( 'NONE',  ( 4.866704567515524715, 117.3073154462328063, -0.4935321157908418299 ) ) ;
#7588=LINE ( 'NONE', #39552, #26048 ) ;
#7591=CARTESIAN_POINT ( 'NONE',  ( -0.001319893060213154059, 116.4580521601689185, 0.06605284600166372311 ) ) ;
#7594=CARTESIAN_POINT ( 'NONE',  ( 5.425175176548000522, 120.5927626492978249, -0.5604424002130801163 ) ) ;
#7596=ORIENTED_EDGE ( 'NONE', *, *, #24853, .F. ) ;
#7597=DIRECTION ( 'NONE',  ( 0.9998004120163608288, 5.205824365704081956E-17, 0.01997839162482748995 ) ) ;
#7598=CARTESIAN_POINT ( 'NONE',  ( -3.687801383043832981, 120.9852966486377710, -0.2688355818071223591 ) ) ;
#7599=CARTESIAN_POINT ( 'NONE',  ( 3.797208283716756227, -14.50848223276941873, 5.080264250175951624 ) ) ;
#7601=CARTESIAN_POINT ( 'NONE',  ( -21.93433297169883289, 150.0588410196355937, 0.9994452811612329901 ) ) ;
#7602=CARTESIAN_POINT ( 'NONE',  ( 5.078986093043054595, 69.43546620154572224, 0.1014902294541237815 ) ) ;
#7604=CARTESIAN_POINT ( 'NONE',  ( 15.93236088550697716, 121.0320206851898206, 0.3693416020086465190 ) ) ;
#7606=CARTESIAN_POINT ( 'NONE',  ( 4.560281875334545099, -11.68902278883368595, 0.6958564903332965512 ) ) ;
#7607=B_SPLINE_CURVE_WITH_KNOTS ( 'NONE', 3,
 ( #16647, #39034, #10260, #36268, #703, #26665, #6661, #33281, #7087, #20050, #13674, #13035, #4110, #26026, #22602, #30073, #38823 ),
 .UNSPECIFIED., .F., .F.,
 ( 4, 1, 1, 1, 1, 1, 1, 1, 1, 1, 1, 1, 1, 1, 4 ),
 ( 0.000000000000000000, 0.08300113939718137268, 0.1732806554784933895, 0.2717672377176819087, 0.3752096606209606167, 0.4787223716043260135, 0.5772295444745598747, 0.6668133826162351285, 0.7470991451079272982, 0.7815930070524458317, 0.8169452614683294644, 0.8547689062991584708, 0.8968063284581728745, 0.9447228702782888288, 1.000000000000000000 ),
 .UNSPECIFIED. ) ;
#7608=CARTESIAN_POINT ( 'NONE',  ( -15.19604463793445959, 156.0859089222169587, -0.3036531364422413448 ) ) ;
#7612=CARTESIAN_POINT ( 'NONE',  ( -8.213274639754041928, 120.6581850290335609, 1.077640066613805070 ) ) ;
#7613=CARTESIAN_POINT ( 'NONE',  ( 4.264856162967361364, -5.269518785209044154, -1.792273654951743067 ) ) ;
#7614=CARTESIAN_POINT ( 'NONE',  ( 6.860783072103382452, 117.8105958006179890, 0.8866969874101000570 ) ) ;
#7617=CARTESIAN_POINT ( 'NONE',  ( 20.82688902969335487, 148.9555414352193168, -1.562960617212841186 ) ) ;
#7619=CARTESIAN_POINT ( 'NONE',  ( -2.900346660479264482, -2.445871450894649968, -3.618988008572288972 ) ) ;
#7620=CARTESIAN_POINT ( 'NONE',  ( -7.681555067352650035, 158.5863655655865330, -1.054772010160866857 ) ) ;
#7621=EDGE_CURVE ( 'NONE', #36646, #38078, #9140, .T. ) ;
#7623=CARTESIAN_POINT ( 'NONE',  ( -1.597555633484793125, 120.9451058151398399, 0.06333991727891977175 ) ) ;
#7624=CARTESIAN_POINT ( 'NONE',  ( 3.842082824490853810, -15.33115451161810938, 5.194229279690915746 ) ) ;
#7629=CARTESIAN_POINT ( 'NONE',  ( 11.88796246241977883, 122.6721150436042223, 1.770419579776735697 ) ) ;
#7630=CARTESIAN_POINT ( 'NONE',  ( -6.606344270946872901E-14, 95.34346620154573770, 1.014423412895214384E-29 ) ) ;
#7633=CARTESIAN_POINT ( 'NONE',  ( -8.071933480009693795, 118.1206512225135015, 0.6391883341457642587 ) ) ;
#7634=CARTESIAN_POINT ( 'NONE',  ( -5.321447747238043036, 7.245273219182337243, -6.556399146060885919 ) ) ;
#7635=CARTESIAN_POINT ( 'NONE',  ( 16.47979853205664824, 146.5532241433796230, 1.607449420861547962 ) ) ;
#7637=CARTESIAN_POINT ( 'NONE',  ( 21.01068656986052829, 132.3427885975763161, -0.3612206858233396600 ) ) ;
#7638=CARTESIAN_POINT ( 'NONE',  ( 4.698556703264293866, 117.9254231662981738, -0.7749991471470429882 ) ) ;
#7644=CARTESIAN_POINT ( 'NONE',  ( -4.482462170607306895, 118.1125532305710664, 0.5757334087516573495 ) ) ;
#7645=CARTESIAN_POINT ( 'NONE',  ( 1.899379616367111279, 106.4949638843779809, -4.984221880255138792 ) ) ;
#7650=CARTESIAN_POINT ( 'NONE',  ( 3.950356500571747809, 119.0647496460593686, -0.7685950494401324606 ) ) ;
#7651=CARTESIAN_POINT ( 'NONE',  ( -5.384759902136890375, 117.1811293437636721, -0.8990931802006211226 ) ) ;
#7652=CARTESIAN_POINT ( 'NONE',  ( 4.500448308262108732, 118.1244505159430247, 0.6707133188938370072 ) ) ;
#7653=CARTESIAN_POINT ( 'NONE',  ( -1.710293758672658759, 156.3676537730497387, -0.7734167093480263100 ) ) ;
#7656=CARTESIAN_POINT ( 'NONE',  ( 1.144237119838787287, 117.3993836041131402, -1.432026387098619402 ) ) ;
#7657=CARTESIAN_POINT ( 'NONE',  ( -4.559029627765868398, 31.49133049583988253, -0.6947656260628575220 ) ) ;
#7658=CARTESIAN_POINT ( 'NONE',  ( -6.627928625996650780, 155.5185402614932570, -1.342408143365147577 ) ) ;
#7659=CARTESIAN_POINT ( 'NONE',  ( -4.559649833866270541, 116.0444662015457169, -3.750543233647261498 ) ) ;
#7661=CARTESIAN_POINT ( 'NONE',  ( 8.072253591115288174, 121.3304565451444574, -0.9161511751189075348 ) ) ;
#7662=CARTESIAN_POINT ( 'NONE',  ( -1.638793754983947304, 120.9957929572446886, 0.06788950568023216503 ) ) ;
#7664=CARTESIAN_POINT ( 'NONE',  ( 0.9824256172934900944, 116.9078805053781025, 0.3575799159885131306 ) ) ;
#7666=CARTESIAN_POINT ( 'NONE',  ( 3.351397644842732948, -15.05179984492975542, 2.935234935891222641 ) ) ;
#7667=CARTESIAN_POINT ( 'NONE',  ( -3.344131534676259232, 119.2933411826354728, 0.7437009012386071038 ) ) ;
#7668=CARTESIAN_POINT ( 'NONE',  ( 0.7703063551133444431, -5.692625084440793515, -0.5956917769006077057 ) ) ;
#7669=CARTESIAN_POINT ( 'NONE',  ( -19.79238143276398176, 128.7876384977266468, -1.131474956103616814 ) ) ;
#7671=CARTESIAN_POINT ( 'NONE',  ( -0.8573366540693068139, -6.603747334586292261, -0.4721712316449505620 ) ) ;
#7672=VERTEX_POINT ( 'NONE', #818 ) ;
#7674=CARTESIAN_POINT ( 'NONE',  ( 5.590287297675133438, 117.9270669303711117, 0.7481252288361714964 ) ) ;
#7675=CARTESIAN_POINT ( 'NONE',  ( -10.87798892776825177, 126.1616406593870607, 0.4640774846651396501 ) ) ;
#7676=CARTESIAN_POINT ( 'NONE',  ( 4.673344545167823938, -12.29283961637177214, 1.688191869143181201 ) ) ;
#7677=CARTESIAN_POINT ( 'NONE',  ( 10.38102865001212471, 154.1877054190025262, -1.364427777124047170 ) ) ;
#7679=CARTESIAN_POINT ( 'NONE',  ( -11.81048985551422703, 122.0047285378078357, -1.760929439237068017 ) ) ;
#7680=CARTESIAN_POINT ( 'NONE',  ( 3.601325883493490920, 115.7029493296494707, 1.622373432873002175 ) ) ;
#7681=CARTESIAN_POINT ( 'NONE',  ( 2.569204629087775693, -14.95572128602136530, 4.738577790166504933 ) ) ;
#7682=CARTESIAN_POINT ( 'NONE',  ( -4.912057176082959664, 117.6260355129238491, -0.9592288914727921112 ) ) ;
#7683=CARTESIAN_POINT ( 'NONE',  ( 9.164740666423933035, 153.8946005065304803, -0.1038620377607962914 ) ) ;
#7687=DIRECTION ( 'NONE',  ( 0.01997839162482749689, 1.040247600000945640E-18, -0.9998004120163610509 ) ) ;
#7688=FACE_BOUND ( 'NONE', #23877, .T. ) ;
#7691=CARTESIAN_POINT ( 'NONE',  ( 10.80084657379828528, 157.9251727141802633, 0.03745751586626431401 ) ) ;
#7695=CARTESIAN_POINT ( 'NONE',  ( 1.799054236152410224, -15.56691960250831919, 5.455207115090923153 ) ) ;
#7697=CARTESIAN_POINT ( 'NONE',  ( -1.067875954944055072, 33.20386983296905470, 0.7215342646006036587 ) ) ;
#7698=CARTESIAN_POINT ( 'NONE',  ( 13.21388725472894166, 155.5383117973235585, 2.112422614401995080 ) ) ;
#7700=CARTESIAN_POINT ( 'NONE',  ( -3.973931221679809056, 20.38425861574787490, -7.466160517099206473 ) ) ;
#7701=CARTESIAN_POINT ( 'NONE',  ( 2.373934424165132118, 117.2554555581296825, -0.5878954194807157752 ) ) ;
#7702=CARTESIAN_POINT ( 'NONE',  ( -0.5479319383246573638, 107.0594419416054848, -4.854436055212456580 ) ) ;
#7705=CARTESIAN_POINT ( 'NONE',  ( -0.01111760956215399228, 120.5507043431653784, 0.5563706444133253992 ) ) ;
#7706=CARTESIAN_POINT ( 'NONE',  ( -1.214995109038484067, 0.9429784454696930052, -4.460028654918597901 ) ) ;
#7707=EDGE_CURVE ( 'NONE', #26452, #37991, #2291, .T. ) ;
#7709=CARTESIAN_POINT ( 'NONE',  ( -4.766160292286565792, 118.5264896598256854, 0.8411326837336940976 ) ) ;
#7710=CARTESIAN_POINT ( 'NONE',  ( 3.215637690559757456, -14.25221971482225314, 3.321654998001884795 ) ) ;
#7711=CARTESIAN_POINT ( 'NONE',  ( 2.721163413801359177, 112.7379566594982663, -2.570110030560514236 ) ) ;
#7712=CARTESIAN_POINT ( 'NONE',  ( -16.58356254348282732, 122.7279807066903032, 0.3948093068319186716 ) ) ;
#7713=CARTESIAN_POINT ( 'NONE',  ( -0.5795191656544192993, 34.20384076381332505, 3.605158861677521642 ) ) ;
#7716=CARTESIAN_POINT ( 'NONE',  ( -5.182787013109720675, 104.6144662015412905, -1.273143517811092584 ) ) ;
#7717=CARTESIAN_POINT ( 'NONE',  ( 5.315755633098069310, -15.26259334675766866, -0.1387823706055290596 ) ) ;
#7718=CARTESIAN_POINT ( 'NONE',  ( -16.12894526037929666, 128.5601350900737998, 1.548733376446669086 ) ) ;
#7719=CARTESIAN_POINT ( 'NONE',  ( -4.187759052228169132, -5.978784877027076838, 2.003160513425938483 ) ) ;
#7722=CARTESIAN_POINT ( 'NONE',  ( 0.8420595575567756397, 109.5507526474568607, 3.867914470699520102 ) ) ;
#7723=CARTESIAN_POINT ( 'NONE',  ( -16.48541106618858976, 147.8801373804967341, 1.108338632072817465 ) ) ;
#7725=CARTESIAN_POINT ( 'NONE',  ( 7.478391884465288797, 120.4750020944285609, -1.007254920367567808 ) ) ;
#7726=CARTESIAN_POINT ( 'NONE',  ( 0.01111639779257688268, 118.2594330468507593, -0.5563100024230159812 ) ) ;
#7727=CARTESIAN_POINT ( 'NONE',  ( -5.078986093043186045, 82.13546620154573930, -0.1014902294541231570 ) ) ;
#7728=CARTESIAN_POINT ( 'NONE',  ( 4.171308675837464008, 118.2392932148226095, -0.2183557931388009354 ) ) ;
#7730=CARTESIAN_POINT ( 'NONE',  ( 4.443995521150066352, 155.8637389808261275, -0.5396741685193006122 ) ) ;
#7732=CARTESIAN_POINT ( 'NONE',  ( 3.240743527130751200, -15.12236442990058727, 3.435505395146291274 ) ) ;
#7736=CARTESIAN_POINT ( 'NONE',  ( 0.4327634382839667393, 5.975216699623357108, -4.620561613140377055 ) ) ;
#7737=CARTESIAN_POINT ( 'NONE',  ( 10.85577430263303356, 123.7747955097422476, 1.451053175688577390 ) ) ;
#7738=CARTESIAN_POINT ( 'NONE',  ( 0.9281906404964570534, 34.59732502943162302, 2.863135987906453739 ) ) ;
#7739=CARTESIAN_POINT ( 'NONE',  ( -6.932344361571818325, 124.3275308867733600, -0.1272746869527292546 ) ) ;
#7740=CARTESIAN_POINT ( 'NONE',  ( 4.585487687326599726, 17.13547844546973309, 0.5842699607688729424 ) ) ;
#7741=CARTESIAN_POINT ( 'NONE',  ( 15.78392762965199303, 146.2390805666957192, 0.3668625800963858929 ) ) ;
#7745=CARTESIAN_POINT ( 'NONE',  ( 5.563757564550819268, 116.7201818126403197, -0.05438542879854482009 ) ) ;
#7748=CARTESIAN_POINT ( 'NONE',  ( -4.611806494114576438, 117.9324678712513759, -0.9633187536371230486 ) ) ;
#7749=CARTESIAN_POINT ( 'NONE',  ( -0.6996024724826829244, 105.8261742744577276, 5.294786660180783144 ) ) ;
#7751=CARTESIAN_POINT ( 'NONE',  ( 7.936949992814905208, -1.433721018288910853, -2.821688713676304250 ) ) ;
#7757=CARTESIAN_POINT ( 'NONE',  ( -23.25176476241890455, 142.6711341654318801, -0.007203867522443983124 ) ) ;
#7758=AXIS2_PLACEMENT_3D ( 'NONE', #530, #6907, #23060 ) ;
#7764=CARTESIAN_POINT ( 'NONE',  ( -7.044606587285223931, 122.0729346620515088, -0.1407680048458704314 ) ) ;
#7765=CARTESIAN_POINT ( 'NONE',  ( 4.690731670358166738, -15.11132977793584686, 4.439372980131230939 ) ) ;
#7766=CARTESIAN_POINT ( 'NONE',  ( -16.68922378205042634, 153.6190162071354735, 1.533137601955099516 ) ) ;
#7768=CARTESIAN_POINT ( 'NONE',  ( 23.16247218334346414, 146.6831645211815101, 1.199661776592803486 ) ) ;
#7769=CARTESIAN_POINT ( 'NONE',  ( 22.07843093565568893, 149.7938220333360846, -0.9986438184040019594 ) ) ;
#7770=CARTESIAN_POINT ( 'NONE',  ( -4.507778648822867495, 31.37953541088120346, -1.025544427737863362 ) ) ;
#7771=CARTESIAN_POINT ( 'NONE',  ( -23.24214586660315263, 149.3282167461061931, -0.7955682979737040972 ) ) ;
#7775=CARTESIAN_POINT ( 'NONE',  ( -8.767692638887638168, 117.8781970347225609, 0.2943759000137591841 ) ) ;
#7776=CARTESIAN_POINT ( 'NONE',  ( -17.86368224974588514, 148.4245508482893854, 1.618106657999740516 ) ) ;
#7778=CARTESIAN_POINT ( 'NONE',  ( 5.031139012175321668, 119.0545008048120366, -0.9043826811606222593 ) ) ;
#7781=CARTESIAN_POINT ( 'NONE',  ( -0.9317526520580600158, -11.96253880033681050, -0.2928614735302202954 ) ) ;
#7782=CARTESIAN_POINT ( 'NONE',  ( -13.69970117413534361, 155.7522398296385404, -1.951476099255863517 ) ) ;
#7784=CARTESIAN_POINT ( 'NONE',  ( -3.009276887026423264, 50.13146620154573441, 1.210121013456480377 ) ) ;
#7785=CARTESIAN_POINT ( 'NONE',  ( 1.846154440359644600, 156.5029897098349636, -0.9826124536999807368 ) ) ;
#7786=CARTESIAN_POINT ( 'NONE',  ( -10.18105065676974519, 125.9743313966586129, -0.2034416216762103546 ) ) ;
#7788=CARTESIAN_POINT ( 'NONE',  ( -10.84669103489419761, 122.6724665872831679, -1.607685377936339810 ) ) ;
#7789=CARTESIAN_POINT ( 'NONE',  ( 5.320894714828252603, -15.22957080661538320, -0.4730099507937148284 ) ) ;
#7792=CARTESIAN_POINT ( 'NONE',  ( -4.437756799117888562, 118.1258187118189369, -0.7325781917677525179 ) ) ;
#7794=CARTESIAN_POINT ( 'NONE',  ( 4.065926199369043204, 118.2429491485453497, 0.3080910687088499467 ) ) ;
#7795=CARTESIAN_POINT ( 'NONE',  ( 5.440231158483206819, 156.5946142756450570, 1.801097700867929863 ) ) ;
#7797=CARTESIAN_POINT ( 'NONE',  ( 3.703049682113265018, 116.6240124373522065, 0.07399574541707880371 ) ) ;
#7798=CARTESIAN_POINT ( 'NONE',  ( -3.861838729977780993, 14.11015702457025078, 7.483763204152318771 ) ) ;
#7799=CARTESIAN_POINT ( 'NONE',  ( 9.821648630411557335, 124.8790005272986861, 0.5336917924355371046 ) ) ;
#7800=CARTESIAN_POINT ( 'NONE',  ( 14.68046753700549623, 156.0817623197167450, -0.7569547985229806430 ) ) ;
#7801=CARTESIAN_POINT ( 'NONE',  ( 5.334231700979342961, 105.1224708049047649, -0.08243647111397434113 ) ) ;
#7802=CARTESIAN_POINT ( 'NONE',  ( -5.078986093043186045, 97.88346620154572975, -0.1014902294541238092 ) ) ;
#7805=CARTESIAN_POINT ( 'NONE',  ( -15.93439728059136939, 121.0320206851898206, -0.2674320648195325223 ) ) ;
#7808=CARTESIAN_POINT ( 'NONE',  ( 7.890037743085640543, 122.1789050061608179, -0.5073752957019501686 ) ) ;
#7810=ORIENTED_EDGE ( 'NONE', *, *, #1083, .T. ) ;
#7811=CARTESIAN_POINT ( 'NONE',  ( 2.051715782278035416, 115.6909491485438650, -1.638092376821394192 ) ) ;
#7812=CARTESIAN_POINT ( 'NONE',  ( -15.49830880841133585, 147.8629129908177049, -0.8994996151558259934 ) ) ;
#7813=CARTESIAN_POINT ( 'NONE',  ( 4.637598599007382916, -11.68863464395987428, 0.6963472677309354708 ) ) ;
#7814=CARTESIAN_POINT ( 'NONE',  ( -10.16518949684075324, 157.7687470436769388, 1.006875576665116956 ) ) ;
#7816=CARTESIAN_POINT ( 'NONE',  ( 15.69471450241202426, 120.8333755831694702, 0.3643268586347851445 ) ) ;
#7818=CARTESIAN_POINT ( 'NONE',  ( 3.315635589170360831, -10.27688868798473720, -3.234826238065521053 ) ) ;
#7819=CARTESIAN_POINT ( 'NONE',  ( -6.896076486346299994, 117.1676486657671177, -0.1523180551073340938 ) ) ;
#7823=CARTESIAN_POINT ( 'NONE',  ( 6.312484072712937433, 119.3915106940810205, 1.259512802889745764 ) ) ;
#7824=CARTESIAN_POINT ( 'NONE',  ( -1.959332070151295291, -8.942847522256865744, 4.198131957625402144 ) ) ;
#7825=CARTESIAN_POINT ( 'NONE',  ( 10.11685142855833774, 157.7687470436769388, 1.412159022929360797 ) ) ;
#7827=CARTESIAN_POINT ( 'NONE',  ( 20.41374081727966328, 149.7738053052645171, -1.564883410832889288 ) ) ;
#7828=CARTESIAN_POINT ( 'NONE',  ( 0.2036312542886812293, -3.545347522689146214, -4.628372119175537591 ) ) ;
#7829=CARTESIAN_POINT ( 'NONE',  ( -12.78669781772278924, 156.8686255264331635, -1.389142476906146673 ) ) ;
#7830=VERTEX_POINT ( 'NONE', #16560 ) ;
#7831=CARTESIAN_POINT ( 'NONE',  ( -1.594039003485612227, 156.2604006213118453, 0.1692965565027966801 ) ) ;
#7832=CARTESIAN_POINT ( 'NONE',  ( 5.611968257679588845, -14.69514533571547688, 3.041973840610588287 ) ) ;
#7834=CARTESIAN_POINT ( 'NONE',  ( -4.731576593360331096, 114.9758031406737615, -1.766933436629785525 ) ) ;
#7836=CARTESIAN_POINT ( 'NONE',  ( 10.89600635431576592, 121.6366708983051836, 1.687201357748379316 ) ) ;
#7838=EDGE_CURVE ( 'NONE', #20535, #6660, #9093, .T. ) ;
#7840=CARTESIAN_POINT ( 'NONE',  ( -9.476822779618647274, 118.5748184150550060, 0.6643292918320550244 ) ) ;
#7841=CARTESIAN_POINT ( 'NONE',  ( -0.4402761300873825334, 6.286315195291644287, -8.460265346311377499 ) ) ;
#7842=CARTESIAN_POINT ( 'NONE',  ( 16.21957319403749054, 147.1082353761072454, 1.436993664011567029 ) ) ;
#7846=CARTESIAN_POINT ( 'NONE',  ( 22.28323889858834050, 137.0232865695268458, -0.2611169771296153463 ) ) ;
#7853=CARTESIAN_POINT ( 'NONE',  ( -4.415273592266121483, 118.1795755137017352, 0.3920396191190627100 ) ) ;
#7854=CARTESIAN_POINT ( 'NONE',  ( 1.156078607266118219, 106.1808064897588224, -5.165548525996213058 ) ) ;
#7857=CARTESIAN_POINT ( 'NONE',  ( 8.278265034794616284, 120.3444625154268266, -1.110562897522293868 ) ) ;
#7858=CARTESIAN_POINT ( 'NONE',  ( -6.134665891606804422, 119.5049778551863682, -0.5179261928985368080 ) ) ;
#7859=CARTESIAN_POINT ( 'NONE',  ( 4.390279874354320988, 118.1641264082274745, 0.6591387255275874546 ) ) ;
#7860=CARTESIAN_POINT ( 'NONE',  ( -16.28325953274117310, 146.1553843108282820, -1.442930602569014953 ) ) ;
#7861=CARTESIAN_POINT ( 'NONE',  ( -0.5919055904364763920, 115.7030221220078658, -1.760227757477109467 ) ) ;
#7862=CARTESIAN_POINT ( 'NONE',  ( 4.320748297369637392, 118.1651004037386059, -0.5003675618858194341 ) ) ;
#7864=CARTESIAN_POINT ( 'NONE',  ( 5.284833012248379980, 116.4655405006298849, -0.8823810258511326499 ) ) ;
#7865=CARTESIAN_POINT ( 'NONE',  ( -10.87485472805872000, 124.6990478933366404, -1.296628760762302823 ) ) ;
#7867=CARTESIAN_POINT ( 'NONE',  ( 0.09004192032669379453, 116.0444662015457169, -6.160295767268807232 ) ) ;
#7870=CARTESIAN_POINT ( 'NONE',  ( -7.767741303917714113, 154.6911059042232353, 0.01209887248576701525 ) ) ;
#7872=CARTESIAN_POINT ( 'NONE',  ( 22.58684024723470785, 150.0155710288180444, 1.417619447182237646 ) ) ;
#7874=CARTESIAN_POINT ( 'NONE',  ( 3.172822981795960562, -14.65879537465078464, 0.2101774045261552148 ) ) ;
#7875=CARTESIAN_POINT ( 'NONE',  ( -17.49586834669434765, 149.8167423968465073, 1.704004628023328083 ) ) ;
#7876=CARTESIAN_POINT ( 'NONE',  ( -0.4938630982110026046, -9.903502963049303887, 0.8462501600425517134 ) ) ;
#7877=CARTESIAN_POINT ( 'NONE',  ( -22.91074218474016178, 142.4877946823990271, -1.320775467724695007 ) ) ;
#7878=CARTESIAN_POINT ( 'NONE',  ( 0.04477287412000752198, 14.82196177864132380, -0.9729305925282246692 ) ) ;
#7883=CARTESIAN_POINT ( 'NONE',  ( -16.10174665100988989, 146.3760696504137684, 0.5323012926561623281 ) ) ;
#7884=CARTESIAN_POINT ( 'NONE',  ( 4.982342844640083257, -12.32172870019713962, 1.713706004506841740 ) ) ;
#7885=CARTESIAN_POINT ( 'NONE',  ( 7.013665818177395650, 155.6889469082406947, -1.337060831506289071 ) ) ;
#7887=CARTESIAN_POINT ( 'NONE',  ( 3.999473940548379680, 115.7036087109788838, 1.581720450462331673 ) ) ;
#7888=CARTESIAN_POINT ( 'NONE',  ( 3.136003201302111076, -14.34114629734795088, 4.029177829137042366 ) ) ;
#7889=CARTESIAN_POINT ( 'NONE',  ( -4.753076465732039679, 117.6359550804434662, -1.138063527254628671 ) ) ;
#7890=EDGE_CURVE ( 'NONE', #26236, #20434, #2190, .T. ) ;
#7891=CARTESIAN_POINT ( 'NONE',  ( 5.978688551911849558, 155.3719879121972838, 0.01966617979267130945 ) ) ;
#7893=CARTESIAN_POINT ( 'NONE',  ( 6.715107731706551064, 119.1290971219625021, 1.270026890958220855 ) ) ;
#7894=CARTESIAN_POINT ( 'NONE',  ( 1.698749669598698109, 106.4949638843832247, 5.056121066458325153 ) ) ;
#7896=EDGE_CURVE ( 'NONE', #15736, #15805, #2979, .T. ) ;
#7897=DIRECTION ( 'NONE',  ( -0.02488342977054593119, -0.9876883405951414341, -0.1544427297585422298 ) ) ;
#7898=CARTESIAN_POINT ( 'NONE',  ( 14.75425959148282828, 120.3062992333385921, 0.06863422566743783426 ) ) ;
#7900=CARTESIAN_POINT ( 'NONE',  ( 1.920978177995904979, -15.71867150285087611, 5.654812409921664340 ) ) ;
#7901=CARTESIAN_POINT ( 'NONE',  ( -4.943487193438446781, 117.5911938081067092, -0.9706830346222778960 ) ) ;
#7902=CARTESIAN_POINT ( 'NONE',  ( 16.23079787743079194, 153.4734386769207504, 2.282812701028141600 ) ) ;
#7905=CARTESIAN_POINT ( 'NONE',  ( -8.420209349088564110, 12.38497237326411415, -0.2929423126682718648 ) ) ;
#7906=CARTESIAN_POINT ( 'NONE',  ( 8.624984000141996177, 118.6231719595668892, -0.7976843706328619055 ) ) ;
#7907=CARTESIAN_POINT ( 'NONE',  ( -3.137457178758016330, 117.8122656274855871, -0.9631651297103497322 ) ) ;
#7909=CARTESIAN_POINT ( 'NONE',  ( -5.586884702347496123, 94.32746620154571815, -0.1116392523995361624 ) ) ;
#7910=CARTESIAN_POINT ( 'NONE',  ( -4.888957423522264811, 105.1215310813731207, 2.142498686656161055 ) ) ;
#7911=CARTESIAN_POINT ( 'NONE',  ( 3.102408547967445696, -0.5812848888516047863, -3.453265078539196509 ) ) ;
#7913=CARTESIAN_POINT ( 'NONE',  ( -4.766356317893496453, 118.5264896598256854, 0.8410930105509721866 ) ) ;
#7914=CARTESIAN_POINT ( 'NONE',  ( 2.376025398756717699, -14.92724974027714779, 5.073178661078445728 ) ) ;
#7915=CARTESIAN_POINT ( 'NONE',  ( 4.585195778441632619, 124.9344662015457459, 0.09162312381275083961 ) ) ;
#7916=EDGE_CURVE ( 'NONE', #25568, #27127, #18591, .T. ) ;
#7917=CARTESIAN_POINT ( 'NONE',  ( 2.958531772299236362, 39.20946620154573026, 1.329372033065076453 ) ) ;
#7920=CARTESIAN_POINT ( 'NONE',  ( -5.255166069342940283, 105.1223876010384259, -0.9307257834050973733 ) ) ;
#7921=CARTESIAN_POINT ( 'NONE',  ( 2.341541575351651083, -15.74615379138004378, 5.495207524874286875 ) ) ;
#7922=CARTESIAN_POINT ( 'NONE',  ( -13.00445675891842257, 122.7019651155717384, 1.321991537619922719 ) ) ;
#7923=CARTESIAN_POINT ( 'NONE',  ( 0.2723526006440308844, 25.78125159710042169, 0.9401034630801221592 ) ) ;
#7924=ORIENTED_EDGE ( 'NONE', *, *, #26964, .F. ) ;
#7925=ORIENTED_EDGE ( 'NONE', *, *, #14409, .T. ) ;
#7926=CARTESIAN_POINT ( 'NONE',  ( -6.606029807653651701E-14, 92.04146620154574521, -3.372746026535634231E-18 ) ) ;
#7927=CARTESIAN_POINT ( 'NONE',  ( -0.1065646865916382441, 105.8844662015457061, 5.332932678536314697 ) ) ;
#7928=CARTESIAN_POINT ( 'NONE',  ( -9.413719431533529303, 122.9055586947561522, 0.7725895697485187785 ) ) ;
#7931=CARTESIAN_POINT ( 'NONE',  ( 12.69375283655731934, 153.7453525671159298, -1.672805011026380573 ) ) ;
#7932=CARTESIAN_POINT ( 'NONE',  ( -13.64080552068802277, 122.3361261571837986, -1.764911742735522315 ) ) ;
#7934=CARTESIAN_POINT ( 'NONE',  ( 4.401000572156880786, 118.1832674401186409, -0.4088722398549547998 ) ) ;
#7935=CARTESIAN_POINT ( 'NONE',  ( 9.191362964797985313, 123.9301100385560943, -0.1344743934557742215 ) ) ;
#7937=ORIENTED_EDGE ( 'NONE', *, *, #7916, .F. ) ;
#7938=CARTESIAN_POINT ( 'NONE',  ( 3.205191379615736746, -14.47393913169138102, 3.051678166811226500 ) ) ;
#7940=CARTESIAN_POINT ( 'NONE',  ( -4.890164892654324191, 117.4101971730238461, 0.9753743779596022456 ) ) ;
#7943=CARTESIAN_POINT ( 'NONE',  ( 1.463615122064738427, -3.970138727222522590, -4.384008014421088895 ) ) ;
#7944=CARTESIAN_POINT ( 'NONE',  ( 14.05412825714257608, 131.1061190467503934, 1.842221413061617241 ) ) ;
#7945=CARTESIAN_POINT ( 'NONE',  ( 2.393982948168581704, 36.72379010448016601, 1.601961539505906806 ) ) ;
#7946=CARTESIAN_POINT ( 'NONE',  ( -6.983605877934339290, 124.9344662015457175, -0.1395490654994202828 ) ) ;
#7947=CARTESIAN_POINT ( 'NONE',  ( -4.636761822055341042, 12.60011390031314349, 0.2095705037016724059 ) ) ;
#7948=CARTESIAN_POINT ( 'NONE',  ( 15.38115207166213594, 147.8278496344100859, 0.4352178850651141073 ) ) ;
#7949=CARTESIAN_POINT ( 'NONE',  ( 4.834527910505758364, 118.7629491485453030, -0.4653476702560417344 ) ) ;
#7951=CARTESIAN_POINT ( 'NONE',  ( -5.538962611300139116, 116.7971013310818620, -0.4462307559783619815 ) ) ;
#7952=VECTOR ( 'NONE', #27624, 1000.000000000000000 ) ;
#7953=CARTESIAN_POINT ( 'NONE',  ( 0.005099097580972779785, 122.5569158606516993, -0.2551796940110859224 ) ) ;
#7955=CARTESIAN_POINT ( 'NONE',  ( 2.074264724554227612, -15.58053249244905381, 5.900626476732243830 ) ) ;
#7957=CARTESIAN_POINT ( 'NONE',  ( 6.431785950458272616, 8.712657024569978148, -5.436233950049250474 ) ) ;
#7959=CARTESIAN_POINT ( 'NONE',  ( -5.586884702347497011, 104.6144662015457243, -0.1116392523995361624 ) ) ;
#7961=CARTESIAN_POINT ( 'NONE',  ( 0.001261869788119350478, 124.3520329708341876, -0.06314912420803914239 ) ) ;
#7962=CARTESIAN_POINT ( 'NONE',  ( -8.196853576810003261, 117.5993832199734328, 0.1745776481207347852 ) ) ;
#7968=CARTESIAN_POINT ( 'NONE',  ( -11.83539255247756117, 152.0195595274622349, -0.2364993098673504601 ) ) ;
#7969=CARTESIAN_POINT ( 'NONE',  ( 2.850629920820032748, -15.47419331854960056, 5.714803783126763292 ) ) ;
#7970=CARTESIAN_POINT ( 'NONE',  ( -9.089826843847044202, 119.3941581119689204, 1.016340006442031374 ) ) ;
#7971=CARTESIAN_POINT ( 'NONE',  ( 13.85601021432049684, 120.6843904051541898, -0.7167389240433504893 ) ) ;
#7973=CARTESIAN_POINT ( 'NONE',  ( -0.3042230016543463478, 116.5226405152084652, -0.1306790058978155589 ) ) ;
#7976=EDGE_LOOP ( 'NONE', ( #6703, #30391, #22393 ) ) ;
#7977=CARTESIAN_POINT ( 'NONE',  ( -5.563241772947201902, 116.6983512803620471, -0.09199628343113541717 ) ) ;
#7978=CARTESIAN_POINT ( 'NONE',  ( -5.873652769538547425, 120.2771794157441008, 0.8114825934776858096 ) ) ;
#7980=CARTESIAN_POINT ( 'NONE',  ( 19.24794053165960150, 147.9830121424878939, -1.736014841626597471 ) ) ;
#7981=CARTESIAN_POINT ( 'NONE',  ( -21.52700195390597671, 148.3057046726078170, -2.246165485461372846 ) ) ;
#7984=CARTESIAN_POINT ( 'NONE',  ( 1.496072496114335904, 120.3785564700922492, -0.3614901595391030176 ) ) ;
#7987=CARTESIAN_POINT ( 'NONE',  ( -11.45041423386219215, 122.9335272575421669, -1.692945391654126386 ) ) ;
#7988=CARTESIAN_POINT ( 'NONE',  ( 4.174810697594108611, -15.62279056926031728, 2.935701831792822514 ) ) ;
#7989=CIRCLE ( 'NONE', #12053, 3.683000000000001162 ) ;
#7991=CARTESIAN_POINT ( 'NONE',  ( -4.269880260387894033, 118.2136455867637466, -0.5281148321755492203 ) ) ;
#7995=CARTESIAN_POINT ( 'NONE',  ( -4.970228710897478308, 117.5383302079596746, 0.8106020663343151966 ) ) ;
#7996=CARTESIAN_POINT ( 'NONE',  ( 18.00824595900788694, 147.8422069945528108, 2.338981374327670171 ) ) ;
#7998=CARTESIAN_POINT ( 'NONE',  ( 13.67717291712360961, 119.6429072192227494, 0.2244666789651033056 ) ) ;
#7999=CARTESIAN_POINT ( 'NONE',  ( 4.095665791538102063, 15.60827804425945331, 7.401523448874606892 ) ) ;
#8000=CARTESIAN_POINT ( 'NONE',  ( 15.84614414026241924, 146.9522167609303267, 0.9100203137935939379 ) ) ;
#8001=CARTESIAN_POINT ( 'NONE',  ( 4.973152232786927307, 117.3993868326352015, 0.9753084504214339923 ) ) ;
#8002=CARTESIAN_POINT ( 'NONE',  ( 5.314256983240370324, 105.1224655745845382, -0.4585143440169748841 ) ) ;
#8005=CARTESIAN_POINT ( 'NONE',  ( -6.904872195170285387, 117.1762911274595496, -0.05199240921585723124 ) ) ;
#8008=CARTESIAN_POINT ( 'NONE',  ( 5.796788256709977105, 121.1606928603264492, -0.2966676035594191796 ) ) ;
#8009=CARTESIAN_POINT ( 'NONE',  ( -8.709803600792287881, 118.1821829479768553, 0.5645179937759793320 ) ) ;
#8012=CARTESIAN_POINT ( 'NONE',  ( -15.82044549406361611, 146.2622375132148989, -0.6472507553222681675 ) ) ;
#8013=CARTESIAN_POINT ( 'NONE',  ( 4.828046317437772572, -12.99562652935115636, 2.825559498992329832 ) ) ;
#8014=CARTESIAN_POINT ( 'NONE',  ( -15.58647730463680325, 154.9569273371780298, 1.293949759430877533 ) ) ;
#8016=CARTESIAN_POINT ( 'NONE',  ( 16.23049043870583930, 121.3954344197762083, 0.4305223454732414190 ) ) ;
#8017=CARTESIAN_POINT ( 'NONE',  ( 10.39928917620358817, 153.1223395828141918, 0.2078025466733119664 ) ) ;
#8019=CARTESIAN_POINT ( 'NONE',  ( 0.9593126492114073534, 18.43563504644844642, -0.1793159252426369810 ) ) ;
#8020=CARTESIAN_POINT ( 'NONE',  ( -22.98446660148367826, 150.1594536303649932, -0.4849100737359563484 ) ) ;
#8021=CARTESIAN_POINT ( 'NONE',  ( 5.008579095262371439, 117.3966161975143052, -0.7759206765000108419 ) ) ;
#8023=CARTESIAN_POINT ( 'NONE',  ( 5.078986093043053707, 94.83546620154572793, 0.1014902294541237954 ) ) ;
#8025=CARTESIAN_POINT ( 'NONE',  ( -3.063299625903500800, 117.4009674993953780, 0.6350039608490424259 ) ) ;
#8026=CARTESIAN_POINT ( 'NONE',  ( 3.679437910380295218, 2.726752568732802917, 2.794697870780981752 ) ) ;
#8027=CARTESIAN_POINT ( 'NONE',  ( 22.07432572979840657, 148.5290936231802448, 2.031061984987305280 ) ) ;
#8029=CARTESIAN_POINT ( 'NONE',  ( 20.28847770310427734, 149.9354415288716780, -1.565775960057087524 ) ) ;
#8030=CARTESIAN_POINT ( 'NONE',  ( 0.8067276567327370529, -3.745225398377231674, -4.556403025205434609 ) ) ;
#8031=CARTESIAN_POINT ( 'NONE',  ( -11.19826879832072031, 119.1264784044212632, -1.044736191152864091 ) ) ;
#8032=CARTESIAN_POINT ( 'NONE',  ( 4.980187925143842342, 117.5315200247294456, -0.7740374538369801938 ) ) ;
#8033=ORIENTED_EDGE ( 'NONE', *, *, #22149, .T. ) ;
#8034=CARTESIAN_POINT ( 'NONE',  ( -8.102825354745354147, 122.8525693413601800, -0.01624079103423752349 ) ) ;
#8035=CARTESIAN_POINT ( 'NONE',  ( 4.535621022044703743, -15.16026073378742822, 4.605481170969206062 ) ) ;
#8037=CARTESIAN_POINT ( 'NONE',  ( 0.02808993038205571599, 117.9496054766756288, -1.405735097488628682 ) ) ;
#8039=CARTESIAN_POINT ( 'NONE',  ( 5.971676678096363489, 157.1185343457808301, 1.951309749225692558 ) ) ;
#8042=CARTESIAN_POINT ( 'NONE',  ( -12.95464425825008803, 119.9671592456446803, 0.6090756887631915140 ) ) ;
#8043=CARTESIAN_POINT ( 'NONE',  ( 8.270632439779459943, 13.09856730479051912, 1.690137114335896751 ) ) ;
#8044=CARTESIAN_POINT ( 'NONE',  ( 16.27374876192079256, 146.7930872653447523, 1.439762483169732876 ) ) ;
#8046=CARTESIAN_POINT ( 'NONE',  ( 23.15061725546894067, 148.7607265879045144, -0.2678260907677694758 ) ) ;
#8049=SURFACE_SIDE_STYLE ('',( #1260 ) ) ;
#8053=CARTESIAN_POINT ( 'NONE',  ( -4.254034338640801494, 118.2250400857918038, 0.3060042376985389612 ) ) ;
#8054=CARTESIAN_POINT ( 'NONE',  ( 3.041860522939319189, 107.5209036112489969, -4.373094760128172886 ) ) ;
#8055=EDGE_LOOP ( 'NONE', ( #13032, #42124 ) ) ;
#8057=CARTESIAN_POINT ( 'NONE',  ( -8.270437544260451190, 120.1331483986364503, -1.449690397053889690 ) ) ;
#8058=CARTESIAN_POINT ( 'NONE',  ( -5.183518906920142832, 115.4398124677065596, -1.515634836823671838 ) ) ;
#8059=CARTESIAN_POINT ( 'NONE',  ( 4.303048441523191769, 118.2117257955810317, 0.4941738720055364742 ) ) ;
#8060=CARTESIAN_POINT ( 'NONE',  ( -13.47315239181501845, 134.2048320552371763, -1.097568958570526165 ) ) ;
#8061=CARTESIAN_POINT ( 'NONE',  ( 0.3943891902157575791, 117.3993832487344520, -1.481047929051600986 ) ) ;
#8063=CARTESIAN_POINT ( 'NONE',  ( 4.256838582791900194, 16.71066835407712858, 1.825063967593055558 ) ) ;
#8064=CARTESIAN_POINT ( 'NONE',  ( -4.884089373684617819, 156.1188696671683260, -1.381267178739763235 ) ) ;
#8065=CARTESIAN_POINT ( 'NONE',  ( -6.474089935681887051E-14, 69.94346620154573202, 3.752704589293910110E-29 ) ) ;
#8068=CARTESIAN_POINT ( 'NONE',  ( -5.338855604227259910, 121.3506614897932252, 0.002391977014555100173 ) ) ;
#8070=CARTESIAN_POINT ( 'NONE',  ( 3.682264917456192332, 94.83546620154572793, 0.07358041635423968885 ) ) ;
#8071=CARTESIAN_POINT ( 'NONE',  ( 7.798299699696582543, 158.6358315003295161, 0.8787250540639038876 ) ) ;
#8073=CARTESIAN_POINT ( 'NONE',  ( 3.216700609619024931, -14.42020774479446921, 2.887214088933996337 ) ) ;
#8074=CARTESIAN_POINT ( 'NONE',  ( 12.29982474031027806, 156.6574886424908470, -1.289654987246353857 ) ) ;
#8075=CARTESIAN_POINT ( 'NONE',  ( -12.93728320859319147, 153.8477531742089468, 1.710492906883538167 ) ) ;
#8077=CARTESIAN_POINT ( 'NONE',  ( 0.4551624184790937777, -5.041848893434334400, -0.8611515851349844652 ) ) ;
#8078=CARTESIAN_POINT ( 'NONE',  ( -0.9591953284562637627, 116.7682604261274264, -0.2970936445032629769 ) ) ;
#8079=CARTESIAN_POINT ( 'NONE',  ( -0.07513956969218944792, 19.57165678886816096, 0.9711860325417217554 ) ) ;
#8082=CARTESIAN_POINT ( 'NONE',  ( -9.185752227574177198, 123.6526633469202920, 0.3199782652467454969 ) ) ;
#8083=CARTESIAN_POINT ( 'NONE',  ( 4.994336218630399671, -12.17445384341683834, 1.469335147697719890 ) ) ;
#8084=CARTESIAN_POINT ( 'NONE',  ( 3.633016119382470599, 156.6183338678525558, -1.377765736259032536 ) ) ;
#8086=CARTESIAN_POINT ( 'NONE',  ( 0.7503318161881147308, 115.7029095348785148, 1.755759173997271105 ) ) ;
#8087=CARTESIAN_POINT ( 'NONE',  ( 3.066387819753066069, -14.51305101688413224, 3.912045622741378903 ) ) ;
#8090=CARTESIAN_POINT ( 'NONE',  ( 10.41298992473515561, 153.0987333575537548, 0.09138415589099070646 ) ) ;
#8092=CARTESIAN_POINT ( 'NONE',  ( 20.22212501804812490, 145.4934252350392114, 2.489959791085248231 ) ) ;
#8093=CARTESIAN_POINT ( 'NONE',  ( 2.743188893672867223, 107.9147049449198903, 4.446318134730120164 ) ) ;
#8094=DIRECTION ( 'NONE',  ( -0.9998004120163608288, -5.205824365704082573E-17, -0.01997839162482749342 ) ) ;
#8096=CARTESIAN_POINT ( 'NONE',  ( 23.19846888548980601, 149.6199392087789306, 0.2334144245939554496 ) ) ;
#8097=CIRCLE ( 'NONE', #28497, 5.588000000000006295 ) ;
#8099=CARTESIAN_POINT ( 'NONE',  ( 1.702263513459753907, -15.37342380949326071, 5.866026421007169311 ) ) ;
#8101=FACE_OUTER_BOUND ( 'NONE', #12928, .T. ) ;
#8102=CARTESIAN_POINT ( 'NONE',  ( -4.783018391820325732, 117.8919472439429796, 0.7199156508651073372 ) ) ;
#8104=CARTESIAN_POINT ( 'NONE',  ( 5.064488095677227797, 115.7029491485453150, -1.196137279639045259 ) ) ;
#8105=CARTESIAN_POINT ( 'NONE',  ( -8.512111711805967929, 118.9720400677293810, -1.270775419876498669 ) ) ;
#8106=CARTESIAN_POINT ( 'NONE',  ( -0.3635706870684802805, 106.2969274751293938, -5.168771910137537340 ) ) ;
#8107=CARTESIAN_POINT ( 'NONE',  ( 4.734360898042774046, 117.6653353942706843, 1.129076436732644906 ) ) ;
#8109=CARTESIAN_POINT ( 'NONE',  ( -5.075364051007695387, 105.1217683680384027, 1.652234970701472738 ) ) ;
#8110=CARTESIAN_POINT ( 'NONE',  ( -0.5496829067194369811, 0.7180641350488168317, -4.598301960397928489 ) ) ;
#8112=CARTESIAN_POINT ( 'NONE',  ( -5.237832120027548832, 115.7029491485453860, -1.023639123012231034 ) ) ;
#8113=CARTESIAN_POINT ( 'NONE',  ( 3.302240090359226610, -14.10740904597654399, 3.820541190522989350 ) ) ;
#8115=CARTESIAN_POINT ( 'NONE',  ( 4.036547470782338998, 117.2022048034790487, -0.8857695023546173774 ) ) ;
#8116=CARTESIAN_POINT ( 'NONE',  ( -4.923982053054707819, 28.56637592605547837, 2.110792280427853385 ) ) ;
#8117=CARTESIAN_POINT ( 'NONE',  ( -0.8472532152023458663, 115.7028161379835893, 1.722469557941253226 ) ) ;
#8119=CARTESIAN_POINT ( 'NONE',  ( -5.137756011363697084, 104.6144662015446585, -1.444153010337383192 ) ) ;
#8120=CARTESIAN_POINT ( 'NONE',  ( 4.493636945811098293, -15.48460478268967577, 1.406059860741644574 ) ) ;
#8121=CARTESIAN_POINT ( 'NONE',  ( -12.60853345060003328, 122.2722385251898771, 1.300450782769299929 ) ) ;
#8122=CARTESIAN_POINT ( 'NONE',  ( -0.2871545817224689379, 15.30011720780053430, 0.9385489134671207712 ) ) ;
#8126=CARTESIAN_POINT ( 'NONE',  ( 4.551180572033469929, 124.4408722044843927, 0.1097773164883772967 ) ) ;
#8127=CARTESIAN_POINT ( 'NONE',  ( -4.403754988258326897, 120.5100497556178567, 0.5130326506441985623 ) ) ;
#8130=CARTESIAN_POINT ( 'NONE',  ( 4.625065594204414765, 118.0227253997019261, -0.6695745435591143879 ) ) ;
#8131=CARTESIAN_POINT ( 'NONE',  ( 4.293775319275984437, 119.8084884740358547, -0.7325880323699281993 ) ) ;
#8133=CARTESIAN_POINT ( 'NONE',  ( -3.146714701749098619, 118.3302933575512412, -0.8734028913305706965 ) ) ;
#8136=CARTESIAN_POINT ( 'NONE',  ( 4.298646650716237971, 118.2143447890847767, -0.3450677996601986819 ) ) ;
#8137=CARTESIAN_POINT ( 'NONE',  ( 10.62256650593128349, 126.1357510980948575, -0.2607537273017399571 ) ) ;
#8139=CARTESIAN_POINT ( 'NONE',  ( 3.221735024265227398, -14.36526069886394730, 2.718910799868354378 ) ) ;
#8140=( BOUNDED_SURFACE ( )  B_SPLINE_SURFACE ( 3, 2, ( 
 ( #16191, #41800, #18763 ),
 ( #9607, #18979, #15780 ),
 ( #9400, #6422, #22364 ),
 ( #35389, #6219, #29196 ) ),
 .UNSPECIFIED., .F., .F., .F. ) 
 B_SPLINE_SURFACE_WITH_KNOTS ( ( 4, 4 ),
 ( 3, 3 ),
 ( 0.001248665271192764357, 0.001438387644263458293 ),
 ( 0.000000000000000000, 0.2793900051564218168 ),
 .UNSPECIFIED. ) 
 GEOMETRIC_REPRESENTATION_ITEM ( )  RATIONAL_B_SPLINE_SURFACE ( (
 ( 1.000000000000000000, 0.9330598963482298336, 0.9035245845053385683),
 ( 1.000000000000000000, 0.9330598627208536167, 0.9035245360408918902),
 ( 1.000000000000000000, 0.9330598214100492838, 0.9035244765029348812),
 ( 1.000000000000000000, 0.9330598214935086343, 0.9035244766232181091) ) ) 
 REPRESENTATION_ITEM ( '' )  SURFACE ( )  );
#8141=CARTESIAN_POINT ( 'NONE',  ( -4.801647862234980302, 117.4032733357427105, 1.015449305853463491 ) ) ;
#8144=CARTESIAN_POINT ( 'NONE',  ( 3.440871586586784936, -6.993729544307834445, 3.087053954803492761 ) ) ;
#8145=CARTESIAN_POINT ( 'NONE',  ( 0.7897433827103791382, 156.7682548876429109, 1.239156740209750529 ) ) ;
#8146=CARTESIAN_POINT ( 'NONE',  ( -0.9149567752697743694, 32.47697140010484418, 3.785418454572508473 ) ) ;
#8147=CARTESIAN_POINT ( 'NONE',  ( -7.426015305410983203, 123.6670498955208473, -0.1137005639190685757 ) ) ;
#8148=CARTESIAN_POINT ( 'NONE',  ( 4.440015753948663324, -2.305524871907271400, 1.325333094644747245 ) ) ;
#8149=CARTESIAN_POINT ( 'NONE',  ( 9.144532176012500457, 124.1724329610943300, 0.2170005234668581362 ) ) ;
#8154=CARTESIAN_POINT ( 'NONE',  ( -2.153153780027678099, 116.6795619169676712, -0.4673014195697471340 ) ) ;
#8157=CARTESIAN_POINT ( 'NONE',  ( -1.454323051397943489, 106.2083702520809396, 5.134232663482987569 ) ) ;
#8159=CARTESIAN_POINT ( 'NONE',  ( 7.178138493693461797, 8.485180552427815215, -4.444891729080387321 ) ) ;
#8162=CARTESIAN_POINT ( 'NONE',  ( 1.979187190576821465, -15.21425526833739639, 5.301287498526151332 ) ) ;
#8163=ADVANCED_FACE ( 'NONE', ( #34442 ), #24481, .F. ) ;
#8164=CARTESIAN_POINT ( 'NONE',  ( 0.07157677169882613322, 110.3683645023726569, -3.581994345755985076 ) ) ;
#8165=CARTESIAN_POINT ( 'NONE',  ( -22.47739742037834176, 150.5824416163731314, 0.2728482117335696566 ) ) ;
#8171=CARTESIAN_POINT ( 'NONE',  ( -3.758730197597831779, 121.0943292417197199, -0.07510837462871987336 ) ) ;
#8172=CARTESIAN_POINT ( 'NONE',  ( 5.915669078949217230, -14.48123931593440972, 2.327441804047190033 ) ) ;
#8173=CARTESIAN_POINT ( 'NONE',  ( -18.49784594330485987, 151.8926627062091086, 1.576652458532301182 ) ) ;
#8175=CARTESIAN_POINT ( 'NONE',  ( 8.071933480009564121, 118.1206512225135015, -0.6391883341457641476 ) ) ;
#8176=CARTESIAN_POINT ( 'NONE',  ( -3.366035089439492811, 13.68705809737886447, 3.178168622443589886 ) ) ;
#8177=CARTESIAN_POINT ( 'NONE',  ( -23.25077945365681487, 149.0206351951634076, -0.9193108337986202194 ) ) ;
#8181=CARTESIAN_POINT ( 'NONE',  ( -17.49548072478915728, 148.2779598588913643, 1.530134328283176526 ) ) ;
#8183=CARTESIAN_POINT ( 'NONE',  ( 15.27645447632537490, 153.0676604005411434, -1.747501773188613772 ) ) ;
#8184=CARTESIAN_POINT ( 'NONE',  ( -9.146501239663658467, 119.1751624949753534, -1.313831160619747251 ) ) ;
#8186=CARTESIAN_POINT ( 'NONE',  ( 15.20409169301239949, 148.9716719698033387, -0.7946991634813624916 ) ) ;
#8187=ORIENTED_EDGE ( 'NONE', *, *, #7169, .T. ) ;
#8188=CARTESIAN_POINT ( 'NONE',  ( -13.34752792037781788, 125.8771108566470502, -1.915935069336977659 ) ) ;
#8189=CARTESIAN_POINT ( 'NONE',  ( 3.893829680932177517, -15.58178733528788129, 3.041689768969074503 ) ) ;
#8190=CARTESIAN_POINT ( 'NONE',  ( -4.381356941451189257, 118.1833196942565394, -0.5842306280113004346 ) ) ;
#8192=CARTESIAN_POINT ( 'NONE',  ( -5.003023251195230614, 117.4023580318003184, 0.8028984813139020682 ) ) ;
#8193=CARTESIAN_POINT ( 'NONE',  ( 0.5133504486496096586, 119.5442839488369628, 0.5494766105906194742 ) ) ;
#8194=CARTESIAN_POINT ( 'NONE',  ( -6.651972016613293606E-14, 104.1064662015457287, 7.011588703784780528E-31 ) ) ;
#8195=CARTESIAN_POINT ( 'NONE',  ( 15.19466275752361462, 156.0906695176550443, 0.2814020119901242678 ) ) ;
#8196=CARTESIAN_POINT ( 'NONE',  ( 2.951631207686332470, -3.807527625098089175, 7.891363245966695139 ) ) ;
#8197=CARTESIAN_POINT ( 'NONE',  ( 8.672603809708727240, 123.3259068333282755, 0.4768435845110675642 ) ) ;
#8198=CARTESIAN_POINT ( 'NONE',  ( 4.801257864230994876, 117.4019737406461843, -1.015743596227263179 ) ) ;
#8201=CARTESIAN_POINT ( 'NONE',  ( -4.812480952929572453, 117.4093055390909797, -1.196567565725688231 ) ) ;
#8206=CARTESIAN_POINT ( 'NONE',  ( -3.292377373361788262, 159.4686222989141697, 0.02724393823342696752 ) ) ;
#8207=ORIENTED_EDGE ( 'NONE', *, *, #3230, .F. ) ;
#8209=CARTESIAN_POINT ( 'NONE',  ( 6.905879605078832917, 121.7555842300460682, -0.3103901444470414939 ) ) ;
#8211=CARTESIAN_POINT ( 'NONE',  ( 0.1363104457296995253, 115.6909491485452719, -1.761380027197414266 ) ) ;
#8212=CARTESIAN_POINT ( 'NONE',  ( -0.6270554149911886643, 120.8998192842950488, -0.1385313962210437677 ) ) ;
#8213=CARTESIAN_POINT ( 'NONE',  ( 4.431203275146504694, -13.68733396499126265, 3.949578922469492603 ) ) ;
#8214=CARTESIAN_POINT ( 'NONE',  ( -7.282534483022796934, 158.3006260280594404, 1.262407574188499249 ) ) ;
#8215=CARTESIAN_POINT ( 'NONE',  ( -6.758592445694407663E-14, 130.0144662015457300, 5.650815781856659706E-18 ) ) ;
#8216=CARTESIAN_POINT ( 'NONE',  ( 11.70340384973333059, 118.7242475115495495, 0.3301557443347883924 ) ) ;
#8217=ADVANCED_FACE ( 'NONE', ( #39113 ), #38340, .T. ) ;
#8218=CARTESIAN_POINT ( 'NONE',  ( 5.950997316710809670, 155.3987497974532062, 0.1711121705728039510 ) ) ;
#8220=CARTESIAN_POINT ( 'NONE',  ( -0.8313783143457759151, 22.10655722792919065, -0.5139362334944024280 ) ) ;
#8221=CARTESIAN_POINT ( 'NONE',  ( -17.29877781292331562, 122.7677429521249053, -0.3633837628929260100 ) ) ;
#8222=CYLINDRICAL_SURFACE ( 'NONE', #19441, 5.588000000000006295 ) ;
#8226=ORIENTED_EDGE ( 'NONE', *, *, #21855, .T. ) ;
#8227=CARTESIAN_POINT ( 'NONE',  ( -6.041875895422170295, 118.7642705874486637, 0.9760351844723705872 ) ) ;
#8229=CARTESIAN_POINT ( 'NONE',  ( 19.40029886644210322, 131.9512773411433670, 1.949052778313794088 ) ) ;
#8231=CARTESIAN_POINT ( 'NONE',  ( 20.30545318303836311, 145.4934252350392114, -1.680122328351855598 ) ) ;
#8232=CARTESIAN_POINT ( 'NONE',  ( -6.895871986696200828, 19.14539577913392066, 4.887076909655228896 ) ) ;
#8233=CARTESIAN_POINT ( 'NONE',  ( -2.920589480036270835, 117.1197906563906344, -0.5561477985301582772 ) ) ;
#8234=CARTESIAN_POINT ( 'NONE',  ( 4.785785881226994221, 117.6676823434926149, -0.9347408560558295720 ) ) ;
#8236=ORIENTED_EDGE ( 'NONE', *, *, #11582, .T. ) ;
#8237=CARTESIAN_POINT ( 'NONE',  ( -7.051595240896901373, 122.0586610246435129, -0.007850877590933749012 ) ) ;
#8238=CARTESIAN_POINT ( 'NONE',  ( 5.861737433447875567, -14.68024823731529871, 2.247769314782747774 ) ) ;
#8241=CARTESIAN_POINT ( 'NONE',  ( -4.785365374205540867, 117.3993836135881708, -1.202560736569652677 ) ) ;
#8242=EDGE_LOOP ( 'NONE', ( #4669, #25772, #18551, #39628, #10050, #25815, #27622, #31026, #10615, #14845 ) ) ;
#8243=CARTESIAN_POINT ( 'NONE',  ( 0.4763900686812377883, 119.0154928070276412, 0.6070730232697147954 ) ) ;
#8245=CARTESIAN_POINT ( 'NONE',  ( 4.610436209567292387, 117.9340757871244847, 0.9619774773656434297 ) ) ;
#8246=CARTESIAN_POINT ( 'NONE',  ( -0.7593927098684029042, 117.6736730875354766, 1.153084249965024455 ) ) ;
#8247=CARTESIAN_POINT ( 'NONE',  ( -8.389224625646681588, -1.175411479303250628, -1.011143247504549869 ) ) ;
#8248=CARTESIAN_POINT ( 'NONE',  ( 8.969937932052559404, 123.1852847016406685, 0.8267063328025513469 ) ) ;
#8250=CARTESIAN_POINT ( 'NONE',  ( 23.13757068712586573, 148.9583646262859133, -0.2674444443938934768 ) ) ;
#8256=DIRECTION ( 'NONE',  ( 0.9998004120163608288, 0.000000000000000000, 0.01997839162482749342 ) ) ;
#8257=CARTESIAN_POINT ( 'NONE',  ( -4.317796372703391228, 118.2120857186201732, 0.3236837648097654063 ) ) ;
#8258=CARTESIAN_POINT ( 'NONE',  ( 0.1066086480733247077, 105.8844037013956410, -5.332931792593717191 ) ) ;
#8262=CARTESIAN_POINT ( 'NONE',  ( -4.138294784885184541, 119.2769814663382419, -0.9260517387791210586 ) ) ;
#8264=AXIS2_PLACEMENT_3D ( 'NONE', #40228, #11022, #23366 ) ;
#8265=CARTESIAN_POINT ( 'NONE',  ( 4.229037014694107199, 118.2245626801250182, 0.4851524337614830373 ) ) ;
#8266=CARTESIAN_POINT ( 'NONE',  ( -10.85076598842381124, 126.1616406593870607, -0.8982697194533707519 ) ) ;
#8268=CARTESIAN_POINT ( 'NONE',  ( 11.74288454345096788, 118.7273140689154616, 0.2346507796901761422 ) ) ;
#8270=ORIENTED_EDGE ( 'NONE', *, *, #19599, .F. ) ;
#8271=CARTESIAN_POINT ( 'NONE',  ( 4.300553167417687561, 27.50566818391071422, -1.719522505244270860 ) ) ;
#8272=CARTESIAN_POINT ( 'NONE',  ( -10.10772093100563751, 154.1059161911440469, -1.650231108813019043 ) ) ;
#8274=CARTESIAN_POINT ( 'NONE',  ( -0.1064799869812408512, 105.7853621660184444, 5.332934571178566507 ) ) ;
#8276=CARTESIAN_POINT ( 'NONE',  ( 6.070556577249959673, 121.4252507025452559, 0.3080570883581159047 ) ) ;
#8278=CARTESIAN_POINT ( 'NONE',  ( 0.3408176794664849463, 116.9919054422455531, 0.3412737040790792542 ) ) ;
#8279=DIRECTION ( 'NONE',  ( 0.9998004120163608288, 0.000000000000000000, 0.01997839162482736852 ) ) ;
#8280=CARTESIAN_POINT ( 'NONE',  ( 1.822811606207361823, -15.29362660170947841, 5.402418844745947801 ) ) ;
#8281=CARTESIAN_POINT ( 'NONE',  ( 18.85079593648338658, 152.0234722879370111, -1.474728064877437017 ) ) ;
#8282=CARTESIAN_POINT ( 'NONE',  ( -1.325863631979564472, 119.1766673560425858, 0.6173222594915838135 ) ) ;
#8284=CARTESIAN_POINT ( 'NONE',  ( 0.7467592606654794851, -15.18718160513664195, -0.6397234560659120772 ) ) ;
#8285=CARTESIAN_POINT ( 'NONE',  ( -16.63860074592949445, 155.2617138006751532, -0.9902706816744289986 ) ) ;
#8286=CARTESIAN_POINT ( 'NONE',  ( 0.9436776830090995993, 12.87300645547595046, -0.2395577073833762005 ) ) ;
#8289=CARTESIAN_POINT ( 'NONE',  ( -12.39727431377436062, 130.6617397222824479, 0.4182072254281061219 ) ) ;
#8290=CARTESIAN_POINT ( 'NONE',  ( 4.778253948640466042, -14.19231145175180231, 4.234097743872750286 ) ) ;
#8291=CARTESIAN_POINT ( 'NONE',  ( 6.570524231283992656, 120.8223817900871495, -0.7604033795411312413 ) ) ;
#8294=CARTESIAN_POINT ( 'NONE',  ( 1.665672165190749565, 115.7029491485453434, 1.727344103749859583 ) ) ;
#8297=CARTESIAN_POINT ( 'NONE',  ( 2.376025398756717699, -14.92724974027714779, 5.073178661078445728 ) ) ;
#8298=CARTESIAN_POINT ( 'NONE',  ( -4.854266779389924125, 117.7484759862343964, -0.9334171246494462615 ) ) ;
#8299=CARTESIAN_POINT ( 'NONE',  ( 14.68196552533998123, 148.8424012017631242, 0.1663232928928552179 ) ) ;
#8300=ORIENTED_EDGE ( 'NONE', *, *, #13123, .T. ) ;
#8301=CARTESIAN_POINT ( 'NONE',  ( 1.175363150376307564, 118.2527139659984101, 0.6673024542226162481 ) ) ;
#8302=CARTESIAN_POINT ( 'NONE',  ( -6.654617103318593247E-14, 104.6144662015457243, 1.534725424433578570E-31 ) ) ;
#8304=CARTESIAN_POINT ( 'NONE',  ( 0.0008202526017135117458, 159.6052337359418800, -0.04104879434819952433 ) ) ;
#8305=CARTESIAN_POINT ( 'NONE',  ( 0.9174821693851576976, 116.5216256635990391, -0.1124321123350597307 ) ) ;
#8307=CARTESIAN_POINT ( 'NONE',  ( 1.731823037650620289, -15.42244943691900616, 5.436280266706707387 ) ) ;
#8309=DIRECTION ( 'NONE',  ( -0.9998004120163608288, 0.000000000000000000, -0.01997839162482749342 ) ) ;
#8310=CARTESIAN_POINT ( 'NONE',  ( -4.672965529255816541, 117.9840894666471058, 0.6969538851604538676 ) ) ;
#8311=ORIENTED_EDGE ( 'NONE', *, *, #14937, .T. ) ;
#8313=CARTESIAN_POINT ( 'NONE',  ( -2.936339730833952277, 118.0886593047229667, -0.8676653305777561886 ) ) ;
#8314=CARTESIAN_POINT ( 'NONE',  ( -4.551180572033598715, 124.4408722044843927, -0.1097773164883771579 ) ) ;
#8316=CARTESIAN_POINT ( 'NONE',  ( 4.806277061065945766, 117.4760889790769909, 1.179883221431397455 ) ) ;
#8318=CARTESIAN_POINT ( 'NONE',  ( -0.1065646865916158176, 105.8844662015456919, 5.332932678536313809 ) ) ;
#8320=CARTESIAN_POINT ( 'NONE',  ( -3.416230376366909294, -5.529048218071860532, 3.121479803864907865 ) ) ;
#8323=CARTESIAN_POINT ( 'NONE',  ( 3.416089938271958726, -12.71546774565127080, 1.400931973480754822 ) ) ;
#8324=CARTESIAN_POINT ( 'NONE',  ( 0.6941271473898690259, 106.1608668108878817, -5.200699783222979988 ) ) ;
#8326=CARTESIAN_POINT ( 'NONE',  ( -3.216045294022573220, 29.79186273158684983, 3.430717191674401700 ) ) ;
#8327=CARTESIAN_POINT ( 'NONE',  ( -0.3155423528362975016, 115.7029491485453718, 1.753374870527287355 ) ) ;
#8328=CARTESIAN_POINT ( 'NONE',  ( -3.685501180670149424, 30.72893705507438611, -2.802369389919810772 ) ) ;
#8330=CARTESIAN_POINT ( 'NONE',  ( -5.339818517979998624, 105.1224975962397110, -0.2412077680896454468 ) ) ;
#8331=CARTESIAN_POINT ( 'NONE',  ( 4.008975597637738808, -15.55340266690961926, 2.658432704422428738 ) ) ;
#8332=CARTESIAN_POINT ( 'NONE',  ( -1.119065284002324745, 158.2739225783580537, 1.587016747512054238 ) ) ;
#8333=CARTESIAN_POINT ( 'NONE',  ( 0.7290388503741822568, 0.07276798020498101427, -0.6497956273326017662 ) ) ;
#8334=CARTESIAN_POINT ( 'NONE',  ( -0.009113691291695666039, 25.33460033795575583, 0.9756159547818916700 ) ) ;
#8335=ORIENTED_EDGE ( 'NONE', *, *, #18832, .T. ) ;
#8336=AXIS2_PLACEMENT_3D ( 'NONE', #28372, #18982, #38179 ) ;
#8339=CARTESIAN_POINT ( 'NONE',  ( 1.881281939329280117, 113.2583846565721757, 2.513576850050686318 ) ) ;
#8340=CARTESIAN_POINT ( 'NONE',  ( -5.880513813086854391, 121.0368588677253143, 0.5043468530174899378 ) ) ;
#8342=CARTESIAN_POINT ( 'NONE',  ( 4.610465475190451912, 118.0209586553088172, -0.6829666416481755542 ) ) ;
#8343=CARTESIAN_POINT ( 'NONE',  ( 7.441788261791815628, 120.6159063994810055, -0.9748553081951374377 ) ) ;
#8344=CARTESIAN_POINT ( 'NONE',  ( -16.37183938475186906, 128.5611466799914240, -2.176631273311136372 ) ) ;
#8346=CARTESIAN_POINT ( 'NONE',  ( -0.02244247360070322078, 39.09286639261657115, 1.286999615499953231 ) ) ;
#8347=CARTESIAN_POINT ( 'NONE',  ( 7.078188358610526087, 121.9740017686541194, -0.1969649471280497111 ) ) ;
#8349=CARTESIAN_POINT ( 'NONE',  ( 3.117629155811438402, -14.23119940253145188, 1.544136867890079090 ) ) ;
#8351=TOROIDAL_SURFACE ( 'NONE', #19229, 3.683000000000000718, 0.5080000000000000071 ) ;
#8352=B_SPLINE_CURVE_WITH_KNOTS ( 'NONE', 3,
 ( #10506, #29891, #14114, #26266, #36924, #20709, #40125, #36088, #10082, #4353, #23476, #729, #19871, #13706, #7322, #20281, #17314, #20492 ),
 .UNSPECIFIED., .F., .F.,
 ( 4, 2, 2, 2, 2, 2, 2, 2, 4 ),
 ( 0.000000000000000000, 0.0008271500248385261133, 0.001654300049677052227, 0.003308600099354083203, 0.004135750124192599450, 0.004962900149031114830, 0.006617200198708181151, 0.009925800298062312926, 0.01323440039741644383 ),
 .UNSPECIFIED. ) ;
#8354=CARTESIAN_POINT ( 'NONE',  ( -3.522755225739859775, -9.592572062075928940, 3.019445982675781348 ) ) ;
#8355=CARTESIAN_POINT ( 'NONE',  ( 16.72040787068447187, 146.6545634508490821, 1.779279871595184082 ) ) ;
#8356=CARTESIAN_POINT ( 'NONE',  ( 0.9447929531305513384, 34.22797915461067930, 2.226895425005813056 ) ) ;
#8357=CARTESIAN_POINT ( 'NONE',  ( -4.842864477130262912, 117.0601473006971105, 0.7870117353683143691 ) ) ;
#8359=CARTESIAN_POINT ( 'NONE',  ( -3.974385726840726107, -7.478117039488521023, -2.359557994316856533 ) ) ;
#8360=CARTESIAN_POINT ( 'NONE',  ( 1.569753016146328228, 156.2570369995211479, 0.1094014671735940580 ) ) ;
#8362=CARTESIAN_POINT ( 'NONE',  ( 8.423846519715326053, 3.801276092563157682, 0.04266398729441032295 ) ) ;
#8364=CARTESIAN_POINT ( 'NONE',  ( 8.771996676116902592, 117.8544088467123458, -0.2656499505225238256 ) ) ;
#8367=CARTESIAN_POINT ( 'NONE',  ( 1.834459164715509960, -15.41678468052755946, 5.387059099755639124 ) ) ;
#8369=CARTESIAN_POINT ( 'NONE',  ( 2.068261358883969780, 0.06400946394871305511, -8.190863557276260920 ) ) ;
#8370=CARTESIAN_POINT ( 'NONE',  ( 1.960761714621917395, 117.3993839177211242, 1.450045767418920883 ) ) ;
#8371=DIRECTION ( 'NONE',  ( 0.9998004120163608288, 5.205824365704082573E-17, 0.01997839162482749342 ) ) ;
#8372=CARTESIAN_POINT ( 'NONE',  ( 2.671714809844681238, -14.97371442308345380, 4.574436322856921144 ) ) ;
#8373=EDGE_CURVE ( 'NONE', #1213, #5065, #42155, .T. ) ;
#8374=CARTESIAN_POINT ( 'NONE',  ( 0.3585272760097797384, 113.0327356262573915, -2.615547676125327570 ) ) ;
#8375=CARTESIAN_POINT ( 'NONE',  ( -22.54544115201725063, 150.6069110094195764, 0.1392563518891846153 ) ) ;
#8377=CARTESIAN_POINT ( 'NONE',  ( -6.540718711769984318E-14, 75.78546620154573077, -7.235675496349066572E-18 ) ) ;
#8381=CARTESIAN_POINT ( 'NONE',  ( -5.953848250812766807, 121.5461441479843216, -0.08186234018733787310 ) ) ;
#8382=CARTESIAN_POINT ( 'NONE',  ( 5.416639188517969217, -15.16156180871851333, 2.817365454923381307 ) ) ;
#8383=CARTESIAN_POINT ( 'NONE',  ( -4.917623111643208311, 158.3981005702974016, 1.478962986009813685 ) ) ;
#8385=CARTESIAN_POINT ( 'NONE',  ( 22.19718911286642893, 149.5167998366165989, -0.9981983707184384214 ) ) ;
#8386=CARTESIAN_POINT ( 'NONE',  ( -0.5093740622119584671, 14.76157059199007016, 4.595130897425484306 ) ) ;
#8387=CARTESIAN_POINT ( 'NONE',  ( -5.807154922825684018, 117.0096406922080376, -0.3504623104576316539 ) ) ;
#8389=EDGE_CURVE ( 'NONE', #33842, #13325, #33143, .T. ) ;
#8391=CARTESIAN_POINT ( 'NONE',  ( 2.183572936211770177, 116.1951486486012470, 0.06351249239639800148 ) ) ;
#8393=CARTESIAN_POINT ( 'NONE',  ( -0.8914275061361285335, 157.0053619834820324, 1.381823885352171599 ) ) ;
#8395=CARTESIAN_POINT ( 'NONE',  ( 4.356286657365759929, 157.6046910967438066, -1.678189947947346994 ) ) ;
#8396=CARTESIAN_POINT ( 'NONE',  ( -21.26307135201312093, 148.5140355411650717, -2.311892396764663626 ) ) ;
#8398=VECTOR ( 'NONE', #6212, 1000.000000000000227 ) ;
#8399=CARTESIAN_POINT ( 'NONE',  ( 14.98735845036247127, 139.3652335140928074, -0.8263902896301492662 ) ) ;
#8402=CARTESIAN_POINT ( 'NONE',  ( -3.875499641586351629, 157.0187206368471209, -1.749001665105742731 ) ) ;
#8403=CARTESIAN_POINT ( 'NONE',  ( 4.521904862512733381, -15.32733325190937990, -0.1948396341466702986 ) ) ;
#8404=CARTESIAN_POINT ( 'NONE',  ( -4.397284644090289518, 118.1792272226432061, -0.5668491568854608920 ) ) ;
#8407=CARTESIAN_POINT ( 'NONE',  ( -4.804336728621736441, 117.5395540501120877, 0.9846445990501094814 ) ) ;
#8408=CARTESIAN_POINT ( 'NONE',  ( 12.92173176740947760, 125.9520529675768898, 1.821380522590920314 ) ) ;
#8410=CIRCLE ( 'NONE', #945, 3.175000000000001155 ) ;
#8412=CARTESIAN_POINT ( 'NONE',  ( -5.875566536072981627, -5.528788512802195854, 6.048791003748659634 ) ) ;
#8413=CARTESIAN_POINT ( 'NONE',  ( 12.12200908156748547, 130.5412724693565849, 0.6534646642625604462 ) ) ;
#8417=CARTESIAN_POINT ( 'NONE',  ( -1.627066591301449483, 117.3993836555909098, 1.397831962642635872 ) ) ;
#8422=CARTESIAN_POINT ( 'NONE',  ( -20.68286957925308656, 152.5754960671270055, -0.1900957434528338652 ) ) ;
#8425=CARTESIAN_POINT ( 'NONE',  ( -5.872192093296925819, 121.3219910589839685, -0.3926023243202280688 ) ) ;
#8426=CARTESIAN_POINT ( 'NONE',  ( -8.107080057029742548, 121.1657703571620885, 0.9663533087783954256 ) ) ;
#8428=EDGE_LOOP ( 'NONE', ( #13331, #23123, #8963, #10492 ) ) ;
#8429=CARTESIAN_POINT ( 'NONE',  ( 0.03519895179119666290, 115.7029491485446613, -1.761499482103947800 ) ) ;
#8430=CARTESIAN_POINT ( 'NONE',  ( -5.276193270648819933, 121.3253820001177417, -0.2225082926070588163 ) ) ;
#8431=CARTESIAN_POINT ( 'NONE',  ( 3.203739484688298500, -15.10556029324786032, 5.619401687775556375 ) ) ;
#8432=CARTESIAN_POINT ( 'NONE',  ( -16.82967018813389970, 125.2521365416322254, 1.031881933595589995 ) ) ;
#8433=CARTESIAN_POINT ( 'NONE',  ( 0.4298212797809583541, 117.3993833036163181, -1.480797141651997162 ) ) ;
#8434=CARTESIAN_POINT ( 'NONE',  ( 15.48069746188175166, 120.7065362441885981, 0.4134764081404143088 ) ) ;
#8435=CARTESIAN_POINT ( 'NONE',  ( 1.561582345843624431, 156.2588034088681184, 0.03120413162939523685 ) ) ;
#8437=CARTESIAN_POINT ( 'NONE',  ( -0.8918910426314872186, 22.31184809748591391, -0.3959014520797728975 ) ) ;
#8438=CARTESIAN_POINT ( 'NONE',  ( -23.33940156856683856, 149.0646716566344026, -0.5435133253920597651 ) ) ;
#8442=CARTESIAN_POINT ( 'NONE',  ( -4.116559577307818962, 118.3381180974515274, 0.8321499372237044501 ) ) ;
#8443=CARTESIAN_POINT ( 'NONE',  ( -5.322367322403097845, 105.1224774134945790, 0.3643359423292727994 ) ) ;
#8444=CARTESIAN_POINT ( 'NONE',  ( 14.08892660837130606, 121.3807765770047666, 1.491720297716245369 ) ) ;
#8446=CARTESIAN_POINT ( 'NONE',  ( 16.05265579080195337, 153.3736753708079732, -1.680156470693514814 ) ) ;
#8448=CARTESIAN_POINT ( 'NONE',  ( -1.404924415901314561, -12.60368214249519703, -4.422195601339041993 ) ) ;
#8449=CARTESIAN_POINT ( 'NONE',  ( -14.92730792698330866, 121.5307057168427605, -1.330945954902034822 ) ) ;
#8450=CARTESIAN_POINT ( 'NONE',  ( 4.877181834135257965, 117.6443843650974088, -0.8852099847017325107 ) ) ;
#8451=CARTESIAN_POINT ( 'NONE',  ( 6.711594774621037374, 121.2247800624193133, 0.3423702293131484775 ) ) ;
#8453=EDGE_CURVE ( 'NONE', #9800, #29150, #13954, .T. ) ;
#8454=CARTESIAN_POINT ( 'NONE',  ( -13.59948517815245772, 150.2262467139961473, -0.1464537565166197652 ) ) ;
#8455=CARTESIAN_POINT ( 'NONE',  ( -13.13949684203677570, 123.8872625266795211, -1.904607404193280340 ) ) ;
#8456=CARTESIAN_POINT ( 'NONE',  ( 2.291706021380962355, -15.53059561260056221, 5.887745402940570472 ) ) ;
#8460=CARTESIAN_POINT ( 'NONE',  ( -3.903555647324534306, 118.1651005205136897, -0.7209690768601634270 ) ) ;
#8462=CARTESIAN_POINT ( 'NONE',  ( 8.504430935371811273, 120.5511696877957775, 1.462663580662433294 ) ) ;
#8464=EDGE_CURVE ( 'NONE', #3752, #32528, #576, .T. ) ;
#8465=CARTESIAN_POINT ( 'NONE',  ( -3.844008814211067993, 118.0218828919481098, -0.9706315391978014295 ) ) ;
#8467=CARTESIAN_POINT ( 'NONE',  ( -1.590100404673132184, 118.0223913815010377, 0.9765506547304494411 ) ) ;
#8469=CARTESIAN_POINT ( 'NONE',  ( -8.417729735924666556, -0.9468307554896212563, 0.2322036382352700989 ) ) ;
#8470=CARTESIAN_POINT ( 'NONE',  ( 10.42685857375358260, 124.8149993102252182, 1.042337215157124186 ) ) ;
#8471=CARTESIAN_POINT ( 'NONE',  ( -5.240921474315769046, 115.6909491485453003, -1.017345001637511404 ) ) ;
#8472=CARTESIAN_POINT ( 'NONE',  ( 21.63859276624132377, 151.3813297165527274, -0.4067934712883240489 ) ) ;
#8477=CARTESIAN_POINT ( 'NONE',  ( -4.158717781106146205, 118.2391784042057026, 0.2328764324043287315 ) ) ;
#8481=CARTESIAN_POINT ( 'NONE',  ( 8.322108986833429256, 120.1313932179692330, -1.118147983713804194 ) ) ;
#8482=CARTESIAN_POINT ( 'NONE',  ( -0.1524052867847605630, 105.8811906981200934, -5.339394923009169958 ) ) ;
#8483=CARTESIAN_POINT ( 'NONE',  ( 4.345256946659891817, 118.1827420971760887, 0.6195611995493047752 ) ) ;
#8484=CARTESIAN_POINT ( 'NONE',  ( -9.732298487430798062, 124.2227999206177032, -0.8093454005834662679 ) ) ;
#8485=CARTESIAN_POINT ( 'NONE',  ( 4.854908608518735846, 117.4053607954329976, -1.004341486598190558 ) ) ;
#8487=EDGE_LOOP ( 'NONE', ( #39478, #10384, #17593, #18008, #36861 ) ) ;
#8488=CARTESIAN_POINT ( 'NONE',  ( 0.2838385327444274964, 29.22985346960623332, -4.617364983570896086 ) ) ;
#8492=CARTESIAN_POINT ( 'NONE',  ( 6.075699028729387052, 121.3938335755924243, 0.3948700328016164218 ) ) ;
#8493=CARTESIAN_POINT ( 'NONE',  ( 3.707542801486926276, 23.89195667223011910, -2.776928957275885068 ) ) ;
#8494=CARTESIAN_POINT ( 'NONE',  ( 22.70140800483388688, 148.7873826295267747, 1.635989027091525161 ) ) ;
#8496=CARTESIAN_POINT ( 'NONE',  ( 3.047145566129288330, -14.72663143740328806, 3.823360744794035870 ) ) ;
#8497=CARTESIAN_POINT ( 'NONE',  ( 11.93281433870457775, 156.4809912657682673, -1.479000486392926916 ) ) ;
#8498=CARTESIAN_POINT ( 'NONE',  ( -18.43358770356691068, 147.0160646422468744, 1.663356549802410989 ) ) ;
#8499=CARTESIAN_POINT ( 'NONE',  ( -2.133573495637306916, 19.78131850274109382, 4.120466288703205748 ) ) ;
#8500=CARTESIAN_POINT ( 'NONE',  ( -18.33253411489134876, 154.1536317137893661, -1.165609363665846221 ) ) ;
#8501=CARTESIAN_POINT ( 'NONE',  ( 0.5691593726700751033, 20.64373787749807576, 0.7897743370290384313 ) ) ;
#8504=CARTESIAN_POINT ( 'NONE',  ( -12.53742732955040395, 130.7145975665201831, 0.5304871790577964097 ) ) ;
#8505=CARTESIAN_POINT ( 'NONE',  ( 4.077043646397369159, -14.32506836492906999, 4.807529146363894057 ) ) ;
#8506=CARTESIAN_POINT ( 'NONE',  ( 13.27577938203601526, 128.5100244389050204, -1.209575533060949892 ) ) ;
#8508=CARTESIAN_POINT ( 'NONE',  ( 2.225394578381316268, 115.7029491485453150, 1.707871263558881969 ) ) ;
#8510=CARTESIAN_POINT ( 'NONE',  ( 3.188489192988832155, -14.31930622237681483, 3.473944028487384372 ) ) ;
#8511=CARTESIAN_POINT ( 'NONE',  ( -4.691900465594415870, 117.8976975978048642, -0.9735392405797208548 ) ) ;
#8512=CARTESIAN_POINT ( 'NONE',  ( 3.751144962740032618, 121.0949217282140182, 0.04819499160668145460 ) ) ;
#8513=ORIENTED_EDGE ( 'NONE', *, *, #33182, .T. ) ;
#8514=CARTESIAN_POINT ( 'NONE',  ( 19.69933843609242530, 149.7343351798865285, 2.455316921491699667 ) ) ;
#8515=LINE ( 'NONE', #27887, #10887 ) ;
#8516=DIRECTION ( 'NONE',  ( -0.9998004120163608288, 0.000000000000000000, -0.01997839162482749342 ) ) ;
#8518=CARTESIAN_POINT ( 'NONE',  ( 0.03153862713803012863, 157.4657262375360176, -1.578321868909182246 ) ) ;
#8519=CARTESIAN_POINT ( 'NONE',  ( 1.411700740068499993, 159.5982469381528972, -0.1593474270858732111 ) ) ;
#8521=CARTESIAN_POINT ( 'NONE',  ( 1.760709524605698961, -15.18916190965080659, 5.866327383715185917 ) ) ;
#8524=CARTESIAN_POINT ( 'NONE',  ( -4.894527635837473412, 117.7423471277129607, 0.7194462064511487620 ) ) ;
#8529=CARTESIAN_POINT ( 'NONE',  ( -2.865660977700466017, 118.0055230577426073, -0.8541496112950387465 ) ) ;
#8530=CARTESIAN_POINT ( 'NONE',  ( -4.807558371750645598, 117.0601473006971105, -0.9798501506189060128 ) ) ;
#8531=CARTESIAN_POINT ( 'NONE',  ( 4.909831060657428026, 117.4773178990584483, 1.095440290055193389 ) ) ;
#8533=CARTESIAN_POINT ( 'NONE',  ( -0.8223074630897415638, 121.2007779179981384, 0.3881979734473210431 ) ) ;
#8534=CARTESIAN_POINT ( 'NONE',  ( 4.529186081025091681, -11.15152372915077095, -0.9203776863585164669 ) ) ;
#8536=DIRECTION ( 'NONE',  ( -4.017660918040594346E-17, 1.000000000000000000, 2.376309959284834438E-19 ) ) ;
#8537=CARTESIAN_POINT ( 'NONE',  ( 3.214659515886821861, -12.19625089790456229, 0.4983212145216010525 ) ) ;
#8538=CARTESIAN_POINT ( 'NONE',  ( 6.675377558974045833, 121.2389289720308199, -0.07470202506228480754 ) ) ;
#8539=CARTESIAN_POINT ( 'NONE',  ( 6.076994399821980863, 121.4412224314809521, 0.1214066477987181120 ) ) ;
#8540=CARTESIAN_POINT ( 'NONE',  ( -5.361994333976945803, 30.20544108279508677, 3.344879823269458985 ) ) ;
#8542=CARTESIAN_POINT ( 'NONE',  ( -0.7578723423243420854, 115.7030198846401134, 1.728701198025235364 ) ) ;
#8543=CARTESIAN_POINT ( 'NONE',  ( -2.136650056307613621, 10.86338872207680950, -4.114640003288728920 ) ) ;
#8544=CARTESIAN_POINT ( 'NONE',  ( 23.18613385382694503, 148.9919839608952827, 1.059503902452021640 ) ) ;
#8545=EDGE_LOOP ( 'NONE', ( #15802, #37512, #23781, #12479 ) ) ;
#8546=CARTESIAN_POINT ( 'NONE',  ( 5.024936854470411163, 105.1216725936605201, -1.825215542048775674 ) ) ;
#8547=CARTESIAN_POINT ( 'NONE',  ( 2.631420558634286255, -15.64638348417481062, 4.926794133592228064 ) ) ;
#8548=CARTESIAN_POINT ( 'NONE',  ( -2.301458206243153892, 118.5910164976458532, 0.7067537174111425680 ) ) ;
#8549=CARTESIAN_POINT ( 'NONE',  ( -0.9107729336552147226, 17.84451472381387305, 0.3451692354151053577 ) ) ;
#8550=CARTESIAN_POINT ( 'NONE',  ( -0.8615061033338488050, 12.60145565637890286, -0.4637196408544374537 ) ) ;
#8551=EDGE_LOOP ( 'NONE', ( #32545, #28515, #21808 ) ) ;
#8554=CARTESIAN_POINT ( 'NONE',  ( 3.315491766441247101, 124.7872298565087021, 0.07248898146901455730 ) ) ;
#8556=CARTESIAN_POINT ( 'NONE',  ( -13.46182233857078536, 130.9706359334022920, 1.049250031952806861 ) ) ;
#8557=DIRECTION ( 'NONE',  ( -4.017660918040594346E-17, 1.000000000000000000, 2.376309959284834438E-19 ) ) ;
#8558=CARTESIAN_POINT ( 'NONE',  ( 2.265044067826554652, -14.95788512594138631, 5.210342366881125287 ) ) ;
#8559=CARTESIAN_POINT ( 'NONE',  ( 18.15383854178424272, 147.5382818419693649, -1.618175512470155120 ) ) ;
#8560=CARTESIAN_POINT ( 'NONE',  ( -12.21120734956430809, 121.7247091083657153, -1.742548127100890243 ) ) ;
#8562=CARTESIAN_POINT ( 'NONE',  ( -6.442297258278467886, 29.65178619621697464, 0.8020365093557801917 ) ) ;
#8563=CARTESIAN_POINT ( 'NONE',  ( 9.242439611670231869, 123.9961275534082148, -0.1349267066575718654 ) ) ;
#8565=CARTESIAN_POINT ( 'NONE',  ( 2.568134854143032442, -15.02010252187911554, 4.714990346623905815 ) ) ;
#8569=CARTESIAN_POINT ( 'NONE',  ( 3.417104117279694098, -14.34023910220586906, -3.129441506049576383 ) ) ;
#8570=CARTESIAN_POINT ( 'NONE',  ( 16.94675455810613229, 147.0740084267719396, 1.925552282123431436 ) ) ;
#8571=CARTESIAN_POINT ( 'NONE',  ( 2.887677632297840802, 37.80609079512323234, 0.7577488597010552107 ) ) ;
#8572=CARTESIAN_POINT ( 'NONE',  ( -7.588858076165209354, 124.2943531750336490, -0.1426133663090954629 ) ) ;
#8573=CARTESIAN_POINT ( 'NONE',  ( 0.05711764529616595448, 0.5181683540770932739, -4.631227783250111862 ) ) ;
#8574=CARTESIAN_POINT ( 'NONE',  ( -0.0005468344959659662699, 156.3034662015456604, 0.02736583427618497280 ) ) ;
#8575=CARTESIAN_POINT ( 'NONE',  ( 4.050812540078617019, -7.421221357003889629, 7.384888961799156881 ) ) ;
#8577=CARTESIAN_POINT ( 'NONE',  ( 2.159899147946715114, 116.3864810981202851, -0.2326697378273381023 ) ) ;
#8578=CARTESIAN_POINT ( 'NONE',  ( -0.3665064675492638036, 121.9236798544226730, -0.3444762419765420303 ) ) ;
#8581=CARTESIAN_POINT ( 'NONE',  ( 4.622858883031034871, 26.85595184169372374, 0.2084198311932836112 ) ) ;
#8585=CARTESIAN_POINT ( 'NONE',  ( 0.1065646865914871289, 105.8844662015457203, -5.332932678536313809 ) ) ;
#8586=CARTESIAN_POINT ( 'NONE',  ( -19.95587765737807828, 128.8226523212408949, 0.2284701554834995540 ) ) ;
#8589=VERTEX_POINT ( 'NONE', #10130 ) ;
#8590=DIRECTION ( 'NONE',  ( 0.9998004120163609398, 4.016384292689130894E-17, 0.01997839162482749689 ) ) ;
#8591=CARTESIAN_POINT ( 'NONE',  ( -9.104209967888042598, 153.9432936505793066, -0.1819237819739442652 ) ) ;
#8592=CARTESIAN_POINT ( 'NONE',  ( 3.829091000068871598, -15.41100336169511031, 5.152250049158875633 ) ) ;
#8593=CARTESIAN_POINT ( 'NONE',  ( -13.79335258734193914, 122.1113760975138263, 1.168436778447113689 ) ) ;
#8594=CARTESIAN_POINT ( 'NONE',  ( 0.01645572339161061742, 159.4324016994384010, -0.8235116888278192215 ) ) ;
#8595=CARTESIAN_POINT ( 'NONE',  ( -4.603678009535974169, 12.38766144714272066, -0.4343361176327051321 ) ) ;
#8597=CARTESIAN_POINT ( 'NONE',  ( -3.781797959329980863, 116.7736770086926867, -0.3417761088697101601 ) ) ;
#8600=CARTESIAN_POINT ( 'NONE',  ( -2.183475033498248230, 116.1883682894288796, -0.03369517848931347787 ) ) ;
#8602=CARTESIAN_POINT ( 'NONE',  ( -11.26369337785518709, 123.4744472594011739, 1.139971239082961052 ) ) ;
#8605=CARTESIAN_POINT ( 'NONE',  ( 19.29133405012190750, 147.6776069388173767, -1.737063910747457030 ) ) ;
#8606=CARTESIAN_POINT ( 'NONE',  ( -21.19397400757792482, 145.8710773725474610, -2.320968965272669937 ) ) ;
#8608=CARTESIAN_POINT ( 'NONE',  ( 9.599121003648848571, 153.9312916436033447, -0.7969471826422132033 ) ) ;
#8609=ORIENTED_EDGE ( 'NONE', *, *, #7707, .F. ) ;
#8610=CARTESIAN_POINT ( 'NONE',  ( -17.59644933020973667, 144.4767212251450417, -2.299577266864829994 ) ) ;
#8611=CARTESIAN_POINT ( 'NONE',  ( 3.857521300888583582, -15.67877420849868386, 3.673684628067402702 ) ) ;
#8612=CARTESIAN_POINT ( 'NONE',  ( -4.065972646788793554, 118.2429491485453070, -0.3080848862740693250 ) ) ;
#8616=CARTESIAN_POINT ( 'NONE',  ( -4.987820457167934762, 117.4712984309037438, 0.8194575654087326022 ) ) ;
#8617=CARTESIAN_POINT ( 'NONE',  ( 2.063908814988649532, 157.0334531201187644, 1.539797002863053210 ) ) ;
#8618=DIRECTION ( 'NONE',  ( -5.206863593109713045E-17, 1.000000000000000000, -1.077750396879097359E-30 ) ) ;
#8619=CARTESIAN_POINT ( 'NONE',  ( -3.210878647048973189, -8.553304832117262890, -7.794174491370510438 ) ) ;
#8620=CARTESIAN_POINT ( 'NONE',  ( 6.044022022451693843, 155.3491655920357459, 0.4731370799734938015 ) ) ;
#8623=ORIENTED_EDGE ( 'NONE', *, *, #38592, .F. ) ;
#8624=CARTESIAN_POINT ( 'NONE',  ( -4.862565162136183616, 117.4116260025058693, -1.165543200563879056 ) ) ;
#8625=CARTESIAN_POINT ( 'NONE',  ( -7.836093358135542530, 122.3276016517421994, -0.6978168763808364483 ) ) ;
#8628=CARTESIAN_POINT ( 'NONE',  ( -23.28495812418893607, 149.3453998935430604, -0.3112269551726869476 ) ) ;
#8632=CARTESIAN_POINT ( 'NONE',  ( -7.841358516840601034, 122.2961712410880324, -0.7253305154435645274 ) ) ;
#8633=CARTESIAN_POINT ( 'NONE',  ( -8.262035544818829180, 120.4240392771559414, 1.115000201712872618 ) ) ;
#8634=ORIENTED_EDGE ( 'NONE', *, *, #18492, .T. ) ;
#8636=CARTESIAN_POINT ( 'NONE',  ( -13.02783148976621774, 133.9378623523624299, -0.5757418746946230126 ) ) ;
#8637=CARTESIAN_POINT ( 'NONE',  ( 4.896986379477733742, -14.09362661677580952, 4.057159877996594055 ) ) ;
#8638=CARTESIAN_POINT ( 'NONE',  ( -7.994725381675435116, 118.4344479264803169, 0.7928399906090751736 ) ) ;
#8640=DIRECTION ( 'NONE',  ( -4.017660918040594346E-17, 1.000000000000000000, 2.376309959284834438E-19 ) ) ;
#8641=CARTESIAN_POINT ( 'NONE',  ( 22.97436839085978733, 150.1579452496398801, 0.6125673049107098755 ) ) ;
#8642=TOROIDAL_SURFACE ( 'NONE', #19510, 4.826000000000000512, 0.5080000000000000071 ) ;
#8643=CARTESIAN_POINT ( 'NONE',  ( 9.126830667405478437, 124.2274448616014411, 0.2272647324663854829 ) ) ;
#8644=CARTESIAN_POINT ( 'NONE',  ( -4.903827551164339660, 117.7626876103193325, 0.5344712183346053136 ) ) ;
#8645=CARTESIAN_POINT ( 'NONE',  ( 0.7580923926444932404, 28.79380631387826028, -0.6184068814828035388 ) ) ;
#8647=CARTESIAN_POINT ( 'NONE',  ( -23.21042342040066231, 149.6290410902582551, -0.5408589295980601452 ) ) ;
#8651=CARTESIAN_POINT ( 'NONE',  ( 8.283808458469433589, 120.0678368811737755, 1.450790680561929280 ) ) ;
#8652=LINE ( 'NONE', #41246, #27933 ) ;
#8653=CARTESIAN_POINT ( 'NONE',  ( 19.72970310060704335, 132.0165317526581816, 1.843001364771305939 ) ) ;
#8654=AXIS2_PLACEMENT_3D ( 'NONE', #32729, #39118, #154 ) ;
#8655=CARTESIAN_POINT ( 'NONE',  ( 4.992797058274879518, 118.5534682650580862, -0.8674252695128576995 ) ) ;
#8656=CARTESIAN_POINT ( 'NONE',  ( -4.326994387844902867, 19.77997674669536465, 7.266063235268683584 ) ) ;
#8657=CARTESIAN_POINT ( 'NONE',  ( -22.23208127788764443, 149.2301036976659816, -1.887777678714757768 ) ) ;
#8658=CARTESIAN_POINT ( 'NONE',  ( 4.907634972350170877, 117.7148210790128360, -0.7337193700908156702 ) ) ;
#8659=CARTESIAN_POINT ( 'NONE',  ( 5.011858831344538245, 114.3657942991566472, 1.958205155698268696 ) ) ;
#8660=ORIENTED_EDGE ( 'NONE', *, *, #18578, .T. ) ;
#8662=CARTESIAN_POINT ( 'NONE',  ( -9.001127587916252892, 123.9218113011205986, -0.09563458650452036358 ) ) ;
#8663=CARTESIAN_POINT ( 'NONE',  ( -13.10180873912566035, 153.9517556018257096, -2.260155593826742582 ) ) ;
#8664=CARTESIAN_POINT ( 'NONE',  ( 5.095505811086057157, -15.28584205578724386, 3.479711806413861908 ) ) ;
#8666=CARTESIAN_POINT ( 'NONE',  ( -0.6964149855636846409, 117.3993842960376099, -1.488886793157482957 ) ) ;
#8668=CARTESIAN_POINT ( 'NONE',  ( 18.59210649535962290, 147.7499600834086948, 2.443498639627972313 ) ) ;
#8670=CARTESIAN_POINT ( 'NONE',  ( 4.756814333351318425, 117.4032681585794791, 1.206529664789174339 ) ) ;
#8672=CARTESIAN_POINT ( 'NONE',  ( -0.3374525697216100295, 106.5118632461160217, 5.070939582669566903 ) ) ;
#8673=CARTESIAN_POINT ( 'NONE',  ( -5.378050908718009282, 0.3500678860072145016, 6.480130142454380682 ) ) ;
#8674=CARTESIAN_POINT ( 'NONE',  ( 9.619667158014634012, 123.8920215319950842, 0.8772578247576550137 ) ) ;
#8676=EDGE_CURVE ( 'NONE', #41701, #2340, #5433, .T. ) ;
#8677=CARTESIAN_POINT ( 'NONE',  ( 5.566083668711077515, 159.0643023895801491, -0.5661052595122396669 ) ) ;
#8681=CARTESIAN_POINT ( 'NONE',  ( -4.118105137886063360, 118.2429491485453354, 0.1865571212249754751 ) ) ;
#8682=CARTESIAN_POINT ( 'NONE',  ( -23.29144772315980916, 149.3526176766912101, -0.4654185560736369132 ) ) ;
#8685=EDGE_CURVE ( 'NONE', #12906, #16433, #11712, .T. ) ;
#8687=CARTESIAN_POINT ( 'NONE',  ( -6.268960521413761811, 119.8969868274346027, -1.221708021102049901 ) ) ;
#8688=CARTESIAN_POINT ( 'NONE',  ( -5.336420303164543633, 104.6144662015457101, 0.06783417913549341649 ) ) ;
#8689=CARTESIAN_POINT ( 'NONE',  ( -9.371428955827290963, 153.8930958044198576, -0.9350090023289892027 ) ) ;
#8691=CARTESIAN_POINT ( 'NONE',  ( 16.18905205736044906, 121.2598130428683447, 0.3234957879086921562 ) ) ;
#8693=CARTESIAN_POINT ( 'NONE',  ( -0.1328416520900886078, 24.48205809745167372, 4.627450821846854190 ) ) ;
#8695=CARTESIAN_POINT ( 'NONE',  ( -5.078986093043185157, 66.13346620154574396, -0.1014902294541238092 ) ) ;
#8697=DIRECTION ( 'NONE',  ( 0.01997839162482749689, 1.040247600000945640E-18, -0.9998004120163610509 ) ) ;
#8698=CARTESIAN_POINT ( 'NONE',  ( 6.990876450665549413, 121.9332825538419200, 0.2917046836452048542 ) ) ;
#8699=EDGE_CURVE ( 'NONE', #28106, #5804, #17662, .T. ) ;
#8701=CARTESIAN_POINT ( 'NONE',  ( 1.336693583852395673, 159.4956652290339605, 0.6991310044172547311 ) ) ;
#8702=CARTESIAN_POINT ( 'NONE',  ( -4.694219104381005536, 104.6144662015457953, -1.165030450612820623 ) ) ;
#8703=CARTESIAN_POINT ( 'NONE',  ( 3.186936940905604754, -14.67134942876716153, 3.163583609075255598 ) ) ;
#8704=CARTESIAN_POINT ( 'NONE',  ( 13.10001109591386559, 121.1598417376693533, -1.052633080380691144 ) ) ;
#8705=CARTESIAN_POINT ( 'NONE',  ( -7.718355369771888519, 156.1362479297160348, 1.656311413603696936 ) ) ;
#8706=CARTESIAN_POINT ( 'NONE',  ( -0.1338072975148606736, -13.68656151007796495, -0.9662261747338762863 ) ) ;
#8707=CARTESIAN_POINT ( 'NONE',  ( -8.135778112230864778, 117.7673425867732249, -0.7050676646501271572 ) ) ;
#8710=CARTESIAN_POINT ( 'NONE',  ( -0.3421040304481134942, 19.14286131909006272, 0.9136164113388466346 ) ) ;
#8713=CARTESIAN_POINT ( 'NONE',  ( -8.002172173406888689, 154.6030710842251494, 0.4507127070663228263 ) ) ;
#8714=CARTESIAN_POINT ( 'NONE',  ( 5.820712434538892310, -12.64545009755467575, 1.387492028720230364 ) ) ;
#8715=CARTESIAN_POINT ( 'NONE',  ( 6.842818979164380089, 155.5980657034081105, -1.215443052661050460 ) ) ;
#8717=CARTESIAN_POINT ( 'NONE',  ( 0.6864031510614769793, 115.7029491485453576, 1.757686897103055923 ) ) ;
#8718=CARTESIAN_POINT ( 'NONE',  ( -4.742366482708093578, 117.6343161886170208, -1.141804636843513965 ) ) ;
#8719=CARTESIAN_POINT ( 'NONE',  ( 12.91960671971514252, 133.8340822528099636, 0.1412842392263899960 ) ) ;
#8722=CARTESIAN_POINT ( 'NONE',  ( -0.01147819631913261050, 118.5605975114896609, 0.5744158801423953076 ) ) ;
#8723=DIRECTION ( 'NONE',  ( -5.206863593109713661E-17, 1.000000000000000000, -1.077750396879097183E-30 ) ) ;
#8725=CARTESIAN_POINT ( 'NONE',  ( 0.02156508032615568615, 159.2730288250082538, -1.079204802879467406 ) ) ;
#8726=CARTESIAN_POINT ( 'NONE',  ( 23.31467963135034438, 142.7201128741078833, 0.1336249016415858304 ) ) ;
#8729=CARTESIAN_POINT ( 'NONE',  ( 1.801801447854238569, -15.42219197509341022, 5.395122923460818676 ) ) ;
#8731=CARTESIAN_POINT ( 'NONE',  ( -6.564189886853176475E-14, 81.62746620154572952, -5.847435218134868453E-18 ) ) ;
#8732=EDGE_CURVE ( 'NONE', #11424, #4990, #93, .T. ) ;
#8733=CARTESIAN_POINT ( 'NONE',  ( -4.662673704711017386, 117.9838541597224406, 0.7073371538211529197 ) ) ;
#8735=ORIENTED_EDGE ( 'NONE', *, *, #21417, .T. ) ;
#8737=CARTESIAN_POINT ( 'NONE',  ( -5.968544434436104299E-14, 66.13346620154574396, 9.705588791358230112E-17 ) ) ;
#8738=CARTESIAN_POINT ( 'NONE',  ( -8.527069590570199864, 118.9013125089547600, -1.248037646211100249 ) ) ;
#8739=CARTESIAN_POINT ( 'NONE',  ( -4.183818394377370353, 118.4033805524614849, -0.7412457532797813720 ) ) ;
#8740=CARTESIAN_POINT ( 'NONE',  ( 4.859669866895486301, 117.7242276672350272, 0.9631597096148959425 ) ) ;
#8742=CARTESIAN_POINT ( 'NONE',  ( -0.07157677169895493297, 110.3683645023726569, 3.581994345755985076 ) ) ;
#8744=CARTESIAN_POINT ( 'NONE',  ( 5.005702202344075147, 117.4009237673399610, -0.7895530272732956822 ) ) ;
#8746=CARTESIAN_POINT ( 'NONE',  ( 3.427377709871179512, -13.85078959623727002, 3.379007147668904754 ) ) ;
#8747=CARTESIAN_POINT ( 'NONE',  ( 6.300951452924033802, 121.9812576474260055, -0.03014847038595253048 ) ) ;
#8748=CARTESIAN_POINT ( 'NONE',  ( -10.53370020345052893, 154.2769816202975051, -1.888232850154634823 ) ) ;
#8749=CARTESIAN_POINT ( 'NONE',  ( -7.785932599179138158, 122.6147803075941454, -0.2294614199791660536 ) ) ;
#8750=CARTESIAN_POINT ( 'NONE',  ( -2.169500164636429140, 35.42160933236649356, 3.123960633263313635 ) ) ;
#8751=CARTESIAN_POINT ( 'NONE',  ( -0.2889451677547653641, 115.7029882247660879, 1.754375496046200578 ) ) ;
#8752=CARTESIAN_POINT ( 'NONE',  ( 4.617411384770501392, 7.639850289152962048, 0.2838591255797697777 ) ) ;
#8753=CARTESIAN_POINT ( 'NONE',  ( -0.006534887713674795984, 159.5822087645323393, 0.3270325034788581497 ) ) ;
#8755=CARTESIAN_POINT ( 'NONE',  ( 4.270891071783644577, 105.1220196924935237, -3.200937537902331709 ) ) ;
#8756=CARTESIAN_POINT ( 'NONE',  ( 2.294714809908028119, -15.51018114022951977, 5.078884642465592236 ) ) ;
#8757=CARTESIAN_POINT ( 'NONE',  ( -9.796729639280952640, 120.9522862504114897, 1.196371290339073079 ) ) ;
#8759=CARTESIAN_POINT ( 'NONE',  ( 0.9476013557874021220, 22.48150014755712078, -0.2491751695904415032 ) ) ;
#8760=ADVANCED_FACE ( 'NONE', ( #2613, #15147 ), #37168, .F. ) ;
#8761=CARTESIAN_POINT ( 'NONE',  ( -0.5883093083485460006, 14.76436220226899465, 0.7776626239079347247 ) ) ;
#8762=ORIENTED_EDGE ( 'NONE', *, *, #21447, .F. ) ;
#8765=CARTESIAN_POINT ( 'NONE',  ( 3.009276887026298031, 39.20946620154573736, -1.210121013456480599 ) ) ;
#8766=CARTESIAN_POINT ( 'NONE',  ( 2.972890788444304988, 110.6400929099055332, 3.409217096083849263 ) ) ;
#8768=CARTESIAN_POINT ( 'NONE',  ( -16.24447748055638385, 147.7868695473139553, 0.9462090312511077794 ) ) ;
#8770=( BOUNDED_CURVE ( )  B_SPLINE_CURVE ( 3, ( #36657, #37076, #40692, #1303 ),
 .UNSPECIFIED., .F., .T. ) 
 B_SPLINE_CURVE_WITH_KNOTS ( ( 4, 4 ),
 ( 0.5508374472049354376, 0.6038647612415126709 ),
 .UNSPECIFIED. ) 
 CURVE ( )  GEOMETRIC_REPRESENTATION_ITEM ( )  RATIONAL_B_SPLINE_CURVE ( ( 0.8173257794870510962, 0.7610001515862588883, 0.7121729131092952025, 0.6708440640561601498 ) ) 
 REPRESENTATION_ITEM ( '' )  );
#8771=CARTESIAN_POINT ( 'NONE',  ( 3.513860297840244673, -13.27766151250851756, 2.382095677556017588 ) ) ;
#8772=CARTESIAN_POINT ( 'NONE',  ( 16.98902716506006882, 149.6223975874448229, -1.623990461445592892 ) ) ;
#8773=CARTESIAN_POINT ( 'NONE',  ( -8.895965109948988925, 157.0267672960688969, -2.032209471265452816 ) ) ;
#8775=CARTESIAN_POINT ( 'NONE',  ( -11.03183784343237583, 128.0124916018596650, -0.2204423744267033636 ) ) ;
#8776=CARTESIAN_POINT ( 'NONE',  ( -6.203946039754976383, 30.82792567283054552, 2.070158528702760403 ) ) ;
#8777=CARTESIAN_POINT ( 'NONE',  ( 11.48476400923499341, 128.2561452373498980, -0.2810130423614016770 ) ) ;
#8779=CARTESIAN_POINT ( 'NONE',  ( 3.130567944924658175, -14.75736435017342707, 3.480214150758962788 ) ) ;
#8785=CARTESIAN_POINT ( 'NONE',  ( -2.900346660479264482, -2.445871450894649968, -3.618988008572288972 ) ) ;
#8786=CARTESIAN_POINT ( 'NONE',  ( 16.40533521683933316, 148.4304801786341272, 1.905158959863711310 ) ) ;
#8787=CARTESIAN_POINT ( 'NONE',  ( -6.552838421881942555E-14, 85.18346620154574111, 1.207165459533130484E-19 ) ) ;
#8788=CARTESIAN_POINT ( 'NONE',  ( -0.1065646865916158176, 105.8844662015456919, 5.332932678536313809 ) ) ;
#8789=CARTESIAN_POINT ( 'NONE',  ( -3.832284926465886254, -5.753926550059754064, 2.584458424559757272 ) ) ;
#8790=CARTESIAN_POINT ( 'NONE',  ( 0.6407465451153555591, 156.3034662015456888, 0.04018040219424109244 ) ) ;
#8791=CARTESIAN_POINT ( 'NONE',  ( -7.766292583485225443, -1.596223907437250844, -3.263082884517814364 ) ) ;
#8793=CARTESIAN_POINT ( 'NONE',  ( -5.502499940525628297, 117.0098869289899142, -0.6785148692947098326 ) ) ;
#8794=CARTESIAN_POINT ( 'NONE',  ( 0.07931638298543132459, 106.1822392402443143, -5.212590348647615279 ) ) ;
#8795=CARTESIAN_POINT ( 'NONE',  ( -6.505112547751767921E-14, 75.78546620154573077, -1.207165459009924652E-19 ) ) ;
#8796=CARTESIAN_POINT ( 'NONE',  ( -1.386537629721184883, 36.36735770096321829, 2.585368322340788172 ) ) ;
#8797=CARTESIAN_POINT ( 'NONE',  ( -1.648064503646425649, 29.87956589480163316, -4.325937074807028715 ) ) ;
#8798=CARTESIAN_POINT ( 'NONE',  ( 1.083433792273709839, 117.9394488523357580, 1.391098255892824653 ) ) ;
#8801=CARTESIAN_POINT ( 'NONE',  ( 0.3981704103449270060, 123.4679809879532542, -0.1459118279324086442 ) ) ;
#8802=CARTESIAN_POINT ( 'NONE',  ( -16.66487874612770881, 155.2617138006751532, 0.3247879035468689835 ) ) ;
#8806=VERTEX_POINT ( 'NONE', #41585 ) ;
#8808=CARTESIAN_POINT ( 'NONE',  ( -4.211726112319180260, 155.8650792863299159, -0.03635988582397711028 ) ) ;
#8809=CARTESIAN_POINT ( 'NONE',  ( 3.194259428633707376, -15.59200274161393018, 5.439406988142795107 ) ) ;
#8810=CARTESIAN_POINT ( 'NONE',  ( -18.27466214341559336, 151.8090458617612057, 1.628071726616033610 ) ) ;
#8811=CARTESIAN_POINT ( 'NONE',  ( 18.64118049546047118, 128.6297099747515347, -0.9949054493987050662 ) ) ;
#8812=CARTESIAN_POINT ( 'NONE',  ( 4.573446973487649281, 17.56025517495590904, -0.6989348988664985107 ) ) ;
#8813=CARTESIAN_POINT ( 'NONE',  ( -22.58226468115107011, 150.6256779753201158, -0.9011697351191819694 ) ) ;
#8816=CARTESIAN_POINT ( 'NONE',  ( 8.790925543711857415, 117.7045849823074946, 0.3245846052679721705 ) ) ;
#8818=CARTESIAN_POINT ( 'NONE',  ( -5.120154531940317000, 120.2090573957402455, 0.7231840875875846786 ) ) ;
#8820=CARTESIAN_POINT ( 'NONE',  ( 2.359155998022406830, 118.9063233352275972, -0.7056007782052503563 ) ) ;
#8821=CARTESIAN_POINT ( 'NONE',  ( -14.79112219052239752, 123.2524255416106342, -1.763561952744265859 ) ) ;
#8823=CARTESIAN_POINT ( 'NONE',  ( 6.503815726751999371, 121.4942169270607053, -0.3795357812798487163 ) ) ;
#8825=CARTESIAN_POINT ( 'NONE',  ( -13.94976549039478186, 152.5802402909829425, -2.190326936676450398 ) ) ;
#8826=CARTESIAN_POINT ( 'NONE',  ( 4.296659151754357531, -15.58794764271442901, 2.529927869898711545 ) ) ;
#8827=CARTESIAN_POINT ( 'NONE',  ( -4.254363289858590136, 118.2238500054434382, -0.4591314105454073480 ) ) ;
#8830=CARTESIAN_POINT ( 'NONE',  ( -4.812647089374579856, 117.4736139279835072, 1.001469096630185796 ) ) ;
#8831=CARTESIAN_POINT ( 'NONE',  ( 0.8526219981721140373, 157.1001331247151143, 1.466586365881669574 ) ) ;
#8832=CARTESIAN_POINT ( 'NONE',  ( -5.010144981628188887, 117.3993855238222608, -0.7522679339500687457 ) ) ;
#8833=CARTESIAN_POINT ( 'NONE',  ( -8.332721659230562850, 3.087680552427906733, 1.359589815967415127 ) ) ;
#8834=CARTESIAN_POINT ( 'NONE',  ( 0.6512579105864789719, 156.3106852680424765, 0.2006220687487344223 ) ) ;
#8838=CARTESIAN_POINT ( 'NONE',  ( -0.4424955508668900750, 117.9394511451274781, 1.393115402039464268 ) ) ;
#8840=CARTESIAN_POINT ( 'NONE',  ( -7.948460536704424761, 121.7397034463535874, -1.077183805330166999 ) ) ;
#8843=CARTESIAN_POINT ( 'NONE',  ( -22.83127913370414674, 150.4067493646842593, -0.3029848903584387854 ) ) ;
#8846=CARTESIAN_POINT ( 'NONE',  ( 6.029423134339813473, 121.4446780596064315, 0.06661046868258485576 ) ) ;
#8848=ORIENTED_EDGE ( 'NONE', *, *, #17811, .F. ) ;
#8849=CARTESIAN_POINT ( 'NONE',  ( 2.147067015561635817, 115.7025572403689750, -1.628760164966848389 ) ) ;
#8850=CARTESIAN_POINT ( 'NONE',  ( -7.046279781204644266, 122.0586610246435129, -0.2738582164285299214 ) ) ;
#8851=CARTESIAN_POINT ( 'NONE',  ( 5.386302285778954868, -11.84411807400357475, 0.7125209553660817319 ) ) ;
#8852=CARTESIAN_POINT ( 'NONE',  ( -21.83021172428713896, 149.6930991844618291, 1.147003836765864593 ) ) ;
#8854=CARTESIAN_POINT ( 'NONE',  ( 11.65197432296780278, 118.7334002725740874, 0.4428703322330642123 ) ) ;
#8855=CARTESIAN_POINT ( 'NONE',  ( 13.58953805363860745, 150.2515523695257116, 0.3364537918566254393 ) ) ;
#8856=CARTESIAN_POINT ( 'NONE',  ( -6.639407854763120941E-14, 101.6934662015457320, 3.307182826377456566E-30 ) ) ;
#8857=CARTESIAN_POINT ( 'NONE',  ( -0.8176680875534481086, 23.83313504737664346, 0.5327793711180701663 ) ) ;
#8858=CARTESIAN_POINT ( 'NONE',  ( -3.295257134497992180, 159.4684106755469202, -0.1128235000732132204 ) ) ;
#8860=CIRCLE ( 'NONE', #25183, 0.5080000000000002292 ) ;
#8863=CARTESIAN_POINT ( 'NONE',  ( -8.425645715861348251, 119.6231226099808254, 1.083608480663881490 ) ) ;
#8865=CARTESIAN_POINT ( 'NONE',  ( 2.066728864738883953, 117.5043770775735510, 0.6257643424168405355 ) ) ;
#8866=CARTESIAN_POINT ( 'NONE',  ( 12.87447296688122300, 155.3440856034525837, -1.681555337288024754 ) ) ;
#8867=CARTESIAN_POINT ( 'NONE',  ( 4.581731014592691054, -15.30239759458089388, -0.5121113081912510578 ) ) ;
#8868=CARTESIAN_POINT ( 'NONE',  ( -20.05503673871689685, 132.0867704272472452, -1.718978086785434733 ) ) ;
#8869=CARTESIAN_POINT ( 'NONE',  ( 4.805319368223364584, 117.6713915772949974, -0.9245024293283279349 ) ) ;
#8870=CARTESIAN_POINT ( 'NONE',  ( 2.913298842129254496, 107.8271213589905386, 4.473571949258134950 ) ) ;
#8871=CARTESIAN_POINT ( 'NONE',  ( -15.79043079689205697, 145.9231181611787918, -0.08479106802855317093 ) ) ;
#8872=CARTESIAN_POINT ( 'NONE',  ( -18.85642017384699898, 148.8558894138562039, -2.490767737705128049 ) ) ;
#8873=CARTESIAN_POINT ( 'NONE',  ( 6.347728850385006005, -14.18411723689298753, 0.2678442101147658905 ) ) ;
#8878=CARTESIAN_POINT ( 'NONE',  ( 14.78649082109369672, 128.5561590274816126, 2.111834004041170498 ) ) ;
#8881=CARTESIAN_POINT ( 'NONE',  ( -3.159661387648548647, 123.6198120039584154, 0.01957516827081343461 ) ) ;
#8882=CARTESIAN_POINT ( 'NONE',  ( -2.078203845413400863, -12.60517393744602721, -8.197436486331740824 ) ) ;
#8883=CARTESIAN_POINT ( 'NONE',  ( 8.116318325016090185, 154.6259123219959690, 0.9857874811295551654 ) ) ;
#8884=CARTESIAN_POINT ( 'NONE',  ( -5.012889280905649336, 115.6909491485453003, -1.400213983655213212 ) ) ;
#8885=CARTESIAN_POINT ( 'NONE',  ( 22.56840570087976872, 150.3096427868838987, -0.3971349512683050031 ) ) ;
#8888=CARTESIAN_POINT ( 'NONE',  ( -8.793333135444262538, 117.6964036462294274, -0.2880565789670351817 ) ) ;
#8895=CARTESIAN_POINT ( 'NONE',  ( 8.213282778328196088, 120.6581456215331372, -1.077642949125763083 ) ) ;
#8896=CARTESIAN_POINT ( 'NONE',  ( -4.171990346301578612, 104.6144662015457385, -4.124402238216698713 ) ) ;
#8897=CARTESIAN_POINT ( 'NONE',  ( -14.94204527009774175, 148.8997249754567349, -1.137790122619589228 ) ) ;
#8900=CARTESIAN_POINT ( 'NONE',  ( -6.439570805302779653E-14, 116.4254662015457313, -3.894619736530179447E-17 ) ) ;
#8903=CARTESIAN_POINT ( 'NONE',  ( -2.201963191602333225, 30.07953629247752758, -4.075912811544394998 ) ) ;
#8906=CARTESIAN_POINT ( 'NONE',  ( -3.174366308152013705, 104.6144662015457243, -0.06343139340882732180 ) ) ;
#8908=CARTESIAN_POINT ( 'NONE',  ( -6.994445320580605419, 121.9510454495767817, -0.1010066434573844985 ) ) ;
#8909=CARTESIAN_POINT ( 'NONE',  ( 0.4006815055314143503, 20.64345356492705719, 4.603752038498275745 ) ) ;
#8910=CARTESIAN_POINT ( 'NONE',  ( 22.81419135200704673, 148.8343141121478652, 1.537101565576850959 ) ) ;
#8912=CARTESIAN_POINT ( 'NONE',  ( 3.216763585201820153, -14.58149021785123978, 2.832987347109013676 ) ) ;
#8913=CARTESIAN_POINT ( 'NONE',  ( 20.90199038452897184, 141.6159226613069109, -1.473829418026497029 ) ) ;
#8914=CARTESIAN_POINT ( 'NONE',  ( -5.874384117068585098, 120.0568572605186546, 0.8667843538975030793 ) ) ;
#8915=CARTESIAN_POINT ( 'NONE',  ( -4.628372119175923949, 18.04465247731148381, -0.2036312542868722320 ) ) ;
#8916=CARTESIAN_POINT ( 'NONE',  ( -22.92073667220936883, 148.8788797244430384, -1.430292205038964815 ) ) ;
#8917=CARTESIAN_POINT ( 'NONE',  ( -0.6014681082635296994, -0.5174402789662015945, 0.7683055774679631300 ) ) ;
#8921=CARTESIAN_POINT ( 'NONE',  ( -9.260187833317626627, 153.8817031120973411, 0.3320757922997039646 ) ) ;
#8922=CARTESIAN_POINT ( 'NONE',  ( 2.095434763668091005, -15.29852786734210746, 5.959135360315205077 ) ) ;
#8923=CARTESIAN_POINT ( 'NONE',  ( 16.74402619291549144, 146.1290494286844819, -1.112937342747913672 ) ) ;
#8924=EDGE_LOOP ( 'NONE', ( #40682, #36696, #8300, #35309, #19220, #16470, #28126, #39116, #40558 ) ) ;
#8925=CARTESIAN_POINT ( 'NONE',  ( 2.413036817438981352, 115.7029552731866886, 1.699863360245213117 ) ) ;
#8926=CARTESIAN_POINT ( 'NONE',  ( -4.807653879508299255, 117.8307963401735776, -0.8997078521567819509 ) ) ;
#8927=CARTESIAN_POINT ( 'NONE',  ( 15.78437780952694069, 146.2378312303354448, 0.3154094333657936899 ) ) ;
#8929=CARTESIAN_POINT ( 'NONE',  ( 12.54651694896164749, 122.2722385251898771, 1.803108555445325445 ) ) ;
#8930=CARTESIAN_POINT ( 'NONE',  ( 5.959810334499592521, 155.3892724211786742, 0.1190911940436167188 ) ) ;
#8933=CARTESIAN_POINT ( 'NONE',  ( 4.992456132208793029, 117.4692012670405319, -0.8003051716943823113 ) ) ;
#8934=CARTESIAN_POINT ( 'NONE',  ( 16.05353943441293296, 121.3766923467913585, -0.004207837007976880303 ) ) ;
#8937=CIRCLE ( 'NONE', #13710, 5.588000000000006295 ) ;
#8940=EDGE_CURVE ( 'NONE', #4233, #30281, #12393, .T. ) ;
#8941=CARTESIAN_POINT ( 'NONE',  ( 1.826821012229639996, -15.37444383369212986, 5.378835944469607888 ) ) ;
#8943=DIRECTION ( 'NONE',  ( -5.206863593109713661E-17, 1.000000000000000000, -1.077750396879097183E-30 ) ) ;
#8944=CARTESIAN_POINT ( 'NONE',  ( -4.680719045354315710, 117.9631509934803972, 0.7257729203454069689 ) ) ;
#8947=CARTESIAN_POINT ( 'NONE',  ( 8.462540607029417572, 119.4400513420865906, -1.051277921553159356 ) ) ;
#8948=CARTESIAN_POINT ( 'NONE',  ( -5.090087584497108075, 118.2545999410811106, -0.7183934583778603944 ) ) ;
#8949=CARTESIAN_POINT ( 'NONE',  ( 4.794056055625289581, 117.6746627338869047, 1.099109741275124952 ) ) ;
#8951=CARTESIAN_POINT ( 'NONE',  ( 2.233078627056604759, -15.14192004606506536, 5.083345892419886880 ) ) ;
#8952=CARTESIAN_POINT ( 'NONE',  ( -0.1041500444720373508, 106.1822392402443143, 5.212094112990285133 ) ) ;
#8953=CARTESIAN_POINT ( 'NONE',  ( -3.178183004559932190, -7.902942162671289239, -3.366045245292264010 ) ) ;
#8956=CARTESIAN_POINT ( 'NONE',  ( 4.405468973772799224, 113.1344509532474376, -2.291157639236350185 ) ) ;
#8957=CARTESIAN_POINT ( 'NONE',  ( -10.57849499609994304, 123.4307455932968765, -1.421577474458307400 ) ) ;
#8958=CARTESIAN_POINT ( 'NONE',  ( 6.997680356709169658, 121.9559740633448115, 0.1243954239949175838 ) ) ;
#8959=DIRECTION ( 'NONE',  ( 0.1548479172700143736, -0.9876883405951387696, -0.02222305941043778779 ) ) ;
#8960=CARTESIAN_POINT ( 'NONE',  ( -1.944923406237783814, 115.7029431175197658, 1.643877071207305418 ) ) ;
#8961=CARTESIAN_POINT ( 'NONE',  ( -3.158589313471108273, 4.191505055319899142, 3.400481138232230194 ) ) ;
#8962=CARTESIAN_POINT ( 'NONE',  ( 11.50728102546029064, 118.8226552325407397, 0.6924515317502046852 ) ) ;
#8963=ORIENTED_EDGE ( 'NONE', *, *, #40501, .T. ) ;
#8964=CARTESIAN_POINT ( 'NONE',  ( 1.773712854446913623, 104.6144662015413758, -5.033492136046540111 ) ) ;
#8965=CARTESIAN_POINT ( 'NONE',  ( 3.297442402085044133, -15.64565814434701352, 4.209479195861737466 ) ) ;
#8966=CARTESIAN_POINT ( 'NONE',  ( -17.85428843624176665, 135.5811125208551857, 1.719929978336786514 ) ) ;
#8967=CARTESIAN_POINT ( 'NONE',  ( 0.7510871189337386955, -11.68616409646884158, 0.6196617644748384501 ) ) ;
#8969=CARTESIAN_POINT ( 'NONE',  ( 0.1178611003048646577, 6.342877585758503578, 0.9680126135609015137 ) ) ;
#8974=CARTESIAN_POINT ( 'NONE',  ( 4.531575537551966626, 119.7344140837147819, 0.5249638875923486880 ) ) ;
#8975=CARTESIAN_POINT ( 'NONE',  ( -5.884536728138022532, 121.1554468101848130, 0.4284271420130267849 ) ) ;
#8977=CARTESIAN_POINT ( 'NONE',  ( 3.449548791184131602, -12.83738641323306595, 1.613555780903996206 ) ) ;
#8978=CARTESIAN_POINT ( 'NONE',  ( 5.108784305046350838, 120.0747842884402132, -0.7604166522187120192 ) ) ;
#8979=CARTESIAN_POINT ( 'NONE',  ( -19.69933843609255675, 149.7343351798865285, -2.455316921491699222 ) ) ;
#8981=CARTESIAN_POINT ( 'NONE',  ( 3.131015516031846690, -14.62848841321586946, 3.524024012273756501 ) ) ;
#8982=CARTESIAN_POINT ( 'NONE',  ( -0.05411207418350773291, 38.74323431000957640, 0.9275608492890762280 ) ) ;
#8983=CARTESIAN_POINT ( 'NONE',  ( 15.82110658236419631, 145.7390459690742830, -0.1389873312028085395 ) ) ;
#8984=EDGE_CURVE ( 'NONE', #39579, #20685, #13596, .T. ) ;
#8985=ORIENTED_EDGE ( 'NONE', *, *, #14121, .T. ) ;
#8989=CARTESIAN_POINT ( 'NONE',  ( 4.968851538487103703, 117.5943734491196722, 0.8206492525603533705 ) ) ;
#8991=CARTESIAN_POINT ( 'NONE',  ( 8.327223946240280839, 23.24253473731531727, -1.329248712143314748 ) ) ;
#8992=CARTESIAN_POINT ( 'NONE',  ( 6.627928625996522882, 155.5185402614932570, 1.342408143365148021 ) ) ;
#8994=CARTESIAN_POINT ( 'NONE',  ( 22.98549031890215844, 150.1594536303649932, 0.4336790679505427293 ) ) ;
#8995=CARTESIAN_POINT ( 'NONE',  ( -4.812383263389278021, 112.7966860322829206, 2.369499567760593450 ) ) ;
#8996=B_SPLINE_CURVE_WITH_KNOTS ( 'NONE', 3,
 ( #1879, #5293, #34048, #41062, #5087, #40853, #34258, #11656, #11873, #14842, #21858, #14634, #18242, #5498, #3091 ),
 .UNSPECIFIED., .F., .F.,
 ( 4, 2, 2, 2, 1, 2, 2, 4 ),
 ( 0.000000000000000000, 0.06249999999999900080, 0.1249999999999978906, 0.2499999999999956701, 0.2812499999999951150, 0.3749999999999934497, 0.4374999999999933387, 0.5000000000000000000 ),
 .UNSPECIFIED. ) ;
#8999=CARTESIAN_POINT ( 'NONE',  ( -1.504723661876595786, -8.552649586842417051, -4.374500482163298898 ) ) ;
#9000=CARTESIAN_POINT ( 'NONE',  ( 5.959810334499592521, 155.3892724211786742, 0.1190911940436167188 ) ) ;
#9001=CARTESIAN_POINT ( 'NONE',  ( 7.688107727944508696, 4.450669244509953160, -3.435853896805545649 ) ) ;
#9002=CARTESIAN_POINT ( 'NONE',  ( -2.150834356787523660, 116.6630246571967575, -0.4597420995432478508 ) ) ;
#9003=CARTESIAN_POINT ( 'NONE',  ( 0.01635612298154385039, 119.2343925067225427, -0.8185272769043290264 ) ) ;
#9007=CARTESIAN_POINT ( 'NONE',  ( -8.092465427151658730, -6.292564624861634037, 2.510960718618908238 ) ) ;
#9008=CARTESIAN_POINT ( 'NONE',  ( 0.07507557030359549022, 117.9394488564931009, 1.409405562719200811 ) ) ;
#9011=CARTESIAN_POINT ( 'NONE',  ( 0.7690845662405288996, 119.7070660435176279, -0.6575911349602956424 ) ) ;
#9012=CARTESIAN_POINT ( 'NONE',  ( -7.924482676426956473, 158.6683511845044734, 0.3722227806660352578 ) ) ;
#9013=AXIS2_PLACEMENT_3D ( 'NONE', #8787, #5812, #21961 ) ;
#9016=( BOUNDED_CURVE ( )  B_SPLINE_CURVE ( 3, ( #3685, #19422, #26455, #17070 ),
 .UNSPECIFIED., .F., .F. ) 
 B_SPLINE_CURVE_WITH_KNOTS ( ( 4, 4 ),
 ( 0.7252176650374851929, 0.9253411388830656836 ),
 .UNSPECIFIED. ) 
 CURVE ( )  GEOMETRIC_REPRESENTATION_ITEM ( )  RATIONAL_B_SPLINE_CURVE ( ( 0.5049133130095756483, 0.4784625025417720279, 0.5588101048313269814, 0.7459561198782403979 ) ) 
 REPRESENTATION_ITEM ( '' )  );
#9019=CARTESIAN_POINT ( 'NONE',  ( -9.100602120603912937, 153.9557227532744150, -0.1238295526561323939 ) ) ;
#9020=CARTESIAN_POINT ( 'NONE',  ( 6.478224611219328466, -13.79365725417489053, 0.02984861787792387686 ) ) ;
#9021=CARTESIAN_POINT ( 'NONE',  ( -19.44243145639594061, 150.5708382285403388, 1.622132703307645807 ) ) ;
#9022=CARTESIAN_POINT ( 'NONE',  ( 2.057861540686706459, 117.3535355059730705, -0.5007145131239726377 ) ) ;
#9023=CARTESIAN_POINT ( 'NONE',  ( 2.003160574663116034, 15.61121511114846960, 4.187759092076685619 ) ) ;
#9024=CARTESIAN_POINT ( 'NONE',  ( -15.09710430809812642, 156.1437908837410191, -0.6951944926208389886 ) ) ;
#9027=FACE_OUTER_BOUND ( 'NONE', #6994, .T. ) ;
#9029=CARTESIAN_POINT ( 'NONE',  ( -13.47719143446468948, 152.3772590505219569, 1.474657383304484259 ) ) ;
#9031=CARTESIAN_POINT ( 'NONE',  ( 13.98553986197810062, 125.7699432187419575, -1.444593012458400105 ) ) ;
#9032=CARTESIAN_POINT ( 'NONE',  ( -4.922209265113230536, 118.1424809852657773, -0.9875327093606014461 ) ) ;
#9034=CIRCLE ( 'NONE', #24669, 4.826000000000001400 ) ;
#9035=B_SPLINE_CURVE_WITH_KNOTS ( 'NONE', 3,
 ( #21401, #37620, #28024, #21201, #8443, #28242 ),
 .UNSPECIFIED., .F., .F.,
 ( 4, 2, 4 ),
 ( 0.000000000000000000, 0.0002825957426950183467, 0.0005651914853900366935 ),
 .UNSPECIFIED. ) ;
#9036=CARTESIAN_POINT ( 'NONE',  ( 5.888833980634776921, 121.2452591720019370, -0.3608419296047722380 ) ) ;
#9037=CARTESIAN_POINT ( 'NONE',  ( -17.78478073489628031, 148.4245508482893854, -2.330447787059697795 ) ) ;
#9038=CARTESIAN_POINT ( 'NONE',  ( 3.431757876926103012, -15.17734022545018391, 2.935651181724953318 ) ) ;
#9039=CARTESIAN_POINT ( 'NONE',  ( -4.065972646788793554, 118.2429491485453070, -0.3080848862740693250 ) ) ;
#9041=CARTESIAN_POINT ( 'NONE',  ( -4.793595683501052918, 117.7335357436302559, 0.8914022784051079951 ) ) ;
#9042=CARTESIAN_POINT ( 'NONE',  ( 3.724242145611105670, 156.8112981010400802, 1.651639321868204613 ) ) ;
#9045=CARTESIAN_POINT ( 'NONE',  ( 0.1224881284885083327, 5.266211660758980173, 8.431793989537572642 ) ) ;
#9046=CARTESIAN_POINT ( 'NONE',  ( 4.292261259499645654, 155.8363458669846864, 0.4108933393057505601 ) ) ;
#9050=ORIENTED_EDGE ( 'NONE', *, *, #19791, .T. ) ;
#9051=CARTESIAN_POINT ( 'NONE',  ( -0.5175973550576450366, 118.1588899065644966, 0.8875034609994335577 ) ) ;
#9054=CARTESIAN_POINT ( 'NONE',  ( -7.851552067626940357, 122.2419137942978864, -0.7720006874763839511 ) ) ;
#9055=VECTOR ( 'NONE', #39192, 1000.000000000000000 ) ;
#9058=CARTESIAN_POINT ( 'NONE',  ( -16.84917212821883581, 155.2300590059875844, -0.1976545469556808265 ) ) ;
#9059=EDGE_LOOP ( 'NONE', ( #15896, #6491, #22265, #36267 ) ) ;
#9061=CARTESIAN_POINT ( 'NONE',  ( -6.015894240732284182, 121.4385361577320595, -0.1720725319338911041 ) ) ;
#9062=CARTESIAN_POINT ( 'NONE',  ( -7.878666962121352313, 122.2304107671814251, 0.4668939114535545221 ) ) ;
#9064=CARTESIAN_POINT ( 'NONE',  ( 1.895611262766748295, 115.7029491485453434, -1.647518854579561820 ) ) ;
#9065=CARTESIAN_POINT ( 'NONE',  ( 0.001255909994487175050, 120.9722815239556439, -0.06285087176068875070 ) ) ;
#9066=CARTESIAN_POINT ( 'NONE',  ( 5.009217890960311337, -13.99182267686448178, 3.873128360714999552 ) ) ;
#9067=CARTESIAN_POINT ( 'NONE',  ( -20.26345141861418142, 136.2683111393718320, 1.346723181737012665 ) ) ;
#9070=CARTESIAN_POINT ( 'NONE',  ( 0.3042230016542175619, 116.5226405152084652, 0.1306790058978156699 ) ) ;
#9071=CARTESIAN_POINT ( 'NONE',  ( 15.19842606723472400, 143.4031501637221879, 0.4388155327730876021 ) ) ;
#9073=CARTESIAN_POINT ( 'NONE',  ( 0.2560056206704328097, 6.564126901726701213, 0.9442708342526761056 ) ) ;
#9074=CARTESIAN_POINT ( 'NONE',  ( -15.69471450241215571, 120.8333755831694702, -0.3643268586347850335 ) ) ;
#9076=CARTESIAN_POINT ( 'NONE',  ( -5.152689475313444234, 116.8412042432202185, -0.1029630068797482562 ) ) ;
#9078=CARTESIAN_POINT ( 'NONE',  ( -8.651804384430541006, 118.4863469498705797, 0.7357695435087184821 ) ) ;
#9080=CARTESIAN_POINT ( 'NONE',  ( 20.19347568108150526, 136.2683111393718320, 2.155148867324337747 ) ) ;
#9081=CARTESIAN_POINT ( 'NONE',  ( 14.15994444794823259, 154.3735777161816429, -1.715400944796409144 ) ) ;
#9082=CARTESIAN_POINT ( 'NONE',  ( -2.276242205911199523, 25.81146128161704567, -8.137376054096339573 ) ) ;
#9083=CARTESIAN_POINT ( 'NONE',  ( -22.02091170609381976, 149.7938220333360846, -1.879853634988783329 ) ) ;
#9084=CARTESIAN_POINT ( 'NONE',  ( 4.811064755782845204, 117.8746741567870373, -0.6667383956446522042 ) ) ;
#9085=CARTESIAN_POINT ( 'NONE',  ( 5.281229466409561368, 116.7000894413872629, 1.021210189368793486 ) ) ;
#9086=CARTESIAN_POINT ( 'NONE',  ( -15.53315888837599168, 147.5314071815517138, -0.1823436108899490204 ) ) ;
#9087=CARTESIAN_POINT ( 'NONE',  ( -18.07722773961213747, 140.6071502257508143, -2.476399831607924096 ) ) ;
#9088=CARTESIAN_POINT ( 'NONE',  ( 6.311525104866394287, -14.07095602924590594, 0.9561848504773229340 ) ) ;
#9091=B_SPLINE_CURVE_WITH_KNOTS ( 'NONE', 3,
 ( #24923, #37921, #2993, #35355, #35781, #39181, #9574, #38555, #6, #218, #15953, #9368, #19154, #5980, #35572, #6595, #13193, #3625, #22544, #6390, #22332, #18943, #25965, #28949 ),
 .UNSPECIFIED., .F., .F.,
 ( 4, 2, 2, 2, 2, 2, 2, 2, 2, 2, 2, 4 ),
 ( 0.0006020626168661550497, 0.003690437786238830956, 0.006778812955611506971, 0.008323000540297826114, 0.009095094332641003032, 0.009867188124984181685, 0.01063928191732735860, 0.01141137570967053552, 0.01218346950201371418, 0.01256951639818529483, 0.01276253984627108429, 0.01295556329435687375 ),
 .UNSPECIFIED. ) ;
#9092=CARTESIAN_POINT ( 'NONE',  ( -0.9909088102708097923, 117.3993836601271568, -1.479711866447754876 ) ) ;
#9093=CIRCLE ( 'NONE', #26072, 0.5080000000000002292 ) ;
#9095=CARTESIAN_POINT ( 'NONE',  ( 0.9451225546579952175, 157.6350123088122359, 1.628263479412583870 ) ) ;
#9096=CARTESIAN_POINT ( 'NONE',  ( -4.854024325513706550, 118.7629491485453599, 0.1807258574060142675 ) ) ;
#9097=CIRCLE ( 'NONE', #18600, 3.175000000000001155 ) ;
#9098=CARTESIAN_POINT ( 'NONE',  ( -2.578112510118048206, 120.6526784328644339, 0.3421008684282442203 ) ) ;
#9099=CARTESIAN_POINT ( 'NONE',  ( 0.6424836204703546771, -8.070646579680392563, 8.395564330620057802 ) ) ;
#9100=CARTESIAN_POINT ( 'NONE',  ( 11.72694347678944915, 128.3321206738457647, 0.9702521317530999889 ) ) ;
#9102=CARTESIAN_POINT ( 'NONE',  ( 22.74771312706160131, 149.7444054411783441, -0.5134062617908412562 ) ) ;
#9108=CARTESIAN_POINT ( 'NONE',  ( 4.875296837154728280, 115.9539249584174314, -1.177764552249251917 ) ) ;
#9110=CARTESIAN_POINT ( 'NONE',  ( -4.362246989847086809, 119.4897582430469498, -0.9267953991463255825 ) ) ;
#9112=CARTESIAN_POINT ( 'NONE',  ( 4.141126571459865069, 104.6144662015457243, 4.161112031276615220 ) ) ;
#9113=AXIS2_PLACEMENT_3D ( 'NONE', #30282, #37729, #17293 ) ;
#9114=CARTESIAN_POINT ( 'NONE',  ( -9.577010982344122070, 124.1734284925964573, -0.7139017932201209282 ) ) ;
#9116=CARTESIAN_POINT ( 'NONE',  ( 13.43845804798103316, 156.9141898299356512, 0.2685323735513602261 ) ) ;
#9117=EDGE_LOOP ( 'NONE', ( #17167, #36828, #12871, #22664, #29614, #34122, #12514, #38042 ) ) ;
#9118=CARTESIAN_POINT ( 'NONE',  ( -1.756104463947763206, 14.33678105357426702, 4.288642365192034234 ) ) ;
#9120=CARTESIAN_POINT ( 'NONE',  ( -4.828962989263914984, 117.4049964369462060, 1.009641684917192306 ) ) ;
#9121=CARTESIAN_POINT ( 'NONE',  ( -5.008948584507881385, 27.92152162925472325, 0.4889012661100834434 ) ) ;
#9123=DIRECTION ( 'NONE',  ( 0.01997839162482749689, 1.040247600000945640E-18, -0.9998004120163610509 ) ) ;
#9124=CARTESIAN_POINT ( 'NONE',  ( 7.784332241379921413, 122.6279634482064154, 0.1742627236427056192 ) ) ;
#9125=CARTESIAN_POINT ( 'NONE',  ( 3.308978306493741250, 24.09187545982852541, -3.235542752117448018 ) ) ;
#9126=CARTESIAN_POINT ( 'NONE',  ( 13.03166249679904354, 119.8917521002241955, 1.045815086349644929 ) ) ;
#9127=CARTESIAN_POINT ( 'NONE',  ( -4.074141608589817665, 104.6144662015457669, -2.607666899705321395 ) ) ;
#9129=CARTESIAN_POINT ( 'NONE',  ( 21.19479858968361796, 149.1058327099893290, -1.460163390594824806 ) ) ;
#9130=CARTESIAN_POINT ( 'NONE',  ( -11.45258232062230697, 123.1738952066917534, 1.204891439250160623 ) ) ;
#9131=CARTESIAN_POINT ( 'NONE',  ( 2.264360804680111805, 21.29314879275315064, 4.027482774281332389 ) ) ;
#9132=CARTESIAN_POINT ( 'NONE',  ( -11.33669861507968157, 118.9804978796424706, -0.9069902030348426791 ) ) ;
#9133=AXIS2_PLACEMENT_3D ( 'NONE', #13322, #39318, #35282 ) ;
#9134=CARTESIAN_POINT ( 'NONE',  ( 0.6271221672387817803, 4.229989959315594739, -0.7487545302041328510 ) ) ;
#9137=CARTESIAN_POINT ( 'NONE',  ( -15.96529520877018626, 145.8030804522035737, 0.4114451159501718580 ) ) ;
#9138=CARTESIAN_POINT ( 'NONE',  ( 5.061152751093137780, -13.25450807444039647, 3.067510535416694495 ) ) ;
#9139=CARTESIAN_POINT ( 'NONE',  ( 15.84185526851198489, 139.7295799824062499, -1.277977597745375560 ) ) ;
#9140=CIRCLE ( 'NONE', #32953, 5.588000000000006295 ) ;
#9141=DIRECTION ( 'NONE',  ( 4.017660918040594346E-17, -1.000000000000000000, -2.376309959284834438E-19 ) ) ;
#9142=CARTESIAN_POINT ( 'NONE',  ( -4.820638971607948520, 117.6752190542308227, -1.075962066314599008 ) ) ;
#9143=CARTESIAN_POINT ( 'NONE',  ( 8.487687333566158898, 123.3253871723413368, 0.1696041924978712867 ) ) ;
#9145=CARTESIAN_POINT ( 'NONE',  ( 13.17434061382155441, 122.5785676075921060, 1.825321299320728397 ) ) ;
#9146=CARTESIAN_POINT ( 'NONE',  ( 10.39928917620358817, 153.1223395828141918, 0.2078025466733119664 ) ) ;
#9149=CARTESIAN_POINT ( 'NONE',  ( 4.828127062081292387, 117.4060377263907213, -1.008211717711906541 ) ) ;
#9150=CARTESIAN_POINT ( 'NONE',  ( 16.78241155767104331, 155.2615993841311877, -0.07296080027729302808 ) ) ;
#9151=PLANE ( 'NONE',  #22684 ) ;
#9154=CARTESIAN_POINT ( 'NONE',  ( 1.912964346608580835, -15.38803350473924603, 5.361940315677870217 ) ) ;
#9158=CARTESIAN_POINT ( 'NONE',  ( -4.625240786758006095, 118.0596839624423495, 0.5387667837598054676 ) ) ;
#9161=CARTESIAN_POINT ( 'NONE',  ( -1.378789611427061912, 115.6909491485452577, -1.738307004888806961 ) ) ;
#9162=CARTESIAN_POINT ( 'NONE',  ( 3.566060519644585369, 118.7008415277600903, -0.7946426777497477278 ) ) ;
#9163=CARTESIAN_POINT ( 'NONE',  ( -4.979866836074960723, 117.8491495069952748, -0.7948704875671745995 ) ) ;
#9164=CARTESIAN_POINT ( 'NONE',  ( 4.648305118706619332, 118.0133915895967931, 0.7935454642018273663 ) ) ;
#9166=CARTESIAN_POINT ( 'NONE',  ( -0.2562694446383195213, 108.5751225745497806, 4.260274975123000019 ) ) ;
#9170=CARTESIAN_POINT ( 'NONE',  ( 0.1065646865914871566, 105.8844662015456777, -5.332932678536312032 ) ) ;
#9171=CARTESIAN_POINT ( 'NONE',  ( -10.79132569999989144, 123.6843197456346672, -1.443847663909934242 ) ) ;
#9172=CARTESIAN_POINT ( 'NONE',  ( -3.702526914408131642, 33.15860816321391979, 4.132160499251987140 ) ) ;
#9173=CARTESIAN_POINT ( 'NONE',  ( -2.103092518242876796, 115.7026983564594644, 1.632052075412017134 ) ) ;
#9174=CARTESIAN_POINT ( 'NONE',  ( 4.636458409304901274, 17.36039413176390411, -0.09481320587925551324 ) ) ;
#9175=CARTESIAN_POINT ( 'NONE',  ( 16.79208607122037833, 122.6968688451475771, 0.8807046615161950864 ) ) ;
#9176=EDGE_LOOP ( 'NONE', ( #14854, #40929, #14912, #35893, #16485 ) ) ;
#9177=CARTESIAN_POINT ( 'NONE',  ( 3.700855694654260564, 104.6144662015545208, -3.857327698788455717 ) ) ;
#9178=CARTESIAN_POINT ( 'NONE',  ( 3.184821769958268600, -15.26663968290864482, 3.758507235160873261 ) ) ;
#9179=CARTESIAN_POINT ( 'NONE',  ( -5.043395383124352982, 119.2220797256985350, 0.8992592568097313999 ) ) ;
#9180=CARTESIAN_POINT ( 'NONE',  ( 0.9697834966998255535, 21.94565095173003400, 0.09096683575692042500 ) ) ;
#9181=CARTESIAN_POINT ( 'NONE',  ( -0.5327793704965378963, 2.243135046448306191, -0.8176680881360027797 ) ) ;
#9182=EDGE_CURVE ( 'NONE', #23570, #11667, #6128, .T. ) ;
#9186=CARTESIAN_POINT ( 'NONE',  ( 3.197921176416294919, 118.4615047536228047, 0.7906167528392611388 ) ) ;
#9187=CARTESIAN_POINT ( 'NONE',  ( -13.84625834149343326, 134.3516747369166069, 0.8047173373260270157 ) ) ;
#9189=CARTESIAN_POINT ( 'NONE',  ( 3.107604131292615257, -12.52806217606054773, 0.6782401946156415562 ) ) ;
#9190=CARTESIAN_POINT ( 'NONE',  ( 10.06933303711900507, 122.3915136462027817, -1.070338282017660791 ) ) ;
#9191=CARTESIAN_POINT ( 'NONE',  ( -17.37713502592725590, 151.5007859583534753, -2.430116715062250243 ) ) ;
#9192=LINE ( 'NONE', #5799, #21534 ) ;
#9193=CARTESIAN_POINT ( 'NONE',  ( 7.931513209474629456, 121.8264860997418140, 1.035788693698372676 ) ) ;
#9194=CARTESIAN_POINT ( 'NONE',  ( 4.122826845240182614, 118.2429491485453354, -0.1811473218594779611 ) ) ;
#9195=CARTESIAN_POINT ( 'NONE',  ( 15.76950829013769351, 146.9135488020124001, -0.01503653553346920996 ) ) ;
#9197=CARTESIAN_POINT ( 'NONE',  ( 0.1066086480732678088, 105.8844037013956410, -5.332931792593708309 ) ) ;
#9201=CARTESIAN_POINT ( 'NONE',  ( -7.300781474974964880, 17.39199087320084658, -4.267473507878162486 ) ) ;
#9202=CARTESIAN_POINT ( 'NONE',  ( 12.92681072397279074, 152.2092440956282076, 1.775214794609845548 ) ) ;
#9204=CARTESIAN_POINT ( 'NONE',  ( 18.63485108555815373, 154.1203422869290023, 0.3484461891417475754 ) ) ;
#9205=B_SPLINE_CURVE_WITH_KNOTS ( 'NONE', 3,
 ( #29685, #10085, #16257, #26489, #944, #26703, #106, #3934, #20284, #36303, #3511, #33312, #19454 ),
 .UNSPECIFIED., .F., .F.,
 ( 4, 1, 1, 1, 1, 1, 1, 1, 1, 1, 4 ),
 ( 0.000000000000000000, 0.1250000000000002498, 0.2500000000000004996, 0.3750000000000000555, 0.4109712969816595729, 0.4999999999999996669, 0.6249999999999995559, 0.7500000000000001110, 0.8232913890944979496, 0.8750000000000001110, 1.000000000000000000 ),
 .UNSPECIFIED. ) ;
#9206=CARTESIAN_POINT ( 'NONE',  ( -7.450817465826296448, 123.6645382909113664, -0.1143006167400526935 ) ) ;
#9207=CARTESIAN_POINT ( 'NONE',  ( -2.070226828232369254, -8.352695179381779411, -4.151654383260235726 ) ) ;
#9208=CARTESIAN_POINT ( 'NONE',  ( 8.935197197525127422, 123.9063447689825779, 0.1785465045940572426 ) ) ;
#9210=CARTESIAN_POINT ( 'NONE',  ( 11.72614449088015043, 156.4111399680655552, 2.003450915338490734 ) ) ;
#9212=CARTESIAN_POINT ( 'NONE',  ( 0.8732425085435751022, -3.549726780817298977, -8.398906084147368389 ) ) ;
#9213=CARTESIAN_POINT ( 'NONE',  ( -2.190167605149390351, 116.8639141099391452, -0.5450301620853724716 ) ) ;
#9214=CARTESIAN_POINT ( 'NONE',  ( 0.02135216056670925094, 118.1497763966934258, -1.068549427312529554 ) ) ;
#9215=DIRECTION ( 'NONE',  ( -4.017660918040594346E-17, 1.000000000000000000, 2.376309959284834438E-19 ) ) ;
#9217=CARTESIAN_POINT ( 'NONE',  ( 2.598967704003971146, -9.625211180298204994, -8.041545772114961466 ) ) ;
#9218=CARTESIAN_POINT ( 'NONE',  ( 0.4816777417134468497, 118.1588880427148212, 0.9074776130548274367 ) ) ;
#9220=CARTESIAN_POINT ( 'NONE',  ( 2.766857707386623400, -13.29092698609396450, 0.4080254275553683585 ) ) ;
#9221=CARTESIAN_POINT ( 'NONE',  ( 0.3095834102097976270, 110.3683645023726427, -3.577238406694227546 ) ) ;
#9222=CARTESIAN_POINT ( 'NONE',  ( -18.19405586666668739, 125.1529741258727597, 0.3179404471852275704 ) ) ;
#9223=ORIENTED_EDGE ( 'NONE', *, *, #23245, .T. ) ;
#9227=CARTESIAN_POINT ( 'NONE',  ( -5.078986093043185157, 75.27746620154573520, -0.1014902294541231847 ) ) ;
#9228=CARTESIAN_POINT ( 'NONE',  ( 3.628834229889370544, -15.44114452258853198, 5.288308529986511353 ) ) ;
#9229=CARTESIAN_POINT ( 'NONE',  ( -4.979196860906144551, 118.3881331334009985, 0.8414419690753370817 ) ) ;
#9230=CARTESIAN_POINT ( 'NONE',  ( 22.14298845881043221, 148.3267584643486146, -1.148356825654135438 ) ) ;
#9231=CARTESIAN_POINT ( 'NONE',  ( -3.998286381996895233, 3.741657206818807424, 2.332027183294827832 ) ) ;
#9233=ORIENTED_EDGE ( 'NONE', *, *, #26102, .T. ) ;
#9236=FACE_OUTER_BOUND ( 'NONE', #33251, .T. ) ;
#9237=B_SPLINE_SURFACE_WITH_KNOTS ( 'NONE', 3, 3, ( 
 ( #22009, #41426, #32251, #35040, #2663, #3081, #38647, #16040, #42061, #3503, #309, #3927, #13908, #23050, #32669, #29679, #3715 ),
 ( #13279, #39913, #17094, #26263, #10291, #10706, #23903, #23685, #10914, #522, #36706, #19653, #16887, #40120, #36296, #29888, #16462 ),
 ( #13495, #30097, #726, #938, #16674, #23473, #23261, #29469, #39702, #10502, #7116, #20074, #39273, #10079, #4135, #36084, #7527 ),
 ( #13701, #33515, #33096, #39485, #6898, #36498, #20488, #26695, #7318, #6686, #19868, #26900, #1143, #4349, #17311, #32883, #20278 ),
 ( #26481, #33305, #30300, #14110, #27108, #31141, #37123, #24115, #4553, #17717, #33730, #27944, #18346, #11757, #24745, #4765, #17928 ),
 ( #21117, #37747, #8571, #24526, #11128, #8356, #34143, #30933, #14942, #1568, #24324, #21532, #1772, #40745, #33937, #11542, #2195 ),
 ( #40952, #30511, #4970, #7945, #30716, #14732, #18136, #11969, #14524, #15153, #34564, #5391, #20914, #1351, #27734, #31352, #28157 ),
 ( #20704, #27321, #41163, #36920, #27534, #7738, #37531, #8146, #17513, #21324, #1980, #14308, #40541, #40334, #11336, #34352, #37330 ) ),
 .UNSPECIFIED., .F., .F., .F.,
 ( 4, 1, 2, 1, 4 ),
 ( 4, 1, 1, 1, 1, 1, 1, 1, 1, 1, 1, 1, 1, 1, 4 ),
 ( 0.000000000000000000, 0.2500000000000000000, 0.4999999999999996669, 0.7500000000000000000, 1.000000000000000000 ),
 ( 0.000000000000000000, 0.08300113939718137268, 0.1732806554784933895, 0.2717672377176819087, 0.3752096606209606167, 0.4787223716043260135, 0.5772295444745598747, 0.6668133826162351285, 0.7470991451079272982, 0.7815930070524458317, 0.8169452614683294644, 0.8547689062991584708, 0.8968063284581728745, 0.9447228702782888288, 1.000000000000000000 ),
 .UNSPECIFIED. ) ;
#9238=CARTESIAN_POINT ( 'NONE',  ( -13.27577938203614316, 128.5100244389050204, 1.209575533060950114 ) ) ;
#9239=DIRECTION ( 'NONE',  ( -0.9963102427714440879, 0.000000000000000000, 0.08582482245076958338 ) ) ;
#9241=CARTESIAN_POINT ( 'NONE',  ( 0.03212616895145502249, 157.6269964811067155, -1.607724863813388971 ) ) ;
#9242=CARTESIAN_POINT ( 'NONE',  ( -21.07518769967747119, 148.4376209648218321, -2.358402543220755820 ) ) ;
#9245=CARTESIAN_POINT ( 'NONE',  ( 9.867693216206284035, 124.1914461168675530, -0.5013480754756757252 ) ) ;
#9247=ORIENTED_EDGE ( 'NONE', *, *, #30525, .T. ) ;
#9248=CARTESIAN_POINT ( 'NONE',  ( -15.61558020634891975, 150.8349565870724120, -2.213412335539846509 ) ) ;
#9249=CARTESIAN_POINT ( 'NONE',  ( 3.525547644170144324, -15.07001638954266731, 1.996499786560847367 ) ) ;
#9250=CARTESIAN_POINT ( 'NONE',  ( -4.233202534921607807, 118.2249641308060859, -0.4810777853349767486 ) ) ;
#9253=CARTESIAN_POINT ( 'NONE',  ( -4.935446760104023944, 117.6551691763225875, 0.7496835391351150957 ) ) ;
#9254=CARTESIAN_POINT ( 'NONE',  ( 16.55051581791493476, 149.4842840675632658, 2.199106316832546870 ) ) ;
#9256=CARTESIAN_POINT ( 'NONE',  ( 8.411406395146093118, -11.38171290258811119, -0.9481482025471229536 ) ) ;
#9257=CARTESIAN_POINT ( 'NONE',  ( 4.562414174745239137, 121.1702857069421100, 0.2029539227048861583 ) ) ;
#9260=VERTEX_POINT ( 'NONE', #42000 ) ;
#9264=CARTESIAN_POINT ( 'NONE',  ( -8.517743499764725001, 118.9454930948057125, -1.260829469820966553 ) ) ;
#9268=CARTESIAN_POINT ( 'NONE',  ( -3.286349204026867810, 159.4678586119998442, 0.07386938312792028227 ) ) ;
#9272=CARTESIAN_POINT ( 'NONE',  ( -7.804241651921540956, 122.5006630351903709, -0.4842881838540384343 ) ) ;
#9273=CARTESIAN_POINT ( 'NONE',  ( 4.901481263995191462, 117.4107946624300638, -0.9679066200967618716 ) ) ;
#9275=CARTESIAN_POINT ( 'NONE',  ( 2.448094588128645110, 115.7029487073275504, -1.604675776025721978 ) ) ;
#9276=CARTESIAN_POINT ( 'NONE',  ( -11.10900461081884494, 128.0707465396788507, -0.3225556591789269789 ) ) ;
#9277=CARTESIAN_POINT ( 'NONE',  ( 5.061152751093137780, -13.25450807444039647, 3.067510535416694495 ) ) ;
#9278=CARTESIAN_POINT ( 'NONE',  ( -21.60128648486327663, 148.1022500232506616, 1.385191265705788322 ) ) ;
#9280=CARTESIAN_POINT ( 'NONE',  ( 17.10498822929443108, 122.7072422303320707, 0.5849822763170867690 ) ) ;
#9281=CARTESIAN_POINT ( 'NONE',  ( 6.513934358062148711, 121.7796322531078346, 0.2438456569635198967 ) ) ;
#9282=CARTESIAN_POINT ( 'NONE',  ( 4.851371946308560723, 115.6909491485453145, -1.282097887966950900 ) ) ;
#9283=CARTESIAN_POINT ( 'NONE',  ( 0.5069063945870452281, 6.992850521020996801, 0.8331330811856124674 ) ) ;
#9284=CARTESIAN_POINT ( 'NONE',  ( -10.82257311662895916, 157.9086237439880733, -0.2761350859956693826 ) ) ;
#9287=ORIENTED_EDGE ( 'NONE', *, *, #31822, .F. ) ;
#9288=CARTESIAN_POINT ( 'NONE',  ( 2.333515971706682013, 116.4819875861390841, 0.3626728605129332927 ) ) ;
#9290=CARTESIAN_POINT ( 'NONE',  ( 4.901975893987065902, 117.8999350694477926, 0.9234475893805553781 ) ) ;
#9291=CARTESIAN_POINT ( 'NONE',  ( 12.27107220260955067, 121.7247091083657153, -1.253333917061305147 ) ) ;
#9292=CARTESIAN_POINT ( 'NONE',  ( -4.837940364245437941, 10.07446788996644038, 6.911991265526966188 ) ) ;
#9293=CARTESIAN_POINT ( 'NONE',  ( -20.95410280040443496, 151.1643092826112138, -1.845047842948928540 ) ) ;
#9294=CARTESIAN_POINT ( 'NONE',  ( 4.725550995308940294, 117.9581936019243642, -0.6734248769522227507 ) ) ;
#9295=ADVANCED_FACE ( 'NONE', ( #13003 ), #5464, .F. ) ;
#9296=CARTESIAN_POINT ( 'NONE',  ( 7.639005212201189998, 124.2918010433613745, 0.1615048153450350521 ) ) ;
#9297=CARTESIAN_POINT ( 'NONE',  ( -8.831233598306610588, 123.6950213215744583, -0.09329271932673267875 ) ) ;
#9298=CARTESIAN_POINT ( 'NONE',  ( -18.70459055478416488, 148.4604323410545987, -2.472120825861215732 ) ) ;
#9299=CARTESIAN_POINT ( 'NONE',  ( 2.631220017305710090, -15.63525587843500553, 5.668892982663133573 ) ) ;
#9301=AXIS2_PLACEMENT_3D ( 'NONE', #24497, #5360, #37718 ) ;
#9305=CARTESIAN_POINT ( 'NONE',  ( 2.387603053075636250, 119.2205458019918751, 0.7760930522211749727 ) ) ;
#9306=CARTESIAN_POINT ( 'NONE',  ( -15.64207015331068185, 147.2204672151589193, -0.3125657877211906466 ) ) ;
#9308=CARTESIAN_POINT ( 'NONE',  ( -2.294838902200274422, 118.2243428780609662, 0.8383363118275912740 ) ) ;
#9309=CARTESIAN_POINT ( 'NONE',  ( -3.973931221679809056, 20.38425861574787490, -7.466160517099206473 ) ) ;
#9310=CARTESIAN_POINT ( 'NONE',  ( 5.204851039067889040, 121.0999079655412203, 0.5006067476712320330 ) ) ;
#9311=CARTESIAN_POINT ( 'NONE',  ( 22.52700986351711165, 149.9757045183965261, -0.6247156920787646506 ) ) ;
#9312=CARTESIAN_POINT ( 'NONE',  ( -4.929842468146641288, 117.6425979561673785, -0.8692111560381230451 ) ) ;
#9314=CARTESIAN_POINT ( 'NONE',  ( 4.659827697873120123, 112.0094687158754994, -2.672315607338379362 ) ) ;
#9315=EDGE_LOOP ( 'NONE', ( #21764, #6215, #31541, #40724 ) ) ;
#9316=CARTESIAN_POINT ( 'NONE',  ( 4.469912121137109118, 119.5537132673701137, -0.7488809508603075926 ) ) ;
#9318=CARTESIAN_POINT ( 'NONE',  ( -9.078381139985740589, 123.6795089456687577, -0.5923855214342146347 ) ) ;
#9320=CARTESIAN_POINT ( 'NONE',  ( 8.078287538471617069, 158.6595088495342338, 0.1614234102745199240 ) ) ;
#9322=CARTESIAN_POINT ( 'NONE',  ( 2.584458374606236841, 15.83607344512877368, 3.832284875798456447 ) ) ;
#9324=CARTESIAN_POINT ( 'NONE',  ( -4.923499976822237834, 117.4076456904317638, 0.9491661484678960425 ) ) ;
#9328=CARTESIAN_POINT ( 'NONE',  ( 6.998514830026701716, 121.6887508624515704, 0.6757143304067796397 ) ) ;
#9329=CARTESIAN_POINT ( 'NONE',  ( -2.961220487682185265, 16.77021669962341477, -3.573240411402743621 ) ) ;
#9330=CARTESIAN_POINT ( 'NONE',  ( 22.55218723263367764, 148.5212373274837319, 1.758973660241909709 ) ) ;
#9332=CARTESIAN_POINT ( 'NONE',  ( 0.4201230711237894933, 106.0157732049497241, 5.283348651899852477 ) ) ;
#9333=CARTESIAN_POINT ( 'NONE',  ( 19.85075266274209937, 150.7280352275851101, -1.521773064777484086 ) ) ;
#9334=CARTESIAN_POINT ( 'NONE',  ( -12.23061257473133878, 124.2599011343719155, 1.262879005329815563 ) ) ;
#9335=CARTESIAN_POINT ( 'NONE',  ( 2.776928087254650013, 2.301956178644051221, 3.707541451904531105 ) ) ;
#9336=CARTESIAN_POINT ( 'NONE',  ( -22.14168286312786549, 150.6715983490228723, -1.403651840795990813 ) ) ;
#9338=CARTESIAN_POINT ( 'NONE',  ( -15.40459090795135566, 148.0444422243178337, 0.2810841713230233241 ) ) ;
#9339=CARTESIAN_POINT ( 'NONE',  ( 4.440325138859688714, -14.57630248335078882, 4.728313687495418804 ) ) ;
#9342=CARTESIAN_POINT ( 'NONE',  ( -4.700796422664683227, 117.9670161556764896, -0.8081787690371831090 ) ) ;
#9343=CARTESIAN_POINT ( 'NONE',  ( 8.770618086120967050, 123.6813396614493712, 0.1752578222716852097 ) ) ;
#9345=CARTESIAN_POINT ( 'NONE',  ( 19.09066119453645172, 140.9752145814059645, 2.516632075137499314 ) ) ;
#9346=DIRECTION ( 'NONE',  ( 5.206863593109713661E-17, -1.000000000000000000, 1.077750396879097183E-30 ) ) ;
#9348=CARTESIAN_POINT ( 'NONE',  ( -15.30245393414170074, 121.3917326167944708, 0.5382413912410557444 ) ) ;
#9349=CARTESIAN_POINT ( 'NONE',  ( 4.814838716269237651, 117.4047667081807305, -1.012532368900667556 ) ) ;
#9351=CARTESIAN_POINT ( 'NONE',  ( 18.55749356256734117, 125.2038358216989735, 0.01254332324266071129 ) ) ;
#9353=CARTESIAN_POINT ( 'NONE',  ( 5.319550251556916187, 115.6909491485453145, -0.5107772461581731038 ) ) ;
#9355=CARTESIAN_POINT ( 'NONE',  ( 2.037787548254768488, -15.06252990901250932, 5.718409153091174701 ) ) ;
#9357=CARTESIAN_POINT ( 'NONE',  ( 3.631129234170231257, -15.30172121837498445, -0.5308806197736579691 ) ) ;
#9358=CARTESIAN_POINT ( 'NONE',  ( -4.596941264179941200, 118.0790773607558606, 0.5324384840013657305 ) ) ;
#9360=ORIENTED_EDGE ( 'NONE', *, *, #33182, .F. ) ;
#9361=CARTESIAN_POINT ( 'NONE',  ( -0.4700442440780402964, 115.6909491485452435, -1.765047585021120469 ) ) ;
#9362=CARTESIAN_POINT ( 'NONE',  ( -5.861813178617722109, 119.0059073072438167, -1.257136650504465658 ) ) ;
#9363=CARTESIAN_POINT ( 'NONE',  ( -5.567295163420557635, 119.7830797108918688, -0.4963393297495871659 ) ) ;
#9364=CARTESIAN_POINT ( 'NONE',  ( 4.641264194575597024, 117.9844048130280640, 0.8831379620347793447 ) ) ;
#9366=CARTESIAN_POINT ( 'NONE',  ( -16.02795213054451651, 143.8376908863262997, -1.609587254066635165 ) ) ;
#9367=CARTESIAN_POINT ( 'NONE',  ( -3.160447555344903403, 115.7029629790199863, -1.658213846050050622 ) ) ;
#9368=CARTESIAN_POINT ( 'NONE',  ( -2.461970253143333842, 107.2456962212051224, 4.635069176697791171 ) ) ;
#9369=CARTESIAN_POINT ( 'NONE',  ( -4.808149584360944750, 104.6144662015457243, 0.4147572885131461939 ) ) ;
#9370=CARTESIAN_POINT ( 'NONE',  ( 6.497658445673516248, 120.6500652548963899, -0.1353193420278798464 ) ) ;
#9371=CARTESIAN_POINT ( 'NONE',  ( -17.48541186233178024, 146.4615580561186050, -2.166240883089540770 ) ) ;
#9373=CARTESIAN_POINT ( 'NONE',  ( -0.7326219338007132764, 37.28220708697721619, 2.048504824603447627 ) ) ;
#9374=CARTESIAN_POINT ( 'NONE',  ( -3.034780876608168754, 115.7029491485453292, 1.550823147752200315 ) ) ;
#9375=CARTESIAN_POINT ( 'NONE',  ( 0.1710433496020407063, 14.98650505531991683, 4.637963194678765610 ) ) ;
#9376=CARTESIAN_POINT ( 'NONE',  ( 22.90231444567481489, 149.5023856264156450, 1.310353656364537045 ) ) ;
#9378=CARTESIAN_POINT ( 'NONE',  ( 4.270515072716039029, 104.6144662015391589, -3.200693163871419333 ) ) ;
#9379=CARTESIAN_POINT ( 'NONE',  ( 3.246941722412215459, -15.25025356868572857, 3.602141857564104210 ) ) ;
#9380=CARTESIAN_POINT ( 'NONE',  ( -18.83801864273527471, 140.8526363637247982, 1.765582951612574503 ) ) ;
#9381=CARTESIAN_POINT ( 'NONE',  ( 0.6271221672387817803, 4.229989959315594739, -0.7487545302041328510 ) ) ;
#9382=CARTESIAN_POINT ( 'NONE',  ( 0.4552753346810295421, 10.21665217803766268, -0.8656630863528285147 ) ) ;
#9386=CARTESIAN_POINT ( 'NONE',  ( 3.231430644863403590, 118.6786177306206014, 0.7432888438146501020 ) ) ;
#9388=CARTESIAN_POINT ( 'NONE',  ( -16.29799532358069669, 145.9442052555630767, 0.7927408685852875836 ) ) ;
#9390=CARTESIAN_POINT ( 'NONE',  ( 3.187032726610941946, -14.26951854355915117, 4.096494115788091861 ) ) ;
#9391=CARTESIAN_POINT ( 'NONE',  ( 11.15120438727540630, 123.3376105302527037, -1.132373765670515287 ) ) ;
#9392=CARTESIAN_POINT ( 'NONE',  ( -4.110343450561661172, 118.7489093234570561, -1.002437571585374609 ) ) ;
#9393=CARTESIAN_POINT ( 'NONE',  ( 8.537663472096003403, 118.8514694301399572, 1.229114518489605290 ) ) ;
#9394=CARTESIAN_POINT ( 'NONE',  ( -0.1060743468339773732, 38.40290746171823599, -0.3145143346692479414 ) ) ;
#9395=CARTESIAN_POINT ( 'NONE',  ( 14.75792966017384344, 148.8440819608433969, -0.1510343195432201913 ) ) ;
#9398=CARTESIAN_POINT ( 'NONE',  ( -2.690315046239569075, 30.48488075981191159, 3.827843980145978264 ) ) ;
#9400=CARTESIAN_POINT ( 'NONE',  ( 5.018724313895222444, 117.3993830154766584, -0.7021450163807499978 ) ) ;
#9401=CARTESIAN_POINT ( 'NONE',  ( -1.740095136297252543, 16.12223834230618635, -8.265420891812045312 ) ) ;
#9402=CARTESIAN_POINT ( 'NONE',  ( 10.11490785437005435, 123.9924233945428682, 1.115122180374878091 ) ) ;
#9403=CARTESIAN_POINT ( 'NONE',  ( 23.34374616560282689, 149.0672090665632936, 0.4407082534803009044 ) ) ;
#9404=CARTESIAN_POINT ( 'NONE',  ( -5.300219172352997887, 116.7134249176580028, 0.8085863681920515411 ) ) ;
#9405=CARTESIAN_POINT ( 'NONE',  ( -1.949331898794882667, 118.1189800858121117, 0.8693949517531047722 ) ) ;
#9406=CARTESIAN_POINT ( 'NONE',  ( 4.560200836559435977, -11.68919918208664122, 0.6963878748952898601 ) ) ;
#9407=FACE_OUTER_BOUND ( 'NONE', #31259, .T. ) ;
#9408=CARTESIAN_POINT ( 'NONE',  ( 20.91063213905296791, 147.8517002469272370, 2.402771019925620255 ) ) ;
#9409=CARTESIAN_POINT ( 'NONE',  ( -7.647780498939813931, -9.906183224868927439, 3.644365410659974991 ) ) ;
#9410=CARTESIAN_POINT ( 'NONE',  ( -2.160025851330804159, 116.7207721880314324, -0.4861172116870683402 ) ) ;
#9411=CARTESIAN_POINT ( 'NONE',  ( -0.3557992751142647903, 119.2343925067223722, -0.8259638274389486945 ) ) ;
#9414=CARTESIAN_POINT ( 'NONE',  ( -3.947349438182777615, 105.1227439526176681, 3.603969139096321772 ) ) ;
#9415=CARTESIAN_POINT ( 'NONE',  ( 8.369577038434204752, -11.69170392490758381, 0.7719616968112763544 ) ) ;
#9417=PLANE ( 'NONE',  #11718 ) ;
#9418=CARTESIAN_POINT ( 'NONE',  ( 2.672745566561993247, -14.90124427853171873, 4.600530618394071070 ) ) ;
#9419=CARTESIAN_POINT ( 'NONE',  ( 0.9965922269826466007, 107.7619142660649203, -4.530701086038176228 ) ) ;
#9420=CARTESIAN_POINT ( 'NONE',  ( -6.914686169612833666, 117.4533518774869947, 0.3713220847589206453 ) ) ;
#9425=CARTESIAN_POINT ( 'NONE',  ( 5.478045763647380717, -15.20773871853380044, 2.260320276039294640 ) ) ;
#9426=CARTESIAN_POINT ( 'NONE',  ( -4.077592138694987156, 118.2594131075661608, 0.7845094026950486521 ) ) ;
#9427=CARTESIAN_POINT ( 'NONE',  ( 0.3953301572311454515, 117.5049145548240972, -0.4632619789290191581 ) ) ;
#9428=CARTESIAN_POINT ( 'NONE',  ( 3.102408547967445696, -0.5812848888516047863, -3.453265078539196509 ) ) ;
#9429=EDGE_CURVE ( 'NONE', #14379, #35331, #2056, .T. ) ;
#9431=ORIENTED_EDGE ( 'NONE', *, *, #40256, .F. ) ;
#9433=CARTESIAN_POINT ( 'NONE',  ( -0.03040743767366425876, 116.4813942609868178, 1.521712522323299677 ) ) ;
#9434=CARTESIAN_POINT ( 'NONE',  ( 0.09641566778496790668, 105.7853610664053008, -4.825034276358896257 ) ) ;
#9435=CARTESIAN_POINT ( 'NONE',  ( -17.30559516374544771, 146.8699245690979751, 1.364999074652126110 ) ) ;
#9438=CARTESIAN_POINT ( 'NONE',  ( 4.149433946629322634, 157.3082466949932723, -1.660590259719063377 ) ) ;
#9440=CARTESIAN_POINT ( 'NONE',  ( -9.223174309219253075, 157.2521837264336853, -1.945851059610182343 ) ) ;
#9443=EDGE_CURVE ( 'NONE', #15268, #12250, #27219, .T. ) ;
#9444=CARTESIAN_POINT ( 'NONE',  ( 13.50624371993741768, 134.2048320552371763, -0.5584564168634338355 ) ) ;
#9446=CARTESIAN_POINT ( 'NONE',  ( -9.425008295912185474, 155.1592096034013366, -1.957465225861826363 ) ) ;
#9447=CARTESIAN_POINT ( 'NONE',  ( 3.303734845180175128, -14.82389436555148166, -0.08037074644983704941 ) ) ;
#9448=CARTESIAN_POINT ( 'NONE',  ( -6.472048963935522405E-14, 69.43546620154573645, -1.207165458941418601E-19 ) ) ;
#9451=CARTESIAN_POINT ( 'NONE',  ( -4.891214509481254247, 117.7454895227670448, 0.7291075753013545047 ) ) ;
#9452=CARTESIAN_POINT ( 'NONE',  ( 11.90495122372358594, 153.4554508723442439, 1.948344234133813302 ) ) ;
#9454=CARTESIAN_POINT ( 'NONE',  ( -4.631227783250409402, 22.10816835407601744, -0.05711764529929251599 ) ) ;
#9455=CARTESIAN_POINT ( 'NONE',  ( 1.598479218588785944, 156.2658572007470639, 0.3094434466263951133 ) ) ;
#9458=ADVANCED_FACE ( 'NONE', ( #35603 ), #41624, .T. ) ;
#9462=DIRECTION ( 'NONE',  ( 4.017660918040594346E-17, -1.000000000000000000, -2.376309959284834438E-19 ) ) ;
#9465=CARTESIAN_POINT ( 'NONE',  ( -8.264889197776337681, 120.1602524387331243, -1.449212996374321438 ) ) ;
#9469=CARTESIAN_POINT ( 'NONE',  ( -0.003550357976012296669, 159.5989787797044812, 0.1776744311461875836 ) ) ;
#9472=CARTESIAN_POINT ( 'NONE',  ( 6.049355777633639519, 121.4441731105445967, 0.09395347381935742481 ) ) ;
#9473=ORIENTED_EDGE ( 'NONE', *, *, #19413, .F. ) ;
#9474=CARTESIAN_POINT ( 'NONE',  ( 1.240160200305893134, 115.7029491485453576, -1.694595060456987712 ) ) ;
#9475=CARTESIAN_POINT ( 'NONE',  ( -11.85612367793094535, 151.9842433124228762, -0.4520816642129336094 ) ) ;
#9476=CARTESIAN_POINT ( 'NONE',  ( 2.467627578834723057, -15.39586678991472546, 5.881674146221526733 ) ) ;
#9477=CARTESIAN_POINT ( 'NONE',  ( -0.4156903444693582084, 117.7785671674745771, 0.5149838300002416158 ) ) ;
#9479=CARTESIAN_POINT ( 'NONE',  ( 21.47487836045312903, 132.5742979909900328, 0.7254175812904737342 ) ) ;
#9480=CARTESIAN_POINT ( 'NONE',  ( 8.833705352582880366, 123.8898140529132803, 0.3087918532372332381 ) ) ;
#9481=CARTESIAN_POINT ( 'NONE',  ( 4.765923672690803414, 118.5266822147775940, -0.8411494563746799713 ) ) ;
#9482=CARTESIAN_POINT ( 'NONE',  ( -0.9350042896817728488, 3.318609271805546435, -0.2773724203853295545 ) ) ;
#9483=CARTESIAN_POINT ( 'NONE',  ( -15.43849248880397873, 120.7004057517279989, -0.4663222373074406568 ) ) ;
#9487=CARTESIAN_POINT ( 'NONE',  ( -2.573107000771836628, 116.8397100664982986, 0.4471336313416622854 ) ) ;
#9488=VERTEX_POINT ( 'NONE', #10447 ) ;
#9490=CARTESIAN_POINT ( 'NONE',  ( 14.06037840947770867, 121.6707806233237363, 1.579157835890536710 ) ) ;
#9491=CARTESIAN_POINT ( 'NONE',  ( 5.882864265865802800, 118.8996324090661147, -0.9452689120681908586 ) ) ;
#9492=CARTESIAN_POINT ( 'NONE',  ( 8.413794655563325620, 13.29309125005104164, 0.5966991197660089785 ) ) ;
#9493=CARTESIAN_POINT ( 'NONE',  ( -18.27285712481730684, 128.6097515361309149, -1.839992588890194458 ) ) ;
#9494=CARTESIAN_POINT ( 'NONE',  ( 4.617617679964085120, 117.9735077130049206, -0.7424316868072086129 ) ) ;
#9495=CARTESIAN_POINT ( 'NONE',  ( 5.246745461247972919, 116.0761519159950552, 1.241752167516083194 ) ) ;
#9497=CARTESIAN_POINT ( 'NONE',  ( -5.940729632618867662, 121.5467800236367424, -0.09028238529180369898 ) ) ;
#9498=CARTESIAN_POINT ( 'NONE',  ( -13.91666582400481644, 125.7699432187419575, -2.002145485623346932 ) ) ;
#9500=CARTESIAN_POINT ( 'NONE',  ( 5.683854215195817794, -15.08228171793801664, 1.486458664383613293 ) ) ;
#9503=ADVANCED_FACE ( 'NONE', ( #23418 ), #29249, .T. ) ;
#9505=CARTESIAN_POINT ( 'NONE',  ( 16.73131056987022092, 135.2943057719725459, 2.348795921478700865 ) ) ;
#9506=DIRECTION ( 'NONE',  ( -4.017660918040594346E-17, 1.000000000000000000, 2.376309959284834438E-19 ) ) ;
#9508=CARTESIAN_POINT ( 'NONE',  ( -0.2613516939666690186, 106.0087397856094356, 5.279363957283110587 ) ) ;
#9509=CARTESIAN_POINT ( 'NONE',  ( -8.368269197548203309, 31.49133049583987187, -0.7708832981534754492 ) ) ;
#9510=CARTESIAN_POINT ( 'NONE',  ( 16.05307823990497340, 146.0544122543811341, 1.176040581308522404 ) ) ;
#9511=CARTESIAN_POINT ( 'NONE',  ( 5.858194661467363673, 117.3723397083485622, -0.4592760973624643861 ) ) ;
#9514=EDGE_CURVE ( 'NONE', #23040, #38078, #8860, .T. ) ;
#9516=CARTESIAN_POINT ( 'NONE',  ( -0.0002734175339917587714, 159.6054662015457382, 0.01368293144939993107 ) ) ;
#9518=ORIENTED_EDGE ( 'NONE', *, *, #34479, .T. ) ;
#9519=CARTESIAN_POINT ( 'NONE',  ( -8.133793902695101607, 120.8064541497650310, -1.378343526931617102 ) ) ;
#9520=CARTESIAN_POINT ( 'NONE',  ( 23.36121599383890768, 148.8756354987169175, 0.4668126921610644131 ) ) ;
#9521=CARTESIAN_POINT ( 'NONE',  ( -7.977778825752325886, 154.6030710842251494, -0.7700301581992886613 ) ) ;
#9522=CARTESIAN_POINT ( 'NONE',  ( 4.143153066788715755, -13.73528615761443561, 4.025237717645509861 ) ) ;
#9523=CARTESIAN_POINT ( 'NONE',  ( 7.002510704594238966, 121.9568449727899520, 0.1399268299516837899 ) ) ;
#9524=CARTESIAN_POINT ( 'NONE',  ( 3.706843470526773654, 116.6237204831772232, 0.08772160974583174953 ) ) ;
#9526=CARTESIAN_POINT ( 'NONE',  ( 4.326043401919948295, 8.289558097378858292, -1.648119079657388353 ) ) ;
#9527=CARTESIAN_POINT ( 'NONE',  ( -23.29144772315980916, 149.3526176766912101, -0.4654185560736369132 ) ) ;
#9529=CARTESIAN_POINT ( 'NONE',  ( 5.157440735887882433, 114.7154655033523198, 1.455969569964357557 ) ) ;
#9530=CARTESIAN_POINT ( 'NONE',  ( 6.105266827213309710, 121.0439321044046039, 0.7736761210806879507 ) ) ;
#9531=CARTESIAN_POINT ( 'NONE',  ( -1.889208318266999198, 10.27326514537015534, 4.227218769941996968 ) ) ;
#9532=CARTESIAN_POINT ( 'NONE',  ( 14.71083544318249281, 121.0688405154646858, 1.213083844406488199 ) ) ;
#9534=CARTESIAN_POINT ( 'NONE',  ( 2.943565496889787525, 108.2627120386935502, 4.302928841461297615 ) ) ;
#9535=CARTESIAN_POINT ( 'NONE',  ( 1.161715739485780885, 117.9723128000925669, -0.5854012653586093684 ) ) ;
#9536=CARTESIAN_POINT ( 'NONE',  ( 3.363087486136625337, 4.875765145370108300, -3.182472177310056605 ) ) ;
#9537=CARTESIAN_POINT ( 'NONE',  ( -13.11470433356391929, 119.8381915656929380, -0.9809890993017411631 ) ) ;
#9538=VERTEX_POINT ( 'NONE', #15306 ) ;
#9539=CARTESIAN_POINT ( 'NONE',  ( -5.903620821223855231, 121.4229528491920576, 0.1845582724821507592 ) ) ;
#9540=CARTESIAN_POINT ( 'NONE',  ( 6.072898904334845582, -12.55662260458653634, 0.7994981368886315831 ) ) ;
#9543=CARTESIAN_POINT ( 'NONE',  ( -4.593215935933216088, 118.0632729301879920, -0.7325469166207362326 ) ) ;
#9544=CARTESIAN_POINT ( 'NONE',  ( 11.83770080265064983, 152.0103986367769551, 0.1887002032782131022 ) ) ;
#9546=CARTESIAN_POINT ( 'NONE',  ( 0.4459748878572474817, 118.5593716040226724, 0.6139719676240720236 ) ) ;
#9549=CARTESIAN_POINT ( 'NONE',  ( -4.852593915752414055, 117.2114307359545649, 0.4396237197203591296 ) ) ;
#9551=CARTESIAN_POINT ( 'NONE',  ( 15.39314341005339948, 120.8297411738997624, -0.1127201291141931155 ) ) ;
#9552=EDGE_CURVE ( 'NONE', #13530, #450, #8515, .T. ) ;
#9558=ADVANCED_FACE ( 'NONE', ( #12335 ), #1720, .T. ) ;
#9561=CARTESIAN_POINT ( 'NONE',  ( -4.632005028902471011, 118.0396561689580324, 0.6218044277692786892 ) ) ;
#9563=B_SPLINE_SURFACE_WITH_KNOTS ( 'NONE', 1, 3, ( 
 ( #19555, #16580, #35564, #18934, #9361, #15946, #38756, #29371, #6798, #9161, #28943, #3617, #9566, #22118, #35772, #39174, #32564, #6382 ),
 ( #3398, #16365, #13185, #210, #31943, #25545, #32358, #41755, #2781, #9981, #19766, #15737, #22955, #35982, #28741, #29798, #10193, #23380 ) ),
 .UNSPECIFIED., .F., .F., .F.,
 ( 2, 2 ),
 ( 4, 2, 2, 2, 2, 2, 2, 2, 4 ),
 ( 0.000000000000000000, 1.000000000000000000 ),
 ( 0.000000000000000000, 0.06250000000000000000, 0.1250000000000000000, 0.1875000000000000000, 0.2500000000000000000, 0.3750000000000000000, 0.5000000000000000000, 0.7500000000000000000, 1.000000000000000000 ),
 .UNSPECIFIED. ) ;
#9566=CARTESIAN_POINT ( 'NONE',  ( -2.186492930797574452, 115.6909491485466646, -1.711433661021510177 ) ) ;
#9567=CARTESIAN_POINT ( 'NONE',  ( -5.931588090995600027, 119.1690655882911329, -1.264883306644118743 ) ) ;
#9568=CARTESIAN_POINT ( 'NONE',  ( -1.966029823418521172, 106.7001829816230725, -4.962286218837188123 ) ) ;
#9570=CARTESIAN_POINT ( 'NONE',  ( 4.742030083010273955, 117.8490966506599307, 0.9897493978187200669 ) ) ;
#9571=CARTESIAN_POINT ( 'NONE',  ( 2.969447359227861405, -13.80100253337253946, 0.9847735008004718793 ) ) ;
#9572=CARTESIAN_POINT ( 'NONE',  ( -15.17477609654696380, 139.4722935914273307, -1.590378199732649600 ) ) ;
#9573=CARTESIAN_POINT ( 'NONE',  ( -2.528362934948840124, 115.7031097563144471, -1.694662335315127777 ) ) ;
#9574=CARTESIAN_POINT ( 'NONE',  ( -3.523571992936364694, 109.1382962752385026, 3.814013227644438064 ) ) ;
#9576=CARTESIAN_POINT ( 'NONE',  ( 2.658992269297059785, 107.2388417251876547, -4.621886736208384860 ) ) ;
#9577=CARTESIAN_POINT ( 'NONE',  ( -17.04317705290392837, 148.4623951536435698, -2.145728921095965358 ) ) ;
#9579=CARTESIAN_POINT ( 'NONE',  ( -0.03067001211942338088, 158.6015251912307633, 1.534852821454057770 ) ) ;
#9580=CARTESIAN_POINT ( 'NONE',  ( -3.399038284204972449, 115.7029691290877906, 1.510463350574593022 ) ) ;
#9581=CARTESIAN_POINT ( 'NONE',  ( -1.214995109038484067, 0.9429784454696930052, -4.460028654918597901 ) ) ;
#9582=CARTESIAN_POINT ( 'NONE',  ( 10.62864291685173512, 157.9324367681937815, 0.7848347606368001328 ) ) ;
#9585=CARTESIAN_POINT ( 'NONE',  ( 3.162278034637682200, -15.50568859125470134, 4.121945908858189789 ) ) ;
#9586=CARTESIAN_POINT ( 'NONE',  ( -19.59580906854019844, 147.4874203640471535, 1.738765900131762798 ) ) ;
#9587=CARTESIAN_POINT ( 'NONE',  ( 0.4410767147925211407, 14.17415678908661469, -0.8685042294053136880 ) ) ;
#9588=CARTESIAN_POINT ( 'NONE',  ( 0.9048393610272945642, 9.142100508531621372, -0.3649321582425499311 ) ) ;
#9590=EDGE_LOOP ( 'NONE', ( #6538, #30234 ) ) ;
#9591=CARTESIAN_POINT ( 'NONE',  ( -4.854186777038641765, 117.7557277303023966, -0.9091791526384296329 ) ) ;
#9592=CARTESIAN_POINT ( 'NONE',  ( 4.672526732406415029, 120.2198808273567892, 0.4623614190293561799 ) ) ;
#9594=CARTESIAN_POINT ( 'NONE',  ( -9.503290916781066855, 123.5188755717998816, 0.5781397488420940700 ) ) ;
#9595=CARTESIAN_POINT ( 'NONE',  ( 3.564576864782785570, -14.06793500455072454, 4.479818044377421593 ) ) ;
#9596=CARTESIAN_POINT ( 'NONE',  ( 14.72636943223149331, 131.2156652454908112, -1.433095336252469654 ) ) ;
#9597=CARTESIAN_POINT ( 'NONE',  ( -2.460791562519598408, 158.0185616612000956, -1.723846131599015230 ) ) ;
#9600=CARTESIAN_POINT ( 'NONE',  ( 8.744610207651122735, 117.8906195244964152, 0.6684397885285150442 ) ) ;
#9601=CARTESIAN_POINT ( 'NONE',  ( -0.4214665657712599045, 37.86644440679212664, 0.8455140659468449726 ) ) ;
#9602=CARTESIAN_POINT ( 'NONE',  ( 7.598614292646840518, 122.4062900713904440, -0.04802449110505816604 ) ) ;
#9604=CARTESIAN_POINT ( 'NONE',  ( -6.651972016613293606E-14, 104.1064662015457287, 7.011588703784780528E-31 ) ) ;
#9607=CARTESIAN_POINT ( 'NONE',  ( 5.028190701329536161, 117.3993840585409316, -0.6260521898566507870 ) ) ;
#9608=CARTESIAN_POINT ( 'NONE',  ( 4.636268038904784561, 155.9604050671876792, 1.079575001969329096 ) ) ;
#9610=CARTESIAN_POINT ( 'NONE',  ( 0.3042766021092446760, 116.4832816433156069, -0.08781055504204327011 ) ) ;
#9611=CARTESIAN_POINT ( 'NONE',  ( -5.434281097240536873, 117.1681999988027911, 0.6838767007579790169 ) ) ;
#9612=CARTESIAN_POINT ( 'NONE',  ( -5.078986093043186045, 92.04146620154574521, -0.1014902294541237954 ) ) ;
#9614=CARTESIAN_POINT ( 'NONE',  ( -4.847303688887219408, 31.57325935411374473, -0.5121714807418957793 ) ) ;
#9615=EDGE_CURVE ( 'NONE', #23143, #17052, #41527, .T. ) ;
#9616=CARTESIAN_POINT ( 'NONE',  ( 21.01875934457253692, 148.7375953542188256, 2.355668865594947370 ) ) ;
#9617=CARTESIAN_POINT ( 'NONE',  ( 1.677595020332960152, 24.74158224480939339, -4.309653081027373211 ) ) ;
#9618=CARTESIAN_POINT ( 'NONE',  ( -8.384998746481384657, -10.44493509673469767, 0.7792886224267949746 ) ) ;
#9619=CARTESIAN_POINT ( 'NONE',  ( -8.725233207679389480, 117.9832267607160929, -0.7526383660895783478 ) ) ;
#9620=CARTESIAN_POINT ( 'NONE',  ( -2.328338358121225582, 124.8000875644994068, -0.05398387088914113896 ) ) ;
#9621=CARTESIAN_POINT ( 'NONE',  ( -23.21373371908098449, 149.6306211361744829, -0.4638656453230912136 ) ) ;
#9622=CARTESIAN_POINT ( 'NONE',  ( 1.958559173108875173, 106.7079595946689494, -4.892068575404730169 ) ) ;
#9623=CARTESIAN_POINT ( 'NONE',  ( 2.359926926834857941, 104.6144662015456817, 4.210384773563669469 ) ) ;
#9625=CARTESIAN_POINT ( 'NONE',  ( 3.548611814566905664, 16.26088872207684943, 2.983771105379771971 ) ) ;
#9628=CARTESIAN_POINT ( 'NONE',  ( 2.967701212693483193, -13.54563334627871463, 1.070011838909553425 ) ) ;
#9629=CARTESIAN_POINT ( 'NONE',  ( 1.979347617175751806, 122.1523088006674840, -0.1944583918105483034 ) ) ;
#9630=CARTESIAN_POINT ( 'NONE',  ( -9.649066847268132463, 118.2334930433176652, 0.3843608719459137291 ) ) ;
#9631=ORIENTED_EDGE ( 'NONE', *, *, #17811, .T. ) ;
#9635=CARTESIAN_POINT ( 'NONE',  ( 2.047221892555406431, -15.65848914036231676, 5.808978358897256555 ) ) ;
#9636=CARTESIAN_POINT ( 'NONE',  ( -13.37375235405036378, 122.3357896625302459, 1.257830042033918350 ) ) ;
#9637=CARTESIAN_POINT ( 'NONE',  ( 19.57327063168399306, 152.2820370773569323, -1.161482255138347686 ) ) ;
#9638=CARTESIAN_POINT ( 'NONE',  ( 3.501419995798253915, -2.955197114699519734, 3.043391175950921568 ) ) ;
#9643=CARTESIAN_POINT ( 'NONE',  ( -0.01331772329000604355, 119.9741034315943864, 0.6664733318051297983 ) ) ;
#9644=CARTESIAN_POINT ( 'NONE',  ( -10.60072409500466861, 154.2769816202975051, 1.465916755537046479 ) ) ;
#9646=CARTESIAN_POINT ( 'NONE',  ( 12.07275429247921039, 123.1955650103826798, -1.290935347410189227 ) ) ;
#9647=CARTESIAN_POINT ( 'NONE',  ( -14.62144676724406089, 123.3142630313093377, -1.799443978378394648 ) ) ;
#9650=CARTESIAN_POINT ( 'NONE',  ( 4.439712258926299171, 118.1647990948395233, -0.4552782637668283394 ) ) ;
#9651=CARTESIAN_POINT ( 'NONE',  ( 12.22709855250464450, 151.9982576965888654, -0.6666368699087850125 ) ) ;
#9653=CARTESIAN_POINT ( 'NONE',  ( 0.009513407573613850629, 119.7614543879625586, -0.4760898169610155994 ) ) ;
#9654=CARTESIAN_POINT ( 'NONE',  ( 3.824421424077324883, -15.38127155850414773, 2.203493915304267858 ) ) ;
#9656=DIRECTION ( 'NONE',  ( -0.01997839162482761832, -1.040247600000951803E-18, 0.9998004120163610509 ) ) ;
#9659=CARTESIAN_POINT ( 'NONE',  ( -4.766718869283322668, 117.7281659001820913, 0.9070997928662917209 ) ) ;
#9660=CARTESIAN_POINT ( 'NONE',  ( 5.087176912069779178, 120.2090573957402455, 0.9271508619376561677 ) ) ;
#9663=CARTESIAN_POINT ( 'NONE',  ( 3.211436584971100849, 28.15539441671475274, -3.345526564039049688 ) ) ;
#9664=CARTESIAN_POINT ( 'NONE',  ( 6.489379754819697865, 121.7611753534313550, 0.2571143975131358617 ) ) ;
#9672=DIRECTION ( 'NONE',  ( -0.03103328369512481019, -0.9876883405951375483, 0.1533253963162051758 ) ) ;
#9677=ADVANCED_FACE ( 'NONE', ( #17874 ), #19718, .T. ) ;
#9678=CARTESIAN_POINT ( 'NONE',  ( -9.765169485063884380, 118.0373187826741486, 0.07890504670268488896 ) ) ;
#9681=CARTESIAN_POINT ( 'NONE',  ( -6.020519723803437806, 121.4387767156620015, -0.1661333497277762139 ) ) ;
#9683=CARTESIAN_POINT ( 'NONE',  ( 3.034504105865374779, 115.7029491485452581, -1.550851629826452083 ) ) ;
#9684=CARTESIAN_POINT ( 'NONE',  ( -15.27574012874729981, 148.0141687878753203, -0.5334971086861884926 ) ) ;
#9685=CARTESIAN_POINT ( 'NONE',  ( 4.517131889307780312, -14.80175198191645336, 4.712020298053779754 ) ) ;
#9686=CARTESIAN_POINT ( 'NONE',  ( -4.003603038177978135, 117.7793252414215317, 0.6798483224588710572 ) ) ;
#9688=CARTESIAN_POINT ( 'NONE',  ( -0.002426349801211070533, 116.5266044092193880, 0.1214244658147705658 ) ) ;
#9689=CARTESIAN_POINT ( 'NONE',  ( 11.82936742863723723, 152.0434717972437682, 0.3612672141402942239 ) ) ;
#9691=CARTESIAN_POINT ( 'NONE',  ( -0.9745549951769645336, 13.24125360461694001, -0.07243667530571006041 ) ) ;
#9692=CARTESIAN_POINT ( 'NONE',  ( -8.055701656131645905, 158.6724238832827609, -0.2706798611393587684 ) ) ;
#9694=FACE_OUTER_BOUND ( 'NONE', #38150, .T. ) ;
#9695=ORIENTED_EDGE ( 'NONE', *, *, #15927, .F. ) ;
#9696=CARTESIAN_POINT ( 'NONE',  ( -2.319837389150895213, 116.4337650663298973, 0.2360035357957355751 ) ) ;
#9697=ORIENTED_EDGE ( 'NONE', *, *, #39980, .T. ) ;
#9700=CARTESIAN_POINT ( 'NONE',  ( 6.809904206821519423, 118.2876074772933492, 1.086328812139343070 ) ) ;
#9701=CARTESIAN_POINT ( 'NONE',  ( 2.301458206243025550, 118.5910164976458532, -0.7067537174111423459 ) ) ;
#9702=CARTESIAN_POINT ( 'NONE',  ( 0.7350785369229140276, 15.66647056970591301, -8.407117359194836936 ) ) ;
#9703=CARTESIAN_POINT ( 'NONE',  ( -0.3765078121169122549, 117.5049145548240972, -0.4786851384288721700 ) ) ;
#9704=CARTESIAN_POINT ( 'NONE',  ( 4.777070507844503489, 117.8483530557036687, -0.7998628223812204174 ) ) ;
#9708=CARTESIAN_POINT ( 'NONE',  ( -7.788912029362665024, 154.6472212274131550, -0.1129171994251847999 ) ) ;
#9710=CARTESIAN_POINT ( 'NONE',  ( -0.9451225546581241144, 157.6350123088122359, -1.628263479412583647 ) ) ;
#9711=CARTESIAN_POINT ( 'NONE',  ( 5.875553665316252783, -14.89341971632543427, 0.3075322240006022056 ) ) ;
#9712=CARTESIAN_POINT ( 'NONE',  ( 4.787316872900306386, 118.5931160184169073, 0.9404912388413474433 ) ) ;
#9713=ADVANCED_FACE ( 'NONE', ( #38117 ), #25839, .T. ) ;
#9715=VERTEX_POINT ( 'NONE', #31500 ) ;
#9716=CARTESIAN_POINT ( 'NONE',  ( 15.37772490044519280, 131.3329289045130679, 2.176645470406190608 ) ) ;
#9720=CARTESIAN_POINT ( 'NONE',  ( -4.687267571634002650, 120.2198808273567892, 0.2753304537621713011 ) ) ;
#9721=CARTESIAN_POINT ( 'NONE',  ( 5.686328549477039473, -14.11678386645415628, -6.209864621142330954 ) ) ;
#9722=CARTESIAN_POINT ( 'NONE',  ( -0.009747742627877935620, 156.3581291470199233, 0.4878169013068173743 ) ) ;
#9723=CARTESIAN_POINT ( 'NONE',  ( 22.87957784423531749, 146.5373477140321938, -0.6332847025415451192 ) ) ;
#9726=CIRCLE ( 'NONE', #2267, 5.080000000000006288 ) ;
#9728=CARTESIAN_POINT ( 'NONE',  ( -22.66443576792692838, 150.6395781703034231, -0.4273611094724394932 ) ) ;
#9730=CARTESIAN_POINT ( 'NONE',  ( -6.306168215838764191, 119.9765817188901451, -1.212549642329949995 ) ) ;
#9732=CARTESIAN_POINT ( 'NONE',  ( -3.002817136647321306, 156.1079525116674631, -0.5547493173044985015 ) ) ;
#9733=CARTESIAN_POINT ( 'NONE',  ( 4.310348487322937849, -12.41951052373176090, 1.878555342735434230 ) ) ;
#9734=CARTESIAN_POINT ( 'NONE',  ( -5.036351857865265735, 117.3993844875897139, 0.5494637324817667201 ) ) ;
#9735=CARTESIAN_POINT ( 'NONE',  ( 22.98488057257191741, 150.1591296352320910, 0.4592926148156237232 ) ) ;
#9737=CARTESIAN_POINT ( 'NONE',  ( 4.617411384770501392, 7.639850289152962048, 0.2838591255797697777 ) ) ;
#9738=CARTESIAN_POINT ( 'NONE',  ( -4.023493262646688606, 105.1225664206005916, 3.517815851256813175 ) ) ;
#9741=EDGE_CURVE ( 'NONE', #38260, #12162, #27466, .T. ) ;
#9742=CARTESIAN_POINT ( 'NONE',  ( 6.996320709379100222, 121.7437260403137884, 0.6222143296915167987 ) ) ;
#9743=CARTESIAN_POINT ( 'NONE',  ( -4.556395268149300293, 8.773967715207941609, 0.7749943352582737699 ) ) ;
#9744=CARTESIAN_POINT ( 'NONE',  ( 3.876365344914114441, 117.1932757116604762, 0.6224469224293306402 ) ) ;
#9745=CARTESIAN_POINT ( 'NONE',  ( -0.05238710762259597004, 113.0327356262574341, 2.621665085262795625 ) ) ;
#9747=CARTESIAN_POINT ( 'NONE',  ( 21.17963693554076343, 147.9292434580435724, -1.516351520135284625 ) ) ;
#9748=TOROIDAL_SURFACE ( 'NONE', #12453, 3.683000000000000718, 0.5080000000000000071 ) ;
#9749=CARTESIAN_POINT ( 'NONE',  ( 0.4327634382839667393, 5.975216699623357108, -4.620561613140377055 ) ) ;
#9750=CARTESIAN_POINT ( 'NONE',  ( -21.41027608214069389, 151.3201912522522719, -1.490379992046949820 ) ) ;
#9753=CARTESIAN_POINT ( 'NONE',  ( -10.50161782422445711, 126.1106773019354819, 0.1489875947030159797 ) ) ;
#9755=CARTESIAN_POINT ( 'NONE',  ( 4.978007909399718045, -14.21992039213325398, 4.057701602070913793 ) ) ;
#9760=CARTESIAN_POINT ( 'NONE',  ( 5.837434872614966963, 119.2401804501882197, 1.198870938642750739 ) ) ;
#9763=CARTESIAN_POINT ( 'NONE',  ( -20.57308965805804846, 132.2049894596293313, 0.6677571715933803276 ) ) ;
#9764=CARTESIAN_POINT ( 'NONE',  ( 0.9434990333792051542, 116.6346273530297850, -0.1892539897508099256 ) ) ;
#9767=CARTESIAN_POINT ( 'NONE',  ( -5.009703114190266149, 117.5236796697281392, 0.6160668906261116406 ) ) ;
#9769=CARTESIAN_POINT ( 'NONE',  ( 1.984180638160394139, -15.05580698533026762, 5.708628072855972846 ) ) ;
#9772=CARTESIAN_POINT ( 'NONE',  ( -4.622025190417427432, 118.0615168869452134, 0.5436107810192618572 ) ) ;
#9776=CARTESIAN_POINT ( 'NONE',  ( 8.421875265154783463, 119.6416590919781697, -1.085143561374857457 ) ) ;
#9777=CARTESIAN_POINT ( 'NONE',  ( -5.148946675964053199, 115.4673366222922368, -1.510641186666999980 ) ) ;
#9778=CARTESIAN_POINT ( 'NONE',  ( 4.656206823194031230, 117.8897762713785227, 0.9969127701094048222 ) ) ;
#9779=CARTESIAN_POINT ( 'NONE',  ( 1.824656174747253168, -15.25388738520313225, 5.420764384989097628 ) ) ;
#9780=CARTESIAN_POINT ( 'NONE',  ( -7.125042791937310938, 121.7184703992695773, -0.7630849752878293701 ) ) ;
#9783=CARTESIAN_POINT ( 'NONE',  ( 6.519249125050485816, 120.6419738463991536, -0.1350556763279781858 ) ) ;
#9784=CARTESIAN_POINT ( 'NONE',  ( -14.69551782889057279, 134.6798445586954927, -1.826766161810339018 ) ) ;
#9785=CARTESIAN_POINT ( 'NONE',  ( 4.808131379915037584, 104.6144662015457527, -0.4149153341867691802 ) ) ;
#9786=CARTESIAN_POINT ( 'NONE',  ( -0.02156534543299366835, 156.6359106937186709, 1.079218069903262744 ) ) ;
#9788=CARTESIAN_POINT ( 'NONE',  ( -11.83487444615315098, 152.0315182889855521, -0.1740310882773943024 ) ) ;
#9789=CARTESIAN_POINT ( 'NONE',  ( 4.114294302962228755, -10.72644468530807416, -2.136776772127288559 ) ) ;
#9790=CARTESIAN_POINT ( 'NONE',  ( 1.374325311229910307, 159.5643428290674990, 0.4556871491110247585 ) ) ;
#9791=ORIENTED_EDGE ( 'NONE', *, *, #38673, .T. ) ;
#9792=CARTESIAN_POINT ( 'NONE',  ( 5.218897159788115303, 104.6144662015501581, -1.155893325450091380 ) ) ;
#9794=CARTESIAN_POINT ( 'NONE',  ( 2.845230715667840027, -15.32736664957809403, 4.381646938852296280 ) ) ;
#9796=CARTESIAN_POINT ( 'NONE',  ( -13.42639911875441605, 154.0568829568526041, 1.747011766586976877 ) ) ;
#9797=CARTESIAN_POINT ( 'NONE',  ( 0.3889013835376298744, 10.72134676413487142, 0.8939893681288630933 ) ) ;
#9798=CARTESIAN_POINT ( 'NONE',  ( -8.168866085573604607, 117.6493956690293317, -0.5746791023534235654 ) ) ;
#9799=CARTESIAN_POINT ( 'NONE',  ( -0.2932310942476468174, 5.691741097161698626, 0.9303163870417268111 ) ) ;
#9800=VERTEX_POINT ( 'NONE', #6161 ) ;
#9801=EDGE_LOOP ( 'NONE', ( #26149, #39152 ) ) ;
#9803=CARTESIAN_POINT ( 'NONE',  ( 5.714359084451690940, 118.4654530710369329, 0.6612863029850992724 ) ) ;
#9805=CARTESIAN_POINT ( 'NONE',  ( -8.389933090069352062, 122.6561726160659731, 0.4454891811124967460 ) ) ;
#9806=CARTESIAN_POINT ( 'NONE',  ( 3.930318996895993955, -12.97851325427171254, 2.595110522791146401 ) ) ;
#9807=CARTESIAN_POINT ( 'NONE',  ( 0.8914275061359997476, 157.0053619834820324, -1.381823885352171377 ) ) ;
#9809=CARTESIAN_POINT ( 'NONE',  ( -12.94126367519716325, 122.7019651155717384, -1.840448779276435687 ) ) ;
#9810=FACE_OUTER_BOUND ( 'NONE', #38219, .T. ) ;
#9812=CARTESIAN_POINT ( 'NONE',  ( 8.158625645752934474, 120.6838676416457048, 1.398799808874931827 ) ) ;
#9813=CARTESIAN_POINT ( 'NONE',  ( -3.430556142055666058, 34.24929622306240162, 1.944567991137617247 ) ) ;
#9814=CARTESIAN_POINT ( 'NONE',  ( 11.25890738108741296, 128.1602342495223468, -0.05278459517149993591 ) ) ;
#9815=ORIENTED_EDGE ( 'NONE', *, *, #23848, .T. ) ;
#9816=DIRECTION ( 'NONE',  ( 5.206863593109713661E-17, -1.000000000000000000, 1.077750396879097183E-30 ) ) ;
#9820=CARTESIAN_POINT ( 'NONE',  ( 22.65966732694881358, 150.6414900647796173, 0.2998287813802534285 ) ) ;
#9821=CARTESIAN_POINT ( 'NONE',  ( -4.844936406558586484, 112.7696648386057632, 2.375766922042533036 ) ) ;
#9822=DIRECTION ( 'NONE',  ( -0.9998004120163608288, 0.000000000000000000, -0.01997839162482747608 ) ) ;
#9823=CARTESIAN_POINT ( 'NONE',  ( -6.540217103314379345E-14, 82.64346620154573486, 2.383338306179204368E-29 ) ) ;
#9824=CARTESIAN_POINT ( 'NONE',  ( -5.176850267262477878, 31.60528704468920580, -0.07969122161898606338 ) ) ;
#9825=CARTESIAN_POINT ( 'NONE',  ( 1.137402291071409444, 117.9723128000925669, 0.6313431152059614249 ) ) ;
#9826=CARTESIAN_POINT ( 'NONE',  ( 2.029292378383023898, 15.02103924000656043, -4.168288449772576065 ) ) ;
#9827=CARTESIAN_POINT ( 'NONE',  ( 1.249529592346430240, 29.00528243095578063, -8.330927077797271707 ) ) ;
#9828=CARTESIAN_POINT ( 'NONE',  ( 5.510702963104994190, 117.2606150369192477, -0.6137602300856868087 ) ) ;
#9829=CARTESIAN_POINT ( 'NONE',  ( -1.618304973946187664, 119.5945091202099348, -0.6420790694971422186 ) ) ;
#9832=CARTESIAN_POINT ( 'NONE',  ( 1.041310694616567556, 104.6144662015456817, 4.721824807668626889 ) ) ;
#9833=CARTESIAN_POINT ( 'NONE',  ( 0.4746723515649934888, 24.68197512780947278, 4.609222710213416896 ) ) ;
#9834=DIRECTION ( 'NONE',  ( -0.01997839162482749689, -1.040247600000944870E-18, 0.9998004120163610509 ) ) ;
#9835=CARTESIAN_POINT ( 'NONE',  ( -15.47023807670837314, 120.6682698389898434, -0.3091321738930619678 ) ) ;
#9836=CARTESIAN_POINT ( 'NONE',  ( 2.663950356258127705, -13.19741034273377878, 0.1528337951401303463 ) ) ;
#9837=CARTESIAN_POINT ( 'NONE',  ( 3.079316153087777508, 123.1875568577169560, -0.05586128712921770156 ) ) ;
#9838=CARTESIAN_POINT ( 'NONE',  ( -15.09612904044937487, 120.9194639129320734, 0.3833380168901106555 ) ) ;
#9843=CARTESIAN_POINT ( 'NONE',  ( 6.046978665186544255, -14.69723126592269224, 0.3844556930898083702 ) ) ;
#9844=CARTESIAN_POINT ( 'NONE',  ( -18.00466200016603580, 151.7072807693909340, 1.676127293294198850 ) ) ;
#9845=CARTESIAN_POINT ( 'NONE',  ( 7.282534483022669036, 158.3006260280594404, -1.262407574188499026 ) ) ;
#9846=CARTESIAN_POINT ( 'NONE',  ( 0.3994026957563919789, 5.465888722076803319, 4.619092260001838923 ) ) ;
#9848=ORIENTED_EDGE ( 'NONE', *, *, #23204, .T. ) ;
#9850=CARTESIAN_POINT ( 'NONE',  ( 0.4207377039450588829, 124.6436471961814050, 0.04080923199211386465 ) ) ;
#9851=CARTESIAN_POINT ( 'NONE',  ( -16.99563481483670913, 148.6336825499269310, 1.463981761124606207 ) ) ;
#9853=CARTESIAN_POINT ( 'NONE',  ( 2.342076541036470783, 157.5529522918930638, -1.611985001046909005 ) ) ;
#9854=CARTESIAN_POINT ( 'NONE',  ( -13.73566407960812263, 122.1113760975138263, -1.718532046871276808 ) ) ;
#9857=CARTESIAN_POINT ( 'NONE',  ( 4.423891049316628354, 118.1653506322867173, -0.4723435439479501396 ) ) ;
#9858=CARTESIAN_POINT ( 'NONE',  ( 16.08279055836830906, 146.6973543426590254, -0.5313625374031879511 ) ) ;
#9860=CARTESIAN_POINT ( 'NONE',  ( -12.73281086834439257, 125.9836878220586556, -1.772748636948828782 ) ) ;
#9861=CARTESIAN_POINT ( 'NONE',  ( 3.418015357486716699, -15.48303273933827917, 3.654867857709153345 ) ) ;
#9862=CARTESIAN_POINT ( 'NONE',  ( -4.622786458448389091, 105.1214642455587978, -2.684754972049111732 ) ) ;
#9865=CARTESIAN_POINT ( 'NONE',  ( -4.773351466264551313, 117.6315869056820418, 0.9547913690014270260 ) ) ;
#9866=CARTESIAN_POINT ( 'NONE',  ( 17.50754485026800111, 146.9817191466759141, 2.164442782320840752 ) ) ;
#9868=CARTESIAN_POINT ( 'NONE',  ( 1.790774717077139089, 25.13178105314743860, 4.274281468382033822 ) ) ;
#9869=CARTESIAN_POINT ( 'NONE',  ( 15.27574012874717191, 148.0141687878753203, 0.5334971086861887146 ) ) ;
#9876=CARTESIAN_POINT ( 'NONE',  ( -8.762201071066225921, 117.8145929003731425, -0.5758305771568995590 ) ) ;
#9878=CARTESIAN_POINT ( 'NONE',  ( -4.074955089416341991, 118.2429491485453354, 0.1454234154749719787 ) ) ;
#9882=CARTESIAN_POINT ( 'NONE',  ( -0.3151558924359575409, 116.5752054743899038, 0.1523977429619430557 ) ) ;
#9883=ORIENTED_EDGE ( 'NONE', *, *, #2992, .T. ) ;
#9885=CARTESIAN_POINT ( 'NONE',  ( 6.970729396409415024, 121.9486231262834934, 0.03295389407336209164 ) ) ;
#9887=CARTESIAN_POINT ( 'NONE',  ( 3.613157353203237054, 115.7029504961088122, -1.483779985806342294 ) ) ;
#9888=CARTESIAN_POINT ( 'NONE',  ( -10.42406139656922548, 153.0845720789597522, -0.4157246174923901472 ) ) ;
#9889=CARTESIAN_POINT ( 'NONE',  ( 5.566531978545880222, -14.14111126781847361, 3.212028819027522797 ) ) ;
#9890=CARTESIAN_POINT ( 'NONE',  ( -3.062634247293312129, 117.6993298527280984, 0.6308921261198922048 ) ) ;
#9892=CARTESIAN_POINT ( 'NONE',  ( 1.404208078696223216, 159.5982469381528972, 0.2156159867753337234 ) ) ;
#9893=CARTESIAN_POINT ( 'NONE',  ( 5.325826159991753350, 121.3512792334589534, 0.1791233883900909540 ) ) ;
#9895=CARTESIAN_POINT ( 'NONE',  ( -0.9163883642843115851, 13.89126970375589032, 0.3362141533434955809 ) ) ;
#9896=CARTESIAN_POINT ( 'NONE',  ( -23.18927481933092594, 149.6199392087789306, -0.6935230913228406235 ) ) ;
#9901=CARTESIAN_POINT ( 'NONE',  ( -5.566147196004182618, 117.2876211984145698, 0.5856085228032834600 ) ) ;
#9904=CARTESIAN_POINT ( 'NONE',  ( 21.34910226488267782, 149.1985357531029308, 2.237902092811237864 ) ) ;
#9905=CARTESIAN_POINT ( 'NONE',  ( 17.46960851010910432, 131.6241255656270255, -1.599527815159631716 ) ) ;
#9906=CARTESIAN_POINT ( 'NONE',  ( -0.6470182227010313758, 8.987660258844066163, 0.7316552229444387434 ) ) ;
#9907=CARTESIAN_POINT ( 'NONE',  ( 2.011605530963595623, 11.37297026005182587, 8.215081034461865883 ) ) ;
#9908=CARTESIAN_POINT ( 'NONE',  ( -5.110479671343788333, 158.7070047875298826, -1.445852496635407380 ) ) ;
#9909=CARTESIAN_POINT ( 'NONE',  ( 4.833421569118034888, 117.8347370731485597, -0.7197543954735053928 ) ) ;
#9911=CARTESIAN_POINT ( 'NONE',  ( -0.1065646865916381608, 105.8844662015456777, 5.332932678536313809 ) ) ;
#9912=ADVANCED_FACE ( 'NONE', ( #35966 ), #39160, .F. ) ;
#9913=CARTESIAN_POINT ( 'NONE',  ( 5.165015969722777989, 120.6777149489875569, -0.5489573293230838313 ) ) ;
#9914=CARTESIAN_POINT ( 'NONE',  ( -8.794423163103219920, 123.6850765633735421, -0.1423839433359066764 ) ) ;
#9916=CARTESIAN_POINT ( 'NONE',  ( -15.71196619591404620, 131.3838724160208926, -2.228970979916469197 ) ) ;
#9917=CARTESIAN_POINT ( 'NONE',  ( 2.810429210790068133, -15.63944505633836712, 5.584101034811558506 ) ) ;
#9919=CARTESIAN_POINT ( 'NONE',  ( -6.529493367164978770E-14, 72.99146620154573384, -7.899616498973244731E-18 ) ) ;
#9922=B_SPLINE_SURFACE_WITH_KNOTS ( 'NONE', 3, 3, ( 
 ( #36739, #10536, #33337, #26729, #4167, #7562 ),
 ( #20736, #3960, #39946, #30330, #30546, #30131 ),
 ( #760, #23505, #17130, #27143, #33760, #39521 ),
 ( #1385, #36532, #26515, #10740, #23936, #17341 ) ),
 .UNSPECIFIED., .F., .F., .F.,
 ( 4, 4 ),
 ( 4, 2, 4 ),
 ( 0.000000000000000000, 1.000000000000000000 ),
 ( 0.000000000000000000, 0.5000000000000000000, 1.000000000000000000 ),
 .UNSPECIFIED. ) ;
#9923=CARTESIAN_POINT ( 'NONE',  ( 17.40616913868953475, 140.3598469681121514, 2.385085200778920278 ) ) ;
#9925=CARTESIAN_POINT ( 'NONE',  ( -6.439947148575337965E-14, 116.4254662015457313, 1.493913655526859821E-16 ) ) ;
#9926=CARTESIAN_POINT ( 'NONE',  ( -1.389742127967517504, 109.2701902778323557, 3.915166117862841411 ) ) ;
#9927=CARTESIAN_POINT ( 'NONE',  ( 0.2611430735369592582, 24.48315862702271417, 8.432237392808469068 ) ) ;
#9928=CARTESIAN_POINT ( 'NONE',  ( 9.499123264218818363, 124.0643708016488063, 0.7086372128104245771 ) ) ;
#9930=CARTESIAN_POINT ( 'NONE',  ( 16.46484310285434205, 122.7513851185756693, -0.4780162726406276819 ) ) ;
#9932=CARTESIAN_POINT ( 'NONE',  ( 6.475684456959278634, -13.49251406434824574, 0.1304084665236045215 ) ) ;
#9934=CARTESIAN_POINT ( 'NONE',  ( -10.83330528665015891, 157.8980211815716928, -0.2164752214609687586 ) ) ;
#9935=EDGE_LOOP ( 'NONE', ( #7924, #8848, #37061, #15277 ) ) ;
#9936=CARTESIAN_POINT ( 'NONE',  ( -7.991460488516994864, 121.5207739338980275, -1.170844661440724632 ) ) ;
#9937=CARTESIAN_POINT ( 'NONE',  ( 4.984401644025001410, -14.86135559163349384, 4.129797103419615922 ) ) ;
#9938=CARTESIAN_POINT ( 'NONE',  ( -11.46436990449512727, 128.2561452373498980, -0.7395913538610450200 ) ) ;
#9939=CARTESIAN_POINT ( 'NONE',  ( 2.668130780779813360, -14.68804970414791455, 5.313657848291281738 ) ) ;
#9940=CARTESIAN_POINT ( 'NONE',  ( -6.564189886853176475E-14, 81.62746620154572952, -5.847435218134868453E-18 ) ) ;
#9941=CARTESIAN_POINT ( 'NONE',  ( 21.68875320759051917, 132.7412702629105468, 0.4333929054516009183 ) ) ;
#9943=CARTESIAN_POINT ( 'NONE',  ( -4.609222696788063622, 3.091975128091568159, 0.4746723485708761459 ) ) ;
#9944=CARTESIAN_POINT ( 'NONE',  ( 5.287133221413552242, 105.1224873763950143, 0.7811871516068193966 ) ) ;
#9945=CARTESIAN_POINT ( 'NONE',  ( -4.902043024275339000, 117.4095900847628826, 0.9678312229368277730 ) ) ;
#9946=CARTESIAN_POINT ( 'NONE',  ( 4.403693129465371392, 110.7916611705323504, 3.072783695400131521 ) ) ;
#9947=CARTESIAN_POINT ( 'NONE',  ( 6.990161945763603057, 121.8758651151647854, 0.4345305272952283415 ) ) ;
#9948=CARTESIAN_POINT ( 'NONE',  ( -3.984361711520921556, 7.699456178644025428, -2.362637291489932068 ) ) ;
#9949=CARTESIAN_POINT ( 'NONE',  ( 11.19826879832059241, 119.1264784044212632, 1.044736191152864313 ) ) ;
#9951=CARTESIAN_POINT ( 'NONE',  ( 2.116451952768004130, 107.0587250333981615, 4.811125309486601331 ) ) ;
#9952=CARTESIAN_POINT ( 'NONE',  ( 10.51304382037001162, 120.0128241960130424, -1.064055063733757134 ) ) ;
#9953=CARTESIAN_POINT ( 'NONE',  ( 4.623297697159335584, 3.588818502778304609, 0.3943307014320480697 ) ) ;
#9954=CARTESIAN_POINT ( 'NONE',  ( -21.93197806114495307, 150.5960492154097778, -1.608405794939391509 ) ) ;
#9956=ADVANCED_FACE ( 'NONE', ( #32340 ), #37208, .F. ) ;
#9959=CARTESIAN_POINT ( 'NONE',  ( -15.87385217746184729, 146.2799285973741519, 0.1369075966739885519 ) ) ;
#9960=CARTESIAN_POINT ( 'NONE',  ( 6.023256536641487635, -13.63339314725699225, 2.031454315062427796 ) ) ;
#9961=DIRECTION ( 'NONE',  ( 0.9998004120163608288, 0.000000000000000000, 0.01997839162482749342 ) ) ;
#9962=CARTESIAN_POINT ( 'NONE',  ( -2.894375511602795381, 107.8343606798795093, -4.471999567165577005 ) ) ;
#9965=CARTESIAN_POINT ( 'NONE',  ( 15.45413117217001542, 153.1703808545849483, 2.356132421238607222 ) ) ;
#9968=CARTESIAN_POINT ( 'NONE',  ( -14.68046753700562412, 156.0817623197167450, 0.7569547985229808651 ) ) ;
#9969=CARTESIAN_POINT ( 'NONE',  ( 8.004298179822232129, 158.6817341734954425, -0.1651967042931133389 ) ) ;
#9974=CARTESIAN_POINT ( 'NONE',  ( -4.757280042987765967, 117.4019780031357527, -1.206666893366715065 ) ) ;
#9977=CARTESIAN_POINT ( 'NONE',  ( -4.731020071145249695, 117.9657514467067472, 0.6165449125908130101 ) ) ;
#9981=CARTESIAN_POINT ( 'NONE',  ( -1.364642409907909748, 118.7629491485454167, -1.251955028465520980 ) ) ;
#9982=EDGE_CURVE ( 'NONE', #9488, #8589, #40011, .T. ) ;
#9983=CARTESIAN_POINT ( 'NONE',  ( -3.548838988669358319, 118.7219257611751857, -0.9358992106884462814 ) ) ;
#9984=CARTESIAN_POINT ( 'NONE',  ( -5.714359084451818838, 118.4654530710369329, -0.6612863029850992724 ) ) ;
#9985=CARTESIAN_POINT ( 'NONE',  ( 4.776791126193284498, 117.8777007509519024, 0.8660848876855279377 ) ) ;
#9987=CARTESIAN_POINT ( 'NONE',  ( -16.04436118421920199, 148.0691544347876345, -1.589228464704729005 ) ) ;
#9991=CARTESIAN_POINT ( 'NONE',  ( 7.643893061813482603, 124.7210964017841377, 0.1527835634684689414 ) ) ;
#9992=CARTESIAN_POINT ( 'NONE',  ( -16.79675997928907449, 147.6865045845431723, -1.918872074639297098 ) ) ;
#9994=CARTESIAN_POINT ( 'NONE',  ( -0.01341678693510457362, 156.4123495908283985, 0.6714308817992611367 ) ) ;
#9995=CARTESIAN_POINT ( 'NONE',  ( 7.862390625383989473, 122.3040693739171587, -0.4082539146964299648 ) ) ;
#9996=CARTESIAN_POINT ( 'NONE',  ( -15.20866760725288103, 143.4108773460236819, -0.2363331269315028793 ) ) ;
#9997=CARTESIAN_POINT ( 'NONE',  ( 2.551540157903699146, -0.3564265548712530207, -3.854280124997286450 ) ) ;
#9998=CARTESIAN_POINT ( 'NONE',  ( 22.36400590086632434, 150.5530013069706285, 1.293239838729947300 ) ) ;
#9999=ORIENTED_EDGE ( 'NONE', *, *, #28468, .F. ) ;
#10001=CARTESIAN_POINT ( 'NONE',  ( 3.395721326281507579, -14.88725931823228699, 0.4187095049187871121 ) ) ;
#10002=CARTESIAN_POINT ( 'NONE',  ( -0.03245814172817904769, 157.7902383798253538, 1.624338139048501883 ) ) ;
#10003=CARTESIAN_POINT ( 'NONE',  ( 0.8415213475290624912, 13.30065917492326122, -0.4928529130785159751 ) ) ;
#10004=CARTESIAN_POINT ( 'NONE',  ( -13.28278499026800752, 156.9705208988102640, -0.7618315876160809408 ) ) ;
#10005=VECTOR ( 'NONE', #12477, 1000.000000000000000 ) ;
#10006=CARTESIAN_POINT ( 'NONE',  ( 0.8610934044332675397, -11.37225059697985863, 0.4573394443077089533 ) ) ;
#10011=CARTESIAN_POINT ( 'NONE',  ( 5.397835693418270964, 119.2618716387835747, 0.5632668535983703650 ) ) ;
#10012=CARTESIAN_POINT ( 'NONE',  ( -15.71237885704647752, 143.6801599334541208, 0.6671153439278900699 ) ) ;
#10013=CARTESIAN_POINT ( 'NONE',  ( 2.527534073033691708, -14.76126024938119485, 5.399385249886175409 ) ) ;
#10014=CARTESIAN_POINT ( 'NONE',  ( 13.68689207195642332, 152.4534842159446271, -1.543072478675916459 ) ) ;
#10015=VECTOR ( 'NONE', #20543, 1000.000000000000227 ) ;
#10016=CARTESIAN_POINT ( 'NONE',  ( -6.695514854630728152, 119.3011930948910759, -1.284729283498812435 ) ) ;
#10017=CARTESIAN_POINT ( 'NONE',  ( -6.555005513994535572E-14, 79.34146620154574236, -6.390659674827382268E-18 ) ) ;
#10018=CARTESIAN_POINT ( 'NONE',  ( 2.829627719599027369, -13.65247383265987757, 0.5238048331051645690 ) ) ;
#10019=CARTESIAN_POINT ( 'NONE',  ( -5.860682609351126615, 31.62183355753281333, 2.274222983814665699 ) ) ;
#10020=CARTESIAN_POINT ( 'NONE',  ( 10.45649748849128713, 153.0728660266736370, -0.08902316335936723279 ) ) ;
#10022=ORIENTED_EDGE ( 'NONE', *, *, #10189, .T. ) ;
#10024=CARTESIAN_POINT ( 'NONE',  ( 0.4435697013598551841, 106.0197932915369847, 5.281582295280689898 ) ) ;
#10028=CARTESIAN_POINT ( 'NONE',  ( 15.19006826215911587, 156.0999766016731769, 0.2361313609475710340 ) ) ;
#10029=CARTESIAN_POINT ( 'NONE',  ( -5.498174961348694545, 117.5088849381099436, 0.6086507346144035546 ) ) ;
#10030=AXIS2_PLACEMENT_3D ( 'NONE', #9434, #12633, #16444 ) ;
#10031=DIRECTION ( 'NONE',  ( -0.9998004120163609398, 0.000000000000000000, -0.01997839162482749689 ) ) ;
#10033=CARTESIAN_POINT ( 'NONE',  ( -4.187219683869615849, 32.60936066482102547, 1.105729851008191877 ) ) ;
#10034=CARTESIAN_POINT ( 'NONE',  ( 13.40516742707908726, 121.5866728338796463, 1.646856811522066311 ) ) ;
#10035=CARTESIAN_POINT ( 'NONE',  ( -4.488006035213030209, 18.49445617864287073, 1.146732334616328286 ) ) ;
#10036=CARTESIAN_POINT ( 'NONE',  ( -7.485859564062662841, -11.32103332335322499, -3.896386919873200405 ) ) ;
#10037=CARTESIAN_POINT ( 'NONE',  ( 5.515726608291020128, 117.1379768558993817, -0.5451333893821521670 ) ) ;
#10038=CARTESIAN_POINT ( 'NONE',  ( -0.7127221660107545542, 117.6736730875354766, -1.182500608623780813 ) ) ;
#10040=CARTESIAN_POINT ( 'NONE',  ( -2.864695162364617076, 104.6144662015458096, 3.894373788996692287 ) ) ;
#10041=CARTESIAN_POINT ( 'NONE',  ( -4.420329592304260480, 21.65838872207745425, -1.398650104627336743 ) ) ;
#10045=CARTESIAN_POINT ( 'NONE',  ( 2.351750233177451133, -15.05367847713771923, 4.985144330900271648 ) ) ;
#10046=CARTESIAN_POINT ( 'NONE',  ( 2.822804308802433493, 121.9077826007922312, -0.1826741318641919576 ) ) ;
#10047=CARTESIAN_POINT ( 'NONE',  ( -0.3352962839985075827, 116.7787044104018861, 0.2500268678974715830 ) ) ;
#10049=CARTESIAN_POINT ( 'NONE',  ( 4.976171711130020547, 117.4097491279395626, -0.8839812355984283387 ) ) ;
#10050=ORIENTED_EDGE ( 'NONE', *, *, #41743, .F. ) ;
#10051=CARTESIAN_POINT ( 'NONE',  ( 5.008145224984434485, 117.3993836135855418, -0.7758584094373792706 ) ) ;
#10053=CARTESIAN_POINT ( 'NONE',  ( -5.274544067074300457, 115.7029491485454002, 0.8135768287290441325 ) ) ;
#10054=CARTESIAN_POINT ( 'NONE',  ( 3.756887254765235440, -15.74060793811991843, 4.623245420838687281 ) ) ;
#10055=CARTESIAN_POINT ( 'NONE',  ( -12.27107220260967857, 121.7247091083657153, 1.253333917061305147 ) ) ;
#10056=CARTESIAN_POINT ( 'NONE',  ( 15.58647730463667536, 154.9569273371780298, -1.293949759430877533 ) ) ;
#10057=CARTESIAN_POINT ( 'NONE',  ( 4.617411384770501392, 7.639850289152962048, 0.2838591255797697777 ) ) ;
#10060=CARTESIAN_POINT ( 'NONE',  ( -4.771056762337200219, 117.4047813638584188, -1.203986021773440385 ) ) ;
#10061=B_SPLINE_CURVE_WITH_KNOTS ( 'NONE', 3,
 ( #12394, #6013, #25583, #2191, #2402, #18342, #34559, #40947, #28368, #9398, #6218, #31136, #15148, #41158, #24740, #11964, #27940 ),
 .UNSPECIFIED., .F., .F.,
 ( 4, 1, 1, 1, 1, 1, 1, 1, 1, 1, 1, 1, 1, 1, 4 ),
 ( 0.000000000000000000, 0.08300113939718137268, 0.1732806554784933895, 0.2717672377176819087, 0.3752096606209606167, 0.4787223716043260135, 0.5772295444745598747, 0.6668133826162351285, 0.7470991451079272982, 0.7815930070524458317, 0.8169452614683294644, 0.8547689062991584708, 0.8968063284581728745, 0.9447228702782888288, 1.000000000000000000 ),
 .UNSPECIFIED. ) ;
#10062=CARTESIAN_POINT ( 'NONE',  ( 0.4574053846281739832, 111.1955024190080223, 3.269098021338873838 ) ) ;
#10063=CARTESIAN_POINT ( 'NONE',  ( -16.86000824444456470, 147.6865045845431723, 1.246329746872388622 ) ) ;
#10065=CARTESIAN_POINT ( 'NONE',  ( 2.279834263381187220, 157.4004113605966211, -1.585270110160261536 ) ) ;
#10066=CARTESIAN_POINT ( 'NONE',  ( -0.4162271216350219571, 118.1045761740670201, -0.5784513839558710346 ) ) ;
#10069=CARTESIAN_POINT ( 'NONE',  ( 4.525059116826507299, 118.1239383869072270, -0.4885259721435726288 ) ) ;
#10070=CARTESIAN_POINT ( 'NONE',  ( 15.77383231466688152, 147.9505201145231865, -0.6473862450635482491 ) ) ;
#10072=CARTESIAN_POINT ( 'NONE',  ( -5.836546232834304959, 120.2771794157441008, -1.045480238269852480 ) ) ;
#10073=CARTESIAN_POINT ( 'NONE',  ( 3.320832222217961593, -15.07605257934231702, 3.106094183260712516 ) ) ;
#10077=CARTESIAN_POINT ( 'NONE',  ( 3.750385610654966229, 4.675867361267946443, -2.714424430587211834 ) ) ;
#10078=CARTESIAN_POINT ( 'NONE',  ( 17.48541186233164879, 146.4615580561186050, 2.166240883089540770 ) ) ;
#10079=CARTESIAN_POINT ( 'NONE',  ( -2.633907558715006481, 30.44407049250143871, 0.6696650445282713582 ) ) ;
#10080=CARTESIAN_POINT ( 'NONE',  ( 3.740357457071568081, -9.854013591530623728, -7.545904704300070875 ) ) ;
#10081=CARTESIAN_POINT ( 'NONE',  ( 12.96905644698476223, 133.8854804328748571, 0.4775921230882992918 ) ) ;
#10082=CARTESIAN_POINT ( 'NONE',  ( -3.104076039314392244, 107.6120347158273631, 4.328431646495224605 ) ) ;
#10085=CARTESIAN_POINT ( 'NONE',  ( 21.90559427349721489, 151.4293160993572371, 0.4377259060014726533 ) ) ;
#10095=CARTESIAN_POINT ( 'NONE',  ( -20.66439279448300326, 152.5811724025633112, -0.09276230403812300851 ) ) ;
#10098=CARTESIAN_POINT ( 'NONE',  ( -6.054156888946658377, 121.4335526797924558, -0.1284449273526937774 ) ) ;
#10100=ORIENTED_EDGE ( 'NONE', *, *, #23999, .F. ) ;
#10102=CARTESIAN_POINT ( 'NONE',  ( -7.796516423212207059, 154.6345575486818404, -0.2631748570402914211 ) ) ;
#10103=CARTESIAN_POINT ( 'NONE',  ( 3.833788745076180060, -15.06587152019073272, 5.274579322627055866 ) ) ;
#10104=CIRCLE ( 'NONE', #615, 0.5080000000000002292 ) ;
#10105=CARTESIAN_POINT ( 'NONE',  ( -14.84976704640063971, 123.2524255416106342, 1.171266444394656103 ) ) ;
#10106=CARTESIAN_POINT ( 'NONE',  ( -4.631227783250409402, 22.10816835407601744, -0.05711764529929251599 ) ) ;
#10107=CARTESIAN_POINT ( 'NONE',  ( 1.396185014843718264, 159.5914066142653098, 0.2870382629871537361 ) ) ;
#10108=CARTESIAN_POINT ( 'NONE',  ( 1.982318871328906384, -15.65638878249517241, 5.868593396322577149 ) ) ;
#10110=CARTESIAN_POINT ( 'NONE',  ( 0.4636875340052978300, -8.988401195314681402, -0.8615772474383697199 ) ) ;
#10111=CARTESIAN_POINT ( 'NONE',  ( -23.42751387171889021, 146.8275480241000253, -0.6231101672962390259 ) ) ;
#10112=CARTESIAN_POINT ( 'NONE',  ( -4.825036788391022569, 50.63946620154572997, -0.09641571798141751470 ) ) ;
#10115=CARTESIAN_POINT ( 'NONE',  ( -8.793818945878454585, 117.7262650372997399, 0.04269669187023553830 ) ) ;
#10116=ORIENTED_EDGE ( 'NONE', *, *, #32316, .F. ) ;
#10117=CARTESIAN_POINT ( 'NONE',  ( -16.98580377952209020, 140.1729163700083518, 1.602912605581681804 ) ) ;
#10119=CARTESIAN_POINT ( 'NONE',  ( 19.90801791207593396, 136.1824594150436383, 2.220825683169746156 ) ) ;
#10120=CARTESIAN_POINT ( 'NONE',  ( 18.83801864273514326, 140.8526363637247982, -1.765582951612574281 ) ) ;
#10121=CARTESIAN_POINT ( 'NONE',  ( -0.7398639285967090196, 8.776656789086558774, 0.6336005302938405581 ) ) ;
#10122=CARTESIAN_POINT ( 'NONE',  ( -21.76696383529571577, 149.6930991844618291, -2.018179159957717683 ) ) ;
#10123=CARTESIAN_POINT ( 'NONE',  ( 4.688774855980650358, 118.0063900739628338, -0.5874540965100417678 ) ) ;
#10125=CARTESIAN_POINT ( 'NONE',  ( 10.51090385015211837, 123.6668265419868646, -0.9186085726806036966 ) ) ;
#10126=CARTESIAN_POINT ( 'NONE',  ( -0.6438746309741667506, 120.9974662015465867, -0.01286614746332133928 ) ) ;
#10128=CARTESIAN_POINT ( 'NONE',  ( -7.475014592328212082, 120.3045338523282197, -1.338105361635808510 ) ) ;
#10129=CARTESIAN_POINT ( 'NONE',  ( 2.047221892555406431, -15.65848914036231676, 5.808978358897256555 ) ) ;
#10130=CARTESIAN_POINT ( 'NONE',  ( 3.009276887026297587, 50.13146620154573441, -1.210121013456480599 ) ) ;
#10132=CARTESIAN_POINT ( 'NONE',  ( 7.823018779267000511, 156.2605297791399437, 2.010767698085225152 ) ) ;
#10133=CARTESIAN_POINT ( 'NONE',  ( 2.958531772299235918, 50.13146620154573441, 1.329372033065076231 ) ) ;
#10136=CARTESIAN_POINT ( 'NONE',  ( -1.676539183893759777, 107.1743931308027129, 4.723177562573835253 ) ) ;
#10138=CARTESIAN_POINT ( 'NONE',  ( -7.287282906664737325, 21.23368160547805061, -4.223004820119153457 ) ) ;
#10139=CARTESIAN_POINT ( 'NONE',  ( 7.977778825752197100, 154.6030710842251494, 0.7700301581992888833 ) ) ;
#10141=CARTESIAN_POINT ( 'NONE',  ( 1.008409768533820250, 116.9791385580615781, -0.3449706568517265648 ) ) ;
#10143=CARTESIAN_POINT ( 'NONE',  ( 4.581726285797169673, -15.30239759124965460, -0.5121114015708873035 ) ) ;
#10144=CARTESIAN_POINT ( 'NONE',  ( -16.17587344042707542, 121.2571949256804089, -0.3060957306870975003 ) ) ;
#10146=CARTESIAN_POINT ( 'NONE',  ( -5.059956948048136560, 120.1989321871395049, -0.8615610664638462257 ) ) ;
#10147=CARTESIAN_POINT ( 'NONE',  ( 3.433723587035138802, -15.33122114496111088, 5.473735664463222683 ) ) ;
#10148=CARTESIAN_POINT ( 'NONE',  ( -2.970866406646269109, 156.0959049650892041, -0.4589190987796909482 ) ) ;
#10149=CARTESIAN_POINT ( 'NONE',  ( 1.930977371672661924, -15.05712096081325591, 5.742647184725750087 ) ) ;
#10150=CARTESIAN_POINT ( 'NONE',  ( -7.538779372106369614, 158.4854300789945398, 0.9926846707982196483 ) ) ;
#10151=CARTESIAN_POINT ( 'NONE',  ( 6.898502017095807126, 117.1694300671557727, 0.1814136226821931042 ) ) ;
#10153=CARTESIAN_POINT ( 'NONE',  ( 4.560362914109654220, -11.68884639558073069, 0.6953251057713033534 ) ) ;
#10154=CARTESIAN_POINT ( 'NONE',  ( -16.31694223957266843, 121.4173703750124531, -0.3260513381110076714 ) ) ;
#10156=CARTESIAN_POINT ( 'NONE',  ( 0.1691645607388194417, 105.7854827236532600, 5.338396616797809635 ) ) ;
#10157=CARTESIAN_POINT ( 'NONE',  ( 6.991010015000402866, 121.8564574889588528, 0.4677317843132159925 ) ) ;
#10159=CARTESIAN_POINT ( 'NONE',  ( 3.750385610654966229, 4.675867361267946443, -2.714424430587211834 ) ) ;
#10160=CARTESIAN_POINT ( 'NONE',  ( 12.60858107845348997, 120.1953580586475567, 1.309872962259287954 ) ) ;
#10161=CARTESIAN_POINT ( 'NONE',  ( -0.1036566276974058148, 106.2435128697216413, 5.187401519901555957 ) ) ;
#10164=CARTESIAN_POINT ( 'NONE',  ( 16.12297089460568955, 125.3625853296581312, -1.240993850804037013 ) ) ;
#10165=CARTESIAN_POINT ( 'NONE',  ( -1.246715508051662535, 10.49814879194060069, 4.449005273994115939 ) ) ;
#10166=CARTESIAN_POINT ( 'NONE',  ( -22.59100494123605074, 149.3758529064199934, -1.630758705999802105 ) ) ;
#10167=ORIENTED_EDGE ( 'NONE', *, *, #19630, .T. ) ;
#10168=CARTESIAN_POINT ( 'NONE',  ( -11.82813386268903955, 130.3161362890850512, -0.2363542639706542603 ) ) ;
#10170=CARTESIAN_POINT ( 'NONE',  ( -5.918555687551815048, 121.5031286879076902, 0.05579296748036354642 ) ) ;
#10171=CARTESIAN_POINT ( 'NONE',  ( 5.414172367154487908, -13.81390647261572546, 3.268633212004894872 ) ) ;
#10173=CARTESIAN_POINT ( 'NONE',  ( -2.987330068958255147, 108.3452252202424404, -4.269296957098151601 ) ) ;
#10174=ORIENTED_EDGE ( 'NONE', *, *, #1083, .F. ) ;
#10175=CARTESIAN_POINT ( 'NONE',  ( 1.027076152783741536, 158.1148137021529578, 1.645667644272182706 ) ) ;
#10177=CARTESIAN_POINT ( 'NONE',  ( 8.770618086120967050, 123.6813396614493712, 0.1752578222716852652 ) ) ;
#10178=CARTESIAN_POINT ( 'NONE',  ( -16.42246607841806849, 155.2191194103077407, 0.6571739840263307597 ) ) ;
#10179=CARTESIAN_POINT ( 'NONE',  ( 4.543739712435177047, -15.19060223592207137, -0.8445694877862246486 ) ) ;
#10181=CARTESIAN_POINT ( 'NONE',  ( 13.44960824739621863, 119.6710471929552000, -0.1296808650140443553 ) ) ;
#10182=CIRCLE ( 'NONE', #28566, 0.5080000000000002292 ) ;
#10189=EDGE_CURVE ( 'NONE', #33842, #24193, #18312, .T. ) ;
#10190=CARTESIAN_POINT ( 'NONE',  ( -4.412045077147967120, 118.1805591891959040, 0.3959213965498911691 ) ) ;
#10193=CARTESIAN_POINT ( 'NONE',  ( -4.336649912933128626, 118.7629491485454309, -1.056103682561591484 ) ) ;
#10194=CARTESIAN_POINT ( 'NONE',  ( 8.331606247052166125, 120.0850720456318896, -1.118075670235503249 ) ) ;
#10195=CARTESIAN_POINT ( 'NONE',  ( -5.210105874137158644, 116.2501875120488393, -1.173469071234783501 ) ) ;
#10196=CARTESIAN_POINT ( 'NONE',  ( 4.433919446672925702, 118.1245909124861129, 0.7354544754953129537 ) ) ;
#10197=CARTESIAN_POINT ( 'NONE',  ( -9.931348751161777955, 124.0638329749226330, -0.9965119107524912367 ) ) ;
#10199=CARTESIAN_POINT ( 'NONE',  ( 0.8479371882405327687, 117.9496053012138077, -1.365999150512961835 ) ) ;
#10200=CARTESIAN_POINT ( 'NONE',  ( 5.615711437771513381, 117.9270669303711117, -0.5242027053071313114 ) ) ;
#10201=CARTESIAN_POINT ( 'NONE',  ( -16.66101725429952651, 148.5304741467402323, -2.032660103712368382 ) ) ;
#10202=EDGE_CURVE ( 'NONE', #26194, #19060, #33900, .T. ) ;
#10203=CARTESIAN_POINT ( 'NONE',  ( 0.09347673290359038989, 104.6144662015457385, -6.110098594576430564 ) ) ;
#10204=CARTESIAN_POINT ( 'NONE',  ( -0.004910621514806326471, 156.3161161488371533, 0.2457475809811482670 ) ) ;
#10205=CARTESIAN_POINT ( 'NONE',  ( 8.262035544818608912, 120.4240392771561119, -1.115000201712876171 ) ) ;
#10206=CARTESIAN_POINT ( 'NONE',  ( -14.15045567233496016, 138.8477291504528353, -0.2164309031519826565 ) ) ;
#10207=CARTESIAN_POINT ( 'NONE',  ( -4.187759052228169132, -5.978784877027076838, 2.003160513425938483 ) ) ;
#10208=CARTESIAN_POINT ( 'NONE',  ( 22.44855437653365726, 150.5824416163731314, 1.170575646458954289 ) ) ;
#10210=CARTESIAN_POINT ( 'NONE',  ( 2.913544029416218262, -15.22775915604775143, 4.213357497968500454 ) ) ;
#10211=CARTESIAN_POINT ( 'NONE',  ( -7.566762702257322282, 120.1328256275108828, 1.061688055624673943 ) ) ;
#10212=CARTESIAN_POINT ( 'NONE',  ( 0.7196250225040555781, 4.026961778641204859, -0.6563066166970625837 ) ) ;
#10213=CARTESIAN_POINT ( 'NONE',  ( -6.903056240602074567, 117.3320596397172721, -0.5256612950045381760 ) ) ;
#10214=CARTESIAN_POINT ( 'NONE',  ( -0.9385480264228447389, -6.289884363042010484, -0.2871545319985167044 ) ) ;
#10215=ORIENTED_EDGE ( 'NONE', *, *, #3283, .F. ) ;
#10218=CARTESIAN_POINT ( 'NONE',  ( 6.073876170729577417, 119.5347744825833871, 0.5156133147040066200 ) ) ;
#10220=CARTESIAN_POINT ( 'NONE',  ( -16.04013775433294242, 147.3640369757652877, 0.6457813799431219026 ) ) ;
#10221=ADVANCED_FACE ( 'NONE', ( #14001 ), #24268, .T. ) ;
#10222=CARTESIAN_POINT ( 'NONE',  ( 2.228616319073483787, -14.90713850702725374, 5.562102343610016320 ) ) ;
#10223=CARTESIAN_POINT ( 'NONE',  ( 17.47151851664378341, 144.3974720067888313, -1.548345126349529366 ) ) ;
#10224=CARTESIAN_POINT ( 'NONE',  ( -16.71878049915338948, 131.5287050380659082, -2.312093064668929721 ) ) ;
#10226=CARTESIAN_POINT ( 'NONE',  ( 2.351750233177451133, -15.05367847713771923, 4.985144330900271648 ) ) ;
#10227=CARTESIAN_POINT ( 'NONE',  ( 0.01691503824229025066, 39.20946620154573026, -0.8464976821738524615 ) ) ;
#10228=EDGE_CURVE ( 'NONE', #21511, #10570, #20379, .T. ) ;
#10229=CARTESIAN_POINT ( 'NONE',  ( 2.805605324221167596, 120.9854572005495044, -0.04483369291007272689 ) ) ;
#10236=CARTESIAN_POINT ( 'NONE',  ( -5.008552712180506461, 117.3993836135855560, 0.7755994290793736257 ) ) ;
#10237=CARTESIAN_POINT ( 'NONE',  ( 0.001640166039733662951, 159.6041700698465036, -0.08208061555506486473 ) ) ;
#10238=CARTESIAN_POINT ( 'NONE',  ( -5.416379098809520620, 117.1811293437636721, 0.6832607176795201243 ) ) ;
#10239=CARTESIAN_POINT ( 'NONE',  ( -0.7907830483637354746, 118.1473448952717860, 0.8952419762006665893 ) ) ;
#10241=CARTESIAN_POINT ( 'NONE',  ( -4.654180141762545908, 32.06930816699426146, 0.6251022194440085666 ) ) ;
#10242=CARTESIAN_POINT ( 'NONE',  ( 10.35908644403297352, 120.1444133044471556, 1.518303869478637491 ) ) ;
#10243=CARTESIAN_POINT ( 'NONE',  ( -4.621022795674669226, 27.76579825817536218, 0.1735962381356405959 ) ) ;
#10244=CARTESIAN_POINT ( 'NONE',  ( 8.391066749008803782, -15.30525627429770097, -0.4359234444501501327 ) ) ;
#10245=CARTESIAN_POINT ( 'NONE',  ( 8.631715985724209617, 118.5888693174204889, -0.7825621615820586019 ) ) ;
#10246=CARTESIAN_POINT ( 'NONE',  ( -3.291481622402053109, 124.4927030837263118, -0.08807361928342474777 ) ) ;
#10247=CARTESIAN_POINT ( 'NONE',  ( 4.970385380909975837, 117.4009584165977600, 0.9889290504008942939 ) ) ;
#10249=CARTESIAN_POINT ( 'NONE',  ( 0.8026539263819157943, 105.1230347856897538, 5.284155675286346110 ) ) ;
#10250=CARTESIAN_POINT ( 'NONE',  ( -0.6244342276652131707, 19.93415720681881353, -4.586363120317934694 ) ) ;
#10252=CARTESIAN_POINT ( 'NONE',  ( -16.18905205736058051, 121.2598130428683447, -0.3234957879086920451 ) ) ;
#10253=CARTESIAN_POINT ( 'NONE',  ( 3.154677723130417277, -14.38507846778283650, 3.622984934187011952 ) ) ;
#10254=CARTESIAN_POINT ( 'NONE',  ( 2.311559032573872408, 118.7862729053988318, -0.6846880608948527902 ) ) ;
#10255=CARTESIAN_POINT ( 'NONE',  ( -22.69192130277354025, 142.3612397021088611, 0.6360799666370220429 ) ) ;
#10260=CARTESIAN_POINT ( 'NONE',  ( 2.711364258112227255, 37.31625399494021877, -1.095520810760639119 ) ) ;
#10261=CARTESIAN_POINT ( 'NONE',  ( 2.573200380748495331, -15.70867456196409151, 5.149826986703908815 ) ) ;
#10262=CARTESIAN_POINT ( 'NONE',  ( -18.89434961005724034, 135.8679125664981484, 1.636908753694952257 ) ) ;
#10264=CARTESIAN_POINT ( 'NONE',  ( 21.87558878470073154, 148.2155681941778482, -1.275940291167070306 ) ) ;
#10265=CARTESIAN_POINT ( 'NONE',  ( -4.476207883417873568, -7.053342675672244155, -1.178223045331058705 ) ) ;
#10269=CARTESIAN_POINT ( 'NONE',  ( -4.958175139285456723, 117.4049635120808972, -1.028653955280601773 ) ) ;
#10270=CARTESIAN_POINT ( 'NONE',  ( 0.3093948633799631920, 109.1907409294041429, 4.022046774707581207 ) ) ;
#10272=CARTESIAN_POINT ( 'NONE',  ( -7.013665818177523548, 155.6889469082406947, 1.337060831506289293 ) ) ;
#10275=CARTESIAN_POINT ( 'NONE',  ( 15.45240368193225322, 131.3329289045130679, -1.560586129702050462 ) ) ;
#10276=CIRCLE ( 'NONE', #3489, 3.175000000000001155 ) ;
#10277=CARTESIAN_POINT ( 'NONE',  ( -20.39340916383850200, 150.0074677946399504, -2.333577254436574044 ) ) ;
#10280=CARTESIAN_POINT ( 'NONE',  ( 4.533610671541467241, 118.1203594940373307, -0.4772282360780506494 ) ) ;
#10281=CARTESIAN_POINT ( 'NONE',  ( 15.99817776903315547, 146.0164801329953548, -0.4101439804456897265 ) ) ;
#10283=CARTESIAN_POINT ( 'NONE',  ( -3.657622835216545631, 156.7231754051992425, -1.598616135119148129 ) ) ;
#10284=CARTESIAN_POINT ( 'NONE',  ( 2.778183380295619287, -15.08691762314898277, 4.378844564414270835 ) ) ;
#10286=CARTESIAN_POINT ( 'NONE',  ( -2.444554238799683255, 105.1244307588895879, -4.750552072186019714 ) ) ;
#10289=CARTESIAN_POINT ( 'NONE',  ( -3.833338661037195561, 9.423677021345861604, 2.587938769098377279 ) ) ;
#10290=CARTESIAN_POINT ( 'NONE',  ( -0.02615319344480391064, 156.8698190429800832, 1.308812744920978544 ) ) ;
#10291=CARTESIAN_POINT ( 'NONE',  ( 1.215845237882275276, 34.83336793224903261, 0.05010825926065069075 ) ) ;
#10293=CIRCLE ( 'NONE', #13702, 3.683000000000001162 ) ;
#10294=CARTESIAN_POINT ( 'NONE',  ( 4.256838582791900194, 16.71066835407712858, 1.825063967593055558 ) ) ;
#10295=CARTESIAN_POINT ( 'NONE',  ( 2.816370844845887955, 121.0122979933374978, 0.1218616300372573624 ) ) ;
#10298=CARTESIAN_POINT ( 'NONE',  ( 2.184308556171625781, 116.2030918562186912, -0.04283386123071435125 ) ) ;
#10302=DIRECTION ( 'NONE',  ( -4.017660918040594346E-17, 1.000000000000000000, 2.376309959284834438E-19 ) ) ;
#10309=CARTESIAN_POINT ( 'NONE',  ( -11.57591774076052893, 118.7825156662901378, 0.1473217720007393150 ) ) ;
#10310=VERTEX_POINT ( 'NONE', #29984 ) ;
#10312=CARTESIAN_POINT ( 'NONE',  ( -6.041016396376916120, 121.4368974476174543, -0.1415500717406000253 ) ) ;
#10315=CARTESIAN_POINT ( 'NONE',  ( -15.52555164710823021, 147.5317938866932366, -0.3613967763117280629 ) ) ;
#10316=CARTESIAN_POINT ( 'NONE',  ( 3.397480601066255712, -15.04020002808364964, 5.521695076403254632 ) ) ;
#10317=AXIS2_PLACEMENT_3D ( 'NONE', #3674, #9834, #3462 ) ;
#10318=CARTESIAN_POINT ( 'NONE',  ( -19.75353020121338332, 136.1149058410947532, 1.478659091479563203 ) ) ;
#10319=CARTESIAN_POINT ( 'NONE',  ( 3.874746376330849618, 18.20996518813934628, -2.522041008920607563 ) ) ;
#10320=CARTESIAN_POINT ( 'NONE',  ( 9.724873038621939969, 118.0756159837034716, 0.5523889259422302134 ) ) ;
#10321=CARTESIAN_POINT ( 'NONE',  ( 1.965399808016191852, -15.70638203882245065, 5.774101002626401247 ) ) ;
#10323=CARTESIAN_POINT ( 'NONE',  ( 0.07244829501375356362, -8.348772924205562163, -0.9745465824848156267 ) ) ;
#10324=CARTESIAN_POINT ( 'NONE',  ( -23.20201897184738371, 149.6253602407241488, -0.6175280007103174373 ) ) ;
#10326=CARTESIAN_POINT ( 'NONE',  ( 4.825036788390895559, 50.63946620154572997, 0.09641571798141809757 ) ) ;
#10327=CARTESIAN_POINT ( 'NONE',  ( -5.554537448396219546, 116.8461671677355156, 0.2570831589019035301 ) ) ;
#10328=ORIENTED_EDGE ( 'NONE', *, *, #30573, .F. ) ;
#10329=CARTESIAN_POINT ( 'NONE',  ( -9.634306097686000214, 155.2307989660268959, 1.622952429610069469 ) ) ;
#10331=CARTESIAN_POINT ( 'NONE',  ( 20.82642717637620677, 141.6159226613069109, 2.307662509007912810 ) ) ;
#10332=CARTESIAN_POINT ( 'NONE',  ( 19.68629672748963344, 145.2539617268756729, -1.742627101631719855 ) ) ;
#10333=CARTESIAN_POINT ( 'NONE',  ( -0.9136164112762927836, -2.447138680932527066, -0.3421040304710446511 ) ) ;
#10334=AXIS2_PLACEMENT_3D ( 'NONE', #20823, #645, #1059 ) ;
#10335=CARTESIAN_POINT ( 'NONE',  ( -17.48314440517399504, 153.9260871938423065, -1.866247694559708403 ) ) ;
#10336=CARTESIAN_POINT ( 'NONE',  ( 4.625020092980742348, 118.0596586542457374, -0.5389086530673455888 ) ) ;
#10337=AXIS2_PLACEMENT_3D ( 'NONE', #24338, #37138, #30527 ) ;
#10338=CARTESIAN_POINT ( 'NONE',  ( 5.314256358593297591, 104.6144662015456959, -0.4585142902082095517 ) ) ;
#10339=CARTESIAN_POINT ( 'NONE',  ( 11.07452758269540105, 153.1537610418535849, -0.9542791616922484677 ) ) ;
#10340=CARTESIAN_POINT ( 'NONE',  ( -11.85733017202539230, 130.3381101163291760, -0.1934038552275227363 ) ) ;
#10341=ORIENTED_EDGE ( 'NONE', *, *, #9982, .F. ) ;
#10342=CARTESIAN_POINT ( 'NONE',  ( -7.432183457866743836, 120.4750020944285609, -1.305203700904508546 ) ) ;
#10343=CARTESIAN_POINT ( 'NONE',  ( 4.858843758304779215, -15.48047902945742749, 1.209346601706016378 ) ) ;
#10344=CARTESIAN_POINT ( 'NONE',  ( -5.274544067074300457, 115.7029491485454002, 0.8135768287290441325 ) ) ;
#10345=CARTESIAN_POINT ( 'NONE',  ( -4.547563907768285674, 118.0745712654054387, -0.7853206451047147763 ) ) ;
#10346=EDGE_CURVE ( 'NONE', #23040, #24227, #38580, .T. ) ;
#10349=CARTESIAN_POINT ( 'NONE',  ( 11.01240597710799030, 122.5598569164413334, 1.651065454484659023 ) ) ;
#10351=CARTESIAN_POINT ( 'NONE',  ( 22.76738278397251136, 137.3906169244638136, 0.4549464913834383450 ) ) ;
#10352=CARTESIAN_POINT ( 'NONE',  ( 0.8142577860443056537, 14.98675861574836077, 8.418590528086960845 ) ) ;
#10353=CARTESIAN_POINT ( 'NONE',  ( 2.729962743038877981, 120.7841308545065431, 0.3244322735474265973 ) ) ;
#10354=CARTESIAN_POINT ( 'NONE',  ( 6.900334503690523036, 117.6856483911789581, -0.5402308543058538248 ) ) ;
#10356=ORIENTED_EDGE ( 'NONE', *, *, #21004, .T. ) ;
#10357=CARTESIAN_POINT ( 'NONE',  ( 0.4613487476409313670, 118.7629491485454025, 1.278559828376704344 ) ) ;
#10360=CARTESIAN_POINT ( 'NONE',  ( -16.86121613381897433, 155.2078297922403465, -0.3138802613840050437 ) ) ;
#10361=VERTEX_POINT ( 'NONE', #27835 ) ;
#10362=CARTESIAN_POINT ( 'NONE',  ( 8.047001766538286915, 121.4495122670571590, -0.8773712736992811401 ) ) ;
#10364=CARTESIAN_POINT ( 'NONE',  ( -9.304959842724306540, 124.0984330410602183, -0.5077435198050487264 ) ) ;
#10365=CARTESIAN_POINT ( 'NONE',  ( 3.969679720280225421, -13.58737529183706627, 3.751183842293267290 ) ) ;
#10366=CARTESIAN_POINT ( 'NONE',  ( -18.64118049546060263, 128.6297099747515347, 0.9949054493987050662 ) ) ;
#10368=CARTESIAN_POINT ( 'NONE',  ( 5.748481425938850364, 159.1178304044242964, 0.1659167284945115006 ) ) ;
#10369=ORIENTED_EDGE ( 'NONE', *, *, #19041, .T. ) ;
#10370=CARTESIAN_POINT ( 'NONE',  ( 1.360477052538118681, -3.804838552850991817, 4.419457122809256511 ) ) ;
#10371=CARTESIAN_POINT ( 'NONE',  ( -17.31377588638430964, 122.7721875394316555, -0.3459704467065360944 ) ) ;
#10374=CARTESIAN_POINT ( 'NONE',  ( 4.652282364505444967, 111.7580701808239070, 2.677127711625311157 ) ) ;
#10375=CARTESIAN_POINT ( 'NONE',  ( 4.647043587409348753, 118.8389947276285881, 1.076879562718962235 ) ) ;
#10376=( BOUNDED_CURVE ( )  B_SPLINE_CURVE ( 3, ( #9932, #16097, #29745, #29103, #10143, #35724, #42122 ),
 .UNSPECIFIED., .F., .T. ) 
 B_SPLINE_CURVE_WITH_KNOTS ( ( 4, 3, 4 ),
 ( 0.7498838476046071344, 1.000185576741208449, 1.000187438830518083 ),
 .UNSPECIFIED. ) 
 CURVE ( )  GEOMETRIC_REPRESENTATION_ITEM ( )  RATIONAL_B_SPLINE_CURVE ( ( 0.5000007283237750677, 0.4995979372591234369, 0.6662643611511984698, 1.000000000000000000, 0.9999975172142537838, 0.9999950344377539491, 0.9999925516705003847 ) ) 
 REPRESENTATION_ITEM ( '' )  );
#10377=CARTESIAN_POINT ( 'NONE',  ( -1.319288878716189828, -8.717950886928733212, 4.428293336331323715 ) ) ;
#10378=CARTESIAN_POINT ( 'NONE',  ( 14.37796933089559381, 121.0470547900126519, 1.299527359048518793 ) ) ;
#10381=CARTESIAN_POINT ( 'NONE',  ( 11.80709641148037470, 120.8928578745602209, -1.148978701482599840 ) ) ;
#10382=CARTESIAN_POINT ( 'NONE',  ( -1.959332070151295291, -8.942847522256865744, 4.198131957625402144 ) ) ;
#10383=CARTESIAN_POINT ( 'NONE',  ( -22.83601474261773134, 146.5373477140321938, -1.546791039490589270 ) ) ;
#10384=ORIENTED_EDGE ( 'NONE', *, *, #21447, .T. ) ;
#10385=CARTESIAN_POINT ( 'NONE',  ( -7.938918103923473524, 154.5997988942315260, 0.3378123388718582421 ) ) ;
#10386=CARTESIAN_POINT ( 'NONE',  ( 4.377062889037126148, -14.98224217357194199, 4.840108967533193862 ) ) ;
#10387=DIRECTION ( 'NONE',  ( 0.01997839162482749689, 1.040247600000945640E-18, -0.9998004120163610509 ) ) ;
#10389=CARTESIAN_POINT ( 'NONE',  ( -1.300523255896344654, 106.1067062490390640, -5.175614940688300081 ) ) ;
#10391=CARTESIAN_POINT ( 'NONE',  ( 12.62197313556516320, 122.7135068550949200, 1.834144044656287109 ) ) ;
#10393=LINE ( 'NONE', #37221, #6906 ) ;
#10395=CARTESIAN_POINT ( 'NONE',  ( -15.27126642897852982, 121.5932973536894934, 0.6323128539531664982 ) ) ;
#10396=CARTESIAN_POINT ( 'NONE',  ( -6.300109353874518980, 26.68925120273002705, -5.586516568188822696 ) ) ;
#10397=CARTESIAN_POINT ( 'NONE',  ( 1.752245784495049863, 156.4219299504922844, 0.9069267871912084500 ) ) ;
#10399=CARTESIAN_POINT ( 'NONE',  ( 2.843964318557650639, 116.7549172960530939, -0.2381273168889445624 ) ) ;
#10405=CARTESIAN_POINT ( 'NONE',  ( -4.466856387348673962, 118.1267949675633417, 0.5517216040399967047 ) ) ;
#10406=CARTESIAN_POINT ( 'NONE',  ( -5.586884702347497011, 110.9644662015457328, -0.1116392523995361624 ) ) ;
#10409=CARTESIAN_POINT ( 'NONE',  ( -8.285659017902016643, 120.0588997814717089, -1.449894828885264664 ) ) ;
#10410=CARTESIAN_POINT ( 'NONE',  ( -4.351830713015083951, 111.2795884869231173, -3.127581853150075197 ) ) ;
#10412=CARTESIAN_POINT ( 'NONE',  ( 4.522265204868332944, 118.1110255742863586, 0.6889464356651477939 ) ) ;
#10413=CARTESIAN_POINT ( 'NONE',  ( -10.75107117262888501, 153.0872561326487187, -1.097343645257591538 ) ) ;
#10415=CARTESIAN_POINT ( 'NONE',  ( -0.8958938016497142165, 115.7029491485453150, -1.751256854871092949 ) ) ;
#10417=CARTESIAN_POINT ( 'NONE',  ( 0.1058213901577000071, 105.9761915687834772, -5.295735085524063024 ) ) ;
#10418=CARTESIAN_POINT ( 'NONE',  ( -10.31823449898719147, 154.1877054190025262, -1.778048316349531088 ) ) ;
#10419=CARTESIAN_POINT ( 'NONE',  ( -5.332935397695335311, 104.6144662015457385, -0.1065647409268299373 ) ) ;
#10420=CARTESIAN_POINT ( 'NONE',  ( -0.009748065369249884343, 159.5507987164374981, 0.4878330526048098581 ) ) ;
#10421=CARTESIAN_POINT ( 'NONE',  ( 8.413874481325049004, 119.6811429777993681, -1.089663159344693488 ) ) ;
#10422=CARTESIAN_POINT ( 'NONE',  ( -11.83435633982874435, 152.0434770505088977, -0.1115628666874381447 ) ) ;
#10424=CARTESIAN_POINT ( 'NONE',  ( -3.178183004559932190, -7.902942162671289239, -3.366045245292264010 ) ) ;
#10425=CARTESIAN_POINT ( 'NONE',  ( 14.80341400616306657, 120.8492938200443092, 1.052940121379140725 ) ) ;
#10427=CARTESIAN_POINT ( 'NONE',  ( 3.154745640343158630, -14.88448557395780014, 3.454683184413806174 ) ) ;
#10428=CARTESIAN_POINT ( 'NONE',  ( -18.37903003504447952, 149.1773161885088825, 1.724610598947830420 ) ) ;
#10429=CARTESIAN_POINT ( 'NONE',  ( -0.5179912613141952615, -13.03896268189918217, -0.8249499322734266116 ) ) ;
#10430=CARTESIAN_POINT ( 'NONE',  ( -14.49621620279169676, 120.3567457872619997, -0.7930654045677064667 ) ) ;
#10431=VECTOR ( 'NONE', #635, 1000.000000000000000 ) ;
#10432=CARTESIAN_POINT ( 'NONE',  ( -0.6011478996571989475, -4.452122406214784611, 0.7678286701737500053 ) ) ;
#10435=CARTESIAN_POINT ( 'NONE',  ( 3.094730188726686482, 108.9521120498200730, 4.030551393973051510 ) ) ;
#10436=CARTESIAN_POINT ( 'NONE',  ( -1.703787162446291914, 156.3322054215483092, 0.5946588160098703613 ) ) ;
#10437=CARTESIAN_POINT ( 'NONE',  ( 2.381342306750187099, -14.83133394530772264, 5.477793184119461145 ) ) ;
#10438=CARTESIAN_POINT ( 'NONE',  ( 11.67916898317097818, 124.4569610989641859, -1.132436424213030035 ) ) ;
#10439=CARTESIAN_POINT ( 'NONE',  ( -18.97962326299262159, 149.2349160008635351, -2.496544457321505650 ) ) ;
#10442=CARTESIAN_POINT ( 'NONE',  ( 1.860714312465608478, -15.17550571231866741, 5.451645902226371021 ) ) ;
#10444=CARTESIAN_POINT ( 'NONE',  ( 7.051595240896772587, 122.0586610246435129, 0.007850877590933884320 ) ) ;
#10445=ORIENTED_EDGE ( 'NONE', *, *, #18832, .F. ) ;
#10446=CARTESIAN_POINT ( 'NONE',  ( -3.764831887694549462, 109.1680670511255897, 3.784283605914390503 ) ) ;
#10447=CARTESIAN_POINT ( 'NONE',  ( 3.527324519276021420, 50.63946620154572997, -1.707870599815379586 ) ) ;
#10451=CARTESIAN_POINT ( 'NONE',  ( 8.070121050663628282, 158.6666700270975525, 0.1062422583151904215 ) ) ;
#10452=CARTESIAN_POINT ( 'NONE',  ( -6.342742252400029201, 120.0627515544778134, 0.2010047130458860465 ) ) ;
#10454=CARTESIAN_POINT ( 'NONE',  ( 1.726544654667829137, -15.62332984182715556, 5.743678577341975178 ) ) ;
#10455=CARTESIAN_POINT ( 'NONE',  ( -5.314278422745059238, 105.1224610256965235, 0.4583187270701644667 ) ) ;
#10456=CARTESIAN_POINT ( 'NONE',  ( 0.9570772947141352738, 38.77965003586765391, -1.217401628196721042 ) ) ;
#10457=CARTESIAN_POINT ( 'NONE',  ( 20.64857576366712522, 148.2641884961211076, 2.442776014760721814 ) ) ;
#10458=CARTESIAN_POINT ( 'NONE',  ( 3.287934792154566299, 21.71798121574904172, 3.254339964430349230 ) ) ;
#10459=CARTESIAN_POINT ( 'NONE',  ( -5.330747076954383878, 11.08732641057851964, -6.519097198751918398 ) ) ;
#10460=CARTESIAN_POINT ( 'NONE',  ( 2.459102646145539417, 117.4060512218794230, -0.6259389031298756567 ) ) ;
#10461=CARTESIAN_POINT ( 'NONE',  ( -0.3557171951619191863, 107.2171362991012842, -4.792661424475801901 ) ) ;
#10462=AXIS2_PLACEMENT_3D ( 'NONE', #35346, #38960, #6793 ) ;
#10464=DIRECTION ( 'NONE',  ( 4.017660918040594346E-17, -1.000000000000000000, -2.376309959284834438E-19 ) ) ;
#10465=CARTESIAN_POINT ( 'NONE',  ( -0.001862839608620314551, 124.0591982226671490, 0.09322411149287226917 ) ) ;
#10466=CARTESIAN_POINT ( 'NONE',  ( -1.932895124392534303, 20.38400505531995321, -4.219463811995566083 ) ) ;
#10469=CARTESIAN_POINT ( 'NONE',  ( 3.254806331274714637, -13.89383896039994504, 2.504907480430248246 ) ) ;
#10470=EDGE_CURVE ( 'NONE', #35682, #18326, #37847, .T. ) ;
#10471=CARTESIAN_POINT ( 'NONE',  ( 3.106711772599447308, 110.6400929099055332, -3.287732168264224430 ) ) ;
#10472=CARTESIAN_POINT ( 'NONE',  ( -20.34281169216131246, 152.5255278361454145, 0.5339126128458231424 ) ) ;
#10473=CARTESIAN_POINT ( 'NONE',  ( 4.801216665950859941, 117.4032681888241143, -1.015537427444714202 ) ) ;
#10477=CARTESIAN_POINT ( 'NONE',  ( 5.320894714828252603, -15.22957080661538320, -0.4730099507937148284 ) ) ;
#10478=CARTESIAN_POINT ( 'NONE',  ( -8.970048054448252373, 157.0267672960688969, 1.675204009492540669 ) ) ;
#10479=CARTESIAN_POINT ( 'NONE',  ( 12.31483450803178314, 120.4651188882986759, -0.9715887866197354672 ) ) ;
#10480=CARTESIAN_POINT ( 'NONE',  ( 4.611808778022512989, -11.57686662695173929, 0.3579861242195471194 ) ) ;
#10484=CARTESIAN_POINT ( 'NONE',  ( 1.846946891755073983, 121.3688471916803451, 0.3635544463458706965 ) ) ;
#10486=CARTESIAN_POINT ( 'NONE',  ( -11.50974670170856129, 153.2879862121713757, 1.252373795633383802 ) ) ;
#10487=CARTESIAN_POINT ( 'NONE',  ( 2.684992056639614599, 118.0925652926021598, 0.9597114035846702196 ) ) ;
#10488=CARTESIAN_POINT ( 'NONE',  ( 18.42722449710328902, 147.3262642721504960, -1.661950199828387875 ) ) ;
#10489=CARTESIAN_POINT ( 'NONE',  ( -5.841774105247432125, 118.7305451321402501, -1.158284778981343521 ) ) ;
#10490=LINE ( 'NONE', #20479, #16780 ) ;
#10491=CIRCLE ( 'NONE', #41799, 0.5080000000000002292 ) ;
#10492=ORIENTED_EDGE ( 'NONE', *, *, #37489, .T. ) ;
#10493=CARTESIAN_POINT ( 'NONE',  ( 4.535015814824959079, 118.1196967487753113, -0.4753252364964687393 ) ) ;
#10494=CARTESIAN_POINT ( 'NONE',  ( 12.39727431377423272, 130.6617397222824479, -0.4182072254281058998 ) ) ;
#10496=CARTESIAN_POINT ( 'NONE',  ( 3.406014632911877893, -14.97454077108105430, 2.395711393442250259 ) ) ;
#10500=CARTESIAN_POINT ( 'NONE',  ( -0.5165578309945342284, 6.287656885725535716, -4.620190224396742984 ) ) ;
#10501=CARTESIAN_POINT ( 'NONE',  ( 17.05487166051791448, 147.7912591418244403, 2.046378512860588028 ) ) ;
#10502=CARTESIAN_POINT ( 'NONE',  ( -2.297029980818328987, 30.88344267599554271, 1.420920951733973814 ) ) ;
#10504=CARTESIAN_POINT ( 'NONE',  ( 2.229080734463354307, 9.364070591990056869, -4.050418370856919914 ) ) ;
#10505=CARTESIAN_POINT ( 'NONE',  ( 7.564868681920670745, 122.4257779438054285, 0.2276018551017724989 ) ) ;
#10506=CARTESIAN_POINT ( 'NONE',  ( -0.1064799869812408512, 105.7853621660184444, 5.332934571178566507 ) ) ;
#10509=CARTESIAN_POINT ( 'NONE',  ( 8.791514164305905155, 117.7407919306599524, -0.07643277369106631081 ) ) ;
#10518=CARTESIAN_POINT ( 'NONE',  ( -18.55749356256747262, 125.2038358216989735, -0.01254332324266062976 ) ) ;
#10521=CARTESIAN_POINT ( 'NONE',  ( -6.971431743821577598, 121.9475450123567839, -0.2149471541011502840 ) ) ;
#10525=CARTESIAN_POINT ( 'NONE',  ( -2.887663853482277165, 156.0927491134738716, -0.09102753749515611614 ) ) ;
#10526=CARTESIAN_POINT ( 'NONE',  ( 5.913917015499376539, -14.05268412609835060, 2.470677959447274308 ) ) ;
#10527=CARTESIAN_POINT ( 'NONE',  ( -5.882407806703863429, 118.3130479344264501, 0.8400364453129069986 ) ) ;
#10528=CARTESIAN_POINT ( 'NONE',  ( 4.537321141924904211, 26.63107350737006840, 0.8823464973398146283 ) ) ;
#10529=CARTESIAN_POINT ( 'NONE',  ( 22.58226468115093866, 150.6256779753201158, 0.9011697351191821914 ) ) ;
#10531=CARTESIAN_POINT ( 'NONE',  ( 15.71988674539023734, 146.8976217521451133, 0.5151081277902610500 ) ) ;
#10532=CARTESIAN_POINT ( 'NONE',  ( 4.537321141924904211, 26.63107350737006840, 0.8823464973398146283 ) ) ;
#10533=CARTESIAN_POINT ( 'NONE',  ( 0.3060232888392590556, -2.951246395405549450, 0.9280917289473271659 ) ) ;
#10534=CARTESIAN_POINT ( 'NONE',  ( -22.51303867192119057, 150.7865899205276321, -0.6781733187083917036 ) ) ;
#10536=CARTESIAN_POINT ( 'NONE',  ( 4.962522518486619738, 117.4026900519639440, 1.030022258927823398 ) ) ;
#10538=CARTESIAN_POINT ( 'NONE',  ( -5.558216936808848097, 116.7820928991152556, 0.1694093166678532214 ) ) ;
#10539=CARTESIAN_POINT ( 'NONE',  ( -1.377724515701776120, 119.5584937100158243, 0.5648184346096531971 ) ) ;
#10541=CARTESIAN_POINT ( 'NONE',  ( 1.123502178401303064, 117.8708904510121016, 0.6147983682407556216 ) ) ;
#10542=CARTESIAN_POINT ( 'NONE',  ( 11.87140890173645857, 122.0047285378078357, -1.287708742280476493 ) ) ;
#10543=CARTESIAN_POINT ( 'NONE',  ( -0.3089908097382615959, -9.589635095254870123, 0.9269408180416041088 ) ) ;
#10544=CARTESIAN_POINT ( 'NONE',  ( -4.901975893987194688, 117.8999350694477926, -0.9234475893805552671 ) ) ;
#10545=CARTESIAN_POINT ( 'NONE',  ( 4.661932672826285540, 118.0285282382062206, -0.5802744411614334519 ) ) ;
#10547=CARTESIAN_POINT ( 'NONE',  ( 5.344295804397718008, 104.6144662015764482, -0.1103522168260312741 ) ) ;
#10548=CARTESIAN_POINT ( 'NONE',  ( 3.236331573563320241, 156.2293907256693331, -0.8668920366435199920 ) ) ;
#10550=CARTESIAN_POINT ( 'NONE',  ( -15.76285804746354380, 145.9067145067653541, -0.3149794173055767699 ) ) ;
#10552=CARTESIAN_POINT ( 'NONE',  ( -18.42282194684162278, 148.3462492009778373, -2.436111078577046118 ) ) ;
#10553=CARTESIAN_POINT ( 'NONE',  ( 5.204094786718133747, -15.42339607600888485, 1.288180339967581967 ) ) ;
#10554=CARTESIAN_POINT ( 'NONE',  ( -4.623307638546573450, 118.0214715435377997, -0.8250825005389410549 ) ) ;
#10556=CARTESIAN_POINT ( 'NONE',  ( 4.146107882323581961, 118.2391775594914520, 0.3988131543976252691 ) ) ;
#10557=CARTESIAN_POINT ( 'NONE',  ( 3.340139884075139509, 119.4525916976722897, 0.8552862985148332875 ) ) ;
#10558=CARTESIAN_POINT ( 'NONE',  ( -5.095652749712312080, 31.83908346630384756, 0.3959475160674750249 ) ) ;
#10559=CARTESIAN_POINT ( 'NONE',  ( 0.8865878252961926220, 116.4323782974132513, 0.004867729696705778465 ) ) ;
#10560=CARTESIAN_POINT ( 'NONE',  ( -6.244303144875123834, 11.31477948022340208, -5.679040650537692692 ) ) ;
#10561=CARTESIAN_POINT ( 'NONE',  ( 15.93611381433498941, 145.8030804522035737, 1.048911189365803853 ) ) ;
#10563=CARTESIAN_POINT ( 'NONE',  ( 14.59306090326458261, 120.9595740141730289, -0.6228583445698288035 ) ) ;
#10565=CARTESIAN_POINT ( 'NONE',  ( 4.401043740403896010, 115.6909491485452435, 1.538549278747252114 ) ) ;
#10566=CARTESIAN_POINT ( 'NONE',  ( -22.66420477949326795, 150.6410255081855212, -0.3761569768119877311 ) ) ;
#10569=CARTESIAN_POINT ( 'NONE',  ( -5.496727918792607248, 120.7378957778092570, -0.7277922162673816642 ) ) ;
#10570=VERTEX_POINT ( 'NONE', #5281 ) ;
#10571=DIRECTION ( 'NONE',  ( -5.206863593109713661E-17, 1.000000000000000000, -1.077750396879097183E-30 ) ) ;
#10572=CARTESIAN_POINT ( 'NONE',  ( -1.571702145576721721, 120.8584627942791627, -0.1987642453017052502 ) ) ;
#10573=CARTESIAN_POINT ( 'NONE',  ( 4.422138279315844578, -13.30579995099732926, 3.341551838899307736 ) ) ;
#10574=CARTESIAN_POINT ( 'NONE',  ( -22.37379725164922561, 146.3189071340513294, 1.009121573351525525 ) ) ;
#10576=CARTESIAN_POINT ( 'NONE',  ( 15.18737561846505102, 156.0999766016731769, 0.3708822620858234775 ) ) ;
#10578=ORIENTED_EDGE ( 'NONE', *, *, #1891, .T. ) ;
#10579=CARTESIAN_POINT ( 'NONE',  ( -1.251853189678833411, -4.679435864505671283, 4.458631606201990394 ) ) ;
#10580=CARTESIAN_POINT ( 'NONE',  ( -18.63504953328976299, 154.1157618415863624, -0.3723726386282264489 ) ) ;
#10583=CARTESIAN_POINT ( 'NONE',  ( -5.358236209449569465, 119.5150064772791012, 0.8961528214930735148 ) ) ;
#10584=CARTESIAN_POINT ( 'NONE',  ( -1.290833045837797455, 0.8901568857254957834, 4.466177308409287505 ) ) ;
#10585=CARTESIAN_POINT ( 'NONE',  ( 5.840790351889470600, 117.5931221156369730, 0.8184019802203833516 ) ) ;
#10588=CARTESIAN_POINT ( 'NONE',  ( 13.62782584980143952, 121.9345505566020194, -1.161422094953211470 ) ) ;
#10589=CARTESIAN_POINT ( 'NONE',  ( 4.471266627501615076, -5.469457446779734333, -1.220754042301255948 ) ) ;
#10590=CARTESIAN_POINT ( 'NONE',  ( -22.48407052889642799, 149.9757045183965261, -1.524144198737067635 ) ) ;
#10591=VERTEX_POINT ( 'NONE', #28258 ) ;
#10592=CARTESIAN_POINT ( 'NONE',  ( -8.684730043605732419, 123.3259068333282755, 0.1300027459630656579 ) ) ;
#10593=CARTESIAN_POINT ( 'NONE',  ( 6.473144302699227026, -13.19137087452153168, 0.2309683151692971392 ) ) ;
#10598=CARTESIAN_POINT ( 'NONE',  ( 12.21694169560761800, 122.3148578561100948, 1.796258641216138541 ) ) ;
#10601=CARTESIAN_POINT ( 'NONE',  ( -5.484805557156832378, 159.0107326448372191, 0.7391455978106867830 ) ) ;
#10602=CARTESIAN_POINT ( 'NONE',  ( 5.585279946883024316, 5.098922668322787288, -6.300588543511215001 ) ) ;
#10603=CARTESIAN_POINT ( 'NONE',  ( -0.006077178772757848950, 120.4695998130595598, 0.3041268764237433087 ) ) ;
#10604=DIRECTION ( 'NONE',  ( -0.9998004120163609398, 0.000000000000000000, -0.01997839162482749342 ) ) ;
#10605=CARTESIAN_POINT ( 'NONE',  ( 0.9702981664978360676, 116.7682604261274264, -0.2585377725347692834 ) ) ;
#10606=CARTESIAN_POINT ( 'NONE',  ( 4.646169936107913401, 117.9325745699973282, -0.7782960047779410306 ) ) ;
#10609=CARTESIAN_POINT ( 'NONE',  ( 2.959734542844846938, 107.4070365762694479, -4.429236197848620549 ) ) ;
#10612=CARTESIAN_POINT ( 'NONE',  ( -4.439880037416177316, 118.1648146445724876, 0.4551947970507644325 ) ) ;
#10613=CARTESIAN_POINT ( 'NONE',  ( 1.814579162714248461, 106.5840813593849248, -4.953779699249533763 ) ) ;
#10614=B_SPLINE_SURFACE_WITH_KNOTS ( 'NONE', 3, 3, ( 
 ( #5716, #18672, #22276, #21434, #12084, #18884, #28691, #25072, #15685, #34670, #21646, #1881, #31679, #2729, #2307, #5500, #35301, #27848, #22072, #34462, #18244, #15267, #2091, #41278, #15055, #41064, #41491, #11875, #8682, #35099, #25286, #38077, #12297, #38290, #5922, #41700, #12508, #25498, #38498, #6129, #19303, #9934, #35938, #32308, #376, #3782, #23114 ),
 ( #19511, #22483, #41912, #22695, #35512, #29321, #3138, #32520, #16100, #16743, #6967, #3351, #16318, #29105, #29747, #6750, #165, #10144, #19938, #42123, #25702, #35726, #26549, #12919, #6333, #587, #38707, #2933, #25910, #32956, #38917, #19093, #19719, #9728, #6537, #13134, #13559, #26126, #10360, #36367, #36150, #39555, #15895, #23331, #39339, #32738, #9516 ),
 ( #32101, #39127, #22904, #3571, #28897, #16532, #29541, #13343, #12712, #26332, #33367, #30363, #30578, #39981, #40394, #4199, #7805, #16952, #20342, #1417, #17163, #20766, #4827, #4619, #11396, #33997, #14374, #40596, #26763, #30162, #13766, #13965, #17574, #10566, #1002, #27384, #7184, #20553, #7383, #10983, #11188, #26970, #10772, #36774, #17779, #14171, #23753 ),
 ( #7591, #24173, #33583, #33791, #29951, #4415, #37183, #17372, #8005, #30778, #20976, #24382, #1627, #14582, #20143, #39772, #1212, #23545, #27175, #27587, #36566, #40189, #33166, #3993, #23966, #36985, #791, #5240, #8628, #35052, #34833, #21806, #8843, #25020, #14793, #12460, #37388, #12245, #9058, #21178, #31839, #15636, #34206, #28434, #8206, #21591, #34620 ),
 ( #5447, #28641, #17991, #2256, #5034, #38241, #1829, #38022, #31196, #5667, #22023, #24589, #41652, #28220, #18407, #2039, #28003, #37803, #40804, #30988, #41012, #11605, #31414, #37596, #15218, #34406, #5872, #25238, #41226, #12029, #18195, #18835, #18624, #31629, #41440, #2679, #8422, #27796, #11820, #21381, #15004, #24809, #2469, #15431, #9268, #32264, #13294 ),
 ( #13080, #41866, #12870, #19463, #19885, #3094, #16690, #536, #328, #6915, #22226, #32900, #3520, #26071, #2884, #3732, #22853, #26280, #16481, #6702, #29486, #29695, #35892, #25454, #22432, #6487, #35255, #116, #16266, #38451, #19042, #32472, #39289, #23068, #6079, #36101, #10095, #32047, #15847, #29269, #28853, #12664, #25654, #19671, #38661, #39080, #9469 ),
 ( #35462, #9882, #6284, #19255, #32685, #16054, #38866, #29057, #42076, #25859, #9678, #22642, #35678, #3302, #20506, #39718, #36723, #36937, #4150, #4570, #10518, #14125, #23277, #26712, #7757, #23489, #27126, #11145, #10932, #17735, #40351, #20722, #4785, #33113, #36515, #20090, #20293, #23921, #16903, #7335, #33746, #13510, #29905, #33321, #17113, #30114, #26916 ),
 ( #40140, #17529, #1160, #3943, #30736, #26499, #30530, #27339, #39503, #7962, #33954, #10309, #1370, #36313, #39930, #10723, #954, #743, #23703, #7133, #13718, #33534, #13922, #14327, #7545, #24132, #4366, #37141, #20930, #17326, #30315, #34579, #40969, #8375, #34366, #1996, #4989, #24341, #5199, #17947, #11773, #1789, #14959, #40762, #41396, #31586, #27960 ),
 ( #27551, #34787, #21133, #34163, #24764, #14751, #37762, #30949, #27752, #18362, #11559, #24544, #21761, #37977, #37551, #21340, #11355, #18153, #40557, #5621, #25192, #8586, #21549, #31157, #5406, #31368, #2211, #24978, #28390, #18577, #5829, #15170, #37345, #8165, #38196, #28176, #41181, #11984, #8802, #2424, #15385, #12201, #9012, #21977, #35009, #18784, #1584 ),
 ( #14542, #10047, #28809, #12823, #15593, #6443, #22597, #23019, #25409, #25810, #19620, #29436, #13249, #275, #35841, #38411, #12417, #35629, #36048, #6656, #9222, #61, #16430, #3254, #26233, #42025, #3468, #38819, #22180, #6862, #16214, #39237, #35210, #6037, #22804, #13031, #18998, #35412, #32633, #31796, #2634, #28598, #12619, #41607, #32002, #2841, #15800 ),
 ( #41825, #19418, #38615, #26021, #29008, #39030, #25606, #22388, #9420, #6240, #9630, #32424, #19210, #32218, #3051, #9838, #29219, #16009, #13879, #7712, #20250, #14080, #13668, #696, #32848, #30068, #27083, #39667, #3680, #23874, #20460, #26873, #26449, #36894, #10677, #30271, #10472, #36261, #905, #4318, #29858, #7081, #23440, #40091, #4105, #20045, #33276 ),
 ( #33063, #39880, #16642, #3894, #7500, #16858, #23659, #10886, #36679, #20674, #33698, #33489, #19835, #23228, #26660, #36469, #7288, #17282, #17065, #1113, #29650, #488, #13461, #39452, #10255, #25734, #29137, #13381, #13170, #196, #29358, #3384, #35335, #32990, #15723, #32773, #29576, #41739, #10178, #36186, #12543, #6782, #28727, #42154, #12950, #19336, #22311 ),
 ( #38533, #22728, #25532, #16567, #6163, #16351, #9549, #26160, #412, #2968, #19974, #6573, #25942, #22520, #6366, #16133, #19132, #9348, #32342, #32136, #38950, #15932, #9763, #12747, #26368, #3603, #35758, #19542, #38741, #39376, #32550, #39162, #19751, #23147, #28928, #41946, #3171, #7005, #35550, #9968, #22940, #35969, #29784, #10601, #33829, #13801, #3817 ),
 ( #33407, #40018, #40436, #23581, #37223, #21015, #20803, #27423, #16986, #17408, #1456, #1253, #8042, #30614, #27214, #16781, #23367, #26799, #10395, #36603, #14208, #7217, #39808, #40229, #623, #20177, #29986, #7423, #20381, #17200, #14416, #11024, #30404, #24005, #33621, #36400, #13592, #26581, #4657, #17613, #39591, #11227, #24213, #33202, #37025, #4028, #30198 ),
 ( #826, #1038, #4238, #14003, #10811, #27009, #23793, #36814, #4450, #7633, #7840, #20591, #36374, #16539, #20562, #20776, #20351, #13349, #383, #40198, #26770, #16749, #29754, #16958, #29957, #10574, #33375, #23975, #3789, #33591, #36784, #39989, #7601, #33800, #26979, #36993, #13565, #39780, #26339, #4207, #7390, #7814, #10150, #23553, #4424, #14181, #10994 ),
 ( #23120, #39345, #17171, #29549, #17382, #36156, #10781, #1221, #30170, #27184, #36574, #30372, #1011, #6973, #19944, #13975, #32964, #593, #26555, #39561, #23761, #10366, #20149, #23337, #7191, #33172, #4000, #797, #13773, #18416, #38032, #8852, #18204, #27805, #14384, #34416, #11405, #15013, #40605, #27392, #28012, #15229, #20985, #37605, #1838, #24392, #37397 ),
 ( #14802, #4836, #17789, #5044, #17999, #40813, #21390, #12038, #34006, #8638, #24818, #41021, #37813, #21816, #11831, #25029, #1637, #11614, #30587, #5249, #8432, #4628, #40403, #24599, #34629, #2265, #28229, #41235, #21601, #11197, #24183, #31205, #17583, #5456, #37192, #31423, #1426, #2048, #8014, #30787, #14591, #27596, #8214, #21187, #34215, #30997, #28443 ),
 ( #3102, #41449, #38460, #25868, #9890, #9686, #39088, #15645, #22652, #6495, #26080, #34842, #6293, #15856, #2479, #22441, #41661, #16063, #32056, #29065, #31848, #25464, #16275, #9067, #12674, #25663, #9278, #35264, #18634, #42085, #2894, #25247, #35470, #5676, #28863, #19473, #22236, #6088, #31638, #38670, #32480, #19051, #41875, #15440, #12254, #38874, #38250 ),
 ( #5882, #9477, #22033, #35061, #19264, #18844, #2688, #12879, #35686, #28650, #12469, #32272, #3309, #29279, #124, #13088, #16913, #20098, #17334, #1169, #19679, #13931, #22863, #7141, #33122, #26507, #29495, #36323, #14133, #3530, #29913, #6711, #23713, #336, #23497, #16698, #32695, #4159, #33542, #39297, #13727, #3951, #29703, #13519, #23286, #26289, #16489 ),
 ( #752, #23076, #26720, #19894, #20514, #10731, #39728, #10527, #32909, #4374, #36524, #7343, #26926, #36731, #36110, #13302, #39512, #30325, #6924, #10105, #27135, #3740, #544, #10318, #7554, #20303, #35900, #33329, #17122, #30122, #962, #40148, #39939, #2220, #28183, #27969, #34585, #7766, #5414, #31164, #40770, #30540, #18369, #8383, #11781, #24348, #11153 ),
 ( #30743, #24140, #40565, #37769, #17955, #37148, #34170, #34373, #1592, #2005, #7970, #11568, #20730, #20938, #5206, #33963, #24553, #8593, #21347, #15179, #21557, #18161, #10941, #1378, #4792, #17538, #17743, #14967, #14336, #14549, #40978, #23930, #27346, #27558, #11363, #37355, #8173, #31376, #24771, #37558, #36945, #33754, #40358, #4580, #21141, #4997, #30956 ),
 ( #1796, #14759, #27759, #41614, #24986, #9426, #9229, #31594, #28816, #32430, #22187, #25817, #2641, #31804, #11991, #32008, #12829, #28604, #15601, #3261, #37985, #32226, #18586, #2431, #12424, #12210, #25416, #28398, #15392, #15808, #41403, #25199, #19216, #35419, #38204, #9021, #8810, #21984, #21768, #3058, #22604, #35217, #38417, #35017, #2848, #6043, #38825 ),
 ( #16015, #16221, #41831, #34795, #5628, #35636, #19005, #5837, #18791, #12625, #25613, #38623, #22396, #6450, #6247, #29014, #42034, #9636, #19424, #41188, #39675, #7507, #26239, #10262, #13038, #3902, #20052, #20466, #22811, #23235, #17072, #26879, #10684, #39887, #33283, #35849, #9844, #33071, #33495, #4112, #6663, #10478, #13886, #705, #23665, #39461, #912 ),
 ( #4325, #13676, #36685, #19626, #32641, #20256, #23447, #3474, #32856, #30075, #29227, #68, #26028, #10055, #39037, #16436, #29443, #282, #26667, #36270, #13255, #16865, #36056, #36475, #26457, #7295, #39246, #19842, #6869, #23026, #496, #3688, #16649, #29656, #13468, #29865, #7090, #34540, #17289, #34331, #31118, #1119, #11731, #37724, #14088, #8332, #30278 ),
 ( #20888, #23880, #30692, #8548, #40097, #24298, #27089, #18113, #36899, #17906, #11105, #10893, #40721, #27919, #33706, #8121, #14497, #24094, #7922, #17693, #20682, #7718, #33912, #4527, #27511, #17491, #1542, #14288, #14915, #5159, #40519, #11311, #27297, #40925, #34119, #37304, #21302, #1955, #30487, #1330, #4740, #24720, #40312, #37104, #21507, #21095, #4946 ),
 ( #30910, #1748, #14707, #27712, #11516, #24501, #37506, #15757, #32170, #18955, #3006, #15554, #19166, #28556, #28129, #25768, #31961, #15965, #41139, #11945, #38567, #28762, #24936, #8966, #9380, #22555, #22344, #9586, #28346, #35367, #28963, #38775, #5366, #2800, #41564, #15126, #35165, #12157, #41776, #2594, #12576, #2381, #38153, #41979, #21719, #25360, #38365 ),
 ( #31323, #25563, #12372, #37934, #5992, #18321, #9179, #12778, #21934, #6197, #2167, #8757, #34743, #5574, #18532, #31537, #15341, #41355, #25150, #34963, #5786, #18741, #31751, #22136, #39194, #19, #6816, #13834, #16168, #444, #19371, #36430, #12985, #36216, #29391, #3206, #16815, #4063, #9796, #26403, #32805, #231, #26190, #36004, #38986, #29173, #10002 ),
 ( #35795, #19786, #32586, #33235, #23399, #3636, #16601, #3419, #17023, #10211, #29609, #26615, #7249, #6607, #25978, #22974, #861, #19578, #22762, #30021, #16386, #32377, #13208, #20208, #13414, #35585, #23181, #39408, #7037, #20005, #26832, #33022, #39839, #10636, #10428, #6402, #3851, #29817, #13624, #656, #39622, #31066, #21049, #24454, #37057, #23829, #27459 ),
 ( #36848, #11057, #8282, #30649, #7667, #4691, #4901, #14241, #14657, #20625, #24249, #33444, #33655, #17856, #4480, #37257, #21252, #34075, #27870, #34282, #30857, #14867, #1069, #17440, #30230, #30437, #1702, #27041, #1283, #27661, #23615, #40050, #27248, #40263, #24042, #7875, #5111, #40672, #8075, #20838, #11464, #37458, #40879, #36636, #18063, #17647, #4271 ),
 ( #1904, #33862, #7458, #1492, #14449, #20416, #10843, #40472, #11263, #17234, #14037, #37675, #22091, #21880, #2114, #41512, #3541, #34906, #38517, #15289, #2329, #24666, #2543, #25517, #41301, #28294, #16502, #8498, #2751, #31271, #15077, #12105, #24885, #25094, #41088, #28077, #28504, #11896, #37882, #31914, #5945, #8705, #21668, #21455, #34692, #34485, #15707 ),
 ( #12319, #5522, #5317, #35118, #22297, #18479, #15504, #8914, #31484, #38099, #5738, #18691, #18268, #31701, #25306, #38310, #9130, #18904, #28711, #9334, #41721, #12526, #35322, #6722, #19690, #32707, #29509, #11679, #30333, #13531, #6936, #16924, #7776, #556, #16711, #40158, #19907, #26301, #7152, #1180, #10329, #348, #30134, #29714, #29924, #36535, #36955 ),
 ( #13940, #27146, #10539, #14143, #23508, #23088, #20739, #26938, #10950, #36122, #32922, #33554, #10743, #3753, #3963, #4386, #17548, #17344, #4589, #23938, #33764, #13315, #39949, #7354, #10117, #973, #20111, #23724, #39740, #36742, #39525, #33133, #39310, #26518, #20313, #33340, #762, #13738, #23299, #7564, #4170, #36336, #20524, #26732, #17132, #15189, #34179 ),
 ( #21355, #2228, #17964, #5005, #34803, #14344, #21565, #7978, #20946, #30964, #1600, #1805, #17750, #33971, #5215, #4799, #30750, #8602, #24780, #14557, #27564, #40367, #11370, #27354, #34593, #12001, #24562, #27768, #40573, #34381, #40779, #28192, #8181, #30549, #5422, #5637, #18169, #11162, #24147, #24994, #11576, #24357, #37361, #14766, #37566, #8393, #31172 ),
 ( #18377, #31386, #11789, #41198, #1388, #40986, #8818, #21149, #2013, #37156, #14976, #27977, #21777, #37778, #37994, #6459, #16229, #78, #29235, #22611, #12218, #41411, #22404, #39045, #35644, #38212, #29024, #3270, #32234, #13046, #28825, #32439, #41839, #25208, #9851, #3066, #26036, #9029, #21994, #9644, #42042, #35025, #22197, #19433, #35858, #22821, #18594 ),
 ( #5846, #12838, #31603, #16024, #2441, #12635, #15402, #25621, #18801, #28406, #25825, #31812, #2648, #15608, #28613, #38834, #41622, #35226, #12431, #25424, #38425, #9238, #6051, #19013, #32018, #2856, #15817, #38632, #9435, #35429, #6254, #19224, #17080, #3911, #918, #3697, #39469, #30284, #23034, #26675, #39683, #10272, #7098, #32649, #30080, #16873, #39256 ),
 ( #36065, #32865, #26464, #16657, #20059, #4330, #4120, #33290, #20263, #36483, #26247, #23888, #6671, #23670, #20474, #3486, #1126, #27094, #16445, #39894, #19634, #33080, #29873, #23243, #13263, #712, #40103, #29451, #13685, #290, #7513, #10063, #7304, #505, #6880, #13893, #17295, #19851, #10486, #23456, #13477, #36277, #26885, #29663, #10691, #36689, #33500 ),
 ( #14095, #10898, #34549, #24729, #37311, #8127, #33918, #5374, #11525, #4953, #27927, #37732, #7928, #1336, #11318, #2176, #37109, #11112, #18329, #14294, #20689, #1550, #8556, #4747, #36905, #24508, #24101, #24306, #30917, #15135, #33714, #40934, #7723, #21102, #34126, #40526, #27305, #17912, #28138, #17497, #1756, #4535, #21515, #40320, #37515, #30700, #30495 ),
 ( #20896, #27718, #14715, #14504, #27519, #40727, #17700, #8340, #21308, #34338, #5166, #18121, #31126, #1963, #31331, #41146, #14925, #11742, #11952, #22564, #41783, #35174, #15972, #12786, #38161, #31544, #41573, #32386, #25160, #41362, #35593, #2390, #8768, #31759, #25776, #34971, #24943, #12583, #12165, #12382, #18963, #19382, #2602, #16179, #29, #41988, #6410 ),
 ( #3015, #25572, #15349, #3217, #22351, #38784, #38373, #8975, #28773, #28970, #15561, #21942, #25369, #9594, #31970, #5794, #6001, #6205, #28564, #29182, #18751, #38576, #34751, #9187, #19176, #22143, #9388, #37943, #35376, #21728, #5584, #32182, #18541, #28354, #2807, #15768, #19795, #23407, #16394, #22985, #7256, #12993, #29400, #39204, #32815, #36012, #26413 ),
 ( #39631, #26622, #664, #32596, #30237, #25987, #30029, #26840, #38996, #7465, #3645, #9805, #3859, #39848, #453, #29618, #17243, #22773, #4071, #3429, #240, #13425, #26200, #39417, #13217, #10012, #29825, #6826, #16610, #33242, #20216, #10220, #23190, #35804, #36224, #6618, #17031, #36643, #7046, #20012, #33031, #16823, #13632, #10643, #10436, #19586, #869 ),
 ( #36438, #13842, #23624, #20425, #33452, #4280, #1291, #14456, #40271, #40885, #31072, #1500, #27468, #11066, #11687, #17863, #11272, #34289, #1912, #14248, #7675, #17654, #8504, #27256, #17447, #24673, #20634, #27050, #7883, #14874, #24050, #1077, #30863, #30446, #30655, #37263, #37682, #20845, #34492, #18276, #18071, #21462, #40057, #5323, #21259, #1709, #33663 ),
 ( #4488, #5118, #11471, #37065, #4700, #27876, #14046, #10850, #23837, #33870, #36858, #40478, #24255, #8082, #14664, #21055, #34081, #27668, #4908, #24460, #40679, #37465, #8289, #21886, #12735, #5528, #9137, #22096, #34914, #31708, #15083, #41727, #41519, #21675, #18910, #22510, #12325, #15921, #5745, #31921, #8713, #6358, #31277, #6153, #2957, #28084, #25725 ),
 ( #22302, #2120, #15510, #28511, #18697, #37888, #2549, #9539, #11902, #38318, #41095, #32126, #34699, #2756, #25102, #24891, #12532, #41936, #18485, #35124, #25313, #38105, #5950, #15713, #31491, #2336, #28716, #15295, #25521, #28301, #38522, #41307, #28919, #19119, #9338, #35326, #12112, #38732, #35538, #8921, #10385, #7208, #32542, #25933, #35960, #26789, #19535 ),
 ( #38942, #3163, #26150, #20168, #29347, #19328, #6995, #35749, #6774, #13372, #13791, #39153, #10592, #36594, #36392, #816, #16125, #39800, #39580, #19964, #9753, #23572, #16770, #33191, #32762, #3375, #23138, #23357, #9959, #16342, #19742, #4020, #26359, #188, #402, #612, #22930, #16977, #13161, #32982, #29128, #3595, #13584, #16558, #3807, #29976, #29775 ),
 ( #26572, #32333, #22721, #29568, #6564, #39366, #42148, #10170, #36176, #12942, #7411, #23783, #33609, #27205, #17399, #20794, #5066, #4856, #34030, #21006, #40628, #24621, #24411, #11636, #30394, #37418, #21209, #40834, #20373, #17812, #30606, #17190, #37215, #14198, #30809, #4647, #1658, #4441, #40218, #31018, #36805, #27413, #40424, #11015, #7831, #33396, #14613 ),
 ( #27617, #4229, #7623, #1243, #23994, #37013, #33819, #18020, #11425, #8237, #34235, #8034, #26999, #30188, #1030, #1861, #14823, #13994, #27826, #40009, #10801, #20582, #17603, #1446, #14405, #11219, #24203, #8871, #15876, #18224, #2498, #21412, #38478, #2069, #38270, #31442, #5274, #18864, #6108, #11853, #28463, #34863, #2285, #28249, #38052, #41043, #31225 ),
 ( #5694, #37835, #21834, #34648, #35283, #25483, #18654, #31659, #5476, #19072, #12276, #15462, #28670, #9297, #8662, #15034, #12061, #2915, #21622, #24840, #32078, #28034, #34439, #15248, #22259, #18436, #37629, #25266, #41254, #25048, #41468, #28883, #9086, #41895, #12693, #12488, #8454, #22052, #35081, #15664, #5902, #31868, #2708, #41681, #26529, #39109, #25888 ),
 ( #3331, #13324, #3121, #771, #25685, #566, #39534, #9497, #20120, #3973, #22461, #16721, #38690, #9914, #22884, #29302, #32292, #35922, #16934, #6313, #32719, #35492, #10340, #16081, #26312, #19492, #19286, #6949, #36347, #42106, #16512, #6732, #32503, #16300, #26104, #29086, #12900, #146, #38895, #19700, #9708, #3553, #22673, #23311, #13540, #29518, #358 ),
 ( #39320, #10126, #29724, #7161, #35708, #6517, #13112, #33145, #23098, #36131, #29933, #19917, #32932, #3762, #2184, #23734, #13748, #1396, #30145, #1191, #7786, #8775, #33564, #5592, #31552, #31339, #37951, #10550, #21735, #33977, #14352, #33350, #34758, #11170, #15142, #27154, #13950, #17556, #18335, #4397, #26948, #14151, #41152, #20747, #39960, #36965, #37163 ) ),
 .UNSPECIFIED., .F., .F., .F.,
 ( 4, 1, 1, 1, 1, 1, 1, 1, 1, 1, 1, 1, 1, 1, 1, 1, 1, 1, 1, 1, 1, 1, 1, 1, 1, 1, 1, 1, 1, 1, 1, 1, 1, 1, 1, 1, 1, 1, 1, 1, 1, 1, 1, 1, 1, 1, 4 ),
 ( 4, 1, 1, 1, 1, 1, 1, 1, 1, 1, 1, 1, 2, 1, 1, 1, 2, 1, 1, 1, 1, 1, 2, 1, 1, 1, 1, 1, 1, 1, 2, 1, 1, 1, 1, 1, 1, 1, 1, 1, 4 ),
 ( 0.000000000000000000, 0.007812500000000000000, 0.01562500000000000000, 0.02343750000000000000, 0.03125000000000000000, 0.04687500000000000000, 0.06250000000000000000, 0.07812500000000000000, 0.09375000000000000000, 0.1093750000000000000, 0.1250000000000000000, 0.1406250000000000000, 0.1562500000000000000, 0.1875000000000000000, 0.2187500000000000000, 0.2500000000000000000, 0.2812500000000000000, 0.3125000000000000000, 0.3281250000000000000, 0.3437500000000000000, 0.3750000000000000000, 0.4062500000000000000, 0.4375000000000000000, 0.4687500000000000000, 0.5000000000000000000, 0.5312500000000000000, 0.5625000000000000000, 0.5937500000000000000, 0.6250000000000000000, 0.6562500000000000000, 0.6718750000000000000, 0.6875000000000000000, 0.7187500000000000000, 0.7500000000000000000, 0.7812500000000000000, 0.8125000000000000000, 0.8437500000000000000, 0.8750000000000000000, 0.8906250000000000000, 0.9062500000000000000, 0.9218750000000000000, 0.9375000000000000000, 0.9531250000000000000, 0.9687500000000000000, 0.9765625000000000000, 0.9843750000000000000, 1.000000000000000000 ),
 ( 0.000000000000000000, 0.01539374999999999945, 0.03078749999999999890, 0.04618125000000002089, 0.06157499999999999779, 0.07696875000000003020, 0.09236250000000004179, 0.1077562499999999979, 0.1231499999999999956, 0.1431375000000000008, 0.1631250000000000200, 0.1831125000000000114, 0.2031000000000000028, 0.2063375000000000070, 0.2095750000000000113, 0.2128125000000000155, 0.2160500000000000198, 0.2667375000000000163, 0.3174250000000000682, 0.3681125000000000647, 0.4188000000000000611, 0.5201750000000000540, 0.6215500000000000469, 0.6266374999999999584, 0.6317250000000000920, 0.6368124999999997815, 0.6418999999999999151, 0.6469874999999999376, 0.6520749999999999602, 0.6571624999999999828, 0.6622500000000000053, 0.7044687500000000879, 0.7466875000000001705, 0.7889062500000000311, 0.8010555555555555207, 0.8311249999999998916, 0.8733437499999998632, 0.9155625000000000568, 0.9403166666666666895, 0.9577812500000000284, 1.000000000000000000 ),
 .UNSPECIFIED. ) ;
#10615=ORIENTED_EDGE ( 'NONE', *, *, #32998, .F. ) ;
#10617=CARTESIAN_POINT ( 'NONE',  ( 8.354336569859343697, 119.9739600045604675, -1.115347381135292970 ) ) ;
#10618=CARTESIAN_POINT ( 'NONE',  ( -2.490049542275868166, 107.2224589468338536, -4.730309301830580182 ) ) ;
#10619=CARTESIAN_POINT ( 'NONE',  ( 4.554505725324297316, 118.0858391265290805, 0.7375152256654264882 ) ) ;
#10620=CARTESIAN_POINT ( 'NONE',  ( -16.25331603292288563, 145.9442052555630767, -1.443193537303810059 ) ) ;
#10621=CARTESIAN_POINT ( 'NONE',  ( -1.187503523883304712, 115.7029482321909200, -1.742292230791464336 ) ) ;
#10622=CARTESIAN_POINT ( 'NONE',  ( 0.7493318530476299477, 117.9496056092839069, -1.372937156641410361 ) ) ;
#10624=DIRECTION ( 'NONE',  ( -0.9998004120163608288, 0.000000000000000000, -0.01997839162482749342 ) ) ;
#10625=CARTESIAN_POINT ( 'NONE',  ( -10.02184412846599315, 123.2077283916686525, -1.294377628214502751 ) ) ;
#10629=CARTESIAN_POINT ( 'NONE',  ( 8.325883379001766116, 120.1130057568717433, -1.118334525995474227 ) ) ;
#10630=CARTESIAN_POINT ( 'NONE',  ( -8.882710456238886110, 123.9526509987454261, -0.04472055067538689005 ) ) ;
#10633=CARTESIAN_POINT ( 'NONE',  ( 22.70904429024572835, 149.7444054411783441, 1.421740456058896207 ) ) ;
#10635=CARTESIAN_POINT ( 'NONE',  ( 2.816406720412386822, -15.24816796146632925, 4.372395393210481984 ) ) ;
#10636=CARTESIAN_POINT ( 'NONE',  ( -18.50101540898971919, 149.0103496150362901, 1.723905467370217437 ) ) ;
#10637=CARTESIAN_POINT ( 'NONE',  ( -0.9160044981361634697, -1.370538221358817310, 0.3309596765904046500 ) ) ;
#10638=CARTESIAN_POINT ( 'NONE',  ( -7.949750681159734711, 158.6775731370129279, -0.5882489250746234521 ) ) ;
#10639=CARTESIAN_POINT ( 'NONE',  ( -0.9749442489646007459, 26.91501818708639249, 0.01812370653153724809 ) ) ;
#10642=CARTESIAN_POINT ( 'NONE',  ( 5.744069310734388090, 120.3160329940760818, 0.4351690567359403072 ) ) ;
#10643=CARTESIAN_POINT ( 'NONE',  ( -3.102522256439491422, 156.1450793681712241, 0.6153187215006974409 ) ) ;
#10644=CARTESIAN_POINT ( 'NONE',  ( 3.520038346949750707, -14.46602075298747359, 5.128058278438484052 ) ) ;
#10645=CARTESIAN_POINT ( 'NONE',  ( 17.77977776825574452, 147.3864036964934598, -1.530147356706996309 ) ) ;
#10647=CARTESIAN_POINT ( 'NONE',  ( -19.28990034181461510, 145.1342744731992127, -2.527759927608660195 ) ) ;
#10648=CARTESIAN_POINT ( 'NONE',  ( 4.835342064185105926, 104.6144662015457527, -0.09903605035092130637 ) ) ;
#10649=CARTESIAN_POINT ( 'NONE',  ( 2.995043271588619493, -14.66878921821561299, 4.005342282345994320 ) ) ;
#10650=CARTESIAN_POINT ( 'NONE',  ( -4.874430425846600023, 117.4785343618161875, -1.135543576852563463 ) ) ;
#10651=CARTESIAN_POINT ( 'NONE',  ( 9.140193528981123805, 153.9061766533773152, -0.01708403265280362612 ) ) ;
#10653=CARTESIAN_POINT ( 'NONE',  ( -5.219734918942418034, 114.8006916078311690, 1.211930405771829866 ) ) ;
#10654=CARTESIAN_POINT ( 'NONE',  ( 4.549352062591466073, 112.0094687158549789, 2.856336935586818448 ) ) ;
#10655=PLANE ( 'NONE',  #32041 ) ;
#10656=CARTESIAN_POINT ( 'NONE',  ( -4.974001918040873882, 117.3966124607983659, -0.9751453929904890794 ) ) ;
#10658=CARTESIAN_POINT ( 'NONE',  ( 15.85175717768486514, 121.0146182718019645, 0.1572851932169303801 ) ) ;
#10659=CARTESIAN_POINT ( 'NONE',  ( -6.555005513994535572E-14, 79.34146620154574236, -6.390659674827382268E-18 ) ) ;
#10660=CARTESIAN_POINT ( 'NONE',  ( 2.108464161424454364, -15.40773383333050894, 5.967785631577029903 ) ) ;
#10663=CARTESIAN_POINT ( 'NONE',  ( 4.785842063580148853, 158.3075559295907055, 1.719165798332183082 ) ) ;
#10664=ORIENTED_EDGE ( 'NONE', *, *, #10228, .F. ) ;
#10665=CARTESIAN_POINT ( 'NONE',  ( -1.660137282266059611, 14.53371390510571004, 8.268994913937449454 ) ) ;
#10666=CARTESIAN_POINT ( 'NONE',  ( -2.311280081344418313, 117.1825730503849456, -0.6599811042350863799 ) ) ;
#10667=CARTESIAN_POINT ( 'NONE',  ( -2.416298757281930776, 119.8248006784163380, -0.5703471319689767949 ) ) ;
#10669=DIRECTION ( 'NONE',  ( 0.01997839162482749689, 1.040247600000945640E-18, -0.9998004120163610509 ) ) ;
#10670=CARTESIAN_POINT ( 'NONE',  ( -5.018108817528237786, 104.6144662015435358, 1.816817646635351613 ) ) ;
#10672=CARTESIAN_POINT ( 'NONE',  ( -4.399545650080316506, 2.442302885307133131, -1.471791394725967095 ) ) ;
#10674=CARTESIAN_POINT ( 'NONE',  ( -4.848171622920200541, 115.6909491485453003, 1.282745750490223324 ) ) ;
#10675=CARTESIAN_POINT ( 'NONE',  ( 3.347306494706169477, -13.94864326390300668, 3.303819676456750898 ) ) ;
#10676=CARTESIAN_POINT ( 'NONE',  ( 3.181806805318111220, 118.0279923103727242, -0.7725587567394767152 ) ) ;
#10677=CARTESIAN_POINT ( 'NONE',  ( -22.18008199021001303, 150.6715983490228723, 0.5179974990882320052 ) ) ;
#10681=VERTEX_POINT ( 'NONE', #25057 ) ;
#10682=CARTESIAN_POINT ( 'NONE',  ( -4.382135906878160903, 104.6144662015457811, -2.048376150530189843 ) ) ;
#10683=CARTESIAN_POINT ( 'NONE',  ( 4.856922264871083250, -15.58127974107270575, 2.741789226191331252 ) ) ;
#10684=CARTESIAN_POINT ( 'NONE',  ( -20.06821085608268618, 149.3093937917295762, 1.664735353294634290 ) ) ;
#10685=CARTESIAN_POINT ( 'NONE',  ( -0.2095918955067871126, -8.989892990265463624, -4.636818132431064221 ) ) ;
#10687=DIRECTION ( 'NONE',  ( -0.9998004120163608288, 1.039227405372657318E-20, -0.01997839162482760098 ) ) ;
#10689=CARTESIAN_POINT ( 'NONE',  ( 0.3459730346047664717, 118.1497763966932695, 1.075889458897477891 ) ) ;
#10691=CARTESIAN_POINT ( 'NONE',  ( -1.906664127224672489, 156.5995568990359175, 1.114948187579593242 ) ) ;
#10693=CARTESIAN_POINT ( 'NONE',  ( 18.32188643113664739, 147.9371514012413229, -1.660510838394361866 ) ) ;
#10694=CARTESIAN_POINT ( 'NONE',  ( -12.41171712301742502, 121.5863879130357503, -1.717582910027388499 ) ) ;
#10697=CARTESIAN_POINT ( 'NONE',  ( 4.118366482596429456, 118.2429491485453354, -0.1862083956823271380 ) ) ;
#10698=CARTESIAN_POINT ( 'NONE',  ( 4.393282770141039961, 155.8497297829079571, -0.4427821657071675521 ) ) ;
#10699=ORIENTED_EDGE ( 'NONE', *, *, #41321, .F. ) ;
#10700=CARTESIAN_POINT ( 'NONE',  ( 2.368424984008928202, -15.31393412036581658, 4.927583237414308037 ) ) ;
#10701=CARTESIAN_POINT ( 'NONE',  ( -5.008552712180506461, 117.3993836135855560, 0.7755994290793736257 ) ) ;
#10702=AXIS2_PLACEMENT_3D ( 'NONE', #40966, #12199, #31366 ) ;
#10704=CARTESIAN_POINT ( 'NONE',  ( -4.468841950160419962, 8.124252568732815760, -1.173904233648782158 ) ) ;
#10705=CARTESIAN_POINT ( 'NONE',  ( -0.008308630153283404207, 120.0570981805881559, 0.4157978282972239481 ) ) ;
#10706=CARTESIAN_POINT ( 'NONE',  ( 0.3073029101277962583, 33.80961766112287847, 0.5411155679567926091 ) ) ;
#10707=B_SPLINE_CURVE_WITH_KNOTS ( 'NONE', 3,
 ( #29023, #3695, #42041, #16872, #289, #38631, #32864, #32438, #35857, #12837, #3484, #13476 ),
 .UNSPECIFIED., .F., .F.,
 ( 4, 2, 2, 2, 2, 4 ),
 ( 0.000000000000000000, 0.1320156187279750426, 0.1980234280919625778, 0.2640312374559500852, 0.3918846486443439692, 0.3959276339151724944 ),
 .UNSPECIFIED. ) ;
#10708=CARTESIAN_POINT ( 'NONE',  ( 0.7007450612751181529, 9.901275517365906609, -4.597291952374415125 ) ) ;
#10709=CARTESIAN_POINT ( 'NONE',  ( 15.52555164710810232, 147.5317938866932366, 0.3613967763117282850 ) ) ;
#10713=CARTESIAN_POINT ( 'NONE',  ( -5.550348810799227373, 116.7477450504428731, -0.3527803593980367580 ) ) ;
#10717=CARTESIAN_POINT ( 'NONE',  ( 5.540715274600516160, 6.338079305180906786, 6.343128766557815545 ) ) ;
#10721=EDGE_CURVE ( 'NONE', #21991, #6038, #25640, .T. ) ;
#10723=CARTESIAN_POINT ( 'NONE',  ( -15.39314341005352738, 120.8297411738997624, 0.1127201291141931849 ) ) ;
#10724=VERTEX_POINT ( 'NONE', #14830 ) ;
#10726=CARTESIAN_POINT ( 'NONE',  ( 7.800415316508575003, 122.5706186015670767, -0.04211976961263740743 ) ) ;
#10728=DIRECTION ( 'NONE',  ( 0.01997839162482749689, 1.040247600000944870E-18, -0.9998004120163610509 ) ) ;
#10729=CARTESIAN_POINT ( 'NONE',  ( -15.64085066085090681, 147.2198192248932571, -0.3637928714071056446 ) ) ;
#10730=CARTESIAN_POINT ( 'NONE',  ( 3.233725904218312408, -15.30436843596319463, 5.598328752637605099 ) ) ;
#10731=CARTESIAN_POINT ( 'NONE',  ( -4.041216738203083914, 118.0179939250997023, 0.7376333572805303662 ) ) ;
#10732=CARTESIAN_POINT ( 'NONE',  ( -4.050807963365556930, 30.95410787014092335, -2.229501126309402448 ) ) ;
#10733=CARTESIAN_POINT ( 'NONE',  ( 23.12711913739482839, 149.5941399179437781, 0.9155080916133792046 ) ) ;
#10735=CARTESIAN_POINT ( 'NONE',  ( 4.377640660406503237, 26.40621510375495973, 1.544744264128281364 ) ) ;
#10736=CARTESIAN_POINT ( 'NONE',  ( -0.06867543354984582959, -8.127513596672324425, -0.9731866935420671050 ) ) ;
#10737=CARTESIAN_POINT ( 'NONE',  ( -22.64163882069516376, 150.6401102206664291, -0.6810593374908544551 ) ) ;
#10739=EDGE_CURVE ( 'NONE', #14389, #11424, #16282, .T. ) ;
#10740=CARTESIAN_POINT ( 'NONE',  ( 4.862091962581056137, 117.4116108956684030, 1.165648838277617338 ) ) ;
#10742=CARTESIAN_POINT ( 'NONE',  ( -5.551342799028650354, 116.9755805007568483, 0.3845323937588601138 ) ) ;
#10743=CARTESIAN_POINT ( 'NONE',  ( -10.18365381109015821, 122.2967958330617648, 1.106735498401915985 ) ) ;
#10745=CARTESIAN_POINT ( 'NONE',  ( 7.877908914988192457, 118.7344292658239340, 1.218006232967851377 ) ) ;
#10746=CARTESIAN_POINT ( 'NONE',  ( 12.77186547895197499, 122.8260676081006153, -1.334005200199291252 ) ) ;
#10747=CARTESIAN_POINT ( 'NONE',  ( -0.7316449863892299232, -12.60219034754442902, -0.6469547163463490458 ) ) ;
#10748=CARTESIAN_POINT ( 'NONE',  ( -20.80232463633032225, 150.1670661137953289, -2.219268881695795059 ) ) ;
#10750=CARTESIAN_POINT ( 'NONE',  ( 4.835304301806635507, 104.6144662015456959, -0.09947441844414706136 ) ) ;
#10751=CARTESIAN_POINT ( 'NONE',  ( 13.14213916796041559, 130.8944540161131442, -0.9043360416341283958 ) ) ;
#10752=CARTESIAN_POINT ( 'NONE',  ( 7.836112336079962049, 122.3275008022818326, 0.6979122178994436876 ) ) ;
#10754=CARTESIAN_POINT ( 'NONE',  ( -17.85978967527205441, 148.7876888829155746, -2.377023446492704473 ) ) ;
#10755=CARTESIAN_POINT ( 'NONE',  ( 3.150932678494966055, -15.78083729861913476, 4.935700751529307873 ) ) ;
#10757=CARTESIAN_POINT ( 'NONE',  ( -4.680464983510406185, 117.9617385798577942, -0.8792464480512792724 ) ) ;
#10760=CARTESIAN_POINT ( 'NONE',  ( 4.065926199369043204, 118.2429491485453497, 0.3080910687088499467 ) ) ;
#10761=CARTESIAN_POINT ( 'NONE',  ( 11.51381720411931830, 123.3156264706956478, 1.674137098916062660 ) ) ;
#10764=CARTESIAN_POINT ( 'NONE',  ( 15.72215902125767606, 120.8394623874526275, 0.2972128523334376382 ) ) ;
#10767=CARTESIAN_POINT ( 'NONE',  ( 6.775881838314501415, 16.25650946394821617, 5.045332117489572887 ) ) ;
#10768=CARTESIAN_POINT ( 'NONE',  ( 0.6211475606395560067, 120.8480686026657196, 0.1701230225530363793 ) ) ;
#10769=CARTESIAN_POINT ( 'NONE',  ( 3.136615966272614742, 159.3365417412370562, -0.7296721229192899560 ) ) ;
#10771=FACE_OUTER_BOUND ( 'NONE', #35325, .T. ) ;
#10772=CARTESIAN_POINT ( 'NONE',  ( -8.070121050663757956, 158.6666700270975525, -0.1062422583151902272 ) ) ;
#10773=ORIENTED_EDGE ( 'NONE', *, *, #25441, .F. ) ;
#10775=CARTESIAN_POINT ( 'NONE',  ( 5.711181965518192349, 121.0140050728914076, -0.3875387523984055727 ) ) ;
#10776=CARTESIAN_POINT ( 'NONE',  ( 6.475569851349685990, -13.49999789469196365, 0.1848929821133123153 ) ) ;
#10778=CARTESIAN_POINT ( 'NONE',  ( -0.6563489144271578146, 156.3175253132196190, -0.2722359314208550041 ) ) ;
#10779=CARTESIAN_POINT ( 'NONE',  ( 2.009495809369673314, -15.14277677434763802, 5.899592854099822148 ) ) ;
#10781=CARTESIAN_POINT ( 'NONE',  ( -4.901524533163420294, 117.5843641943970681, 0.6192240155325965389 ) ) ;
#10783=CARTESIAN_POINT ( 'NONE',  ( 22.53260066761437486, 150.7862151120626777, 0.5269028172337441029 ) ) ;
#10784=ORIENTED_EDGE ( 'NONE', *, *, #36085, .F. ) ;
#10785=CARTESIAN_POINT ( 'NONE',  ( 3.745621265272091716, -10.50169880513956322, -2.708184146228840294 ) ) ;
#10786=CARTESIAN_POINT ( 'NONE',  ( -22.66341594453909281, 150.6395781703034231, -0.4783972420343528542 ) ) ;
#10790=ORIENTED_EDGE ( 'NONE', *, *, #12808, .F. ) ;
#10791=CARTESIAN_POINT ( 'NONE',  ( 6.543339688405037435, 119.8646354556796894, 1.246904736843251982 ) ) ;
#10792=CARTESIAN_POINT ( 'NONE',  ( 3.235533175430977515, 2.501875212487111977, 3.308963532380430284 ) ) ;
#10793=CARTESIAN_POINT ( 'NONE',  ( 19.75679031132823127, 152.3633698111425758, 1.804147069793666347 ) ) ;
#10796=CARTESIAN_POINT ( 'NONE',  ( 5.883429839103449410, 118.5625182843610617, -0.8957466683066145352 ) ) ;
#10797=CARTESIAN_POINT ( 'NONE',  ( 4.571311019248293306, -6.119132638730012452, 0.7325351754658009362 ) ) ;
#10798=CARTESIAN_POINT ( 'NONE',  ( -10.35357550766360646, 157.8614378686282862, -1.168524991271691515 ) ) ;
#10800=EDGE_CURVE ( 'NONE', #24363, #15693, #21541, .T. ) ;
#10801=CARTESIAN_POINT ( 'NONE',  ( -10.33307603652750828, 126.0505730134521230, -0.02860894079130314391 ) ) ;
#10803=CARTESIAN_POINT ( 'NONE',  ( 6.002709446384779213, -13.95775275001606630, 2.224537231649871494 ) ) ;
#10805=CARTESIAN_POINT ( 'NONE',  ( -6.604303299200508256E-14, 94.83546620154572793, -1.207165459215201580E-19 ) ) ;
#10806=CARTESIAN_POINT ( 'NONE',  ( -0.08181223041124258133, 118.1651005001092045, -0.8941161664445478330 ) ) ;
#10808=CARTESIAN_POINT ( 'NONE',  ( 11.41083474541176024, 122.2847249198043471, 1.726555165334429987 ) ) ;
#10811=CARTESIAN_POINT ( 'NONE',  ( -2.968319594835739483, 117.2422168882539211, 0.4889809032577733250 ) ) ;
#10812=EDGE_CURVE ( 'NONE', #14129, #35669, #32457, .T. ) ;
#10813=CARTESIAN_POINT ( 'NONE',  ( 2.407351327831447119, 1.847773219181642057, 8.093752867084216263 ) ) ;
#10814=CARTESIAN_POINT ( 'NONE',  ( 11.38067935084455762, 126.1532465342912985, 1.245950066931533096 ) ) ;
#10815=CARTESIAN_POINT ( 'NONE',  ( -3.682264917456323783, 82.13546620154573930, -0.07358041635423923088 ) ) ;
#10816=CARTESIAN_POINT ( 'NONE',  ( 15.74805233916999292, 121.4292885696920621, -0.3002298764450369584 ) ) ;
#10822=CARTESIAN_POINT ( 'NONE',  ( -4.447578949651058267, 118.1635636769329665, 0.4463883187089059401 ) ) ;
#10824=EDGE_LOOP ( 'NONE', ( #17908, #40243, #6262, #19009 ) ) ;
#10827=CARTESIAN_POINT ( 'NONE',  ( -6.079163865392237298, 119.4949355251708454, -1.258858988448749106 ) ) ;
#10829=CARTESIAN_POINT ( 'NONE',  ( -7.639005212201317896, 124.2918010433613745, -0.1615048153450349133 ) ) ;
#10830=CARTESIAN_POINT ( 'NONE',  ( 4.468651703854161994, 118.1302808690484625, 0.7051366077090519546 ) ) ;
#10831=CARTESIAN_POINT ( 'NONE',  ( -6.262986112992452448, 155.3815620563194955, -0.9009107504210206452 ) ) ;
#10832=CYLINDRICAL_SURFACE ( 'NONE', #15176, 5.588000000000006295 ) ;
#10833=CARTESIAN_POINT ( 'NONE',  ( 3.202712377253894793, 117.9496042817458914, -1.175034297761716529 ) ) ;
#10834=CARTESIAN_POINT ( 'NONE',  ( -10.14627733936766241, 123.6566696788710686, -1.220144418243291007 ) ) ;
#10838=CARTESIAN_POINT ( 'NONE',  ( -7.534622205921475135, 122.4254553736845281, -0.03076868180150949678 ) ) ;
#10840=CARTESIAN_POINT ( 'NONE',  ( 1.349732659537954405, 159.5224216140176168, 0.6194554754934781249 ) ) ;
#10842=CARTESIAN_POINT ( 'NONE',  ( 3.189131052002434963, -14.84934909478852205, 3.295817422932660890 ) ) ;
#10843=CARTESIAN_POINT ( 'NONE',  ( -5.080524353911874513, 119.7208665877771665, 0.8394179162009565154 ) ) ;
#10844=CARTESIAN_POINT ( 'NONE',  ( -0.02964290590182637811, -9.142985105544495283, 0.9735349185509928338 ) ) ;
#10845=CARTESIAN_POINT ( 'NONE',  ( -5.618954885709059432, 159.1014311945586712, -0.6070295849213356298 ) ) ;
#10846=CARTESIAN_POINT ( 'NONE',  ( -0.8651787172165069650, -5.103258934911358402, 0.4504873164067982327 ) ) ;
#10849=CARTESIAN_POINT ( 'NONE',  ( 3.418449710216091564, 108.6681208952157078, 4.126741282752677265 ) ) ;
#10850=CARTESIAN_POINT ( 'NONE',  ( -5.897637645108146032, 121.3687970875902806, 0.2476274089428441572 ) ) ;
#10851=CARTESIAN_POINT ( 'NONE',  ( 3.029556690758328674, -14.73736909467317169, 5.484434072839230012 ) ) ;
#10852=CARTESIAN_POINT ( 'NONE',  ( 13.22964523056185193, 152.2904283036577908, -1.375236710735037837 ) ) ;
#10853=ORIENTED_EDGE ( 'NONE', *, *, #21990, .F. ) ;
#10854=CARTESIAN_POINT ( 'NONE',  ( -6.656653968794013387, 119.6463993818898359, -1.283952750486249572 ) ) ;
#10855=CARTESIAN_POINT ( 'NONE',  ( -4.808149584360944750, 104.6144662015457243, 0.4147572885131461939 ) ) ;
#10856=CARTESIAN_POINT ( 'NONE',  ( 2.932272473696061255, -14.72556872895393276, 4.151486945341092749 ) ) ;
#10858=CARTESIAN_POINT ( 'NONE',  ( 9.295404511957237048, 124.2653519604415067, 0.02360630055292711402 ) ) ;
#10860=ORIENTED_EDGE ( 'NONE', *, *, #26102, .F. ) ;
#10861=CARTESIAN_POINT ( 'NONE',  ( -3.443790112798272407, 108.1634672882648118, 4.064613902700619619 ) ) ;
#10862=DIRECTION ( 'NONE',  ( 0.9998004120163609398, 4.016384292689130894E-17, 0.01997839162482749689 ) ) ;
#10863=EDGE_CURVE ( 'NONE', #1745, #38547, #7989, .T. ) ;
#10864=AXIS2_PLACEMENT_3D ( 'NONE', #35313, #6141, #28494 ) ;
#10868=CARTESIAN_POINT ( 'NONE',  ( 22.65077213736919859, 150.6401102206664291, 0.2239908233986879216 ) ) ;
#10870=CARTESIAN_POINT ( 'NONE',  ( 1.944882249840667710, -15.28710494480188586, 6.001156021306252697 ) ) ;
#10872=CARTESIAN_POINT ( 'NONE',  ( 3.009276887026297143, 39.20946620154573026, -1.210121013456480599 ) ) ;
#10873=CARTESIAN_POINT ( 'NONE',  ( 20.67294874948561656, 147.9587796579421308, 2.444796510662507583 ) ) ;
#10875=CARTESIAN_POINT ( 'NONE',  ( -3.240848860066210868, 23.83156553091082230, 7.781828003744739597 ) ) ;
#10876=CARTESIAN_POINT ( 'NONE',  ( 8.690636420055867006, 118.2864455517542552, -0.6276685427593149402 ) ) ;
#10877=CARTESIAN_POINT ( 'NONE',  ( -5.572611807913307125, 123.3023672762779910, -0.1864456790743028447 ) ) ;
#10878=B_SPLINE_CURVE_WITH_KNOTS ( 'NONE', 3,
 ( #24972, #24536, #17727, #41390, #11553, #8796, #34361, #4983, #18571, #37971, #18147, #14744, #21754, #27953, #1991, #14953, #11349 ),
 .UNSPECIFIED., .F., .F.,
 ( 4, 1, 1, 1, 1, 1, 1, 1, 1, 1, 1, 1, 1, 1, 4 ),
 ( 0.000000000000000000, 0.08300113939718137268, 0.1732806554784933895, 0.2717672377176819087, 0.3752096606209606167, 0.4787223716043260135, 0.5772295444745598747, 0.6668133826162351285, 0.7470991451079272982, 0.7815930070524458317, 0.8169452614683294644, 0.8547689062991584708, 0.8968063284581728745, 0.9447228702782888288, 1.000000000000000000 ),
 .UNSPECIFIED. ) ;
#10881=CARTESIAN_POINT ( 'NONE',  ( -4.722986921911269675, 104.6144662015457811, 1.042082363010505164 ) ) ;
#10882=CARTESIAN_POINT ( 'NONE',  ( 3.345514242732226418, 6.565394131763864216, 3.211428121085859733 ) ) ;
#10884=CARTESIAN_POINT ( 'NONE',  ( 3.136003201302111076, -14.34114629734795088, 4.029177829137042366 ) ) ;
#10885=CARTESIAN_POINT ( 'NONE',  ( 2.458941639547435720, 111.1666841684333633, -3.140650435616773262 ) ) ;
#10886=CARTESIAN_POINT ( 'NONE',  ( -5.853624122459167189, 117.3024554866451865, 0.4121555180536240481 ) ) ;
#10887=VECTOR ( 'NONE', #8723, 1000.000000000000000 ) ;
#10888=CARTESIAN_POINT ( 'NONE',  ( -4.462110519195587877, 27.89918626506305444, 0.8161882792947469101 ) ) ;
#10892=CARTESIAN_POINT ( 'NONE',  ( 4.827739681024636909, -15.50696398224166117, 1.464145260785405522 ) ) ;
#10893=CARTESIAN_POINT ( 'NONE',  ( -10.04363327864691158, 120.6268241347409855, 1.191437567882422943 ) ) ;
#10894=CARTESIAN_POINT ( 'NONE',  ( 0.1724166890850278577, 29.87817833284422875, -0.9617850639438362270 ) ) ;
#10896=CARTESIAN_POINT ( 'NONE',  ( -3.932819197772146946, 27.98301002373793978, 0.4898618918306564263 ) ) ;
#10897=CARTESIAN_POINT ( 'NONE',  ( 0.03413713131413576019, 107.6766875080336376, 4.617405654744151988 ) ) ;
#10898=CARTESIAN_POINT ( 'NONE',  ( -0.5800011805208045157, 120.2131932824006526, 0.3882866552237520530 ) ) ;
#10899=CARTESIAN_POINT ( 'NONE',  ( -4.934731464961845226, 117.4065818953012155, -1.087731638897137643 ) ) ;
#10900=CARTESIAN_POINT ( 'NONE',  ( 15.78846850359692411, 131.3838724160208926, -1.599517327752104201 ) ) ;
#10901=CARTESIAN_POINT ( 'NONE',  ( -18.19503446209947128, 151.8090458617612057, -2.356823057848427716 ) ) ;
#10904=CARTESIAN_POINT ( 'NONE',  ( 4.297048582020653207, 118.2143428055317855, -0.3468108124363870060 ) ) ;
#10905=CARTESIAN_POINT ( 'NONE',  ( 1.566048506583572308, 120.7946061759640486, -0.1772761409975699420 ) ) ;
#10906=ORIENTED_EDGE ( 'NONE', *, *, #36900, .T. ) ;
#10907=CARTESIAN_POINT ( 'NONE',  ( 2.245555723253176872, -15.32365336378345511, 5.046800657416122604 ) ) ;
#10912=CARTESIAN_POINT ( 'NONE',  ( -4.168830513765062307, 9.198770455692846681, 1.997586429550192166 ) ) ;
#10913=CARTESIAN_POINT ( 'NONE',  ( 10.28893712963043328, 123.4707319107414492, 1.320145760562476900 ) ) ;
#10914=CARTESIAN_POINT ( 'NONE',  ( -2.184147097501310419, 31.48929697360260249, 1.237019084378400580 ) ) ;
#10915=CARTESIAN_POINT ( 'NONE',  ( -7.618479139564731106, 124.7215218652630710, -0.1522353441811856445 ) ) ;
#10917=CARTESIAN_POINT ( 'NONE',  ( 1.893578447776079754, 19.08455809737888487, -4.224370802633358402 ) ) ;
#10918=CARTESIAN_POINT ( 'NONE',  ( 7.787205264484002853, 154.6472212274131550, 0.1983306932048341242 ) ) ;
#10921=CARTESIAN_POINT ( 'NONE',  ( 5.561512006252619322, 116.7374906030325263, -0.1055575561059139272 ) ) ;
#10924=CARTESIAN_POINT ( 'NONE',  ( 1.975136073220359556, -15.70315947173593685, 5.621751108460161461 ) ) ;
#10927=CARTESIAN_POINT ( 'NONE',  ( -3.339872139798120809, 10.66371166075841437, -7.743087711851694088 ) ) ;
#10932=CARTESIAN_POINT ( 'NONE',  ( -23.22010346901286937, 149.3105122542552863, -0.009921264925044727401 ) ) ;
#10933=VERTEX_POINT ( 'NONE', #12285 ) ;
#10939=CARTESIAN_POINT ( 'NONE',  ( -5.659482139215807714E-14, 120.9974662015457341, 3.101038099172001777E-16 ) ) ;
#10940=CARTESIAN_POINT ( 'NONE',  ( 4.375071722208805802, -15.20633266255931559, 4.762636924185132514 ) ) ;
#10941=CARTESIAN_POINT ( 'NONE',  ( -18.41670328667959566, 131.7683309214445728, 1.453117541724253670 ) ) ;
#10942=CARTESIAN_POINT ( 'NONE',  ( 13.43369120214907397, 119.6710471929552000, 0.6668731667128946494 ) ) ;
#10943=CARTESIAN_POINT ( 'NONE',  ( 9.086436585086531181, 153.9805727688486456, 0.3555968032218797537 ) ) ;
#10945=CARTESIAN_POINT ( 'NONE',  ( -22.79149376799281868, 150.3987591554885626, -0.7843734907460312433 ) ) ;
#10949=CARTESIAN_POINT ( 'NONE',  ( -8.758561883465446840, 117.9281413055073529, 0.3499703560493910848 ) ) ;
#10950=CARTESIAN_POINT ( 'NONE',  ( -6.615874392072807808, 120.4115791468657903, 0.8913422009562911308 ) ) ;
#10953=CARTESIAN_POINT ( 'NONE',  ( 7.655434399951916546, 119.7866739149480253, -1.082013720931114698 ) ) ;
#10954=CARTESIAN_POINT ( 'NONE',  ( 0.4928529169951482158, -8.289340824275994279, 0.8415213476199340237 ) ) ;
#10955=CARTESIAN_POINT ( 'NONE',  ( -0.3865025759031381902, 117.6538564835029206, -0.5089310662413599751 ) ) ;
#10957=CARTESIAN_POINT ( 'NONE',  ( 4.076263842838947049, 104.6144662015456817, 2.604289233408977111 ) ) ;
#10958=EDGE_CURVE ( 'NONE', #29270, #8806, #32064, .T. ) ;
#10959=CARTESIAN_POINT ( 'NONE',  ( 16.09504119906499753, 148.0691544347876345, -0.9470067175600010989 ) ) ;
#10960=CARTESIAN_POINT ( 'NONE',  ( 7.784012320830338005, 122.6313477005580665, 0.1555430910899518460 ) ) ;
#10961=ORIENTED_EDGE ( 'NONE', *, *, #24547, .T. ) ;
#10962=CARTESIAN_POINT ( 'NONE',  ( -9.373281424700515174, 121.4347015428822374, -1.498606428831740889 ) ) ;
#10963=CARTESIAN_POINT ( 'NONE',  ( 2.830806653267172734, -15.77471167405206032, 5.191726263073638492 ) ) ;
#10965=CARTESIAN_POINT ( 'NONE',  ( -4.407290876230779197, 118.1655354096973554, -0.6431967494569043042 ) ) ;
#10966=CIRCLE ( 'NONE', #12337, 0.5080000000000002292 ) ;
#10969=CARTESIAN_POINT ( 'NONE',  ( 4.065926199369043204, 118.2429491485453354, 0.3080910687088499467 ) ) ;
#10970=B_SPLINE_SURFACE_WITH_KNOTS ( 'NONE', 3, 3, ( 
 ( #15978, #28975, #41995, #32391, #3223, #16184, #29188, #38168, #34, #25992, #39001, #35809, #2396, #15355, #41368, #8981, #33036, #3864, #29623, #30243, #7261, #669, #23630, #20431, #3649, #39210, #7051, #40064, #32820, #6831, #1084, #10018, #16400, #39421, #33459 ),
 ( #20221, #19802, #20018, #26629, #27056, #10226, #23845, #7681, #7472, #14052, #29405, #10856, #10649, #33248, #22990, #36866, #30035, #4286, #16829, #16616, #36443, #36650, #23196, #459, #29831, #17250, #39636, #13432, #13637, #13847, #36230, #32602, #26418, #4077, #245 ),
 ( #875, #10442, #26846, #23413, #17036, #3435, #39853, #13223, #26206, #36016, #11277, #33670, #24466, #8087, #40278, #14670, #8510, #21060, #14879, #14462, #1507, #4494, #30870, #27881, #40483, #27474, #21469, #17454, #5125, #14253, #11071, #24261, #37268, #20850, #40890 ),
 ( #18076, #34295, #37470, #31079, #34499, #8297, #20640, #34086, #1714, #1297, #11477, #40685, #30453, #7888, #27674, #37688, #27262, #24055, #37070, #33877, #4915, #17869, #11694, #4706, #17659, #21266, #30660, #1918, #24680, #38375, #2604, #34973, #9189, #5796, #37734 ),
 ( #11744, #24731, #22145, #28567, #8558, #21731, #35176, #35378, #6003, #22353, #41148, #18965, #31972, #9390, #18123, #31761, #41364, #27929, #18752, #24945, #41575, #15351, #12384, #15137, #8771, #41785, #34551, #38163, #8977, #34753, #18543, #1965, #25371, #28356, #21518 ),
 ( #31128, #5376, #2178, #37946, #28140, #31546, #15770, #15563, #2809, #28775, #12585, #18331, #14929, #40936, #25574, #38578, #31334, #11954, #5587, #2392, #12167, #25163, #21944, #32597, #9806, #12787, #19587, #26624, #28971, #13218, #32184, #7047, #25777, #6827, #30 ),
 ( #3860, #25988, #6207, #10222, #10437, #10013, #3017, #15974, #29826, #16395, #6411, #19383, #6619, #9595, #16180, #454, #19178, #22565, #32387, #38997, #29183, #3430, #16824, #3646, #32816, #19796, #36013, #38785, #23408, #41990, #23191, #20013, #35594, #665, #39632 ),
 ( #3218, #12994, #26414, #13426, #22774, #35805, #29401, #241, #26201, #39418, #13633, #39205, #22986, #16611, #29619, #36225, #33032, #14047, #36439, #40479, #40680, #40272, #33243, #20217, #17864, #4489, #36644, #7466, #36859, #7676, #30447, #11067, #1710, #23625, #11273 ),
 ( #34082, #24051, #17448, #27469, #24256, #20426, #871, #10851, #14665, #33453, #10644, #4909, #13843, #4072, #1078, #37264, #4281, #7257, #37066, #17245, #23838, #1292, #30864, #27051, #27669, #11472, #26841, #14457, #20846, #7884, #8083, #33871, #39849, #17032, #4701 ),
 ( #30238, #17655, #21056, #40058, #20635, #33665, #30030, #14249, #27257, #30656, #1501, #15084, #15511, #8505, #25103, #34290, #37683, #18698, #21463, #38106, #22097, #21887, #28717, #9138, #5746, #15714, #1913, #5324, #31073, #31278, #34916, #35125, #31492, #34493, #5529 ),
 ( #41728, #8922, #18486, #5119, #12113, #2122, #31709, #21676, #2550, #18277, #28085, #5951, #40886, #2337, #15296, #41096, #24892, #8290, #28513, #34700, #14875, #41520, #24461, #28302, #18911, #11903, #37889, #37466, #41308, #38319, #8714, #12326, #21260, #18072, #25314 ),
 ( #31922, #2758, #27877, #11688, #24674, #29348, #2958, #41938, #32763, #6775, #12736, #25726, #22303, #35540, #9339, #3596, #36177, #6566, #9755, #38733, #3376, #22722, #10171, #32334, #12533, #16559, #16772, #16343, #35327, #38523, #6996, #35750, #9540, #22511, #12943 ),
 ( #6359, #23139, #404, #25934, #38943, #19329, #19965, #189, #19536, #29569, #13373, #3165, #19121, #29129, #32983, #16126, #28920, #3808, #32127, #6154, #42149, #26360, #32543, #25523, #13162, #26152, #39154, #9960, #29776, #22931, #15922, #35962, #19743, #39368, #27206 ),
 ( #23358, #21008, #40220, #27414, #36393, #7209, #33820, #11016, #20169, #4230, #4648, #17813, #17605, #10386, #23995, #11220, #16978, #33611, #40010, #7414, #33397, #1031, #4022, #33193, #17191, #29977, #10803, #817, #13995, #39801, #40426, #30607, #27000, #23785, #10593 ),
 ( #4857, #37015, #34031, #23573, #36806, #26573, #17400, #4442, #614, #13792, #7624, #1447, #24204, #37216, #8035, #14407, #26790, #36595, #30395, #13585, #39581, #20374, #7832, #30189, #14200, #20583, #1244, #20795, #1863, #11426, #9088, #15250, #15464, #24413, #37419 ),
 ( #34651, #34865, #8456, #14825, #18226, #28466, #37838, #27829, #11855, #12064, #21415, #21836, #40836, #31445, #40629, #11638, #25050, #24624, #2287, #41471, #28251, #35083, #12278, #38055, #22055, #8238, #37631, #21210, #34441, #41256, #34236, #5276, #8873, #30811, #5068 ),
 ( #31228, #2071, #25268, #5696, #18656, #31661, #18438, #18021, #5904, #1659, #2500, #38272, #14614, #27618, #31019, #15036, #28037, #41045, #24842, #8664, #21624, #5478, #32294, #39323, #41683, #25891, #2712, #19705, #25485, #19495, #12696, #38481, #39112, #3335, #35711 ),
 ( #10129, #16304, #3556, #12490, #9299, #9917, #29305, #22261, #22465, #22887, #36134, #35925, #23102, #41897, #6735, #32722, #18866, #31871, #32506, #42108, #28672, #6520, #25687, #149, #16083, #13116, #15878, #9500, #361, #35285, #38899, #9711, #35494, #19288, #15666 ),
 ( #6112, #28885, #26107, #19075, #32080, #2917, #38692, #6315, #3123, #16515, #29521, #13327, #26315, #29089, #12903, #22676, #6952, #23950, #20751, #32935, #1399, #27367, #3765, #40171, #19920, #33353, #4182, #10553, #13543, #20326, #40378, #29727, #13953, #16724, #7789 ),
 ( #7164, #39963, #17146, #4602, #26746, #569, #10963, #11173, #10755, #26533, #39537, #30560, #30148, #20123, #33148, #7368, #987, #26951, #23737, #14355, #36350, #36968, #27157, #30345, #33775, #24158, #17357, #10343, #3976, #36757, #23314, #7576, #20537, #16937, #29936 ),
 ( #774, #13751, #17559, #39756, #23521, #33567, #36549, #4400, #1194, #14154, #14776, #28415, #12227, #34601, #21575, #8611, #24789, #14567, #37167, #7988, #12010, #8826, #20958, #31611, #15410, #33980, #28201, #4809, #21363, #34390, #40787, #1610, #8403, #41420, #17760 ),
 ( #38004, #27573, #37786, #30973, #30760, #18386, #5647, #11378, #27987, #5224, #1813, #27776, #37576, #40581, #24365, #11587, #37371, #18178, #8189, #31180, #34189, #34812, #25003, #2021, #14985, #5015, #18605, #11800, #40995, #41208, #21786, #21158, #17974, #24570, #2450 ),
 ( #5430, #31394, #2239, #15198, #6681, #22832, #29245, #18811, #5855, #29034, #3497, #90, #2658, #35656, #9861, #38845, #6061, #35868, #22003, #38433, #31820, #16456, #9654, #19647, #15616, #28621, #16242, #6469, #41632, #28835, #13055, #301, #26046, #29462, #19021 ),
 ( #25218, #38221, #22622, #6264, #35035, #12850, #32028, #19444, #22413, #32449, #22205, #15827, #32662, #12440, #3076, #16035, #41848, #25632, #9038, #3281, #35440, #25433, #25836, #9249, #19235, #35236, #12645, #38642, #2866, #42055, #39056, #32245, #9447, #930, #4548 ),
 ( #39480, #33090, #23255, #26686, #10907, #10700, #39907, #26893, #13903, #32877, #30504, #13273, #30294, #27103, #39267, #7732, #33722, #10073, #4343, #26258, #39696, #10496, #16882, #19861, #23466, #17506, #36076, #20272, #23045, #14104, #3708, #23680, #7109, #6893, #36700 ),
 ( #16667, #17304, #29674, #17089, #516, #13489, #36914, #36493, #26476, #10284, #13696, #7312, #33301, #30091, #20699, #36289, #1138, #33509, #7521, #40115, #20068, #20483, #3920, #29883, #4129, #721, #23897, #34347, #34763, #37118, #24519, #31343, #41156, #24955, #11962 ),
 ( #31135, #17711, #30928, #37525, #37955, #21112, #5596, #18552, #20908, #21527, #27938, #18131, #34558, #1973, #33929, #8779, #40945, #2188, #14727, #1560, #5177, #5383, #34137, #14518, #1766, #28150, #8349, #27529, #21319, #24739, #4963, #18340, #40535, #14936, #11122 ),
 ( #11751, #40736, #37742, #11331, #17923, #21739, #30710, #8565, #15146, #27728, #11537, #27314, #1346, #14302, #4760, #24110, #40328, #24316, #7938, #37323, #8139, #28576, #29779, #19968, #31980, #3378, #41584, #617, #6777, #191, #23142, #32985, #2612, #38172, #6011 ) ),
 .UNSPECIFIED., .T., .F., .F.,
 ( 4, 2, 2, 2, 1, 2, 2, 2, 2, 2, 2, 1, 2, 2, 4 ),
 ( 4, 1, 1, 1, 1, 1, 1, 1, 1, 1, 1, 1, 1, 1, 1, 1, 1, 1, 1, 1, 1, 1, 1, 1, 1, 1, 1, 1, 1, 1, 1, 1, 4 ),
 ( 0.000000000000000000, 0.06249999999999900080, 0.1249999999999978906, 0.2499999999999956701, 0.2812499999999951150, 0.3749999999999934497, 0.4374999999999933387, 0.5000000000000000000, 0.5624999999999930056, 0.6249999999999928946, 0.7500000000000000000, 0.7812499999999951150, 0.8749999999999963363, 0.9374999999999982236, 1.000000000000000000 ),
 ( 0.000000000000000000, 0.02711375962671787321, 0.05385523109991235263, 0.08027126036152537614, 0.1064096946071439176, 0.1323192412471900226, 0.1580495177521483718, 0.1882118685537063907, 0.2182788543618764954, 0.2483346178351386324, 0.2784631806910429774, 0.3054937156393619513, 0.3327069032348308197, 0.3601597580799023035, 0.3879077415152338837, 0.4160045136367338525, 0.4445017332217630623, 0.4734489055539064517, 0.5028932750457014711, 0.5328797594123376724, 0.5634509204570880003, 0.5946469669818265080, 0.6265057848166851739, 0.6590629893014032792, 0.6923519956652609553, 0.7264041031822485728, 0.7612485893105871426, 0.7986318966073006065, 0.8369441774603861850, 0.8762126957585177900, 0.9164627945539034481, 0.9577180065289634392, 1.000000000000000000 ),
 .UNSPECIFIED. ) ;
#10971=CARTESIAN_POINT ( 'NONE',  ( 12.41677917861187375, 153.6617311634574037, 2.127417120026097397 ) ) ;
#10973=AXIS2_PLACEMENT_3D ( 'NONE', #37640, #24419, #25059 ) ;
#10974=CARTESIAN_POINT ( 'NONE',  ( 22.66375647020915807, 150.6386093215955100, 0.4528757910175261192 ) ) ;
#10975=CARTESIAN_POINT ( 'NONE',  ( 2.430217625452450569, 5.689826410578260329, 8.062849060857743666 ) ) ;
#10976=CARTESIAN_POINT ( 'NONE',  ( 7.609804580617480774, 122.3831840716419066, 0.4262428003126361165 ) ) ;
#10977=EDGE_CURVE ( 'NONE', #15736, #32767, #5265, .T. ) ;
#10978=CARTESIAN_POINT ( 'NONE',  ( 21.97872426622815922, 150.5960492154097778, -0.7309654607748478083 ) ) ;
#10979=CARTESIAN_POINT ( 'NONE',  ( 5.334825861721729012, 105.1224662015457483, 0.01195819060410700969 ) ) ;
#10981=CARTESIAN_POINT ( 'NONE',  ( -0.03523692298783126509, 115.6909491485452719, 1.763399716047879817 ) ) ;
#10983=CARTESIAN_POINT ( 'NONE',  ( -15.19006826215924555, 156.0999766016731769, -0.2361313609475708120 ) ) ;
#10987=CARTESIAN_POINT ( 'NONE',  ( -6.843608447964458996, 121.5419263055753731, -0.7453496101816521335 ) ) ;
#10990=CARTESIAN_POINT ( 'NONE',  ( 1.044095825906500297, 115.6909491485452719, -1.710621833244764245 ) ) ;
#10991=CARTESIAN_POINT ( 'NONE',  ( -15.83762317627089189, 145.9541952667573810, -0.7712195890315685087 ) ) ;
#10992=CARTESIAN_POINT ( 'NONE',  ( 2.370890509137566937, -15.02769382788871155, 5.804473790077508077 ) ) ;
#10994=CARTESIAN_POINT ( 'NONE',  ( -0.01887972822151516225, 159.3676309965788960, 0.9448188026860502298 ) ) ;
#10995=CARTESIAN_POINT ( 'NONE',  ( -7.783246152616193569, 154.6561476914895081, -0.1555277812256514736 ) ) ;
#10996=AXIS2_PLACEMENT_3D ( 'NONE', #21228, #31041, #8256 ) ;
#10997=CARTESIAN_POINT ( 'NONE',  ( 22.98214253804986384, 150.1595482613961110, 0.5361612621683795599 ) ) ;
#10999=CARTESIAN_POINT ( 'NONE',  ( -4.476207883417873568, -7.053342675672244155, -1.178223045331058705 ) ) ;
#11000=EDGE_CURVE ( 'NONE', #39424, #18094, #3809, .T. ) ;
#11001=CARTESIAN_POINT ( 'NONE',  ( -10.83330528665015891, 157.8980211815716928, -0.2164752214609687586 ) ) ;
#11006=CARTESIAN_POINT ( 'NONE',  ( 6.352347778906425546, 119.4701337457096031, 1.260299788626464190 ) ) ;
#11007=CARTESIAN_POINT ( 'NONE',  ( -2.734508853367146219, 0.3528594962865297391, 3.724956791467788353 ) ) ;
#11008=CARTESIAN_POINT ( 'NONE',  ( 17.34281104028693576, 125.1846915036903027, 1.498326104650645973 ) ) ;
#11010=CARTESIAN_POINT ( 'NONE',  ( 12.66950698665810648, 121.4495935343099688, -1.177842983441547808 ) ) ;
#11011=CARTESIAN_POINT ( 'NONE',  ( -3.029891238501105644, -9.367638731076009861, 3.490193963561483148 ) ) ;
#11012=CARTESIAN_POINT ( 'NONE',  ( -4.857111322523853580, 117.4312795728108227, -0.7492135168955066371 ) ) ;
#11015=CARTESIAN_POINT ( 'NONE',  ( -2.930943089244575805, 156.0861408873597327, 0.1605890987591811481 ) ) ;
#11016=CARTESIAN_POINT ( 'NONE',  ( 3.233725904218312408, -15.30436843596319463, 5.598328752637605099 ) ) ;
#11018=CARTESIAN_POINT ( 'NONE',  ( -0.1816203019703736821, 118.1651005609832907, -0.8950686016172918480 ) ) ;
#11020=CARTESIAN_POINT ( 'NONE',  ( 15.41952259888541121, 128.5596447653542498, 2.179146846741408350 ) ) ;
#11022=DIRECTION ( 'NONE',  ( -0.01997839162482761832, -1.040247600000950455E-18, 0.9998004120163610509 ) ) ;
#11024=CARTESIAN_POINT ( 'NONE',  ( -22.27457866854819812, 149.8733841865972920, 0.8555749715664362487 ) ) ;
#11025=CARTESIAN_POINT ( 'NONE',  ( 8.137580693842743074, 4.222088520697473868, -2.276242723817686997 ) ) ;
#11026=CARTESIAN_POINT ( 'NONE',  ( 16.08743688339769662, 147.0533492130506943, 1.289446542218032787 ) ) ;
#11028=EDGE_CURVE ( 'NONE', #16499, #18999, #39546, .T. ) ;
#11029=CARTESIAN_POINT ( 'NONE',  ( 13.24393851483415752, 156.9672759736256467, -0.3459722171078643549 ) ) ;
#11035=CARTESIAN_POINT ( 'NONE',  ( -4.364241878784717699, 118.1821976670573804, 0.4477677367896528149 ) ) ;
#11036=CARTESIAN_POINT ( 'NONE',  ( 3.182978606911899266, 107.7309519196391534, -4.270837756928458795 ) ) ;
#11037=EDGE_LOOP ( 'NONE', ( #35481, #22247, #19582, #32473 ) ) ;
#11039=CARTESIAN_POINT ( 'NONE',  ( 3.881581157509474078, 119.0007618588171852, -0.7751610500674797066 ) ) ;
#11040=CARTESIAN_POINT ( 'NONE',  ( -7.694663930960380149, 124.9344662015457317, -0.1537576976229973191 ) ) ;
#11041=CARTESIAN_POINT ( 'NONE',  ( 4.160719191527030958, 118.2392048939543798, 0.3834139420345348825 ) ) ;
#11042=CARTESIAN_POINT ( 'NONE',  ( -10.97991518849998549, 126.1652090859982707, -0.9941924553172258872 ) ) ;
#11044=CARTESIAN_POINT ( 'NONE',  ( 1.049180143938831522, 117.3993836601177065, -1.438948719551953248 ) ) ;
#11046=CARTESIAN_POINT ( 'NONE',  ( 4.060783872423706420, 109.8065891650451249, -3.521960838153598505 ) ) ;
#11047=CARTESIAN_POINT ( 'NONE',  ( -9.904299505090595090, 154.0333045108203009, -1.503511620041811714 ) ) ;
#11048=CARTESIAN_POINT ( 'NONE',  ( -5.302405987100971885, 104.6144662015457101, 1.270606870302479541 ) ) ;
#11051=CARTESIAN_POINT ( 'NONE',  ( -8.682609107657992098, 123.6667050411435582, -0.04289417010140435943 ) ) ;
#11054=CARTESIAN_POINT ( 'NONE',  ( 14.30760545269993500, 120.4308286971427862, 0.9551244717093423375 ) ) ;
#11056=CARTESIAN_POINT ( 'NONE',  ( 3.248418650160624033, -14.57852055173261618, 2.075358651653527620 ) ) ;
#11057=CARTESIAN_POINT ( 'NONE',  ( -0.5101717508068956963, 119.1670848682014281, 0.5756831679880034525 ) ) ;
#11058=CARTESIAN_POINT ( 'NONE',  ( 0.9729305924359374913, -6.768038221194544235, 0.04477287409810011554 ) ) ;
#11059=CARTESIAN_POINT ( 'NONE',  ( -15.39807837497279408, 121.0727120035890323, -0.9152850519163394649 ) ) ;
#11060=VECTOR ( 'NONE', #10571, 1000.000000000000000 ) ;
#11061=EDGE_CURVE ( 'NONE', #29150, #4283, #39964, .T. ) ;
#11062=CARTESIAN_POINT ( 'NONE',  ( 0.8997923272943838535, 13.09534505249760805, -0.3740510727227569499 ) ) ;
#11063=B_SPLINE_CURVE_WITH_KNOTS ( 'NONE', 3,
 ( #37877, #40873, #18058, #41083, #35113, #5106, #28706, #41296, #34480, #5940, #25301, #21663, #31061, #12521, #28498, #38304, #31479, #41508, #9125, #8493, #14862, #25089, #38094, #37453, #27865, #2324, #18899, #31909, #2745, #5312, #15284, #24880, #11674, #8909, #21247, #12313, #11891, #18263, #34687, #31696, #31266, #18686, #2538, #34277, #24661, #37670, #15072, #28072, #19527, #29766, #9329, #29338, #29558, #3153, #38723, #19732, #3587, #602, #16117, #39144, #180, #22712, #29120, #6552, #35317, #13149, #32324, #25924, #35529, #38933, #26142, #42139, #6984, #41926, #3366, #32753, #25512, #35740, #32117, #9531, #12934, #26349, #2947, #25716, #22500, #6350, #9743, #19320, #32534, #23129, #16333, #9948, #22921, #38512, #35952, #6765, #16548, #12727, #22292, #15911, #28911, #393, #13360, #39355, #10159, #36166, #19954, #6144, #32972, #3797, #16759, #19109, #33810, #8026, #10792, #17181, #36795, #23346, #1234, #20364, #13986, #10584, #26990, #11007, #17803, #40415, #37005, #23774, #30800, #20158, #39790, #23562, #23986, #24195, #14397, #33183, #13783, #36584, #7402, #33386, #4220, #11211, #30180, #40209, #1021, #13576, #40001, #37205, #7613, #20575, #27405, #39571, #20997, #34022, #33601, #4011, #4847, #26564, #4434, #17392, #16968, #36384, #30383, #4638, #10377, #7824, #14191, #27196, #26779, #20786, #17595, #30599, #1437, #7200, #29967, #807, #5468, #40618, #27609, #25257, #11843, #41461, #11417, #35073, #34640, #40826, #12268, #31651, #2060, #24403, #22044, #21826, #2491, #24830, #34855 ),
 .UNSPECIFIED., .F., .F.,
 ( 4, 1, 1, 1, 1, 1, 1, 1, 1, 1, 1, 1, 1, 1, 1, 1, 1, 1, 1, 1, 1, 1, 1, 1, 1, 1, 1, 1, 1, 1, 1, 1, 1, 1, 1, 1, 1, 1, 1, 1, 1, 1, 1, 1, 1, 1, 1, 1, 1, 1, 1, 1, 1, 1, 1, 1, 1, 1, 1, 1, 1, 1, 1, 1, 1, 1, 1, 1, 1, 1, 1, 1, 1, 1, 1, 1, 1, 1, 1, 1, 1, 1, 1, 1, 1, 1, 1, 1, 1, 1, 1, 1, 1, 1, 1, 1, 1, 1, 1, 1, 1, 1, 1, 1, 1, 1, 1, 1, 1, 1, 1, 1, 1, 1, 1, 1, 1, 1, 1, 1, 1, 1, 1, 1, 1, 1, 1, 1, 1, 1, 1, 1, 1, 1, 1, 1, 1, 1, 1, 1, 1, 1, 1, 1, 1, 1, 1, 1, 1, 1, 1, 1, 1, 1, 1, 1, 1, 1, 1, 1, 1, 1, 1, 1, 1, 1, 1, 1, 1, 1, 1, 1, 1, 1, 1, 1, 1, 1, 1, 1, 1, 1, 1, 1, 1, 1, 1, 1, 1, 1, 1, 1, 4 ),
 ( 0.000000000000000000, 0.007812500000000423273, 0.01388888888888889506, 0.01562500000000000000, 0.02343749999999998959, 0.02777777777777778317, 0.03125000000000092981, 0.03906249999999999306, 0.04166666666666667823, 0.04687500000000000000, 0.05468749999999999306, 0.05555555555555556635, 0.06249999999999997918, 0.06944444444444446141, 0.07031250000000000000, 0.07812500000000000000, 0.08333333333333334259, 0.08593749999999998612, 0.09374999999999603095, 0.09722222222222223764, 0.1015625000000000139, 0.1093750000000000000, 0.1111111111111111188, 0.1171875000000000000, 0.1250000000000000000, 0.1328125000000000000, 0.1388888888888889228, 0.1406250000000000000, 0.1484375000000000000, 0.1527777777777778179, 0.1562500000000039690, 0.1640625000000000000, 0.1666666666666666852, 0.1718750000000000000, 0.1796875000000000000, 0.1805555555555555802, 0.1875000000000000000, 0.1944444444444444753, 0.1953125000000000000, 0.2031250000000000000, 0.2083333333333333703, 0.2109375000000000000, 0.2187499999999960310, 0.2222222222222222376, 0.2265625000000000000, 0.2343750000000000000, 0.2361111111111111327, 0.2421875000000000000, 0.2500000000000000000, 0.2578125000000000000, 0.2638888888888888951, 0.2656250000000000000, 0.2734375000000000000, 0.2777777777777777346, 0.2812500000000039968, 0.2890625000000000000, 0.2916666666666665741, 0.2968750000000000000, 0.3046875000000000000, 0.3055555555555554692, 0.3125000000000000000, 0.3194444444444443088, 0.3203125000000000000, 0.3281250000000000000, 0.3333333333333332038, 0.3359375000000000000, 0.3437499999999960587, 0.3472222222222220434, 0.3515625000000000000, 0.3593750000000000000, 0.3611111111111109384, 0.3671875000000000000, 0.3750000000000000000, 0.3828125000000000000, 0.3888888888888886175, 0.3906250000000000000, 0.3984375000000000000, 0.4027777777777775126, 0.4062500000000039968, 0.4140625000000000000, 0.4166666666666663521, 0.4218750000000000000, 0.4296875000000000000, 0.4305555555555552472, 0.4375000000000000000, 0.4444444444444440867, 0.4453125000000000000, 0.4531250000000000000, 0.4583333333333329818, 0.4609375000000000000, 0.4687499999999960587, 0.4722222222222218768, 0.4765625000000000000, 0.4843750000000000000, 0.4861111111111107719, 0.4921875000000000000, 0.5000000000000000000, 0.5078125000000000000, 0.5138888888888886175, 0.5156250000000000000, 0.5234375000000000000, 0.5277777777777775681, 0.5312500000000039968, 0.5390625000000000000, 0.5416666666666664076, 0.5468750000000000000, 0.5546875000000000000, 0.5555555555555553582, 0.5625000000000000000, 0.5694444444444443088, 0.5703125000000000000, 0.5781250000000000000, 0.5833333333333331483, 0.5859375000000000000, 0.5937499999999960032, 0.5972222222222220989, 0.6015625000000000000, 0.6093750000000000000, 0.6111111111111110494, 0.6171875000000000000, 0.6250000000000000000, 0.6328125000000000000, 0.6388888888888888395, 0.6406250000000000000, 0.6484375000000000000, 0.6527777777777777901, 0.6562500000000039968, 0.6640625000000000000, 0.6666666666666666297, 0.6718750000000000000, 0.6796875000000000000, 0.6805555555555555802, 0.6875000000000000000, 0.6944444444444445308, 0.6953125000000000000, 0.7031250000000000000, 0.7083333333333333703, 0.7109375000000000000, 0.7187499999999960032, 0.7222222222222223209, 0.7265625000000000000, 0.7343750000000000000, 0.7361111111111111605, 0.7421875000000000000, 0.7500000000000000000, 0.7578125000000000000, 0.7638888888888889506, 0.7656250000000000000, 0.7734375000000000000, 0.7777777777777779011, 0.7812500000000039968, 0.7890625000000000000, 0.7916666666666668517, 0.7968750000000000000, 0.8046875000000000000, 0.8055555555555556912, 0.8125000000000000000, 0.8194444444444446418, 0.8203125000000000000, 0.8281250000000000000, 0.8333333333333335924, 0.8359375000000000000, 0.8437499999999960032, 0.8472222222222224319, 0.8515625000000000000, 0.8593750000000000000, 0.8611111111111113825, 0.8671875000000000000, 0.8750000000000000000, 0.8828125000000000000, 0.8888888888888891726, 0.8906250000000000000, 0.8984375000000000000, 0.9027777777777781232, 0.9062500000000039968, 0.9140625000000000000, 0.9166666666666670737, 0.9218750000000000000, 0.9296875000000000000, 0.9305555555555559133, 0.9375000000000000000, 0.9444444444444447528, 0.9453125000000000000, 0.9531250000000000000, 0.9583333333333335924, 0.9609375000000000000, 0.9687499999999991118, 0.9722222222222224319, 0.9765625000000000000, 0.9843750000000000000, 0.9861111111111111605, 0.9921874999999995559, 1.000000000000000000 ),
 .UNSPECIFIED. ) ;
#11066=CARTESIAN_POINT ( 'NONE',  ( -9.279111390949827509, 123.6186430441458981, 0.4039598099628549654 ) ) ;
#11067=CARTESIAN_POINT ( 'NONE',  ( 4.668376822648329316, -11.99306229768662391, 1.198378876927704839 ) ) ;
#11068=CARTESIAN_POINT ( 'NONE',  ( 0.8674473734592740293, 156.8926940187749324, -1.309446568524254451 ) ) ;
#11070=CARTESIAN_POINT ( 'NONE',  ( -4.138103288469840102, 104.6144662015457669, 2.504989205037290834 ) ) ;
#11071=CARTESIAN_POINT ( 'NONE',  ( 2.976679874252225577, -13.20894259333504905, 0.9412263588231246647 ) ) ;
#11072=CARTESIAN_POINT ( 'NONE',  ( -4.884145585883596041, 117.6381453523385687, -1.023340015079030163 ) ) ;
#11073=CARTESIAN_POINT ( 'NONE',  ( 15.64855408859525099, 147.2205073051419504, 0.1844942485914530250 ) ) ;
#11076=CARTESIAN_POINT ( 'NONE',  ( 12.86454329319598067, 121.9120276846612256, 1.753115191834736963 ) ) ;
#11078=CARTESIAN_POINT ( 'NONE',  ( 0.3704050251096834834, 117.3993836136686326, 1.500861956288976007 ) ) ;
#11079=CARTESIAN_POINT ( 'NONE',  ( 0.006534887713546001439, 159.5822087645323393, -0.3270325034788579277 ) ) ;
#11080=CARTESIAN_POINT ( 'NONE',  ( 1.843513859164539248, 116.5452236745340429, -0.1029321673164912687 ) ) ;
#11083=CARTESIAN_POINT ( 'NONE',  ( 2.002795586526139093, -15.67918376216764820, 5.544594217737087938 ) ) ;
#11085=CARTESIAN_POINT ( 'NONE',  ( -3.406197898068538787, 31.16742545776281403, -0.5635140647784588896 ) ) ;
#11086=CARTESIAN_POINT ( 'NONE',  ( 15.63125989577329733, 125.4375369430449609, 1.961567602338091243 ) ) ;
#11088=CARTESIAN_POINT ( 'NONE',  ( -8.431077252155047219, 22.10977948022283357, 0.3997009428958171462 ) ) ;
#11089=CARTESIAN_POINT ( 'NONE',  ( 5.572310759512880907, 117.9647318291645348, -0.8674352534993811092 ) ) ;
#11090=CARTESIAN_POINT ( 'NONE',  ( -3.552294876605587515, 120.2162445758188056, -0.4839898749706282310 ) ) ;
#11092=CARTESIAN_POINT ( 'NONE',  ( -0.02537255736359465483, 39.20946620154573736, 1.269746523260778082 ) ) ;
#11093=CARTESIAN_POINT ( 'NONE',  ( -4.138103289099216653, 104.6144662015456959, 2.504989205464778212 ) ) ;
#11095=CARTESIAN_POINT ( 'NONE',  ( 3.700881553190929374, 8.714383148187751615, -2.768892949411812854 ) ) ;
#11097=CARTESIAN_POINT ( 'NONE',  ( -4.831981401426255651, 118.5264896598256854, 0.7492988386145865709 ) ) ;
#11098=CARTESIAN_POINT ( 'NONE',  ( 3.154356104639033820, -12.65568165217861818, 0.8785170097314246584 ) ) ;
#11099=CARTESIAN_POINT ( 'NONE',  ( 4.469499996959894972, 123.9529229959338608, 0.04273414237147030864 ) ) ;
#11100=CARTESIAN_POINT ( 'NONE',  ( -2.690315046239569519, 30.48488075981191159, 3.827843980145978264 ) ) ;
#11103=CARTESIAN_POINT ( 'NONE',  ( -2.611728715877724039, 105.1243698582466095, -4.651900295541603114 ) ) ;
#11104=CARTESIAN_POINT ( 'NONE',  ( 5.059117473032719303, -15.50674158137822722, 2.046454293345789655 ) ) ;
#11105=CARTESIAN_POINT ( 'NONE',  ( -8.792330854012698538, 120.0394951565550343, 1.134075770671235217 ) ) ;
#11107=CARTESIAN_POINT ( 'NONE',  ( 0.5714185265493636479, 16.70905722793067838, 0.7929698740637279863 ) ) ;
#11111=CARTESIAN_POINT ( 'NONE',  ( 2.562387952376848688, 120.6526784328644339, 0.4448203013800775540 ) ) ;
#11112=CARTESIAN_POINT ( 'NONE',  ( -10.37991283549673227, 123.8962982355681817, 0.8252603836154488448 ) ) ;
#11114=CARTESIAN_POINT ( 'NONE',  ( 11.64488154209785087, 123.4149316504530702, -1.218180013452823562 ) ) ;
#11116=CARTESIAN_POINT ( 'NONE',  ( -14.40940766795072037, 123.3930721568691382, -1.837956572252895882 ) ) ;
#11117=DIRECTION ( 'NONE',  ( -5.206863593109713661E-17, 1.000000000000000000, -1.077750396879097183E-30 ) ) ;
#11118=CARTESIAN_POINT ( 'NONE',  ( 4.414058189832408274, 118.1799051844840704, -0.3934113130358646848 ) ) ;
#11120=CARTESIAN_POINT ( 'NONE',  ( 2.986828117522162263, 156.0959049650892041, -0.3398701836618409633 ) ) ;
#11121=VERTEX_POINT ( 'NONE', #39327 ) ;
#11122=CARTESIAN_POINT ( 'NONE',  ( 2.669030664778226480, -13.79969672238709499, -0.04828590215123814561 ) ) ;
#11126=CARTESIAN_POINT ( 'NONE',  ( -4.360315236241580017, -1.596229544307166348, -1.535301415559372940 ) ) ;
#11127=CARTESIAN_POINT ( 'NONE',  ( 16.94372847238220103, 146.2370505443881257, 1.929411111270964874 ) ) ;
#11128=CARTESIAN_POINT ( 'NONE',  ( 1.737819774751971025, 35.35497751095494579, 1.681281876415605225 ) ) ;
#11129=CARTESIAN_POINT ( 'NONE',  ( -5.756868464772181504, 120.3160329940760818, 0.2053529492706008819 ) ) ;
#11130=CARTESIAN_POINT ( 'NONE',  ( -4.603678009535974169, 12.38766144714272066, -0.4343361176327051321 ) ) ;
#11131=CARTESIAN_POINT ( 'NONE',  ( 15.76687399610631246, 145.9134097338176730, 0.4436328104633036062 ) ) ;
#11134=CARTESIAN_POINT ( 'NONE',  ( -5.552814959551180429, 116.7375731949262700, -0.3279940554716652135 ) ) ;
#11138=CARTESIAN_POINT ( 'NONE',  ( -0.6542591033984136439, 106.0194232803750509, 5.259796465664852150 ) ) ;
#11140=CARTESIAN_POINT ( 'NONE',  ( 8.383109624418931816, 7.835852165998051788, -1.087619381312709077 ) ) ;
#11141=CARTESIAN_POINT ( 'NONE',  ( 5.332935392244917416, 115.7029491189645825, 0.1065647408284378928 ) ) ;
#11145=CARTESIAN_POINT ( 'NONE',  ( -23.26894437362541979, 149.0206351951634076, -0.01026395906018885695 ) ) ;
#11149=EDGE_LOOP ( 'NONE', ( #27571, #19948, #9883, #18592 ) ) ;
#11151=CARTESIAN_POINT ( 'NONE',  ( -8.981069108608934926, 123.9698733229553937, -0.1794631345465900474 ) ) ;
#11152=CARTESIAN_POINT ( 'NONE',  ( 6.307811598796486230, -13.53853427790793695, 1.133914056348525934 ) ) ;
#11153=CARTESIAN_POINT ( 'NONE',  ( -0.02874440110946554008, 158.8294072187990196, 1.438487372358303595 ) ) ;
#11155=CARTESIAN_POINT ( 'NONE',  ( 23.10841651933900209, 148.9583646262859133, 1.191549328111825901 ) ) ;
#11156=CARTESIAN_POINT ( 'NONE',  ( 9.476822779618517600, 118.5748184150550060, -0.6643292918320548024 ) ) ;
#11158=CARTESIAN_POINT ( 'NONE',  ( -23.30750959433838432, 148.8446908248229477, -0.7975424382754975339 ) ) ;
#11161=CARTESIAN_POINT ( 'NONE',  ( -8.796889684792216002, 117.7044376108156172, -0.02762689297412515566 ) ) ;
#11162=CARTESIAN_POINT ( 'NONE',  ( -13.68689207195655122, 152.4534842159446271, 1.543072478675916903 ) ) ;
#11164=CARTESIAN_POINT ( 'NONE',  ( 12.06323264149818364, 122.4500365997666336, -1.303827596403756672 ) ) ;
#11166=CARTESIAN_POINT ( 'NONE',  ( 0.9729305924359374913, -6.768038221194544235, 0.04477287409810011554 ) ) ;
#11167=CARTESIAN_POINT ( 'NONE',  ( 0.009931510163623535892, 117.7854482299006378, -0.4970133802592048844 ) ) ;
#11169=CARTESIAN_POINT ( 'NONE',  ( 16.24447748055625240, 147.7868695473139553, -0.9462090312511075574 ) ) ;
#11170=CARTESIAN_POINT ( 'NONE',  ( -15.38000172822634326, 147.8312228277220868, -0.3073290368998167210 ) ) ;
#11172=CARTESIAN_POINT ( 'NONE',  ( -17.73882382519380840, 148.9562551477873740, -2.372964443305867643 ) ) ;
#11173=CARTESIAN_POINT ( 'NONE',  ( 2.989574797431095554, -15.77888062423098070, 5.070590765341169259 ) ) ;
#11175=CARTESIAN_POINT ( 'NONE',  ( -4.286648012141172082, 118.2141956653288162, -0.5113893019683410923 ) ) ;
#11178=CARTESIAN_POINT ( 'NONE',  ( 15.79265013067990964, 150.9007765090757971, 2.261858994468948225 ) ) ;
#11179=CARTESIAN_POINT ( 'NONE',  ( -6.538677740023618411E-14, 75.27746620154573520, -7.356392042280733227E-18 ) ) ;
#11180=CARTESIAN_POINT ( 'NONE',  ( 23.42514220146282966, 142.8382549601284097, 0.4680900899253090941 ) ) ;
#11181=CARTESIAN_POINT ( 'NONE',  ( 8.429690783291841072, 7.639065531857588631, 0.01617727833786941974 ) ) ;
#11182=CARTESIAN_POINT ( 'NONE',  ( 15.80292465353828568, 145.7390459690742830, 0.7709107363076879160 ) ) ;
#11183=CARTESIAN_POINT ( 'NONE',  ( 21.34935411394454974, 151.2846570542378117, -0.7363345373129175364 ) ) ;
#11188=CARTESIAN_POINT ( 'NONE',  ( -13.43120660244762732, 156.9273374874128137, -0.2039374989780117498 ) ) ;
#11191=CARTESIAN_POINT ( 'NONE',  ( 7.938121089952706377, 121.9582077959725979, -0.6488383765127299085 ) ) ;
#11194=CARTESIAN_POINT ( 'NONE',  ( 1.008887259173379736, 118.7629491485454025, -1.225340056906602415 ) ) ;
#11195=CARTESIAN_POINT ( 'NONE',  ( -9.051149985089010030, 123.9289873439938674, -0.3396360471471666087 ) ) ;
#11196=CARTESIAN_POINT ( 'NONE',  ( 2.037655544652288597, -15.20941935993469585, 5.943311982828837436 ) ) ;
#11197=CARTESIAN_POINT ( 'NONE',  ( -21.77700140173218202, 149.0176745010074342, 1.274060564799276873 ) ) ;
#11198=CARTESIAN_POINT ( 'NONE',  ( -13.59117098936157575, 150.2425924485623057, -0.2715839415567423143 ) ) ;
#11199=CARTESIAN_POINT ( 'NONE',  ( 21.89464077100137018, 151.4392833230981239, 0.5893027811483441125 ) ) ;
#11200=CARTESIAN_POINT ( 'NONE',  ( 7.043631758970988699, 122.0730096003205745, 0.1795708586965836517 ) ) ;
#11203=CARTESIAN_POINT ( 'NONE',  ( 0.9442757308971110319, 28.15415565245834628, -0.2560175424543267297 ) ) ;
#11205=CARTESIAN_POINT ( 'NONE',  ( -13.43845804798116106, 156.9141898299356512, -0.2685323735513600041 ) ) ;
#11207=ORIENTED_EDGE ( 'NONE', *, *, #31822, .T. ) ;
#11208=DIRECTION ( 'NONE',  ( 4.017660918040594346E-17, -1.000000000000000000, -2.376309959284834438E-19 ) ) ;
#11210=CARTESIAN_POINT ( 'NONE',  ( 5.083929588455360360, 119.2653419761957423, 1.105484519010427880 ) ) ;
#11211=CARTESIAN_POINT ( 'NONE',  ( 0.2036312542886812293, -3.545347522689146214, -4.628372119175537591 ) ) ;
#11212=CARTESIAN_POINT ( 'NONE',  ( 20.70408045738742686, 151.0745573368290593, 1.983427051661964535 ) ) ;
#11214=CARTESIAN_POINT ( 'NONE',  ( 13.28772774122543332, 155.5383117973235585, -1.582857276444406436 ) ) ;
#11215=CARTESIAN_POINT ( 'NONE',  ( -2.168033660621066172, 0.5777166996233511487, 4.103230905123370853 ) ) ;
#11216=CARTESIAN_POINT ( 'NONE',  ( 0.01645572339161321951, 159.4324016994384010, -0.8235116888278192215 ) ) ;
#11217=CARTESIAN_POINT ( 'NONE',  ( 4.840817968818798889, 117.7364599323587697, -0.8494325157683647598 ) ) ;
#11219=CARTESIAN_POINT ( 'NONE',  ( -15.25729751669411627, 143.4548391324710224, -0.07249109134377340613 ) ) ;
#11220=CARTESIAN_POINT ( 'NONE',  ( 4.692294315076144251, -14.85586321182354119, 4.526698459197877611 ) ) ;
#11224=CARTESIAN_POINT ( 'NONE',  ( 19.20800265940873786, 147.1635184732690220, 2.509201515169785957 ) ) ;
#11227=CARTESIAN_POINT ( 'NONE',  ( -10.29385411648731186, 157.8242135995235458, 0.8711791838966671531 ) ) ;
#11228=CARTESIAN_POINT ( 'NONE',  ( -7.544985805786585509, 7.895591250050960852, -3.771097921825450783 ) ) ;
#11230=CARTESIAN_POINT ( 'NONE',  ( 6.352854517228291975, 155.4084287100276072, 1.029490774253102758 ) ) ;
#11233=CARTESIAN_POINT ( 'NONE',  ( 15.03447867299173879, 120.7699597703182945, -0.2997422626971646409 ) ) ;
#11236=DIRECTION ( 'NONE',  ( -4.017660918040594346E-17, 1.000000000000000000, 2.376309959284834438E-19 ) ) ;
#11240=CARTESIAN_POINT ( 'NONE',  ( -4.122882846571666704, 118.2429491485453354, 0.1811355980067066163 ) ) ;
#11241=CARTESIAN_POINT ( 'NONE',  ( 2.178604253908287269, 106.5598271223812787, -4.865891711899141825 ) ) ;
#11242=ORIENTED_EDGE ( 'NONE', *, *, #28571, .T. ) ;
#11244=CARTESIAN_POINT ( 'NONE',  ( -8.245768994288328102, 120.2537849201367095, -1.446217431822895083 ) ) ;
#11245=CARTESIAN_POINT ( 'NONE',  ( -5.469471049222605075, 117.5088849381099436, -0.8278104034524697008 ) ) ;
#11246=CARTESIAN_POINT ( 'NONE',  ( 4.242344989534921673, 118.2250577600451180, 0.4716094826914004612 ) ) ;
#11247=CARTESIAN_POINT ( 'NONE',  ( -8.311356586562078874, 122.7091975629380585, -0.7066836605292579065 ) ) ;
#11248=CARTESIAN_POINT ( 'NONE',  ( -0.3866802643631708225, 115.7034476216335150, -1.763796639264662014 ) ) ;
#11252=CARTESIAN_POINT ( 'NONE',  ( 6.943414100881801332, 121.8132169909553966, -0.01755787080488244861 ) ) ;
#11253=CARTESIAN_POINT ( 'NONE',  ( -0.7424407951590874521, 156.5584078035761593, -0.9879031837870262400 ) ) ;
#11256=CARTESIAN_POINT ( 'NONE',  ( 7.794969618361607289, 122.5994144671777519, 0.004875389051802769477 ) ) ;
#11257=CARTESIAN_POINT ( 'NONE',  ( -15.72449225221075508, 145.6795444674731641, -0.1123860360721776058 ) ) ;
#11259=CARTESIAN_POINT ( 'NONE',  ( 2.866641708098013996, 116.8851979753409580, 0.4370437109847169488 ) ) ;
#11261=CARTESIAN_POINT ( 'NONE',  ( 2.930607426163104545, -14.92094031927118714, 4.083576684136651203 ) ) ;
#11262=CARTESIAN_POINT ( 'NONE',  ( 2.946692055775869346, 159.0164033662945258, -1.213088979206726092 ) ) ;
#11263=CARTESIAN_POINT ( 'NONE',  ( -6.644289941094903895, 120.1594786313440011, 0.9502652795725031742 ) ) ;
#11264=CARTESIAN_POINT ( 'NONE',  ( -0.9608913863540493594, -11.74124177384809542, -0.1559992898937096195 ) ) ;
#11265=CARTESIAN_POINT ( 'NONE',  ( -6.899218498549055667, 117.3903047926647787, -0.5887349169472961830 ) ) ;
#11266=CARTESIAN_POINT ( 'NONE',  ( 0.9476013557874021220, 22.48150014755712078, -0.2491751695904415032 ) ) ;
#11268=ADVANCED_FACE ( 'NONE', ( #4191 ), #13549, .F. ) ;
#11272=CARTESIAN_POINT ( 'NONE',  ( -9.625125523471179889, 124.0356975489027036, 0.4152212053287654969 ) ) ;
#11273=CARTESIAN_POINT ( 'NONE',  ( 4.637598599007382916, -11.68863464395987428, 0.6963472677309354708 ) ) ;
#11274=CARTESIAN_POINT ( 'NONE',  ( 6.553475369667514983, 120.9817801663137971, -0.6941111757064588605 ) ) ;
#11276=CARTESIAN_POINT ( 'NONE',  ( 0.7902916588979997936, 115.7028258067067696, 1.754551533761817161 ) ) ;
#11277=CARTESIAN_POINT ( 'NONE',  ( 2.870361413894247260, -14.70454541201141119, 4.341408117703424274 ) ) ;
#11278=CARTESIAN_POINT ( 'NONE',  ( -5.208405493689605592, 31.38331509014777154, -0.6716542322870747705 ) ) ;
#11279=CARTESIAN_POINT ( 'NONE',  ( 15.73072674608048338, 146.8994026175788008, 0.1860059585639197988 ) ) ;
#11281=CARTESIAN_POINT ( 'NONE',  ( 4.966515250750292765, 118.7197616721209670, 1.086191325688556919 ) ) ;
#11282=CARTESIAN_POINT ( 'NONE',  ( 2.987839817974693002, 108.3452893864955087, 4.269252900506888437 ) ) ;
#11283=CARTESIAN_POINT ( 'NONE',  ( -0.02983097946891718685, 117.3993836135855418, 1.492864285907047561 ) ) ;
#11284=EDGE_CURVE ( 'NONE', #8589, #27091, #33782, .T. ) ;
#11286=CARTESIAN_POINT ( 'NONE',  ( 5.797208421814580959, 116.9567987913546006, -0.006983082090869404714 ) ) ;
#11287=EDGE_CURVE ( 'NONE', #3752, #11376, #11685, .T. ) ;
#11290=CARTESIAN_POINT ( 'NONE',  ( 1.779277909118444301, -15.52187590737404221, 5.925248486025581407 ) ) ;
#11291=CARTESIAN_POINT ( 'NONE',  ( 4.756814333351318425, 117.4032681585794791, 1.206529664789174339 ) ) ;
#11293=CARTESIAN_POINT ( 'NONE',  ( -4.692483838673591201, 117.9823884840737094, 0.6748481237222451190 ) ) ;
#11295=EDGE_LOOP ( 'NONE', ( #8270, #35214, #13541, #28004, #5878 ) ) ;
#11296=CARTESIAN_POINT ( 'NONE',  ( -6.616342194955179501, 21.00577804425827111, -5.270772580892629122 ) ) ;
#11297=CARTESIAN_POINT ( 'NONE',  ( -5.678132272250597801, 118.5192932620585111, -1.203295300969776660 ) ) ;
#11298=CARTESIAN_POINT ( 'NONE',  ( -1.155851712377470530, 107.4826764677166864, -4.671650131992445054 ) ) ;
#11299=CARTESIAN_POINT ( 'NONE',  ( 4.886742582885162278, 117.6636387720722325, 0.9830068712545340093 ) ) ;
#11301=CARTESIAN_POINT ( 'NONE',  ( -0.004379098344380600097, 122.8649044353672934, 0.2191479880734042429 ) ) ;
#11302=CARTESIAN_POINT ( 'NONE',  ( 4.617411384770501392, 7.639850289152962048, 0.2838591255797697777 ) ) ;
#11304=CARTESIAN_POINT ( 'NONE',  ( -4.831905115772525683, 118.5264896598256854, 0.7498331390262092944 ) ) ;
#11305=CARTESIAN_POINT ( 'NONE',  ( 2.509002420848308823, -14.82469439542799527, 5.007744185041904217 ) ) ;
#11306=CARTESIAN_POINT ( 'NONE',  ( 4.831936455160824373, 120.7138498849978987, -0.2122769985084470012 ) ) ;
#11307=CARTESIAN_POINT ( 'NONE',  ( -2.010917461066705325, 115.7029473869310010, 1.638936349488617328 ) ) ;
#11308=ORIENTED_EDGE ( 'NONE', *, *, #5033, .F. ) ;
#11309=CARTESIAN_POINT ( 'NONE',  ( -4.505775810132860215, 104.6144662015457527, -1.759455372407346729 ) ) ;
#11310=CARTESIAN_POINT ( 'NONE',  ( 4.228161069935173266, -15.38163066151135361, 0.6048619776675213666 ) ) ;
#11311=CARTESIAN_POINT ( 'NONE',  ( -19.63947405400097779, 148.8045834396381508, 1.723899180582558310 ) ) ;
#11312=CARTESIAN_POINT ( 'NONE',  ( 0.7179688673824197176, 19.28876970375581479, -0.6613080194383522681 ) ) ;
#11314=ORIENTED_EDGE ( 'NONE', *, *, #28462, .F. ) ;
#11316=CARTESIAN_POINT ( 'NONE',  ( 1.574582893473400746, 118.9836165220538504, 0.7747311016372978587 ) ) ;
#11318=CARTESIAN_POINT ( 'NONE',  ( -10.11798836042646244, 123.5826510519420509, 0.8100524519737971607 ) ) ;
#11320=CARTESIAN_POINT ( 'NONE',  ( 4.601232872588083112, 118.0405793793079283, -0.6545214583194519653 ) ) ;
#11321=CARTESIAN_POINT ( 'NONE',  ( 11.08663849088095255, 154.4909003399924643, -1.626836423318808400 ) ) ;
#11322=CARTESIAN_POINT ( 'NONE',  ( -6.753855533487248763, 118.7881172115286148, -1.217991184693928641 ) ) ;
#11326=CARTESIAN_POINT ( 'NONE',  ( 4.172298354059645220, 118.2392279447537220, -0.2172812281923733324 ) ) ;
#11327=CARTESIAN_POINT ( 'NONE',  ( 9.542306315654297322, 124.2661852542617709, -0.2373755145837088965 ) ) ;
#11330=VERTEX_POINT ( 'NONE', #8832 ) ;
#11331=CARTESIAN_POINT ( 'NONE',  ( 2.102813808753936087, -15.18136450426021256, 5.202461169095355942 ) ) ;
#11334=CARTESIAN_POINT ( 'NONE',  ( -4.598078022480850180, -10.86695742004451404, -0.5832510952623800593 ) ) ;
#11335=CARTESIAN_POINT ( 'NONE',  ( 5.120605266512749942, 120.5246234221128248, 0.8194923670329071763 ) ) ;
#11336=CARTESIAN_POINT ( 'NONE',  ( -3.958300029084214522, 28.23836431654049761, 1.224951011016432556 ) ) ;
#11337=CARTESIAN_POINT ( 'NONE',  ( -5.007645675277699659, 117.8491495069952748, 0.5952962186315863269 ) ) ;
#11338=AXIS2_PLACEMENT_3D ( 'NONE', #17918, #31765, #28144 ) ;
#11340=CARTESIAN_POINT ( 'NONE',  ( 1.398650104629075797, 0.06838872207683838189, -4.420329592304430122 ) ) ;
#11341=CARTESIAN_POINT ( 'NONE',  ( 15.73024628025046567, 145.6958675726371553, 0.4429222902984593091 ) ) ;
#11345=CARTESIAN_POINT ( 'NONE',  ( 2.176363917357261979, 116.2587084501870009, -0.1247648271736234021 ) ) ;
#11348=CARTESIAN_POINT ( 'NONE',  ( -1.899626047278970109, 106.4942957007743587, 4.984479252724743681 ) ) ;
#11349=CARTESIAN_POINT ( 'NONE',  ( -6.442660433036017764, 29.32943145771791649, -0.01012415147099491285 ) ) ;
#11350=CARTESIAN_POINT ( 'NONE',  ( 2.469379016249674486, 9.589258615745848147, -8.089366445887874235 ) ) ;
#11355=CARTESIAN_POINT ( 'NONE',  ( -15.52406334459491255, 121.0440340969820596, 0.2084667659489263247 ) ) ;
#11359=VERTEX_POINT ( 'NONE', #14573 ) ;
#11361=CARTESIAN_POINT ( 'NONE',  ( -9.049782359939607446, 124.0675141969884692, -0.1808361888366265546 ) ) ;
#11362=CARTESIAN_POINT ( 'NONE',  ( 4.209311184370442049, -15.24947937046475310, 4.910682269069504891 ) ) ;
#11363=CARTESIAN_POINT ( 'NONE',  ( -20.28847770310441234, 149.9354415288716780, 1.565775960057087746 ) ) ;
#11364=CARTESIAN_POINT ( 'NONE',  ( 22.48855060683864693, 149.3130771379323392, -0.8549704587061032202 ) ) ;
#11365=CARTESIAN_POINT ( 'NONE',  ( 0.4746723515649934888, 24.68197512780947278, 4.609222710213416896 ) ) ;
#11366=CARTESIAN_POINT ( 'NONE',  ( -5.710605682675778283, 159.1232349745254453, -0.3332304182141800353 ) ) ;
#11368=ORIENTED_EDGE ( 'NONE', *, *, #16629, .T. ) ;
#11369=CARTESIAN_POINT ( 'NONE',  ( -8.798071503329609300, 117.6842349159552867, -0.1758064076808953657 ) ) ;
#11370=CARTESIAN_POINT ( 'NONE',  ( -14.72636943223162120, 131.2156652454908112, 1.433095336252470098 ) ) ;
#11372=CARTESIAN_POINT ( 'NONE',  ( 10.43940122747806676, 155.6679353847891321, -1.745147575944303364 ) ) ;
#11373=CARTESIAN_POINT ( 'NONE',  ( -18.99721151120906626, 152.1029585079319020, -2.158688780372492566 ) ) ;
#11375=CARTESIAN_POINT ( 'NONE',  ( 15.86865214134231650, 143.7482200480382346, -0.8098737496861395657 ) ) ;
#11376=VERTEX_POINT ( 'NONE', #18184 ) ;
#11377=CARTESIAN_POINT ( 'NONE',  ( -2.442377090744360935, 119.5064228623769225, -0.7372000016323176919 ) ) ;
#11378=CARTESIAN_POINT ( 'NONE',  ( 2.770358398913809861, -15.65020961539316602, 4.804192819214700982 ) ) ;
#11379=CARTESIAN_POINT ( 'NONE',  ( -4.522469723682791987, 118.1110480853273543, -0.6888394697316272408 ) ) ;
#11382=CARTESIAN_POINT ( 'NONE',  ( -4.916103084303564685, 117.4785598539236986, 0.9401160097163984153 ) ) ;
#11383=CARTESIAN_POINT ( 'NONE',  ( 8.285153246922861925, 121.0263440914440736, 1.363535410649704849 ) ) ;
#11386=CARTESIAN_POINT ( 'NONE',  ( 14.87733005835116096, 120.3210621052586475, 0.2473824415510234298 ) ) ;
#11388=CARTESIAN_POINT ( 'NONE',  ( 7.354229849910361771, -2.730604093522916109, 4.103208822889532925 ) ) ;
#11389=CARTESIAN_POINT ( 'NONE',  ( 15.44350913713179274, 147.8441550597069352, 0.7585189891071874024 ) ) ;
#11390=CARTESIAN_POINT ( 'NONE',  ( 4.263816225517785163, 117.9847045463029076, -0.8023379542233743944 ) ) ;
#11391=CARTESIAN_POINT ( 'NONE',  ( -6.451606698686837575E-14, 65.62546620154573418, 4.217636114931141265E-29 ) ) ;
#11392=CARTESIAN_POINT ( 'NONE',  ( -4.411262628599642355, 117.9394518360175539, 1.007827510414607719 ) ) ;
#11396=CARTESIAN_POINT ( 'NONE',  ( -23.40703704692324649, 142.8142681763856388, -0.3922439843285878136 ) ) ;
#11399=CARTESIAN_POINT ( 'NONE',  ( -5.885250668960954279, 121.3397778740266233, -0.3730483248005934671 ) ) ;
#11400=CARTESIAN_POINT ( 'NONE',  ( -8.044334902818970789, 121.4620208242423018, 0.8712540157608216207 ) ) ;
#11402=CARTESIAN_POINT ( 'NONE',  ( 4.855010706778257301, 115.6909491485452435, -1.281361498471799365 ) ) ;
#11403=CARTESIAN_POINT ( 'NONE',  ( -15.67344897587556396, 147.2319784351455780, -0.6427785636300452632 ) ) ;
#11404=CARTESIAN_POINT ( 'NONE',  ( 4.627184959846470491, -11.70336558297383611, 0.7419505617825855603 ) ) ;
#11405=CARTESIAN_POINT ( 'NONE',  ( -19.57327063168412451, 152.2820370773569323, 1.161482255138348130 ) ) ;
#11407=CARTESIAN_POINT ( 'NONE',  ( 20.68667083660084316, 152.5691845998198346, 0.5628278541506293031 ) ) ;
#11408=CARTESIAN_POINT ( 'NONE',  ( 15.72385166996613570, 146.8976323831864477, 0.3141999770531622160 ) ) ;
#11409=CARTESIAN_POINT ( 'NONE',  ( 1.824656174747253168, -15.25388738520313225, 5.420764384989097628 ) ) ;
#11410=CARTESIAN_POINT ( 'NONE',  ( 0.5513313392710353922, 29.23057874652566923, -0.8050760855368327418 ) ) ;
#11411=CARTESIAN_POINT ( 'NONE',  ( -3.300851927471685432, 159.4676453237595410, -0.08072286411353189750 ) ) ;
#11413=ORIENTED_EDGE ( 'NONE', *, *, #31584, .F. ) ;
#11414=DIRECTION ( 'NONE',  ( -0.9998004120163609398, 0.000000000000000000, -0.01997839162482749689 ) ) ;
#11416=CARTESIAN_POINT ( 'NONE',  ( -6.195589306716754230, 119.0760157020015129, 1.000162390493852138 ) ) ;
#11417=CARTESIAN_POINT ( 'NONE',  ( -0.7749869142727341398, -12.81603963768374044, -4.556214072895795830 ) ) ;
#11418=CARTESIAN_POINT ( 'NONE',  ( 22.03849170948978298, 148.8299554149626260, 2.028895537808247607 ) ) ;
#11420=CARTESIAN_POINT ( 'NONE',  ( 4.101170551582069557, 118.4217611105734846, -0.8082045602434785314 ) ) ;
#11421=CARTESIAN_POINT ( 'NONE',  ( 5.482275759465073506, 24.31437370403141784, -6.390863428313894978 ) ) ;
#11422=CARTESIAN_POINT ( 'NONE',  ( -0.3477286622124562965, 117.0882377308211773, -0.3718801884458513007 ) ) ;
#11423=CARTESIAN_POINT ( 'NONE',  ( 4.953217389033119034, 117.5439133103682110, -0.8526271701310890183 ) ) ;
#11424=VERTEX_POINT ( 'NONE', #17767 ) ;
#11425=CARTESIAN_POINT ( 'NONE',  ( -6.494470876743877241, 121.7611753534313550, -0.002333837952680380395 ) ) ;
#11426=CARTESIAN_POINT ( 'NONE',  ( 6.243909332557862513, -14.15813981987112946, 1.248599486541194681 ) ) ;
#11428=ORIENTED_EDGE ( 'NONE', *, *, #18395, .F. ) ;
#11429=CARTESIAN_POINT ( 'NONE',  ( -0.03245814172817904769, 157.7902383798253538, 1.624338139048501883 ) ) ;
#11432=CARTESIAN_POINT ( 'NONE',  ( -0.9959059386944214554, 109.5507526474568607, 3.831187545969641395 ) ) ;
#11433=CARTESIAN_POINT ( 'NONE',  ( -0.4581589521676752153, 10.92003791307801208, 8.418874016967684781 ) ) ;
#11434=CARTESIAN_POINT ( 'NONE',  ( 2.692664463852532108, 120.6505882111413683, 0.3986361418428905901 ) ) ;
#11435=CARTESIAN_POINT ( 'NONE',  ( -4.744878939582974020, 118.5930653697794384, -1.015278495842544482 ) ) ;
#11436=CARTESIAN_POINT ( 'NONE',  ( 22.64827982350381319, 150.3405807453409579, -0.2709709482530829328 ) ) ;
#11439=DIRECTION ( 'NONE',  ( -0.9998004120163608288, 0.000000000000000000, -0.01997839162482749342 ) ) ;
#11441=DIRECTION ( 'NONE',  ( 0.9998004120163609398, 0.000000000000000000, 0.01997839162482749689 ) ) ;
#11442=CARTESIAN_POINT ( 'NONE',  ( -4.161924923179597613, 118.2393572185476813, 0.2292740676127673349 ) ) ;
#11443=CARTESIAN_POINT ( 'NONE',  ( 2.100690617099141289, 106.6620211890832195, -4.900160429241310567 ) ) ;
#11446=CARTESIAN_POINT ( 'NONE',  ( 6.260578210526342779, 119.7762395299752427, -0.9857573057594839483 ) ) ;
#11448=CARTESIAN_POINT ( 'NONE',  ( 4.374182175873362333, 118.1842224889937256, 0.5915927881597164983 ) ) ;
#11449=CARTESIAN_POINT ( 'NONE',  ( -1.544162262334034308, 120.7289827521893670, -0.2751094044070050981 ) ) ;
#11452=CARTESIAN_POINT ( 'NONE',  ( 3.548611814566905664, 16.26088872207684943, 2.983771105379771971 ) ) ;
#11453=CARTESIAN_POINT ( 'NONE',  ( -11.45052794940122709, 153.2879862121713757, -1.711174725579351463 ) ) ;
#11457=CARTESIAN_POINT ( 'NONE',  ( 6.075908422621684402, 121.4480918675926517, 0.1456406178164729448 ) ) ;
#11458=CIRCLE ( 'NONE', #25748, 3.683000000000001162 ) ;
#11460=CARTESIAN_POINT ( 'NONE',  ( 22.59100494123591929, 149.3758529064199934, 1.630758705999802327 ) ) ;
#11462=CARTESIAN_POINT ( 'NONE',  ( 3.220686968960577712, -14.48737495597347902, 2.486805533510040078 ) ) ;
#11463=CARTESIAN_POINT ( 'NONE',  ( 17.75928342660597181, 128.5843929717815115, -1.279242276855531157 ) ) ;
#11464=CARTESIAN_POINT ( 'NONE',  ( -10.01831529487298234, 155.4362223408194836, 1.706801840347523358 ) ) ;
#11466=CARTESIAN_POINT ( 'NONE',  ( -4.556403025205056245, 17.84477460162305107, -0.8067276567318153457 ) ) ;
#11467=CARTESIAN_POINT ( 'NONE',  ( -1.362313394648154485, 159.5452856091935132, -0.5382632954014162641 ) ) ;
#11468=CARTESIAN_POINT ( 'NONE',  ( 0.9697834966998255535, 21.94565095173003400, 0.09096683575692042500 ) ) ;
#11471=CARTESIAN_POINT ( 'NONE',  ( -1.553919893302708743, 120.7289827521893670, 0.2132023499116274534 ) ) ;
#11472=CARTESIAN_POINT ( 'NONE',  ( 4.871446434089309108, -12.86987818651588711, 2.618604111146097591 ) ) ;
#11473=CARTESIAN_POINT ( 'NONE',  ( 17.12300761254194725, 147.7912591418244403, -1.363423146152763943 ) ) ;
#11475=CARTESIAN_POINT ( 'NONE',  ( 2.609136386454064649, 115.7032548281754458, 1.690807494954503998 ) ) ;
#11477=CARTESIAN_POINT ( 'NONE',  ( 2.917951099372082080, -14.56804730652265434, 4.441407531948645904 ) ) ;
#11478=CARTESIAN_POINT ( 'NONE',  ( -4.794479500060544019, 117.6747142900968015, -1.098999508304763006 ) ) ;
#11479=ADVANCED_FACE ( 'NONE', ( #34820, #14782 ), #5436, .F. ) ;
#11480=CARTESIAN_POINT ( 'NONE',  ( 1.572870384098442376, 156.2570369995211479, -0.04660437260867165976 ) ) ;
#11482=CARTESIAN_POINT ( 'NONE',  ( 17.92333008985171361, 151.7072807693909340, 2.394054079121862078 ) ) ;
#11483=DIRECTION ( 'NONE',  ( -0.9998004120163608288, 0.000000000000000000, -0.01997839162482747608 ) ) ;
#11486=ADVANCED_FACE ( 'NONE', ( #14362 ), #2242, .T. ) ;
#11488=CARTESIAN_POINT ( 'NONE',  ( 21.55438672983820680, 132.6250929350426020, 0.2276674992303582834 ) ) ;
#11491=CARTESIAN_POINT ( 'NONE',  ( 1.870953937135939604, -15.14421219162230514, 5.894613027636500746 ) ) ;
#11495=CARTESIAN_POINT ( 'NONE',  ( -4.639824337899648654, 117.9546834919162279, 0.7580944945253588196 ) ) ;
#11497=ORIENTED_EDGE ( 'NONE', *, *, #870, .F. ) ;
#11499=CARTESIAN_POINT ( 'NONE',  ( 8.597804290853659381, 118.7612935373479814, -0.8549226474316184987 ) ) ;
#11500=CARTESIAN_POINT ( 'NONE',  ( -2.044121638888310777, 114.8832439220486350, -1.972317757894941570 ) ) ;
#11501=CARTESIAN_POINT ( 'NONE',  ( 4.947893305883586557, 117.4718310785403332, 1.024415023481761056 ) ) ;
#11503=CARTESIAN_POINT ( 'NONE',  ( -0.3585272760099085243, 113.0327356262573915, 2.615547676125328014 ) ) ;
#11504=CARTESIAN_POINT ( 'NONE',  ( 3.315635589170360831, -10.27688868798473720, -3.234826238065521053 ) ) ;
#11507=CARTESIAN_POINT ( 'NONE',  ( 3.480220535011376182, -13.66934472092314046, 3.064489479733436106 ) ) ;
#11508=CARTESIAN_POINT ( 'NONE',  ( 6.874578817172041667, 121.8312213470058225, -0.01890686361713992888 ) ) ;
#11509=CARTESIAN_POINT ( 'NONE',  ( 0.9635274152722271834, 39.00291388108365709, 1.327368659714503574 ) ) ;
#11511=DIRECTION ( 'NONE',  ( 0.9998004120163608288, 0.000000000000000000, 0.01997839162482749342 ) ) ;
#11512=CARTESIAN_POINT ( 'NONE',  ( -4.556757383386185190, 31.49269130883712720, -0.6906699653381264126 ) ) ;
#11514=CARTESIAN_POINT ( 'NONE',  ( -3.608349438833787559, 105.1232419943577554, -3.942834359180669601 ) ) ;
#11515=CARTESIAN_POINT ( 'NONE',  ( 4.514867502249738429, -15.46117574218924773, 1.158286244139274279 ) ) ;
#11516=CARTESIAN_POINT ( 'NONE',  ( -3.262238196373905108, 118.8118204130220903, 0.7766580032327177197 ) ) ;
#11517=CARTESIAN_POINT ( 'NONE',  ( 0.9727671068909850005, -1.206248505109467795, 0.1081409728948927729 ) ) ;
#11518=CARTESIAN_POINT ( 'NONE',  ( -0.8572797930410298584, 14.11360927180527014, 0.4650159543037101773 ) ) ;
#11521=ORIENTED_EDGE ( 'NONE', *, *, #8464, .F. ) ;
#11523=CARTESIAN_POINT ( 'NONE',  ( 3.776803835208212501, 121.1194860566822626, 0.3725146398702260386 ) ) ;
#11525=CARTESIAN_POINT ( 'NONE',  ( -6.537359847799236512, 121.1369950346570192, 0.6189803324213468683 ) ) ;
#11526=DIRECTION ( 'NONE',  ( -4.017660918040594346E-17, 1.000000000000000000, 2.376309959284834438E-19 ) ) ;
#11527=ADVANCED_FACE ( 'NONE', ( #21164 ), #25327, .F. ) ;
#11528=CIRCLE ( 'NONE', #31933, 3.175000000000001155 ) ;
#11529=CARTESIAN_POINT ( 'NONE',  ( 4.554470953189297511, 118.0726681490097860, -0.6231005214564631078 ) ) ;
#11530=CARTESIAN_POINT ( 'NONE',  ( 11.27566272104525780, 154.5781333488962446, -1.670651684902623835 ) ) ;
#11531=CARTESIAN_POINT ( 'NONE',  ( -6.715107731706678962, 119.1290971219625021, -1.270026890958220633 ) ) ;
#11533=EDGE_CURVE ( 'NONE', #6038, #21991, #36925, .T. ) ;
#11534=CARTESIAN_POINT ( 'NONE',  ( 4.074910602682932925, 118.2429491485453354, -0.1454311599470142491 ) ) ;
#11535=CARTESIAN_POINT ( 'NONE',  ( 8.758948435532664334, 123.3024417045633498, -0.2233049321804337906 ) ) ;
#11537=CARTESIAN_POINT ( 'NONE',  ( 2.857130780617909149, -14.87311083204414786, 4.269097905712053276 ) ) ;
#11538=CARTESIAN_POINT ( 'NONE',  ( -4.980827880492125992, 117.4083494260662661, 0.8692259800077603016 ) ) ;
#11540=CARTESIAN_POINT ( 'NONE',  ( 4.406646451516359697, -6.344046434980911364, 1.391598188203984288 ) ) ;
#11541=CARTESIAN_POINT ( 'NONE',  ( 4.884089373684489033, 156.1188696671683260, 1.381267178739763457 ) ) ;
#11542=CARTESIAN_POINT ( 'NONE',  ( -3.114615542158560846, 28.50392562220115877, 0.5887488407975547400 ) ) ;
#11543=CARTESIAN_POINT ( 'NONE',  ( -1.441108623025377566, 106.3840144300045409, 5.062828720429449980 ) ) ;
#11544=CARTESIAN_POINT ( 'NONE',  ( 0.3994026957563919789, 5.465888722076803319, 4.619092260001838923 ) ) ;
#11545=CARTESIAN_POINT ( 'NONE',  ( 14.19780223135870045, 138.9094276006951247, 0.4095818057664821765 ) ) ;
#11547=CARTESIAN_POINT ( 'NONE',  ( 1.958624548881832350, -3.744965520567712147, -8.202033116754515518 ) ) ;
#11549=CARTESIAN_POINT ( 'NONE',  ( 8.779668897515529480, 117.8111319902365466, -0.2054863605742794086 ) ) ;
#11550=CARTESIAN_POINT ( 'NONE',  ( 0.0006472084742443534513, 124.6436471961814476, -0.03238895860161133955 ) ) ;
#11553=CARTESIAN_POINT ( 'NONE',  ( -0.7326219338007132764, 37.28220708697721619, 2.048504824603447627 ) ) ;
#11554=CARTESIAN_POINT ( 'NONE',  ( 8.274862188802355689, -1.658786094895864149, -1.630640499628306372 ) ) ;
#11555=CARTESIAN_POINT ( 'NONE',  ( 0.3815321866612710888, 118.1588879786102524, 0.9088679235907958232 ) ) ;
#11556=CARTESIAN_POINT ( 'NONE',  ( 3.174366308151882254, 63.33946620154573282, 0.06343139340882729404 ) ) ;
#11559=CARTESIAN_POINT ( 'NONE',  ( -9.710933996004797564, 118.1218853900603136, 0.2424195399123783012 ) ) ;
#11566=CARTESIAN_POINT ( 'NONE',  ( -8.935197197525255319, 123.9063447689825779, -0.1785465045940570761 ) ) ;
#11567=CARTESIAN_POINT ( 'NONE',  ( 4.578653272329702872, -15.42525073102989097, 4.254151796826286969 ) ) ;
#11568=CARTESIAN_POINT ( 'NONE',  ( -10.51304382037013951, 120.0128241960130424, 1.064055063733757356 ) ) ;
#11569=CARTESIAN_POINT ( 'NONE',  ( 14.77829941377241774, 121.3346631531286164, -0.7297537739211614749 ) ) ;
#11570=CARTESIAN_POINT ( 'NONE',  ( 0.6590154617207463206, 19.50938314818779062, -4.574821423538240950 ) ) ;
#11571=CARTESIAN_POINT ( 'NONE',  ( -22.75358200450901336, 150.3871190066015799, -0.9055542368224056560 ) ) ;
#11573=ORIENTED_EDGE ( 'NONE', *, *, #40256, .T. ) ;
#11574=CARTESIAN_POINT ( 'NONE',  ( -2.185546054340737232, 116.2009413105890019, -0.01666836221661271641 ) ) ;
#11576=CARTESIAN_POINT ( 'NONE',  ( -9.357607378341853632, 155.0893615026619159, 1.530462696531121658 ) ) ;
#11578=EDGE_CURVE ( 'NONE', #5098, #25709, #3584, .T. ) ;
#11579=CARTESIAN_POINT ( 'NONE',  ( 2.387896358646802941, 119.0637060312156024, -0.6953999086667945750 ) ) ;
#11580=CARTESIAN_POINT ( 'NONE',  ( -21.29237892510571584, 148.2102652567764380, -2.313897094871049553 ) ) ;
#11582=EDGE_CURVE ( 'NONE', #10724, #2340, #11806, .T. ) ;
#11583=B_SPLINE_CURVE_WITH_KNOTS ( 'NONE', 3,
 ( #1731, #37705, #15534, #4930, #31301, #8104, #38130, #14688 ),
 .UNSPECIFIED., .F., .F.,
 ( 4, 2, 2, 4 ),
 ( 0.000000000000000000, 0.2500000000000000000, 0.5000000000000000000, 1.000000000000000000 ),
 .UNSPECIFIED. ) ;
#11584=CARTESIAN_POINT ( 'NONE',  ( 6.388910139315798986, 155.4084287100276072, -0.7748799927007736787 ) ) ;
#11586=CARTESIAN_POINT ( 'NONE',  ( -11.77984014550172631, 123.3160021321619695, -1.727726820665321128 ) ) ;
#11587=CARTESIAN_POINT ( 'NONE',  ( 3.676215660907734328, -15.61639409997438221, 3.572853394304201569 ) ) ;
#11589=CARTESIAN_POINT ( 'NONE',  ( -4.491445922219573283, 118.1274274216726923, -0.6813552275993676188 ) ) ;
#11591=CARTESIAN_POINT ( 'NONE',  ( -4.924473681474931475, 117.4782309372925795, 0.9294218393982265347 ) ) ;
#11592=CARTESIAN_POINT ( 'NONE',  ( 17.91131452944944868, 148.1388135707062474, 2.335088068787735782 ) ) ;
#11595=CARTESIAN_POINT ( 'NONE',  ( -7.218840658378264052, 2.017470825009220370, -4.342437029863850384 ) ) ;
#11596=CARTESIAN_POINT ( 'NONE',  ( 1.615823435711507994, 156.2764358050213787, 0.4002269557471578865 ) ) ;
#11600=CARTESIAN_POINT ( 'NONE',  ( -2.011069428279017579, 117.9394519721141421, 1.285232015002204520 ) ) ;
#11605=CARTESIAN_POINT ( 'NONE',  ( -20.37188742667035157, 129.0035756037533758, -0.2165721192533106021 ) ) ;
#11608=CARTESIAN_POINT ( 'NONE',  ( 5.931653563816388974, 121.3754646592592792, -0.09967777454307100160 ) ) ;
#11609=CARTESIAN_POINT ( 'NONE',  ( -8.334503520420923905, 120.0709494557484049, 1.118110265123132718 ) ) ;
#11610=EDGE_LOOP ( 'NONE', ( #22348, #29589, #21399 ) ) ;
#11611=CARTESIAN_POINT ( 'NONE',  ( 0.2209820516631312570, 118.7629491485454025, -1.272057036781818251 ) ) ;
#11612=CARTESIAN_POINT ( 'NONE',  ( 0.003550340867665223877, 156.3099534201614631, -0.1776735749810080256 ) ) ;
#11613=CARTESIAN_POINT ( 'NONE',  ( 5.392686582494618186, -13.55334589181164695, 3.069518437182660264 ) ) ;
#11614=CARTESIAN_POINT ( 'NONE',  ( -14.51588022701143643, 121.7426775721902175, 0.9381456983900906543 ) ) ;
#11615=CARTESIAN_POINT ( 'NONE',  ( 2.026107803274938668, 117.3993837373488134, -1.369929326007458315 ) ) ;
#11616=CARTESIAN_POINT ( 'NONE',  ( 16.84361796505724485, 155.2300590059875844, 0.4756075834919733514 ) ) ;
#11617=CARTESIAN_POINT ( 'NONE',  ( 13.59117098933499790, 150.2425924485890505, 0.2715839415562140702 ) ) ;
#11618=CARTESIAN_POINT ( 'NONE',  ( -5.019158082560326584, 117.3993830232448659, 0.7013206397503667366 ) ) ;
#11619=CARTESIAN_POINT ( 'NONE',  ( -0.8868740923517060004, 23.60745955286466824, 0.4068859645678858938 ) ) ;
#11620=CARTESIAN_POINT ( 'NONE',  ( -13.64397932274300551, 119.6379125180634446, -0.3727430486357817818 ) ) ;
#11624=CARTESIAN_POINT ( 'NONE',  ( 6.152576065035590069, 119.0783712746871572, 1.247159342819149863 ) ) ;
#11626=CARTESIAN_POINT ( 'NONE',  ( 21.74891716461452518, 141.9756885651356413, 2.029123422127836029 ) ) ;
#11628=CARTESIAN_POINT ( 'NONE',  ( 20.05916364549907982, 149.8444905389382882, -1.617669260345511173 ) ) ;
#11629=CARTESIAN_POINT ( 'NONE',  ( 1.217031898716552707, 25.17763362506526192, -8.368877290174015826 ) ) ;
#11630=CARTESIAN_POINT ( 'NONE',  ( -8.073283135001606325, 117.9965348323767671, -0.8851005009521593081 ) ) ;
#11631=CARTESIAN_POINT ( 'NONE',  ( 4.936719870595172921, 117.6322946229582982, -0.7900978698212627327 ) ) ;
#11634=CARTESIAN_POINT ( 'NONE',  ( 5.571761382372238280, 117.9391977826196296, 0.7470240521525302047 ) ) ;
#11636=CARTESIAN_POINT ( 'NONE',  ( -13.04043193504470288, 133.9378623523624299, 0.05483593244790770094 ) ) ;
#11637=CARTESIAN_POINT ( 'NONE',  ( -18.75244783997693787, 140.8526363637247982, -2.516729932275435289 ) ) ;
#11638=CARTESIAN_POINT ( 'NONE',  ( 4.666472529085985421, -15.22678077218547799, 4.383143511210439769 ) ) ;
#11641=CARTESIAN_POINT ( 'NONE',  ( -3.354700091392308181, 117.9496054330418104, -1.286735144063386738 ) ) ;
#11642=B_SPLINE_CURVE_WITH_KNOTS ( 'NONE', 3,
 ( #10960, #20323, #20955, #36546, #7365, #17143, #984, #10752, #36754, #7573, #20534, #12172, #25781, #12999, #18756, #35382, #41791, #9193, #35181, #2815, #5801, #12589, #2608, #15567, #15774, #28779, #38584, #19183, #9812, #31766, #6416, #22569, #38789, #35599, #6624, #12792, #22778, #41580, #25578, #28361, #32188, #28572, #12388, #9393, #25375, #21948, #3022, #34979, #38380, #19387, #9600, #22150, #6007, #25168, #18969 ),
 .UNSPECIFIED., .F., .F.,
 ( 4, 2, 2, 2, 2, 1, 2, 2, 2, 2, 2, 1, 2, 2, 2, 2, 2, 1, 1, 2, 2, 2, 2, 2, 1, 2, 2, 2, 2, 4 ),
 ( 0.000000000000000000, 0.03125000000005594830, 0.06250000000011189660, 0.09375000000016779633, 0.1093750000001957601, 0.1171875000002130657, 0.1210937500002182976, 0.1250000000002235157, 0.1875000000003034240, 0.2187500000003434197, 0.2343750000003604617, 0.2421875000003690104, 0.2460937500003703704, 0.2500000000003717027, 0.3750000000004340972, 0.4375000000004619083, 0.4687500000004758416, 0.4843750000004827250, 0.4921875000004831135, 0.4960937500004862777, 0.5000000000004893863, 0.6250000000003956835, 0.6875000000003488321, 0.7187500000003254064, 0.7343750000003137490, 0.7421875000003078648, 0.7500000000003018696, 0.8750000000001509903, 0.9375000000000754952, 1.000000000000000000 ),
 .UNSPECIFIED. ) ;
#11644=CARTESIAN_POINT ( 'NONE',  ( 19.21961548592736690, 147.3692480224366079, 2.508364867928686071 ) ) ;
#11646=CARTESIAN_POINT ( 'NONE',  ( -5.295281529786937114, 115.6909491485389054, -0.7215990444303079787 ) ) ;
#11647=CARTESIAN_POINT ( 'NONE',  ( -2.327868625978157358, 124.9344662015457175, -0.04651635516647301821 ) ) ;
#11648=CARTESIAN_POINT ( 'NONE',  ( -0.9165671635830696662, -12.81903285835614525, -8.372742598224451882 ) ) ;
#11649=CARTESIAN_POINT ( 'NONE',  ( 16.28325953274104165, 146.1553843108282820, 1.442930602569015175 ) ) ;
#11650=CARTESIAN_POINT ( 'NONE',  ( -4.796232024291369633, 115.6909491485453003, -1.474888944111601319 ) ) ;
#11651=CARTESIAN_POINT ( 'NONE',  ( 22.30840772692673823, 150.5193240506149550, -0.5167903241875734244 ) ) ;
#11656=CARTESIAN_POINT ( 'NONE',  ( 1.975269416564897629, -15.10067923695700642, 5.832845082603782316 ) ) ;
#11657=CARTESIAN_POINT ( 'NONE',  ( -4.297166465714638228, 118.2143479842866611, 0.3467644725669444261 ) ) ;
#11658=CARTESIAN_POINT ( 'NONE',  ( 4.780914974771698134, 111.8766742162016357, -2.439331676452292097 ) ) ;
#11661=CARTESIAN_POINT ( 'NONE',  ( 6.194152875776375744, 119.6356763387034334, -1.001677016561595801 ) ) ;
#11663=CARTESIAN_POINT ( 'NONE',  ( 4.159337697990636684, 118.2392943130565470, 0.3847892076047124688 ) ) ;
#11664=CARTESIAN_POINT ( 'NONE',  ( -16.05307823990510485, 146.0544122543811341, -1.176040581308521960 ) ) ;
#11665=CARTESIAN_POINT ( 'NONE',  ( 4.886022116125724679, 117.7561648045584519, -0.7145573245312663024 ) ) ;
#11666=CARTESIAN_POINT ( 'NONE',  ( 0.3903998909774342718, 117.9496051583923872, -1.393992266905087485 ) ) ;
#11667=VERTEX_POINT ( 'NONE', #32456 ) ;
#11668=CARTESIAN_POINT ( 'NONE',  ( -1.287880193524239658, 20.15907059199006923, -4.440276399826991849 ) ) ;
#11669=CARTESIAN_POINT ( 'NONE',  ( -4.379744549753617378, 120.5100497556178567, -0.6885478749808131571 ) ) ;
#11673=CARTESIAN_POINT ( 'NONE',  ( 7.793607028369248901, 122.5636234448803776, 0.3703801320152458887 ) ) ;
#11674=CARTESIAN_POINT ( 'NONE',  ( 1.072590735131739414, 20.86836736082219801, 4.503669761903479341 ) ) ;
#11675=CARTESIAN_POINT ( 'NONE',  ( 19.50329963654020915, 128.7319734376252143, 1.320013405138365181 ) ) ;
#11676=CARTESIAN_POINT ( 'NONE',  ( -6.486711254249450261E-14, 72.48346620154573827, 1.207165459670006807E-19 ) ) ;
#11677=CARTESIAN_POINT ( 'NONE',  ( 3.151249207183300260, -14.28495848352401332, 1.742053583190615207 ) ) ;
#11678=CARTESIAN_POINT ( 'NONE',  ( 13.58393798013047871, 155.6725583577350278, -1.480266515874766542 ) ) ;
#11679=CARTESIAN_POINT ( 'NONE',  ( -18.19397457907797744, 146.9188445454784357, 1.620492285849223446 ) ) ;
#11681=CARTESIAN_POINT ( 'NONE',  ( 0.4015916885733669117, -14.54189033959780808, -0.8905040343298938899 ) ) ;
#11682=CARTESIAN_POINT ( 'NONE',  ( -21.60506836338294789, 151.3813297165527274, -1.270904734852022377 ) ) ;
#11683=CARTESIAN_POINT ( 'NONE',  ( 0.1924800537393606958, 19.99376482044840486, 0.9543378882872525226 ) ) ;
#11684=ORIENTED_EDGE ( 'NONE', *, *, #42074, .F. ) ;
#11685=B_SPLINE_CURVE_WITH_KNOTS ( 'NONE', 3,
 ( #29736, #17364, #36140, #10558, #36357, #20131, #20333, #23743, #13333, #33359, #16943, #23529, #23106, #6957, #1201, #19926, #14161 ),
 .UNSPECIFIED., .F., .F.,
 ( 4, 1, 1, 1, 1, 1, 1, 1, 1, 1, 1, 1, 1, 1, 4 ),
 ( 0.000000000000000000, 0.05527712972171117123, 0.1031936715418271255, 0.1452310937008415292, 0.1830547385316705356, 0.2184069929475541683, 0.2529008548920727018, 0.3331866173837648715, 0.4227704555254401253, 0.5212776283956739309, 0.6247903393790393833, 0.7282327622823181468, 0.8267193445215066383, 0.9169988606028186551, 1.000000000000000000 ),
 .UNSPECIFIED. ) ;
#11687=CARTESIAN_POINT ( 'NONE',  ( -9.485477581651585055, 123.8597080710187015, 0.4105858232041853517 ) ) ;
#11688=CARTESIAN_POINT ( 'NONE',  ( 2.458590490134419770, -15.31022926314896893, 5.890968354261565842 ) ) ;
#11689=CARTESIAN_POINT ( 'NONE',  ( 1.452025732293782179, 120.0849730816093910, -0.4508766852696773908 ) ) ;
#11691=CIRCLE ( 'NONE', #21851, 5.588000000000006295 ) ;
#11692=CARTESIAN_POINT ( 'NONE',  ( 1.214457255922167134, 115.7029375523520116, 1.741465633879825781 ) ) ;
#11693=CIRCLE ( 'NONE', #23222, 4.826000000000001400 ) ;
#11694=CARTESIAN_POINT ( 'NONE',  ( 3.403332384622693052, -13.60094159685824877, 2.654810364998238192 ) ) ;
#11695=CARTESIAN_POINT ( 'NONE',  ( -4.750525968156759760, 117.8920781161146181, -0.9101660372078754779 ) ) ;
#11696=CARTESIAN_POINT ( 'NONE',  ( 11.06366964751653192, 128.0319838675845290, 0.1805508315534841424 ) ) ;
#11698=CARTESIAN_POINT ( 'NONE',  ( 11.58042324368370046, 121.0393782313542346, 1.653871040030608697 ) ) ;
#11700=DIRECTION ( 'NONE',  ( -0.9998004120163608288, -4.016384292689131511E-17, -0.01997839162482749342 ) ) ;
#11701=CARTESIAN_POINT ( 'NONE',  ( 0.009748065369120871224, 159.5507987164374981, -0.4878330526048096361 ) ) ;
#11702=CARTESIAN_POINT ( 'NONE',  ( 21.84047376210808267, 151.4369626909183637, -0.009531295849831044470 ) ) ;
#11705=CARTESIAN_POINT ( 'NONE',  ( 1.637592558569015644, -15.41088763797304750, 5.642738181119684171 ) ) ;
#11706=CARTESIAN_POINT ( 'NONE',  ( -6.654617103318593247E-14, 104.6144662015457243, 1.534725424433578570E-31 ) ) ;
#11708=CARTESIAN_POINT ( 'NONE',  ( -4.845225939460884312, 117.8262844396378739, 0.6941112827358852932 ) ) ;
#11712=B_SPLINE_CURVE_WITH_KNOTS ( 'NONE', 3,
 ( #4184, #30346, #40172, #3766 ),
 .UNSPECIFIED., .F., .F.,
 ( 4, 4 ),
 ( 0.000000000000000000, 1.000000000000000000 ),
 .UNSPECIFIED. ) ;
#11713=CARTESIAN_POINT ( 'NONE',  ( 3.124214023240655891, 118.2564054494065999, -0.7679563639302000588 ) ) ;
#11714=CARTESIAN_POINT ( 'NONE',  ( -4.119305931990809633, 118.0988315448752530, -0.8046943418515851709 ) ) ;
#11715=CARTESIAN_POINT ( 'NONE',  ( 4.831148843770026069, 117.6432307235636046, 1.088101262527759960 ) ) ;
#11717=CARTESIAN_POINT ( 'NONE',  ( -0.9377939088481974661, 122.9246775559910390, 0.1697371007065933135 ) ) ;
#11718=AXIS2_PLACEMENT_3D ( 'NONE', #22384, #35409, #1994 ) ;
#11719=CARTESIAN_POINT ( 'NONE',  ( 4.349802767100347189, -10.92635770930747796, -1.576909098649299512 ) ) ;
#11721=CARTESIAN_POINT ( 'NONE',  ( 5.586884702347364673, 87.97746620154572383, 0.1116392523995368424 ) ) ;
#11722=CARTESIAN_POINT ( 'NONE',  ( 2.022490532284443088, -15.01207906941262671, 5.472131392975311925 ) ) ;
#11723=CARTESIAN_POINT ( 'NONE',  ( 4.798759560707918759, 116.6039038697339549, -0.9352253033319916087 ) ) ;
#11725=DIRECTION ( 'NONE',  ( -0.9998004120163610509, -4.016384292689131511E-17, -0.01997839162482749689 ) ) ;
#11726=CARTESIAN_POINT ( 'NONE',  ( -1.708516274928095990, 115.7028613054959436, 1.661197570522961575 ) ) ;
#11727=CARTESIAN_POINT ( 'NONE',  ( -4.544942180623752215, 12.81246518813932589, 0.8472608254572608910 ) ) ;
#11729=CARTESIAN_POINT ( 'NONE',  ( 4.653890175952837716, 105.1215341841791258, -2.614083570717117944 ) ) ;
#11730=CARTESIAN_POINT ( 'NONE',  ( 2.493951430369484523, -15.64112390455543711, 5.038688225235472551 ) ) ;
#11731=CARTESIAN_POINT ( 'NONE',  ( -6.464497043865880421, 157.5392376370035095, 1.685792624679405716 ) ) ;
#11732=CARTESIAN_POINT ( 'NONE',  ( -0.9510052327539034733, 17.61975311242802533, 0.2078495401503242801 ) ) ;
#11733=CARTESIAN_POINT ( 'NONE',  ( -0.9148265087109853644, 12.81245955126885505, -0.3394028602373861392 ) ) ;
#11737=TOROIDAL_SURFACE ( 'NONE', #8336, 5.080000000000005400, 0.5080000000000000071 ) ;
#11739=CARTESIAN_POINT ( 'NONE',  ( -4.293188133933578676, 27.89088472858528078, 0.5134395162472098484 ) ) ;
#11740=CARTESIAN_POINT ( 'NONE',  ( 1.569003042721580865, 118.7759820277219944, 0.8276293794157989492 ) ) ;
#11742=CARTESIAN_POINT ( 'NONE',  ( -10.15138120625600138, 123.9924233945428682, 0.7101534938561541166 ) ) ;
#11744=CARTESIAN_POINT ( 'NONE',  ( 1.858891552337619935, -15.10179129218686178, 5.555419934288654993 ) ) ;
#11745=CARTESIAN_POINT ( 'NONE',  ( 9.322612814602670994, 121.5662863950884400, -1.087844926965479742 ) ) ;
#11746=CARTESIAN_POINT ( 'NONE',  ( -12.64856329662766043, 122.0451665396574725, -1.778165442619766834 ) ) ;
#11748=CARTESIAN_POINT ( 'NONE',  ( 4.121223586692221552, 118.2429491485453497, -0.1829416065829389815 ) ) ;
#11749=CARTESIAN_POINT ( 'NONE',  ( 6.491509040564920952, 121.7133186976561205, -0.1169240713195676962 ) ) ;
#11751=CARTESIAN_POINT ( 'NONE',  ( 1.824654213811243819, -15.25386490109567639, 5.420715704377902178 ) ) ;
#11755=CARTESIAN_POINT ( 'NONE',  ( 2.913282581332740762, -14.11548038430587937, -3.586046950971230274 ) ) ;
#11756=CARTESIAN_POINT ( 'NONE',  ( 10.14627733936753451, 123.6566696788710686, 1.220144418243291229 ) ) ;
#11757=CARTESIAN_POINT ( 'NONE',  ( -2.818619619938098175, 29.34630912614251130, 1.292122882726251420 ) ) ;
#11758=CARTESIAN_POINT ( 'NONE',  ( -2.169980103648603720, 106.6933082031156772, 4.882050113528205948 ) ) ;
#11760=CARTESIAN_POINT ( 'NONE',  ( -4.609222696788063622, 3.091975128091568159, 0.4746723485708761459 ) ) ;
#11761=CARTESIAN_POINT ( 'NONE',  ( -0.01249116623180958861, 38.87185441664305330, -1.227828225846576693 ) ) ;
#11763=CARTESIAN_POINT ( 'NONE',  ( -8.165053131321412749, -1.372107735949496421, -2.092221094348168275 ) ) ;
#11765=CARTESIAN_POINT ( 'NONE',  ( 5.538936621065253085, 116.8894077038538768, -0.3445561300999038790 ) ) ;
#11766=CARTESIAN_POINT ( 'NONE',  ( -1.058386756517351923, 124.8229041592835387, -0.03077316225166099040 ) ) ;
#11768=CARTESIAN_POINT ( 'NONE',  ( 4.300553167417687561, 27.50566818391071422, -1.719522505244270860 ) ) ;
#11769=CARTESIAN_POINT ( 'NONE',  ( 0.5436740362654144398, 117.9394487757135295, 1.407118881397579457 ) ) ;
#11772=CARTESIAN_POINT ( 'NONE',  ( 0.3819982885357794955, 122.2435587914033022, -0.2867773152523557245 ) ) ;
#11773=CARTESIAN_POINT ( 'NONE',  ( -13.30261597551697150, 156.9705208988102640, 0.2305920065817563536 ) ) ;
#11779=CARTESIAN_POINT ( 'NONE',  ( -8.041889123127157646, 122.8518031662551948, -0.1606960833125206101 ) ) ;
#11780=CARTESIAN_POINT ( 'NONE',  ( 2.462693652799142541, -15.54209007114785912, 5.820364621994587040 ) ) ;
#11781=CARTESIAN_POINT ( 'NONE',  ( -2.800559387825789948, 158.6924860557018064, 1.442603686385967254 ) ) ;
#11782=CARTESIAN_POINT ( 'NONE',  ( 22.40052491088791697, 148.4347612714453248, -0.9998933253014313793 ) ) ;
#11783=CARTESIAN_POINT ( 'NONE',  ( -1.756104463947763206, 14.33678105357426702, 4.288642365192034234 ) ) ;
#11784=CARTESIAN_POINT ( 'NONE',  ( -2.814065556059573314, 116.6946238705719594, -0.3036003272628903238 ) ) ;
#11787=CARTESIAN_POINT ( 'NONE',  ( -2.183620640279838376, 116.1905378774015105, -0.03043059125181128352 ) ) ;
#11789=CARTESIAN_POINT ( 'NONE',  ( -1.409223554827573999, 119.7856413326322667, 0.5222593444346083080 ) ) ;
#11791=CARTESIAN_POINT ( 'NONE',  ( 11.67114148714781940, 122.1450671466348439, -1.284540048876763096 ) ) ;
#11792=CARTESIAN_POINT ( 'NONE',  ( -7.848884907109314746, 118.8455990504009492, -1.250143668394028129 ) ) ;
#11794=VECTOR ( 'NONE', #15484, 1000.000000000000000 ) ;
#11796=CARTESIAN_POINT ( 'NONE',  ( 16.29799532358056524, 145.9442052555630767, -0.7927408685852873615 ) ) ;
#11798=CARTESIAN_POINT ( 'NONE',  ( -10.71425622041622994, 122.7614441063800399, -1.568315134061840865 ) ) ;
#11799=B_SPLINE_CURVE_WITH_KNOTS ( 'NONE', 3,
 ( #39635, #10648, #20430, #33035, #14051, #1505, #14252, #27055, #30452, #4076, #27260, #7050, #3863, #7470, #17452, #668, #14460, #16827, #33457, #29830, #13636, #7260, #40063, #40275, #30033, #20220, #39852, #37069, #17249, #33246, #11070, #23194, #36649, #23629, #17035, #10855 ),
 .UNSPECIFIED., .F., .F.,
 ( 4, 2, 2, 2, 2, 2, 2, 2, 2, 2, 2, 2, 2, 2, 2, 2, 2, 4 ),
 ( 0.01468215474677663467, 0.01563221235945116278, 0.01658226997212569609, 0.01705729877846295928, 0.01753232758480022246, 0.01848238519747474884, 0.01943244281014927521, 0.02038250042282380159, 0.02133255803549833143, 0.02228261564817285781, 0.02323267326084738418, 0.02418273087352190709, 0.02513278848619643693, 0.02608284609887095984, 0.02703290371154548968, 0.02798296132422001606, 0.02893301893689454243, 0.02988307654956906881 ),
 .UNSPECIFIED. ) ;
#11800=CARTESIAN_POINT ( 'NONE',  ( 4.222520559145931607, -15.42613134656034646, 1.120547993087879446 ) ) ;
#11801=CARTESIAN_POINT ( 'NONE',  ( -4.516505043337477154, 118.0894658202221592, -0.7769319744564929797 ) ) ;
#11803=CARTESIAN_POINT ( 'NONE',  ( -4.901356651777482476, 117.4105916379840266, 0.9668049386046483340 ) ) ;
#11804=CARTESIAN_POINT ( 'NONE',  ( 9.288997298956278570, 155.0893615026619159, 1.903066234436351145 ) ) ;
#11806=LINE ( 'NONE', #31403, #6980 ) ;
#11808=CARTESIAN_POINT ( 'NONE',  ( 7.466160517099046601, -1.205741384250370363, -3.973931221679563919 ) ) ;
#11809=CARTESIAN_POINT ( 'NONE',  ( 2.922188055539069573, 156.0861408873597327, 0.2775485887099104487 ) ) ;
#11814=CARTESIAN_POINT ( 'NONE',  ( -3.414070525044812676, 117.3993835098938661, 1.238193295900473334 ) ) ;
#11815=CARTESIAN_POINT ( 'NONE',  ( 4.722564864159155995, 118.7629491485453741, 0.9939262365100323127 ) ) ;
#11816=AXIS2_PLACEMENT_3D ( 'NONE', #1723, #39862, #13859 ) ;
#11817=ADVANCED_FACE ( 'NONE', ( #18610 ), #9237, .T. ) ;
#11820=CARTESIAN_POINT ( 'NONE',  ( -16.83721787035681317, 155.2408147041404050, -0.1288212628531381632 ) ) ;
#11821=ORIENTED_EDGE ( 'NONE', *, *, #15383, .F. ) ;
#11823=CARTESIAN_POINT ( 'NONE',  ( 7.931070413917881368, 121.9907963680717558, -0.6304219912953731297 ) ) ;
#11824=CARTESIAN_POINT ( 'NONE',  ( -7.845668857088636372, 122.3864107004520889, 0.3364293298510350194 ) ) ;
#11827=CARTESIAN_POINT ( 'NONE',  ( 0.3836050358042789599, 115.7029491485453292, -1.750603908414250176 ) ) ;
#11828=CARTESIAN_POINT ( 'NONE',  ( -15.41061421316654823, 147.8340308814284754, -0.6362464400602065862 ) ) ;
#11829=CIRCLE ( 'NONE', #20665, 0.5080000000000002292 ) ;
#11830=CARTESIAN_POINT ( 'NONE',  ( 5.123467091704872800, -13.13098499675426112, 2.859697440480786668 ) ) ;
#11831=CARTESIAN_POINT ( 'NONE',  ( -13.99438190394165282, 121.2764344996515717, 0.9244547817413872881 ) ) ;
#11833=CARTESIAN_POINT ( 'NONE',  ( 23.32994265436196457, 149.0590277239482475, 0.6203886826157013479 ) ) ;
#11834=CARTESIAN_POINT ( 'NONE',  ( 9.104209967887914701, 153.9432936505793066, 0.1819237819739444872 ) ) ;
#11836=CARTESIAN_POINT ( 'NONE',  ( 0.8015440831811396771, 19.08345756868062892, -0.5584349385947994238 ) ) ;
#11837=CARTESIAN_POINT ( 'NONE',  ( -6.898502017095935912, 117.1694300671557727, -0.1814136226821929376 ) ) ;
#11838=CARTESIAN_POINT ( 'NONE',  ( 5.008434261519718156, 117.3975399490705342, -0.7758999597088642730 ) ) ;
#11840=ADVANCED_FACE ( 'NONE', ( #5184 ), #31777, .T. ) ;
#11841=EDGE_LOOP ( 'NONE', ( #13671, #25984, #9287, #6100 ) ) ;
#11842=CARTESIAN_POINT ( 'NONE',  ( -8.556400685085039370, 118.9707913172079543, 0.9328110640611807503 ) ) ;
#11843=CARTESIAN_POINT ( 'NONE',  ( -1.997604609866625580, -12.39122764300357105, -4.168859717980781809 ) ) ;
#11844=CARTESIAN_POINT ( 'NONE',  ( 21.88420111187364725, 149.4141677464492091, 2.022441453707984227 ) ) ;
#11846=CARTESIAN_POINT ( 'NONE',  ( 12.47042458399945986, 121.5863879130357503, -1.220378502514999797 ) ) ;
#11848=CARTESIAN_POINT ( 'NONE',  ( 4.770677904581660300, 21.51973835935561041, 6.970347630165958819 ) ) ;
#11849=CARTESIAN_POINT ( 'NONE',  ( -14.16249321059125599, 121.1589565784038456, -1.397539518993202723 ) ) ;
#11850=CARTESIAN_POINT ( 'NONE',  ( 4.908480440954034130, 117.5478834382789302, -0.9161991286228470255 ) ) ;
#11851=CARTESIAN_POINT ( 'NONE',  ( 7.277551686224362548, 123.0424313102424492, 0.2142739940110135466 ) ) ;
#11853=CARTESIAN_POINT ( 'NONE',  ( -9.140193528981251703, 153.9061766533773152, 0.01708403265280381694 ) ) ;
#11854=CARTESIAN_POINT ( 'NONE',  ( 0.01133701094395666610, 119.0130636887059410, -0.5673503866435168908 ) ) ;
#11855=CARTESIAN_POINT ( 'NONE',  ( 3.423347803338410156, -15.46749709811699702, 5.412694551837634371 ) ) ;
#11857=EDGE_CURVE ( 'NONE', #41093, #19493, #1545, .T. ) ;
#11858=CARTESIAN_POINT ( 'NONE',  ( -4.297733157312593200, 118.1651005001141925, -0.6725186956912113656 ) ) ;
#11860=EDGE_LOOP ( 'NONE', ( #25357, #41608, #19765, #24136, #12824, #33750, #8311, #10853, #16518, #5121 ) ) ;
#11861=CARTESIAN_POINT ( 'NONE',  ( 4.079782966556019908, 157.3082466949932723, 1.825029598092313909 ) ) ;
#11864=CARTESIAN_POINT ( 'NONE',  ( -0.7355314204969178871, 116.0160817474902331, 1.626749668116675318 ) ) ;
#11865=CARTESIAN_POINT ( 'NONE',  ( -4.948315225313974608, -9.142465695005178361, 6.828157318318492486 ) ) ;
#11866=CARTESIAN_POINT ( 'NONE',  ( 12.05573777011642100, 128.3964238929853252, 1.202367467897996089 ) ) ;
#11868=CARTESIAN_POINT ( 'NONE',  ( 16.51027305157931480, 155.2380866766625047, -0.5525915368032876529 ) ) ;
#11871=CARTESIAN_POINT ( 'NONE',  ( -4.556757383386185190, 31.49269130883712720, -0.6906699653381264126 ) ) ;
#11873=CARTESIAN_POINT ( 'NONE',  ( 2.009495809369670649, -15.14277677434764335, 5.899592854099827477 ) ) ;
#11874=CARTESIAN_POINT ( 'NONE',  ( -4.250218791031737275, 118.2249388686620080, 0.3102279370716315432 ) ) ;
#11875=CARTESIAN_POINT ( 'NONE',  ( -23.34372044207216845, 149.0681261006882039, -0.4664630893996629113 ) ) ;
#11878=CARTESIAN_POINT ( 'NONE',  ( -6.145739716626447802, 119.6364497148305901, -1.247725477666507654 ) ) ;
#11879=CARTESIAN_POINT ( 'NONE',  ( -5.302405987100971885, 104.6144662015457101, 1.270606870302479541 ) ) ;
#11880=CARTESIAN_POINT ( 'NONE',  ( 4.357495859860891940, 118.1846395343606275, 0.6082252339746802017 ) ) ;
#11881=CARTESIAN_POINT ( 'NONE',  ( -15.79391552826349354, 147.6293441119438512, -1.163731531224506677 ) ) ;
#11883=CARTESIAN_POINT ( 'NONE',  ( 15.97340373827820947, 121.0409387471171101, 0.3191866212789526425 ) ) ;
#11885=CARTESIAN_POINT ( 'NONE',  ( -1.648064503646425649, 29.87956589480163316, -4.325937074807028715 ) ) ;
#11887=CARTESIAN_POINT ( 'NONE',  ( 5.008579095262371439, 117.3966161975143052, -0.7759206765000108419 ) ) ;
#11890=CARTESIAN_POINT ( 'NONE',  ( 7.788256506714744454, 122.5981892255041572, 0.2834234761349876397 ) ) ;
#11891=CARTESIAN_POINT ( 'NONE',  ( -1.535301415185580609, 19.99377045568717293, 4.360315235486975638 ) ) ;
#11892=CARTESIAN_POINT ( 'NONE',  ( 12.99089357651411980, 156.9259531928012734, 1.181820989919032838 ) ) ;
#11893=CARTESIAN_POINT ( 'NONE',  ( -4.831223284439005283, 104.6144662015457669, -0.2225614094029600976 ) ) ;
#11894=CARTESIAN_POINT ( 'NONE',  ( 3.162461164278121739, -14.57801340048104777, 3.369881103115548893 ) ) ;
#11895=CARTESIAN_POINT ( 'NONE',  ( 16.85638304633359752, 153.6818489539412553, -1.479736204719017900 ) ) ;
#11896=CARTESIAN_POINT ( 'NONE',  ( -14.24002733280072164, 152.6618899727951089, 1.673933364105639088 ) ) ;
#11897=CARTESIAN_POINT ( 'NONE',  ( 4.064150447026247726, 23.66704930264554818, -2.198397014704132513 ) ) ;
#11898=CARTESIAN_POINT ( 'NONE',  ( -22.95323918608241343, 146.5883926500602001, -1.439717189780889584 ) ) ;
#11899=CARTESIAN_POINT ( 'NONE',  ( -0.3594991891230457370, 15.46976683256975704, -0.9053751552070300468 ) ) ;
#11900=VERTEX_POINT ( 'NONE', #32198 ) ;
#11902=CARTESIAN_POINT ( 'NONE',  ( -6.492529462933222639, 121.6679077367135591, 0.1901135952749838376 ) ) ;
#11903=CARTESIAN_POINT ( 'NONE',  ( 5.545296128261989033, -13.31524510490228508, 2.629257322947794684 ) ) ;
#11904=CARTESIAN_POINT ( 'NONE',  ( 7.932268303790880992, 121.8456834504061845, -0.6952039612942494395 ) ) ;
#11906=CARTESIAN_POINT ( 'NONE',  ( 0.6559343604812126749, 115.7031630020738504, 1.758495348668634772 ) ) ;
#11908=CARTESIAN_POINT ( 'NONE',  ( -4.765159595197983933, 117.6707466944635456, -1.115707916067754546 ) ) ;
#11909=CARTESIAN_POINT ( 'NONE',  ( 8.831233598306480914, 123.6950213215744583, 0.09329271932673280365 ) ) ;
#11910=VECTOR ( 'NONE', #21853, 1000.000000000000000 ) ;
#11912=CARTESIAN_POINT ( 'NONE',  ( 12.21120734956418019, 121.7247091083657153, 1.742548127100890243 ) ) ;
#11915=CARTESIAN_POINT ( 'NONE',  ( 0.02400040557466870741, 156.7459281804771365, -1.201078436782489378 ) ) ;
#11916=CARTESIAN_POINT ( 'NONE',  ( 10.78032506485370945, 157.9328640892066460, -0.04097195671286529839 ) ) ;
#11918=CARTESIAN_POINT ( 'NONE',  ( 2.058562980619487615, -15.15559995322061937, 5.883026903270092589 ) ) ;
#11920=CARTESIAN_POINT ( 'NONE',  ( -6.442348895218290093E-14, 63.84746620154572838, 4.408874939877717575E-29 ) ) ;
#11921=CARTESIAN_POINT ( 'NONE',  ( -4.657921323837626915, 117.9598333327476638, 0.7454012569311468939 ) ) ;
#11923=ORIENTED_EDGE ( 'NONE', *, *, #30489, .T. ) ;
#11924=CARTESIAN_POINT ( 'NONE',  ( -0.02551629667440783247, 118.7629491485454025, 1.276939826302096348 ) ) ;
#11925=CARTESIAN_POINT ( 'NONE',  ( 2.764682666223415630, 117.8403247707871628, -0.7160347503476400810 ) ) ;
#11926=CARTESIAN_POINT ( 'NONE',  ( -0.4858112859843613518, 106.1608668108878817, -5.224277761219202176 ) ) ;
#11927=CARTESIAN_POINT ( 'NONE',  ( 4.851132313076204738, 117.6731831347222794, 1.041893731173013204 ) ) ;
#11928=CARTESIAN_POINT ( 'NONE',  ( -4.612970356601876709, 117.9306742281530660, -0.9648483343165797921 ) ) ;
#11929=CARTESIAN_POINT ( 'NONE',  ( -0.9632506926928976476, 123.2612876230388395, 0.1349244037310163846 ) ) ;
#11930=CARTESIAN_POINT ( 'NONE',  ( 0.4343283552818534288, -9.202337043772711667, -4.603842121470758997 ) ) ;
#11933=CARTESIAN_POINT ( 'NONE',  ( 3.537338181458673070, -13.91857904597952533, 4.048280000481319973 ) ) ;
#11934=CARTESIAN_POINT ( 'NONE',  ( 2.376338430377524347, 108.4767889311100362, -4.155189222081930644 ) ) ;
#11935=CARTESIAN_POINT ( 'NONE',  ( -15.22212811258888898, 150.6904849259475441, -2.083262412922771922 ) ) ;
#11936=CARTESIAN_POINT ( 'NONE',  ( 6.079889189570776509, 121.4459138077559714, 0.1214906566337395633 ) ) ;
#11939=CARTESIAN_POINT ( 'NONE',  ( -1.821252105156915713, 115.7029441824943063, 1.652972720107705573 ) ) ;
#11940=CARTESIAN_POINT ( 'NONE',  ( -0.9211762648548540433, 10.43857344512876040, -4.529598961101950927 ) ) ;
#11941=CARTESIAN_POINT ( 'NONE',  ( 22.39330865153371874, 150.7562895891929031, 1.036336034128335415 ) ) ;
#11942=VERTEX_POINT ( 'NONE', #34771 ) ;
#11943=CARTESIAN_POINT ( 'NONE',  ( 3.944401187668185038, 104.6144662015587983, -3.607510279707207168 ) ) ;
#11944=CARTESIAN_POINT ( 'NONE',  ( 4.191701569836151720, -15.46661069841161229, 1.593937231346424843 ) ) ;
#11945=CARTESIAN_POINT ( 'NONE',  ( -13.45896140341262637, 123.7870877700634509, 1.380644293323453065 ) ) ;
#11946=CARTESIAN_POINT ( 'NONE',  ( -0.9667957141098567631, 26.69201124214932719, -0.1227653459084327853 ) ) ;
#11947=CARTESIAN_POINT ( 'NONE',  ( 0.8487236205744517203, 17.35912690172634143, 0.4866769997786373203 ) ) ;
#11948=ORIENTED_EDGE ( 'NONE', *, *, #41205, .F. ) ;
#11951=CARTESIAN_POINT ( 'NONE',  ( 1.507062556099364459, 116.9323294830472122, 1.352967057238088300 ) ) ;
#11952=CARTESIAN_POINT ( 'NONE',  ( -10.20798870728745200, 124.0743415861677903, 0.7134647857254747816 ) ) ;
#11954=CARTESIAN_POINT ( 'NONE',  ( 3.666546702136318725, -13.72720857325485078, 3.759896688191319836 ) ) ;
#11955=CARTESIAN_POINT ( 'NONE',  ( 0.9295719194792341211, 157.1975648536147787, -1.475660455335214616 ) ) ;
#11956=CARTESIAN_POINT ( 'NONE',  ( -0.4360227397042136244, 118.4074432378348689, -0.6062663470103504260 ) ) ;
#11958=CARTESIAN_POINT ( 'NONE',  ( -4.897950286213627713, 117.7356713384708087, 0.7215056066125844492 ) ) ;
#11959=CARTESIAN_POINT ( 'NONE',  ( -2.169500164636428696, 35.42160933236649356, 3.123960633263314968 ) ) ;
#11960=CARTESIAN_POINT ( 'NONE',  ( 15.92043486079644943, 145.9828583539951126, -0.2780828054990247544 ) ) ;
#11962=CARTESIAN_POINT ( 'NONE',  ( 2.755019269514601632, -14.09852029293599784, -0.1464032776252038315 ) ) ;
#11964=CARTESIAN_POINT ( 'NONE',  ( -3.938977128594349342, 28.07268674286775223, 0.7495841607770360460 ) ) ;
#11966=CIRCLE ( 'NONE', #26965, 0.5079999999999997851 ) ;
#11967=CARTESIAN_POINT ( 'NONE',  ( 0.8067276567327370529, -3.745225398377231674, -4.556403025205434609 ) ) ;
#11968=CARTESIAN_POINT ( 'NONE',  ( 11.65596162629424626, 126.1299551460304542, 1.384704262848757805 ) ) ;
#11969=CARTESIAN_POINT ( 'NONE',  ( -0.8587611443208003070, 32.35200983223521121, 3.578619333304415839 ) ) ;
#11970=CARTESIAN_POINT ( 'NONE',  ( -7.093755517943445277, 122.4291926079955317, -0.03209900709771745103 ) ) ;
#11971=CARTESIAN_POINT ( 'NONE',  ( 1.360477052538118681, -3.804838552850991817, 4.419457122809256511 ) ) ;
#11972=CARTESIAN_POINT ( 'NONE',  ( 6.503408402854558013, 121.7799126398724354, 0.1299535771408518448 ) ) ;
#11973=CARTESIAN_POINT ( 'NONE',  ( 8.086262078954034038, 3.373778641329666872, 2.357548046588672008 ) ) ;
#11975=CARTESIAN_POINT ( 'NONE',  ( -5.526528724494175648, 116.8573403164261464, -0.5291618397137183294 ) ) ;
#11976=CARTESIAN_POINT ( 'NONE',  ( -0.3558893179482170432, 120.1716774721349168, -0.6349178681961804571 ) ) ;
#11979=CARTESIAN_POINT ( 'NONE',  ( 7.253464168720983096, -10.72948646729439659, -4.330533999219945862 ) ) ;
#11980=CARTESIAN_POINT ( 'NONE',  ( 3.969496458384241588, 117.3993838096581754, 1.318317423491925933 ) ) ;
#11982=DIRECTION ( 'NONE',  ( -4.017660918040594346E-17, 1.000000000000000000, 2.376309959284834438E-19 ) ) ;
#11983=CARTESIAN_POINT ( 'NONE',  ( 0.3766127027001021088, 114.7739974199301116, -2.035987775551919565 ) ) ;
#11984=CARTESIAN_POINT ( 'NONE',  ( -18.44051311885898059, 154.1649927243852858, 0.3121108635588942803 ) ) ;
#11987=ORIENTED_EDGE ( 'NONE', *, *, #27682, .T. ) ;
#11988=CARTESIAN_POINT ( 'NONE',  ( -6.640726327341849406E-14, 100.6774662015457409, -1.320564745697255449E-18 ) ) ;
#11989=CARTESIAN_POINT ( 'NONE',  ( -14.67804715971658602, 148.8626627518845282, -0.1611556191706381425 ) ) ;
#11990=CARTESIAN_POINT ( 'NONE',  ( 2.090134903116885656, -15.63197564439436427, 5.828951795168951122 ) ) ;
#11991=CARTESIAN_POINT ( 'NONE',  ( -13.13885824085865828, 121.7804325175133755, 1.194399340605180049 ) ) ;
#11992=CARTESIAN_POINT ( 'NONE',  ( 20.10769848529506021, 132.0867704272472452, -0.9164310550120229326 ) ) ;
#11993=CARTESIAN_POINT ( 'NONE',  ( 3.548611814566905664, 16.26088872207684943, 2.983771105379771971 ) ) ;
#11995=CARTESIAN_POINT ( 'NONE',  ( -11.61197380483888608, 118.7506923092098674, -0.5208889651483785688 ) ) ;
#11999=CARTESIAN_POINT ( 'NONE',  ( -8.798384421702362346, 117.6845712617741526, -0.1566951044598125509 ) ) ;
#12000=DIRECTION ( 'NONE',  ( -0.9998004120163609398, 0.000000000000000000, -0.01997839162482749689 ) ) ;
#12001=CARTESIAN_POINT ( 'NONE',  ( -17.47151851664391842, 144.3974720067888313, 1.548345126349529810 ) ) ;
#12004=CARTESIAN_POINT ( 'NONE',  ( 12.31762543427494627, 122.6846661264431191, -1.317417697584883030 ) ) ;
#12005=CARTESIAN_POINT ( 'NONE',  ( -21.20529034131901369, 148.8133262010608462, -2.309157841868048067 ) ) ;
#12007=CARTESIAN_POINT ( 'NONE',  ( 9.588254403178050111, 123.8224200044116827, -0.4900104160083061933 ) ) ;
#12009=CARTESIAN_POINT ( 'NONE',  ( -6.574985064279145419, 120.4115791468657903, -1.154926965394999172 ) ) ;
#12010=CARTESIAN_POINT ( 'NONE',  ( 4.238804029399687145, -15.60588767656335918, 2.735912002563000822 ) ) ;
#12011=CARTESIAN_POINT ( 'NONE',  ( -4.158055769619781294, 118.2393601024573542, -0.3861629315888617242 ) ) ;
#12013=CARTESIAN_POINT ( 'NONE',  ( -4.922306677375791750, 117.4109580117980016, 0.9480543157666212473 ) ) ;
#12014=CARTESIAN_POINT ( 'NONE',  ( 2.483060992037590786, 119.7126118883416410, 0.6995635895845426777 ) ) ;
#12018=CARTESIAN_POINT ( 'NONE',  ( -1.495267265506447174, 0.7142801726123456652, -8.304712878169773660 ) ) ;
#12019=CARTESIAN_POINT ( 'NONE',  ( 1.593749994915877100, 120.9451058151398399, 0.1271097986196582930 ) ) ;
#12023=VERTEX_POINT ( 'NONE', #25792 ) ;
#12025=CARTESIAN_POINT ( 'NONE',  ( 2.168162777261974927, 118.7629491485453883, 1.225215063869133703 ) ) ;
#12029=CARTESIAN_POINT ( 'NONE',  ( -23.19846888548993746, 149.6199392087789306, -0.2334144245939552276 ) ) ;
#12030=ORIENTED_EDGE ( 'NONE', *, *, #6503, .F. ) ;
#12032=CARTESIAN_POINT ( 'NONE',  ( 6.935819294119811573, 121.8978577362516234, -0.1235646913352505261 ) ) ;
#12035=CARTESIAN_POINT ( 'NONE',  ( 1.835530157581306332, 115.7029480720426591, -1.651926545036461302 ) ) ;
#12036=CARTESIAN_POINT ( 'NONE',  ( -6.489379754819826651, 121.7611753534313550, -0.2571143975131356951 ) ) ;
#12037=CARTESIAN_POINT ( 'NONE',  ( 5.228661469329079381, -12.87456325985388084, 2.426867231591100182 ) ) ;
#12038=CARTESIAN_POINT ( 'NONE',  ( -5.877369116562103812, 117.9059190437751141, 0.7167914486236911520 ) ) ;
#12040=CARTESIAN_POINT ( 'NONE',  ( 0.8290186328064587107, 117.3993839335269485, -1.455277270773371434 ) ) ;
#12041=CARTESIAN_POINT ( 'NONE',  ( 9.803363283900793590, 117.9968303279965340, 0.2884128246907768922 ) ) ;
#12042=TOROIDAL_SURFACE ( 'NONE', #14771, 3.683000000000000718, 0.5080000000000000071 ) ;
#12043=CARTESIAN_POINT ( 'NONE',  ( 15.64098958305955023, 147.2213129253950399, 0.3794339001978928594 ) ) ;
#12045=CARTESIAN_POINT ( 'NONE',  ( -0.7219274401084647685, 31.37879824840181442, -0.6700674276139703123 ) ) ;
#12046=CARTESIAN_POINT ( 'NONE',  ( -8.067923148479989592, 158.6666700270975525, -0.2162342711943721629 ) ) ;
#12047=DIRECTION ( 'NONE',  ( -0.9998004120163609398, 0.000000000000000000, -0.01997839162482749689 ) ) ;
#12050=CARTESIAN_POINT ( 'NONE',  ( -6.005079809368049304, 118.6866504246635685, 0.9671915185187860420 ) ) ;
#12051=DIRECTION ( 'NONE',  ( 0.01997839162482749342, 1.040247600000944484E-18, -0.9998004120163608288 ) ) ;
#12052=CARTESIAN_POINT ( 'NONE',  ( 7.361208496634183973, 158.3992165788449711, 1.430753602065345298 ) ) ;
#12053=AXIS2_PLACEMENT_3D ( 'NONE', #31877, #38277, #41903 ) ;
#12054=CARTESIAN_POINT ( 'NONE',  ( 19.44243145639580916, 150.5708382285403388, -1.622132703307645585 ) ) ;
#12055=CARTESIAN_POINT ( 'NONE',  ( 4.581910832313284665, -15.30292673639559098, -0.5105377408573423814 ) ) ;
#12056=CARTESIAN_POINT ( 'NONE',  ( -2.976591712665178857, 117.3922842568077698, -0.6615242749010380452 ) ) ;
#12057=CARTESIAN_POINT ( 'NONE',  ( 4.888091618989467868, 117.6742611811322377, -0.8477283077776146536 ) ) ;
#12058=CARTESIAN_POINT ( 'NONE',  ( 0.1515127994569460956, 105.8822825325953261, 5.338933990912773098 ) ) ;
#12059=EDGE_CURVE ( 'NONE', #35669, #14129, #19872, .T. ) ;
#12061=CARTESIAN_POINT ( 'NONE',  ( -9.118838228053551376, 124.0847320388339625, -0.09724818526966641508 ) ) ;
#12062=CARTESIAN_POINT ( 'NONE',  ( -8.179471065859175383, 156.5149677146980309, -2.065073912022258984 ) ) ;
#12064=CARTESIAN_POINT ( 'NONE',  ( 3.628834229889370544, -15.44114452258853198, 5.288308529986511353 ) ) ;
#12065=CARTESIAN_POINT ( 'NONE',  ( 4.795789683585542029, 115.6909491485453145, 1.474960089930022145 ) ) ;
#12067=CARTESIAN_POINT ( 'NONE',  ( -2.526208763716937700, 118.1651004855683880, -0.8247881296101019499 ) ) ;
#12069=CARTESIAN_POINT ( 'NONE',  ( 6.619107555072841542, 119.9895581359321994, 1.245414878088068278 ) ) ;
#12070=CARTESIAN_POINT ( 'NONE',  ( -2.958531772299361151, 39.20946620154573736, -1.329372033065077119 ) ) ;
#12071=CARTESIAN_POINT ( 'NONE',  ( -4.228827370592760815, 117.9846523178514985, -0.9720340673296122835 ) ) ;
#12072=AXIS2_PLACEMENT_3D ( 'NONE', #21776, #2227, #41410 ) ;
#12073=CARTESIAN_POINT ( 'NONE',  ( -3.315740949751885491, 124.7872298565087021, -0.06001882965729953001 ) ) ;
#12074=CARTESIAN_POINT ( 'NONE',  ( -2.878135459294852705, -8.718908198948343014, 7.912908975683875745 ) ) ;
#12075=CARTESIAN_POINT ( 'NONE',  ( 4.469395743914975405, 155.8822484669112214, 0.8121950557409373106 ) ) ;
#12077=CARTESIAN_POINT ( 'NONE',  ( 3.207477133065330221, 159.4163042773305676, -0.4796247595147197784 ) ) ;
#12082=DIRECTION ( 'NONE',  ( -0.9998004120163608288, 0.000000000000000000, -0.01997839162482750383 ) ) ;
#12083=CARTESIAN_POINT ( 'NONE',  ( -4.160656731207808434, 118.2392941210594017, 0.2307236797113647875 ) ) ;
#12084=CARTESIAN_POINT ( 'NONE',  ( -2.732111087507159475, 116.5293111276780849, -0.05459408159141355271 ) ) ;
#12087=CARTESIAN_POINT ( 'NONE',  ( 4.076354001419692175, 119.1815227253801055, -0.7633122449047639035 ) ) ;
#12088=CARTESIAN_POINT ( 'NONE',  ( 0.1065646865915093611, 105.8844662015456777, -5.332932678536313809 ) ) ;
#12089=CARTESIAN_POINT ( 'NONE',  ( -5.883037304650423849, 121.3687970875902806, -0.4830333308872107878 ) ) ;
#12090=LINE ( 'NONE', #37443, #22634 ) ;
#12093=CARTESIAN_POINT ( 'NONE',  ( -1.471791394198959102, 24.03230288535706549, 4.399545648925609065 ) ) ;
#12095=CARTESIAN_POINT ( 'NONE',  ( 2.666490510518176649, -13.49855353256042712, 0.05227394649444803282 ) ) ;
#12098=CARTESIAN_POINT ( 'NONE',  ( -6.080819731615315860, 121.3676167066096241, 0.1940160119882017309 ) ) ;
#12101=CARTESIAN_POINT ( 'NONE',  ( 19.35449845750112274, 128.7092500879292345, 1.403651888282934079 ) ) ;
#12102=DIRECTION ( 'NONE',  ( -0.9998004120163609398, 0.000000000000000000, -0.01997839162482749689 ) ) ;
#12103=CARTESIAN_POINT ( 'NONE',  ( 1.979187190576821465, -15.21425526833739639, 5.301287498526151332 ) ) ;
#12104=CARTESIAN_POINT ( 'NONE',  ( 21.36815210116601804, 148.0064520001644723, -1.462276224275803838 ) ) ;
#12105=CARTESIAN_POINT ( 'NONE',  ( -18.22365405440210395, 148.2327041560005512, 1.660465927639720451 ) ) ;
#12106=CARTESIAN_POINT ( 'NONE',  ( -2.673854242087471356, 19.56896771519852862, 3.769861741755948348 ) ) ;
#12107=CARTESIAN_POINT ( 'NONE',  ( -5.539025187978821485, 159.0643023895801491, -0.7880117631591500027 ) ) ;
#12109=CARTESIAN_POINT ( 'NONE',  ( 0.7196250225040555781, 4.026961778641204859, -0.6563066166970625837 ) ) ;
#12110=EDGE_LOOP ( 'NONE', ( #14983, #33747, #33115, #21411, #30259, #9247, #17002, #880, #16285, #29177, #20885, #985, #19047 ) ) ;
#12112=CARTESIAN_POINT ( 'NONE',  ( -13.73699108721726425, 150.2158912636999730, 0.3005180155469770464 ) ) ;
#12113=CARTESIAN_POINT ( 'NONE',  ( 2.642260502442670855, -15.21879886190521880, 5.833332612881661383 ) ) ;
#12114=CARTESIAN_POINT ( 'NONE',  ( 13.46182233857065746, 130.9706359334022920, -1.049250031952806639 ) ) ;
#12115=ORIENTED_EDGE ( 'NONE', *, *, #27647, .T. ) ;
#12116=CARTESIAN_POINT ( 'NONE',  ( 2.402331870585372897, 115.7029513689469837, 1.700325149627530896 ) ) ;
#12117=ADVANCED_FACE ( 'NONE', ( #18559 ), #25178, .F. ) ;
#12118=ORIENTED_EDGE ( 'NONE', *, *, #11533, .F. ) ;
#12119=CARTESIAN_POINT ( 'NONE',  ( -4.798808526209403347, 117.8360179528525009, -0.9160348425365787417 ) ) ;
#12120=CARTESIAN_POINT ( 'NONE',  ( 15.72486432277149504, 146.8976350983841144, 0.2628874744899977189 ) ) ;
#12122=CARTESIAN_POINT ( 'NONE',  ( 19.54281269640863883, 149.4594839399872512, 2.484111515072797260 ) ) ;
#12126=CARTESIAN_POINT ( 'NONE',  ( 3.174366308151882254, 65.62546620154573418, 0.06343139340882768262 ) ) ;
#12127=CARTESIAN_POINT ( 'NONE',  ( 23.07880092997886834, 149.8841935741895384, 0.1310273949726225018 ) ) ;
#12128=CARTESIAN_POINT ( 'NONE',  ( 0.03519895179119666290, 115.7029491485446613, -1.761499482103947800 ) ) ;
#12129=CARTESIAN_POINT ( 'NONE',  ( 4.794367976492847738, 118.7629491485453030, -0.7451781752328570096 ) ) ;
#12131=CARTESIAN_POINT ( 'NONE',  ( 1.689144583495898244, -15.40064781548841566, 5.488289493485431159 ) ) ;
#12133=CARTESIAN_POINT ( 'NONE',  ( -4.691480036221459038, 117.9634116254975851, 0.7149672312120951556 ) ) ;
#12138=CARTESIAN_POINT ( 'NONE',  ( -5.705078924488119263, 118.5997860065700706, -1.215602027761154336 ) ) ;
#12139=CARTESIAN_POINT ( 'NONE',  ( -3.997939770797883874, 117.2022048034790487, -1.046317678458332345 ) ) ;
#12140=CARTESIAN_POINT ( 'NONE',  ( 4.768425879922006949, 117.4736019235508451, 1.192991665150185066 ) ) ;
#12142=CARTESIAN_POINT ( 'NONE',  ( -0.3095834102099264129, 110.3683645023726427, 3.577238406694227546 ) ) ;
#12143=CARTESIAN_POINT ( 'NONE',  ( 4.224370802630715183, -2.505441902618962935, 1.893578447770203566 ) ) ;
#12145=CARTESIAN_POINT ( 'NONE',  ( -6.580517660824093636E-14, 85.69146620154573668, -4.881702850681514412E-18 ) ) ;
#12146=CARTESIAN_POINT ( 'NONE',  ( 3.475384634610537038, -12.95405113104661154, 1.817132104271814264 ) ) ;
#12147=CARTESIAN_POINT ( 'NONE',  ( 4.802295984089199443, 116.4582014290525507, -0.9960034115346418915 ) ) ;
#12148=CARTESIAN_POINT ( 'NONE',  ( -9.709460118793561634, 122.6450757329969434, -1.337221984871323599 ) ) ;
#12149=CARTESIAN_POINT ( 'NONE',  ( 5.586884702347365561, 66.64146620154573952, 0.1116392523995368286 ) ) ;
#12150=CARTESIAN_POINT ( 'NONE',  ( 0.4719448309135433339, 39.20946620154573026, 1.279684108228161143 ) ) ;
#12151=CARTESIAN_POINT ( 'NONE',  ( -1.114995187443168945, 115.7029400263136125, 1.703459770062234702 ) ) ;
#12152=CARTESIAN_POINT ( 'NONE',  ( -3.366035089439492811, 13.68705809737886447, 3.178168622443589886 ) ) ;
#12153=CARTESIAN_POINT ( 'NONE',  ( 4.790162199822003863, 116.9482543694763166, 0.4383784235352166658 ) ) ;
#12155=CARTESIAN_POINT ( 'NONE',  ( 4.373232311943012540, 105.1218443201365602, -3.060007391163885870 ) ) ;
#12156=CARTESIAN_POINT ( 'NONE',  ( 2.350550293776238586, -15.63281720864678803, 5.143235457246400522 ) ) ;
#12157=CARTESIAN_POINT ( 'NONE',  ( -15.27645447632550280, 153.0676604005411434, 1.747501773188613994 ) ) ;
#12159=CARTESIAN_POINT ( 'NONE',  ( 0.3717569628964236816, 23.89034148085472964, -0.9007439114964531646 ) ) ;
#12160=CARTESIAN_POINT ( 'NONE',  ( 0.6184700321857297123, 7.203955656377674543, 0.7581051976356608657 ) ) ;
#12162=VERTEX_POINT ( 'NONE', #2824 ) ;
#12164=CARTESIAN_POINT ( 'NONE',  ( 2.331513492273026511, 111.1666841684333633, 3.236375129800146411 ) ) ;
#12165=CARTESIAN_POINT ( 'NONE',  ( -11.07452758269552895, 153.1537610418535849, 0.9542791616922486897 ) ) ;
#12167=CARTESIAN_POINT ( 'NONE',  ( 3.815374714676033729, -13.42234902974577615, 3.291045305163978085 ) ) ;
#12168=CARTESIAN_POINT ( 'NONE',  ( 2.509025565091295373, 119.7126118883416410, -0.5998098196673841143 ) ) ;
#12169=CARTESIAN_POINT ( 'NONE',  ( -20.22212501804825635, 145.4934252350392114, -2.489959791085248231 ) ) ;
#12171=ADVANCED_FACE ( 'NONE', ( #2406 ), #11737, .T. ) ;
#12172=CARTESIAN_POINT ( 'NONE',  ( 7.849374513171908596, 122.2536118085260171, 0.7624099742200379781 ) ) ;
#12173=CARTESIAN_POINT ( 'NONE',  ( 4.074910602682932925, 118.2429491485453354, -0.1454311599470142491 ) ) ;
#12174=CARTESIAN_POINT ( 'NONE',  ( 12.04197430995775164, 130.4833683797432684, -0.05493623226408298615 ) ) ;
#12175=ORIENTED_EDGE ( 'NONE', *, *, #790, .F. ) ;
#12176=CARTESIAN_POINT ( 'NONE',  ( -1.248055628918211646, 106.2083702520889119, -5.188232620816602747 ) ) ;
#12183=CARTESIAN_POINT ( 'NONE',  ( 8.093748642744952093, 23.43776531741863423, -2.407353130276413733 ) ) ;
#12184=CARTESIAN_POINT ( 'NONE',  ( 9.904299505090465416, 154.0333045108203009, 1.503511620041811936 ) ) ;
#12186=CARTESIAN_POINT ( 'NONE',  ( 20.47124607682627584, 129.0748834149669904, 0.3487454591146179061 ) ) ;
#12187=CARTESIAN_POINT ( 'NONE',  ( -5.326805317745573198, 116.9650601603920279, 0.7421267338694930160 ) ) ;
#12188=CARTESIAN_POINT ( 'NONE',  ( -4.157303687089163979, 2.242350289152962528, -2.029258473605290103 ) ) ;
#12189=CARTESIAN_POINT ( 'NONE',  ( 11.83539255247743149, 152.0195595274622349, 0.2364993098673506822 ) ) ;
#12190=CARTESIAN_POINT ( 'NONE',  ( 2.407351327831447119, 1.847773219181642057, 8.093752867084216263 ) ) ;
#12192=CARTESIAN_POINT ( 'NONE',  ( -8.737319200505471173, 117.9293801533141419, -0.7003869330726086861 ) ) ;
#12193=CARTESIAN_POINT ( 'NONE',  ( -1.032349031751560231, 124.2655319029901335, -0.08020592950830171541 ) ) ;
#12195=CARTESIAN_POINT ( 'NONE',  ( -6.618965589514436111E-14, 97.88346620154572975, 1.207165459396359365E-19 ) ) ;
#12196=CARTESIAN_POINT ( 'NONE',  ( -4.349660437102230048, 31.17966527223318707, -1.615541842050199461 ) ) ;
#12197=CARTESIAN_POINT ( 'NONE',  ( 0.4921998799175691941, 117.3993826277446146, 1.493758782920931338 ) ) ;
#12199=DIRECTION ( 'NONE',  ( -5.206863593109713661E-17, 1.000000000000000000, -1.077750396879097183E-30 ) ) ;
#12200=CARTESIAN_POINT ( 'NONE',  ( 0.2185697341916492398, 107.6766875080336376, -4.612355970162428598 ) ) ;
#12201=CARTESIAN_POINT ( 'NONE',  ( -10.65151157945287785, 157.9324367681937815, 0.3596066298475820155 ) ) ;
#12204=AXIS2_PLACEMENT_3D ( 'NONE', #40342, #37542, #17724 ) ;
#12206=ORIENTED_EDGE ( 'NONE', *, *, #19359, .F. ) ;
#12208=CARTESIAN_POINT ( 'NONE',  ( -15.20382161411771271, 143.4031467678206297, -0.1686640459771217015 ) ) ;
#12209=CARTESIAN_POINT ( 'NONE',  ( 6.238852630440780977, -14.32403127715267743, 0.8647906437036265714 ) ) ;
#12210=CARTESIAN_POINT ( 'NONE',  ( -20.61281631175405238, 145.6130255286810495, 1.629730044589046578 ) ) ;
#12211=CARTESIAN_POINT ( 'NONE',  ( 7.538779372106241716, 158.4854300789945398, -0.9926846707982194262 ) ) ;
#12212=CARTESIAN_POINT ( 'NONE',  ( -3.562413952978887632, 23.18266144714348798, 2.948169924785601470 ) ) ;
#12213=CARTESIAN_POINT ( 'NONE',  ( -22.49834027909124501, 137.1624432810789358, -0.8864494676080413305 ) ) ;
#12216=CARTESIAN_POINT ( 'NONE',  ( -0.004379098345612333562, 122.8649044353672934, 0.2191479880733796237 ) ) ;
#12218=CARTESIAN_POINT ( 'NONE',  ( -12.55519531044868486, 126.0212559692275249, 1.204658208757142468 ) ) ;
#12220=CARTESIAN_POINT ( 'NONE',  ( 10.61219202124994609, 121.9340018749941663, -1.210411277014657561 ) ) ;
#12221=CARTESIAN_POINT ( 'NONE',  ( -18.79035964875408382, 131.8417273817641444, -2.102833481017198025 ) ) ;
#12223=EDGE_CURVE ( 'NONE', #41093, #9715, #35552, .T. ) ;
#12224=CARTESIAN_POINT ( 'NONE',  ( 2.706440023329436340, 120.6505882111413683, -0.2907491850344327555 ) ) ;
#12226=CARTESIAN_POINT ( 'NONE',  ( -17.60198365394341735, 148.3509993576462307, -2.281626375285575214 ) ) ;
#12227=CARTESIAN_POINT ( 'NONE',  ( 3.555176734920527437, -15.70662665601262020, 4.164229356387482817 ) ) ;
#12228=CARTESIAN_POINT ( 'NONE',  ( -6.540217103314379345E-14, 82.64346620154573486, 2.383338306179204368E-29 ) ) ;
#12231=CARTESIAN_POINT ( 'NONE',  ( -4.899759748343297083, 117.5479811350548829, 0.9251532171549939898 ) ) ;
#12232=CARTESIAN_POINT ( 'NONE',  ( 16.68865417205000767, 140.0893442862094673, 2.224985475129671819 ) ) ;
#12234=CARTESIAN_POINT ( 'NONE',  ( 1.223683442775902463, 5.461509463947571419, 8.358860550006438572 ) ) ;
#12235=CARTESIAN_POINT ( 'NONE',  ( 6.485149764178022913, 121.7431354732680973, 0.3115821950655747186 ) ) ;
#12239=CARTESIAN_POINT ( 'NONE',  ( -0.1178540848408428932, 118.1588900175827774, 0.9046132285812910068 ) ) ;
#12242=CARTESIAN_POINT ( 'NONE',  ( -7.920550782940143364, 121.8828277235336657, -1.006747304157872502 ) ) ;
#12245=CARTESIAN_POINT ( 'NONE',  ( -18.62524206359434231, 154.1412379532633850, -0.2279367985168733735 ) ) ;
#12248=CARTESIAN_POINT ( 'NONE',  ( -7.794982761785219871, 122.5553005452032664, -0.3869435098480608626 ) ) ;
#12249=FACE_OUTER_BOUND ( 'NONE', #9315, .T. ) ;
#12250=VERTEX_POINT ( 'NONE', #12601 ) ;
#12251=CARTESIAN_POINT ( 'NONE',  ( 2.010736835508156961, 115.7029473884088446, -1.638949895126919687 ) ) ;
#12252=CARTESIAN_POINT ( 'NONE',  ( -15.80103543825248025, 146.2514283349100594, -0.5462135236119773918 ) ) ;
#12253=CARTESIAN_POINT ( 'NONE',  ( 2.063686733023943898, -15.30319371230426384, 5.972472134935498111 ) ) ;
#12254=CARTESIAN_POINT ( 'NONE',  ( -2.888962495635027050, 158.8946464937287999, 1.317949658345222153 ) ) ;
#12256=CARTESIAN_POINT ( 'NONE',  ( 6.905720769004601856, 117.2044255678715814, 0.3198409844323961138 ) ) ;
#12257=CARTESIAN_POINT ( 'NONE',  ( 10.94874868616072305, 127.9616117985000443, 0.3245695131468429584 ) ) ;
#12259=CARTESIAN_POINT ( 'NONE',  ( -0.2871545817224689379, 15.30011720780053430, 0.9385489134671207712 ) ) ;
#12260=CARTESIAN_POINT ( 'NONE',  ( -5.786284826928912217, 116.9447284183608389, -0.1988161383433786344 ) ) ;
#12262=EDGE_CURVE ( 'NONE', #38547, #1745, #28055, .T. ) ;
#12266=B_SPLINE_CURVE_WITH_KNOTS ( 'NONE', 3,
 ( #39141, #9529, #32751, #10374, #9946, #600, #22709, #35738, #32114, #3585, #13573, #13357, #29556, #26346, #19105, #29117, #10156, #22497 ),
 .UNSPECIFIED., .F., .F.,
 ( 4, 2, 2, 2, 2, 2, 2, 2, 4 ),
 ( 0.0003740220254444729222, 0.003617377532827396533, 0.006860733040210320252, 0.008482410793901782112, 0.009293249670747497429, 0.01010408854759321275, 0.01172576630128463991, 0.01253660517813036390, 0.01334744405497608789 ),
 .UNSPECIFIED. ) ;
#12267=CARTESIAN_POINT ( 'NONE',  ( 3.447093754558173462, 117.7853021311141930, 0.8661349407177386661 ) ) ;
#12268=CARTESIAN_POINT ( 'NONE',  ( 1.818839793882075506, -13.69063247836898434, -4.255424433905749204 ) ) ;
#12269=CARTESIAN_POINT ( 'NONE',  ( 0.3947855200658545449, 117.7785671674745771, 0.5311790665990140381 ) ) ;
#12270=CARTESIAN_POINT ( 'NONE',  ( 5.883382875664553424, 118.7305451321402501, -0.9239882381799516819 ) ) ;
#12271=CARTESIAN_POINT ( 'NONE',  ( 4.581790953832888924, -15.30257397518579232, -0.5115867857466148694 ) ) ;
#12272=CARTESIAN_POINT ( 'NONE',  ( -15.97393847379854215, 155.1095016151506911, -1.658827062323852575 ) ) ;
#12273=CARTESIAN_POINT ( 'NONE',  ( 4.809314660303178890, 117.8761932044920684, -0.6706302678270985584 ) ) ;
#12275=CARTESIAN_POINT ( 'NONE',  ( -0.1065646865916381608, 105.8844662015456777, 5.332932678536313809 ) ) ;
#12276=CARTESIAN_POINT ( 'NONE',  ( -7.567922279963403831, 122.4257779438054285, -0.07478732235760089664 ) ) ;
#12277=CARTESIAN_POINT ( 'NONE',  ( -11.88796246241990673, 122.6721150436042223, -1.770419579776735697 ) ) ;
#12278=CARTESIAN_POINT ( 'NONE',  ( 5.567940837815767097, -14.86657585147074734, 2.969021103613282531 ) ) ;
#12279=CARTESIAN_POINT ( 'NONE',  ( 5.239656519176586258, 115.6909491485453145, 1.022206641662168236 ) ) ;
#12281=CARTESIAN_POINT ( 'NONE',  ( -0.7927369056973760930, 117.9496054624362245, -1.398781258546966555 ) ) ;
#12282=EDGE_CURVE ( 'NONE', #5065, #1213, #38289, .T. ) ;
#12283=VERTEX_POINT ( 'NONE', #10815 ) ;
#12284=CARTESIAN_POINT ( 'NONE',  ( 18.87709319873806990, 147.8663216482595146, 2.479723349601893112 ) ) ;
#12285=CARTESIAN_POINT ( 'NONE',  ( 5.237379388564934679, 115.7029491485453292, 1.024072862575109655 ) ) ;
#12286=TOROIDAL_SURFACE ( 'NONE', #33365, 3.683000000000000718, 0.5080000000000000071 ) ;
#12288=CARTESIAN_POINT ( 'NONE',  ( -1.642663419667714564, 119.5945091202099348, 0.5769171603192790876 ) ) ;
#12289=CARTESIAN_POINT ( 'NONE',  ( -4.020893062959163267, -8.947226795047690473, 7.425401991387179379 ) ) ;
#12290=CARTESIAN_POINT ( 'NONE',  ( 9.732298487430668388, 124.2227999206177032, 0.8093454005834664899 ) ) ;
#12291=CARTESIAN_POINT ( 'NONE',  ( 14.92885934485193289, 156.1361208441215922, -0.4494106821051803702 ) ) ;
#12294=CARTESIAN_POINT ( 'NONE',  ( -5.560415744471473687, 116.7072868167284980, -0.2237494900823625843 ) ) ;
#12296=CARTESIAN_POINT ( 'NONE',  ( -4.074955089416341991, 118.2429491485453354, 0.1454234154749719787 ) ) ;
#12297=CARTESIAN_POINT ( 'NONE',  ( -22.83540780336928577, 150.4058779721138421, -0.4563057931615319140 ) ) ;
#12299=CARTESIAN_POINT ( 'NONE',  ( 8.251510532373199425, 120.4738826143435944, -1.099784515884263403 ) ) ;
#12300=CARTESIAN_POINT ( 'NONE',  ( 5.329260751456349254, 104.6144662015457527, 0.2904590649852882289 ) ) ;
#12301=CARTESIAN_POINT ( 'NONE',  ( -10.03827118703590848, 124.8772485319846055, -0.7459150106818384085 ) ) ;
#12303=AXIS2_PLACEMENT_3D ( 'NONE', #21613, #31435, #15241 ) ;
#12304=CARTESIAN_POINT ( 'NONE',  ( 1.797937260761245382, 116.4670535197835051, 0.04904229828524086371 ) ) ;
#12307=CARTESIAN_POINT ( 'NONE',  ( -2.029258473809828711, 23.83235028914373288, 4.157303687431403993 ) ) ;
#12309=CARTESIAN_POINT ( 'NONE',  ( -4.999995268433905515, 117.4036871737256007, 0.8306561334194828561 ) ) ;
#12312=CARTESIAN_POINT ( 'NONE',  ( -7.796775163588184121, 122.5850086010226363, 0.007623726692081094630 ) ) ;
#12313=CARTESIAN_POINT ( 'NONE',  ( -0.8806307086779237014, 20.21867702141905099, 4.540528814573361771 ) ) ;
#12314=CARTESIAN_POINT ( 'NONE',  ( -0.006370369177400351211, 117.0014201992989058, 0.3187993231787207837 ) ) ;
#12315=CARTESIAN_POINT ( 'NONE',  ( -1.644049521069662845, 104.6144662015457243, -4.546677564578934572 ) ) ;
#12316=CARTESIAN_POINT ( 'NONE',  ( 4.799643950526473191, 115.7029491485453292, 1.472414092453835588 ) ) ;
#12317=CARTESIAN_POINT ( 'NONE',  ( 14.20167894085449944, 122.0820592118662091, -1.087754808798858219 ) ) ;
#12318=AXIS2_PLACEMENT_3D ( 'NONE', #21528, #34767, #35188 ) ;
#12319=CARTESIAN_POINT ( 'NONE',  ( -0.01051219832188539718, 119.4384375980492194, 0.5260733902271050866 ) ) ;
#12320=CARTESIAN_POINT ( 'NONE',  ( -3.618988008572157522, 19.14412854911201123, 2.900346660497036044 ) ) ;
#12321=CARTESIAN_POINT ( 'NONE',  ( -22.80589948333492600, 149.4631731099488832, -1.425235564609340422 ) ) ;
#12322=CARTESIAN_POINT ( 'NONE',  ( 0.8777592251401162837, 3.590160258842859164, -0.4283581310676968790 ) ) ;
#12325=CARTESIAN_POINT ( 'NONE',  ( -13.80952258003161148, 150.2278160098252329, 0.4282869786672489076 ) ) ;
#12326=CARTESIAN_POINT ( 'NONE',  ( 5.856266048228023990, -12.49204451700697227, 1.108958003446382845 ) ) ;
#12327=CARTESIAN_POINT ( 'NONE',  ( 4.935370518415115981, 156.1188696671683260, -1.185051001079852062 ) ) ;
#12330=CARTESIAN_POINT ( 'NONE',  ( -4.773031995702506691, 117.8805138891626427, -0.8734539205960981656 ) ) ;
#12332=CARTESIAN_POINT ( 'NONE',  ( 9.538359384048550993, 124.8019839352694476, 0.1905991205270209932 ) ) ;
#12334=CARTESIAN_POINT ( 'NONE',  ( 19.70389350229440595, 149.1964539096042870, 2.489783701940901928 ) ) ;
#12335=FACE_OUTER_BOUND ( 'NONE', #20507, .T. ) ;
#12337=AXIS2_PLACEMENT_3D ( 'NONE', #16874, #26676, #7099 ) ;
#12338=CARTESIAN_POINT ( 'NONE',  ( 4.879798404911957377, 117.5475425101833196, -0.9415396859558378129 ) ) ;
#12339=CARTESIAN_POINT ( 'NONE',  ( 22.60023854264588294, 150.6256779753201158, 0.001684207673827021372 ) ) ;
#12345=CARTESIAN_POINT ( 'NONE',  ( 1.926753168619404377, -15.13879046584015775, 5.903414407318583024 ) ) ;
#12348=CARTESIAN_POINT ( 'NONE',  ( -4.732736203862330626, 117.9644780015066914, 0.6133938389771328437 ) ) ;
#12353=CARTESIAN_POINT ( 'NONE',  ( 3.478480445305584645, 118.6155477304225343, -0.7926535167593043996 ) ) ;
#12354=CARTESIAN_POINT ( 'NONE',  ( -0.1274156416095612032, 105.9117620634264370, -5.326488824310051662 ) ) ;
#12355=CARTESIAN_POINT ( 'NONE',  ( 4.659798553400928078, 118.0075236409115149, 0.7771128701194636168 ) ) ;
#12357=CARTESIAN_POINT ( 'NONE',  ( -6.654617103318593247E-14, 104.6144662015457243, 1.534725424433578570E-31 ) ) ;
#12358=CARTESIAN_POINT ( 'NONE',  ( -0.09221630143787259981, 107.6766875080336376, 4.614880812453306724 ) ) ;
#12359=CARTESIAN_POINT ( 'NONE',  ( -2.070226828232369254, -8.352695179381779411, -4.151654383260235726 ) ) ;
#12362=CARTESIAN_POINT ( 'NONE',  ( 4.842864477130134127, 117.0601473006971105, -0.7870117353683143691 ) ) ;
#12363=CARTESIAN_POINT ( 'NONE',  ( -0.8144440842626328170, 156.8926940187749324, -1.343054762528749890 ) ) ;
#12364=CARTESIAN_POINT ( 'NONE',  ( 5.035933200060415338, 117.3993844219003648, -0.5513780243448201945 ) ) ;
#12365=CARTESIAN_POINT ( 'NONE',  ( -5.997746767061387985, 28.36824686342176349, 0.3198938015187350881 ) ) ;
#12367=CARTESIAN_POINT ( 'NONE',  ( -3.640175008984333882, 11.51306413504884318, -2.862805987297033727 ) ) ;
#12368=CARTESIAN_POINT ( 'NONE',  ( 5.820459347748528245, 117.1115750087645608, 0.4818200784724925301 ) ) ;
#12370=CARTESIAN_POINT ( 'NONE',  ( -2.149574005142933508, 105.1243567940866654, -4.891951615042300361 ) ) ;
#12371=CARTESIAN_POINT ( 'NONE',  ( 3.885732391871624447, -15.29168275415018741, 1.106840230638412192 ) ) ;
#12372=CARTESIAN_POINT ( 'NONE',  ( -1.284628845569858679, 118.8689652838214244, 0.6394392525890020273 ) ) ;
#12374=CARTESIAN_POINT ( 'NONE',  ( -0.3421040304481134942, 19.14286131909006272, 0.9136164113388466346 ) ) ;
#12376=CARTESIAN_POINT ( 'NONE',  ( -0.8667032531718782407, 4.505117207799016477, 0.4606053492026337959 ) ) ;
#12379=ORIENTED_EDGE ( 'NONE', *, *, #26485, .T. ) ;
#12381=CARTESIAN_POINT ( 'NONE',  ( 1.464138133146175580, 108.1711930243730109, 4.389422119207357476 ) ) ;
#12382=CARTESIAN_POINT ( 'NONE',  ( -9.755760200704729712, 153.9716628027005925, 0.9476658408544212930 ) ) ;
#12384=CARTESIAN_POINT ( 'NONE',  ( 3.509037099356659084, -13.47856448578629873, 2.732507022889707038 ) ) ;
#12385=CARTESIAN_POINT ( 'NONE',  ( 17.80491421350291503, 148.0643276405518804, -1.576192721057972923 ) ) ;
#12386=CARTESIAN_POINT ( 'NONE',  ( -17.92333008985184506, 151.7072807693909340, -2.394054079121861633 ) ) ;
#12388=CARTESIAN_POINT ( 'NONE',  ( 8.517627334839968256, 118.9460427874306703, 1.261003614275605367 ) ) ;
#12389=CARTESIAN_POINT ( 'NONE',  ( -4.128276239086840604, 33.50807246189903310, 3.501313855992088442 ) ) ;
#12390=CARTESIAN_POINT ( 'NONE',  ( 0.004910621514677531059, 156.3161161488371533, -0.2457475809811480449 ) ) ;
#12392=CARTESIAN_POINT ( 'NONE',  ( 4.973152232786927307, 117.3993868326352015, 0.9753084504214339923 ) ) ;
#12393=LINE ( 'NONE', #6012, #34668 ) ;
#12394=CARTESIAN_POINT ( 'NONE',  ( 2.958531772299236362, 39.20946620154573736, 1.329372033065076231 ) ) ;
#12397=CARTESIAN_POINT ( 'NONE',  ( -8.202033116754899211, 17.84503447943221843, -1.958624548878737492 ) ) ;
#12398=CARTESIAN_POINT ( 'NONE',  ( 7.898163624196731902, 121.8456834504061845, 1.011533665549599226 ) ) ;
#12400=CARTESIAN_POINT ( 'NONE',  ( 23.29167281398205347, 149.3519930085110161, 0.4396919384238295314 ) ) ;
#12401=CARTESIAN_POINT ( 'NONE',  ( -5.380575101947485450, 117.2069880336854197, 0.6820287515226023389 ) ) ;
#12404=CARTESIAN_POINT ( 'NONE',  ( 2.887663853482148824, 156.0927491134738716, 0.09102753749515629655 ) ) ;
#12405=CARTESIAN_POINT ( 'NONE',  ( 7.819746389599702141, 118.9574329095587757, 1.279815391681077497 ) ) ;
#12406=CARTESIAN_POINT ( 'NONE',  ( -0.5966991250155297966, -8.296908750894687046, 8.413794654835093922 ) ) ;
#12407=CARTESIAN_POINT ( 'NONE',  ( 5.509056870513385995, 117.3456113441247766, -0.6578241769142348927 ) ) ;
#12408=CARTESIAN_POINT ( 'NONE',  ( -0.4230288213599560088, 124.8375573595198063, -0.01946820596077788318 ) ) ;
#12409=CARTESIAN_POINT ( 'NONE',  ( 6.465544251997671132, -12.29036122045927470, 0.5318397859568593233 ) ) ;
#12411=CARTESIAN_POINT ( 'NONE',  ( -3.210878647048973189, -8.553304832117262890, -7.794174491370510438 ) ) ;
#12413=CARTESIAN_POINT ( 'NONE',  ( 1.567127437766292486, 117.9394488752349588, 1.376223268243407682 ) ) ;
#12415=CARTESIAN_POINT ( 'NONE',  ( 3.047145566129288330, -14.72663143740328806, 3.823360744794035870 ) ) ;
#12416=CARTESIAN_POINT ( 'NONE',  ( 0.3827772581120965079, 119.9741034315941732, -0.6590906510345961866 ) ) ;
#12417=CARTESIAN_POINT ( 'NONE',  ( -15.42235106321975735, 121.0727120035890323, 0.2994195231956990888 ) ) ;
#12418=AXIS2_PLACEMENT_3D ( 'NONE', #31986, #35608, #19397 ) ;
#12420=CARTESIAN_POINT ( 'NONE',  ( 5.018852221467176022, 117.3993836729720073, -0.7012530358412483178 ) ) ;
#12422=CARTESIAN_POINT ( 'NONE',  ( -6.060001926025549144E-14, 82.13546620154573930, 9.542986963510498366E-17 ) ) ;
#12423=CARTESIAN_POINT ( 'NONE',  ( 4.954452526664399059, -15.13560178954495505, 4.019779494548574306 ) ) ;
#12424=CARTESIAN_POINT ( 'NONE',  ( -20.18437654629515166, 141.3454246894093274, 1.633934361538418312 ) ) ;
#12425=CARTESIAN_POINT ( 'NONE',  ( 22.09732278473114420, 146.2042277794223537, -1.157738048209832948 ) ) ;
#12426=CARTESIAN_POINT ( 'NONE',  ( 3.263621351691376571, 8.939281053574255509, -3.290156819607050753 ) ) ;
#12431=CARTESIAN_POINT ( 'NONE',  ( -10.90507628433470622, 123.7747955097422476, 1.016219593014794143 ) ) ;
#12433=CARTESIAN_POINT ( 'NONE',  ( 12.09213366837439629, 122.8144071692085504, -1.302296015248258110 ) ) ;
#12434=CARTESIAN_POINT ( 'NONE',  ( -17.69400247866234466, 128.5843929717815115, -1.987683303373968480 ) ) ;
#12437=CARTESIAN_POINT ( 'NONE',  ( 11.01086703061197447, 126.1652090859982707, -0.5547642914263288816 ) ) ;
#12439=CARTESIAN_POINT ( 'NONE',  ( -11.36144155339852446, 123.3954635094115702, -1.633191427152098196 ) ) ;
#12440=CARTESIAN_POINT ( 'NONE',  ( 3.184821769958268600, -15.26663968290864482, 3.758507235160873261 ) ) ;
#12441=CARTESIAN_POINT ( 'NONE',  ( -4.262962905417929882, 118.2124953749421081, -0.5347562978372674136 ) ) ;
#12445=CARTESIAN_POINT ( 'NONE',  ( -4.877607691258805112, 117.6444329028332021, 0.8850603751916138462 ) ) ;
#12446=CARTESIAN_POINT ( 'NONE',  ( 17.14693169618184854, 148.7218176724978775, 2.218585656167708198 ) ) ;
#12448=CARTESIAN_POINT ( 'NONE',  ( -0.8828713250188725548, -8.991384785216279596, -8.412059017423759499 ) ) ;
#12449=CARTESIAN_POINT ( 'NONE',  ( 15.80537369954022608, 146.5893318786020814, 0.6464893008334199331 ) ) ;
#12453=AXIS2_PLACEMENT_3D ( 'NONE', #34677, #28279, #38084 ) ;
#12460=CARTESIAN_POINT ( 'NONE',  ( -21.90070483041515814, 151.4392833230981239, -0.2858324510978370037 ) ) ;
#12463=CARTESIAN_POINT ( 'NONE',  ( 6.931668681496168105, 121.8844402723393188, -0.1473822194997169155 ) ) ;
#12464=CARTESIAN_POINT ( 'NONE',  ( 4.922683227735471512, 117.4111498278341799, -0.9488309096965314993 ) ) ;
#12465=ORIENTED_EDGE ( 'NONE', *, *, #16784, .T. ) ;
#12466=CARTESIAN_POINT ( 'NONE',  ( 2.103206696568210354, 115.7026987777287417, -1.632043270026867221 ) ) ;
#12467=CARTESIAN_POINT ( 'NONE',  ( -9.231158399652327873, 124.2544328994657405, -0.2701740761454695661 ) ) ;
#12468=CARTESIAN_POINT ( 'NONE',  ( 4.651167782940357931, -13.82644354294225408, 4.017274338905189701 ) ) ;
#12469=CARTESIAN_POINT ( 'NONE',  ( -9.191685830660496492, 119.1751624949753534, 0.9473905404949719555 ) ) ;
#12472=CARTESIAN_POINT ( 'NONE',  ( 8.204617290884259617, 117.5299140688306352, 0.3545595769132393049 ) ) ;
#12473=CARTESIAN_POINT ( 'NONE',  ( 15.76801079384962101, 146.5674410900921885, 0.4492571464743756460 ) ) ;
#12474=CARTESIAN_POINT ( 'NONE',  ( 4.789005780339384621, 118.5266822147775940, -0.8321226176749365600 ) ) ;
#12475=CARTESIAN_POINT ( 'NONE',  ( 0.9479787518424646064, 8.937585264489511516, -0.2400550011337005962 ) ) ;
#12476=CARTESIAN_POINT ( 'NONE',  ( -0.8970928355478778871, 116.4604358222411236, -0.08699291512134188498 ) ) ;
#12477=DIRECTION ( 'NONE',  ( -4.017660918040594346E-17, 1.000000000000000000, 2.376309959284834438E-19 ) ) ;
#12479=ORIENTED_EDGE ( 'NONE', *, *, #41725, .T. ) ;
#12480=CARTESIAN_POINT ( 'NONE',  ( -8.748663343918041235, 117.9815668471614600, 0.4028670228981990342 ) ) ;
#12482=CARTESIAN_POINT ( 'NONE',  ( 16.48954130525386574, 125.2933801378020888, 1.785035858276809106 ) ) ;
#12483=CARTESIAN_POINT ( 'NONE',  ( 6.760483308329369834, 119.1290971219625021, -1.000752511853992832 ) ) ;
#12484=CARTESIAN_POINT ( 'NONE',  ( 7.384888961195664514, 14.16877864132934839, -4.050812539764339526 ) ) ;
#12485=CARTESIAN_POINT ( 'NONE',  ( -14.34385702226365922, 155.9958976045614349, -1.592240502911361766 ) ) ;
#12486=CARTESIAN_POINT ( 'NONE',  ( 4.843100780571696795, 117.8277630096203836, -0.6985884806925111157 ) ) ;
#12487=CARTESIAN_POINT ( 'NONE',  ( 5.262805716459999950, 116.4520502601644409, 1.094458988799881682 ) ) ;
#12488=CARTESIAN_POINT ( 'NONE',  ( -14.68196552534010912, 148.8424012017631242, -0.1663232928928549959 ) ) ;
#12489=CARTESIAN_POINT ( 'NONE',  ( -19.20654067994522762, 147.6776069388173767, -2.506343067704080774 ) ) ;
#12490=CARTESIAN_POINT ( 'NONE',  ( 2.438853454531733966, -15.63545089637397112, 5.735818209389550226 ) ) ;
#12492=CARTESIAN_POINT ( 'NONE',  ( -4.689789358878839742, 118.1651005001179158, -0.6093517961627712420 ) ) ;
#12495=CARTESIAN_POINT ( 'NONE',  ( 18.52244049926375880, 148.0519089404264150, 2.440181727699358927 ) ) ;
#12496=CARTESIAN_POINT ( 'NONE',  ( -15.78437780952707215, 146.2378312303354448, -0.3154094333657934679 ) ) ;
#12497=( BOUNDED_SURFACE ( )  B_SPLINE_SURFACE ( 3, 2, ( 
 ( #14535, #4359, #20923 ),
 ( #1362, #27544, #1153 ),
 ( #11138, #36930, #7749 ),
 ( #24334, #33946, #20715 ),
 ( #30522, #8157, #40550 ),
 ( #33739, #11348, #4563 ),
 ( #17522, #14320, #1578 ),
 ( #36654, #33040, #40068 ),
 ( #7055, #3868, #17255 ),
 ( #39857, #23635, #36235 ),
 ( #26850, #4083, #20022 ),
 ( #29627, #7265, #10861 ),
 ( #7477, #26210, #673 ),
 ( #13437, #10446, #13851 ),
 ( #463, #23850, #30247 ),
 ( #32825, #39214, #13642 ),
 ( #16834, #3439, #249 ),
 ( #20226, #6835, #29835 ),
 ( #26634, #30041, #10653 ),
 ( #36870, #23200, #26422 ) ),
 .UNSPECIFIED., .F., .F., .F. ) 
 B_SPLINE_SURFACE_WITH_KNOTS ( ( 4, 2, 2, 2, 2, 2, 2, 2, 2, 4 ),
 ( 3, 3 ),
 ( -7.203168183450570083E-17, 0.0008043714308976360541, 0.001608742861795344099, 0.002413114292693052144, 0.003217485723590760190, 0.004021857154488468235, 0.004826228585386176280, 0.006434971447181592370, 0.009652457170772425418, 0.01286994289436325760 ),
 ( 0.000000000000000000, 1.000000000000000000 ),
 .UNSPECIFIED. ) 
 GEOMETRIC_REPRESENTATION_ITEM ( )  RATIONAL_B_SPLINE_SURFACE ( (
 ( 1.000000000000000000, 0.9815197824473234078, 1.000000000000000000),
 ( 1.000000000000000000, 0.9811723635260756193, 1.000000000000000000),
 ( 1.000000000000000000, 0.9803956462535394767, 1.000000000000000000),
 ( 1.000000000000000000, 0.9775604298910611778, 1.000000000000000000),
 ( 1.000000000000000000, 0.9755054586171506559, 1.000000000000000000),
 ( 1.000000000000000000, 0.9704993482276272898, 1.000000000000000000),
 ( 1.000000000000000000, 0.9675447666325507345, 1.000000000000000000),
 ( 1.000000000000000000, 0.9610561756478790407, 1.000000000000000000),
 ( 1.000000000000000000, 0.9575813355048414799, 1.000000000000000000),
 ( 1.000000000000000000, 0.9503236772853900227, 1.000000000000000000),
 ( 1.000000000000000000, 0.9465499958463368113, 1.000000000000000000),
 ( 1.000000000000000000, 0.9387344193236741852, 1.000000000000000000),
 ( 1.000000000000000000, 0.9346745718249651613, 1.000000000000000000),
 ( 1.000000000000000000, 0.9222609948217221909, 1.000000000000000000),
 ( 1.000000000000000000, 0.9134583146195013326, 1.000000000000000000),
 ( 1.000000000000000000, 0.8860507374704946759, 1.000000000000000000),
 ( 1.000000000000000000, 0.8669451626883383222, 1.000000000000000000),
 ( 1.000000000000000000, 0.8330907799442855977, 1.000000000000000000),
 ( 1.000000000000000000, 0.8189901318545821374, 1.000000000000000000),
 ( 1.000000000000000000, 0.8121911378917013868, 1.000000000000000000) ) ) 
 REPRESENTATION_ITEM ( '' )  SURFACE ( )  );
#12498=CARTESIAN_POINT ( 'NONE',  ( 5.237379388564934679, 115.7029491485453292, 1.024072862575109655 ) ) ;
#12499=AXIS2_PLACEMENT_3D ( 'NONE', #40631, #40429, #21010 ) ;
#12500=CARTESIAN_POINT ( 'NONE',  ( -1.638321535317357025, 108.1711930243730109, 4.327427591587794886 ) ) ;
#12501=CARTESIAN_POINT ( 'NONE',  ( -8.302162399154521921, -10.86525386290528594, -1.555404731216454284 ) ) ;
#12502=CARTESIAN_POINT ( 'NONE',  ( 8.892178686619965688, 123.2307073318660855, 0.7481024605839379227 ) ) ;
#12503=CARTESIAN_POINT ( 'NONE',  ( 22.95957815304923599, 148.8788797244430384, -0.5134943257494377633 ) ) ;
#12505=AXIS2_PLACEMENT_3D ( 'NONE', #6173, #25742, #3394 ) ;
#12507=EDGE_CURVE ( 'NONE', #35669, #10570, #37614, .T. ) ;
#12508=CARTESIAN_POINT ( 'NONE',  ( -20.69909148798433662, 152.5508394022679113, -0.4136171090298727537 ) ) ;
#12510=CARTESIAN_POINT ( 'NONE',  ( 6.495737268896391470, 120.2913924786790147, -0.9109853078430656392 ) ) ;
#12511=CARTESIAN_POINT ( 'NONE',  ( 6.420735782905913958, -13.61083692044810434, 0.4627584258721888499 ) ) ;
#12512=CARTESIAN_POINT ( 'NONE',  ( -6.141611553833193682, 155.3548635187015350, -0.6951709773850850427 ) ) ;
#12513=CARTESIAN_POINT ( 'NONE',  ( 23.21309708346254652, 149.6303025714371131, 0.4895544115752262782 ) ) ;
#12514=ORIENTED_EDGE ( 'NONE', *, *, #20230, .T. ) ;
#12515=CARTESIAN_POINT ( 'NONE',  ( -3.426874451426485724, 1.805113900313119357, -3.130497002818263930 ) ) ;
#12517=CARTESIAN_POINT ( 'NONE',  ( -4.801729350823258358, 117.4006813127757027, 1.015859690946131932 ) ) ;
#12520=CARTESIAN_POINT ( 'NONE',  ( 6.083635286984732993, 120.8261725085448717, 0.8936664544520765974 ) ) ;
#12521=CARTESIAN_POINT ( 'NONE',  ( 0.3943543298815788134, 25.17882533764851871, -4.623353113333005915 ) ) ;
#12522=CARTESIAN_POINT ( 'NONE',  ( 20.09973570640914176, 152.4688535085772685, 1.548630484586873246 ) ) ;
#12524=CARTESIAN_POINT ( 'NONE',  ( 2.274844673354063040, 107.2461735399431717, 4.729530331960789979 ) ) ;
#12525=CARTESIAN_POINT ( 'NONE',  ( 4.984194916311421863, 158.4862278396301178, -1.425929471103634327 ) ) ;
#12526=CARTESIAN_POINT ( 'NONE',  ( -14.27712035414131897, 128.5469532985352714, 1.439506347022430299 ) ) ;
#12527=CARTESIAN_POINT ( 'NONE',  ( 2.854375549615681962, 5.100648791940559867, -3.633247542873777380 ) ) ;
#12528=CARTESIAN_POINT ( 'NONE',  ( -11.39485104697116569, 118.9229013597968247, -0.8408094927682291386 ) ) ;
#12529=CIRCLE ( 'NONE', #35650, 5.588000000000006295 ) ;
#12532=CARTESIAN_POINT ( 'NONE',  ( -9.417214020844317801, 124.0858766813489780, 0.2349654282845520803 ) ) ;
#12533=CARTESIAN_POINT ( 'NONE',  ( 5.593658044048013700, -13.59245692957503060, 2.833247147397068399 ) ) ;
#12536=CARTESIAN_POINT ( 'NONE',  ( -4.605880960340654973, 117.9546811930534744, -0.9428398339839773046 ) ) ;
#12537=ADVANCED_FACE ( 'NONE', ( #29990 ), #23584, .T. ) ;
#12538=CARTESIAN_POINT ( 'NONE',  ( 4.224755116449876446, 155.8535809751167562, 0.04780361979672674566 ) ) ;
#12540=CARTESIAN_POINT ( 'NONE',  ( 12.94126367519703535, 122.7019651155717384, 1.840448779276435909 ) ) ;
#12543=CARTESIAN_POINT ( 'NONE',  ( -13.02773564672695095, 156.9259531928012734, 0.6619068571425155145 ) ) ;
#12544=CARTESIAN_POINT ( 'NONE',  ( 4.980372089298493954, 117.4083386159582005, -0.8694277117261164367 ) ) ;
#12545=CARTESIAN_POINT ( 'NONE',  ( 8.030623918766011116, 158.6806155330135084, -0.07574440115180935962 ) ) ;
#12547=CARTESIAN_POINT ( 'NONE',  ( 5.275990361836080389, 115.6909491485453145, -0.8142983086532559200 ) ) ;
#12549=CARTESIAN_POINT ( 'NONE',  ( 1.853238020027676125, -15.15240415584193023, 5.472168462869254846 ) ) ;
#12553=CARTESIAN_POINT ( 'NONE',  ( -4.515249553929252535, 118.0822497875658712, 0.6203405485297761590 ) ) ;
#12555=ORIENTED_EDGE ( 'NONE', *, *, #19378, .F. ) ;
#12557=CARTESIAN_POINT ( 'NONE',  ( 3.435244954865206868, 118.5730363814739690, -0.7907002124901647555 ) ) ;
#12558=CARTESIAN_POINT ( 'NONE',  ( -4.902456202886120273, 117.5302216577071874, -0.8631654989601054151 ) ) ;
#12559=CARTESIAN_POINT ( 'NONE',  ( 4.605563930170307962, 117.9546322641617309, 0.9429387650545777433 ) ) ;
#12561=CARTESIAN_POINT ( 'NONE',  ( -0.7201697038422463226, 156.4767055779393559, -0.8425024029193185493 ) ) ;
#12562=CARTESIAN_POINT ( 'NONE',  ( -2.609347773700347872, 115.7032548454379253, -1.690797176400070212 ) ) ;
#12565=CARTESIAN_POINT ( 'NONE',  ( 5.344534118436166992, 116.9519127983885340, -0.7428430495679890777 ) ) ;
#12566=CARTESIAN_POINT ( 'NONE',  ( -4.298694136813268507, 120.0471566133196291, -0.8457497992440219381 ) ) ;
#12568=CARTESIAN_POINT ( 'NONE',  ( 23.36555825341164550, 148.7788340588663800, 0.4668994608413311043 ) ) ;
#12571=CARTESIAN_POINT ( 'NONE',  ( -4.274281473441157608, 3.541781053574249327, 1.790774723582081451 ) ) ;
#12572=CARTESIAN_POINT ( 'NONE',  ( 21.60506836338281644, 151.3813297165527274, 1.270904734852022600 ) ) ;
#12574=CARTESIAN_POINT ( 'NONE',  ( -1.039979636890616455, 104.6144662015457527, -4.722350110998245754 ) ) ;
#12575=CARTESIAN_POINT ( 'NONE',  ( 2.733372102295486439, -15.34075898222114809, 4.536119796583970576 ) ) ;
#12576=CARTESIAN_POINT ( 'NONE',  ( -10.65007529713519929, 155.7851685111067184, 1.746298732392691511 ) ) ;
#12577=CARTESIAN_POINT ( 'NONE',  ( -0.5432096421966324806, 25.39095905668347797, -0.8082079942862561150 ) ) ;
#12578=CARTESIAN_POINT ( 'NONE',  ( 0.8800754956866637668, -0.3565347152210476267, -0.4212773433312864690 ) ) ;
#12581=CARTESIAN_POINT ( 'NONE',  ( 3.333432127168501680, 112.1633951907056996, 2.855042910325920946 ) ) ;
#12583=CARTESIAN_POINT ( 'NONE',  ( -12.52894620082573773, 152.0704867801853766, 0.9584603128924423787 ) ) ;
#12584=CARTESIAN_POINT ( 'NONE',  ( 3.174366308151880922, 91.02546620154572565, 0.06343139340882768262 ) ) ;
#12585=CARTESIAN_POINT ( 'NONE',  ( 3.093634585129180881, -14.37226628243755400, 4.703574289890697813 ) ) ;
#12586=CARTESIAN_POINT ( 'NONE',  ( 8.228482648312512637, 121.2453320564195280, -0.9666412201339348309 ) ) ;
#12587=CARTESIAN_POINT ( 'NONE',  ( -19.79373099999713403, 147.4002846799066333, -2.520905760949471386 ) ) ;
#12589=CARTESIAN_POINT ( 'NONE',  ( 7.967454197907589908, 121.6427856937929022, 1.120273065806566271 ) ) ;
#12590=CARTESIAN_POINT ( 'NONE',  ( -5.095652749712312080, 31.83908346630384756, 0.3959475160674749139 ) ) ;
#12592=CARTESIAN_POINT ( 'NONE',  ( 14.72002613302106866, 148.8393470518043955, -0.03138755845351924589 ) ) ;
#12599=CARTESIAN_POINT ( 'NONE',  ( -1.011143250135940530, 20.41458852336931074, 8.389224627043086358 ) ) ;
#12600=CARTESIAN_POINT ( 'NONE',  ( 0.7201697038421175368, 156.4767055779393559, 0.8425024029193187713 ) ) ;
#12601=CARTESIAN_POINT ( 'NONE',  ( 3.174366308151880478, 104.1064662015457287, 0.06343139340882768262 ) ) ;
#12602=CARTESIAN_POINT ( 'NONE',  ( 23.21350185287833767, 149.6290410902582551, 0.3868015801638794993 ) ) ;
#12603=CARTESIAN_POINT ( 'NONE',  ( -5.344534118436294889, 116.9519127983885340, 0.7428430495679891887 ) ) ;
#12605=CARTESIAN_POINT ( 'NONE',  ( 7.552512487614144732, 122.4261604937442485, 0.1509171734833088807 ) ) ;
#12606=CARTESIAN_POINT ( 'NONE',  ( 16.61465421735657699, 153.6190162071354735, 2.198628343207905900 ) ) ;
#12607=AXIS2_PLACEMENT_3D ( 'NONE', #17620, #15050, #30829 ) ;
#12608=CARTESIAN_POINT ( 'NONE',  ( -8.215080244096204964, -10.21703095211954704, 2.011605797521776928 ) ) ;
#12609=CARTESIAN_POINT ( 'NONE',  ( -5.487573023729679811, 117.1580262016726692, -0.7772556852123772009 ) ) ;
#12610=CARTESIAN_POINT ( 'NONE',  ( -0.9570916872346277859, 123.2612876230388395, -0.1732974146428331030 ) ) ;
#12613=CARTESIAN_POINT ( 'NONE',  ( 3.486869749996455603, 104.6144662015456674, 3.351517260060684844 ) ) ;
#12614=CARTESIAN_POINT ( 'NONE',  ( -2.857158067608712493, -4.877720491018326499, 7.942258620001617864 ) ) ;
#12615=DIRECTION ( 'NONE',  ( -0.9998004120163608288, -4.016384292689131511E-17, -0.01997839162482749342 ) ) ;
#12617=CARTESIAN_POINT ( 'NONE',  ( 2.829627719599027369, -13.65247383265987757, 0.5238048331051645690 ) ) ;
#12618=CARTESIAN_POINT ( 'NONE',  ( 0.5876368209472652149, 111.1955024190080223, -3.248215591009249170 ) ) ;
#12619=CARTESIAN_POINT ( 'NONE',  ( -7.877688851764539812, 158.6543443936584481, 0.4710593659051899307 ) ) ;
#12624=CARTESIAN_POINT ( 'NONE',  ( 2.911953930276938607, -15.74143402046077078, 5.333341296191352221 ) ) ;
#12625=CARTESIAN_POINT ( 'NONE',  ( -7.786520497867201129, 119.2688035297948659, 1.033142384104571265 ) ) ;
#12626=CARTESIAN_POINT ( 'NONE',  ( 0.008945125900376662068, 117.5133074443058945, -0.4476506782301716836 ) ) ;
#12627=CARTESIAN_POINT ( 'NONE',  ( 0.7336086519982951692, 0.2932837538699786251, -4.563195415240439701 ) ) ;
#12629=ADVANCED_FACE ( 'NONE', ( #31239 ), #37777, .F. ) ;
#12632=CARTESIAN_POINT ( 'NONE',  ( 0.4230288213598272229, 124.8375573595198063, 0.01946820596077801155 ) ) ;
#12633=DIRECTION ( 'NONE',  ( 0.9997969816188602143, 0.0004114442613071361528, 0.02014512991857449892 ) ) ;
#12634=B_SPLINE_SURFACE_WITH_KNOTS ( 'NONE', 3, 3, ( 
 ( #20874, #24081, #33481, #1106, #10465, #27077, #13662, #33898, #11301, #30682, #17477, #23434, #40085, #7282, #36887, #21083, #7705, #27286, #20668, #40300, #1530, #27499, #24285, #37290, #34108, #20244, #41123, #8742, #1943, #21703, #12358, #34318, #8952, #14694 ),
 ( #21918, #15110, #38137, #34948, #18101, #14902, #27905, #31307, #41550, #28113, #5772, #2579, #28542, #15541, #18726, #40707, #27699, #34728, #25345, #31736, #5559, #25134, #40912, #38348, #1736, #11503, #2151, #12142, #24489, #9166, #31521, #22122, #37494, #8318 ),
 ( #18515, #4934, #24704, #31104, #34525, #17893, #11929, #11717, #24921, #28331, #37710, #30896, #8533, #2365, #21289, #21493, #41339, #5351, #15324, #5147, #18305, #37918, #8246, #11864, #24852, #37642, #34451, #17823, #2297, #2079, #24420, #21633, #25275, #15043 ),
 ( #11647, #1871, #5284, #31669, #31453, #18447, #5487, #34659, #15257, #1668, #28476, #28045, #5706, #30822, #41480, #12288, #14623, #25060, #34038, #18234, #31236, #8467, #40638, #41054, #38280, #27626, #37849, #11432, #37425, #31030, #21845, #8672, #28260, #41267 ),
 ( #21218, #12073, #34247, #38064, #8881, #34873, #18663, #40845, #21423, #2510, #15473, #9098, #14833, #4866, #5078, #18028, #27837, #24632, #32514, #12910, #9308, #3345, #369, #19087, #3131, #13335, #6744, #9926, #22270, #15677, #35090, #16092, #26324, #35294 ),
 ( #35505, #29315, #13126, #25695, #25492, #16311, #35719, #38701, #38489, #2925, #32090, #19712, #22895, #22476, #32732, #3563, #41690, #26117, #32301, #39120, #35932, #6121, #15887, #28891, #6324, #16524, #41905, #29532, #12500, #5913, #12705, #39330, #9508, #22064 ),
 ( #25902, #18875, #31882, #38907, #157, #19295, #2720, #28681, #29098, #42117, #9720, #22685, #6527, #19503, #37532, #3775, #16734, #1773, #21118, #29738, #14309, #14733, #27945, #27735, #14943, #33731, #40746, #24527, #1981, #10136, #24325, #33938, #19930, #40542 ),
 ( #7946, #4971, #7739, #1352, #34353, #27109, #30717, #1569, #27322, #11129, #36144, #34144, #20915, #579, #11337, #23108, #4766, #8357, #40335, #24116, #6959, #14525, #21325, #37124, #17718, #32947, #14111, #18137, #5185, #30512, #11543, #23904, #27535, #40121 ),
 ( #31142, #10915, #37331, #8147, #17929, #36921, #30934, #20705, #4554, #17514, #24746, #2196, #37963, #28793, #41381, #12401, #12187, #25392, #25180, #2826, #18984, #38181, #25590, #8995, #6021, #31988, #2408, #15154, #35194, #38394, #15369, #28158, #21746, #8788 ),
 ( #41164, #15785, #8572, #9206, #31780, #11970, #22164, #19193, #34772, #21963, #32200, #38597, #41806, #24962, #34565, #34993, #12603, #9404, #22370, #35394, #6223, #5392, #21533, #2620, #3034, #15990, #15580, #40953, #5605, #11758, #37748, #18347, #5814, #31353 ),
 ( #18561, #31567, #28374, #18770, #28585, #41593, #32830, #33045, #6637, #43, #16410, #13649, #36030, #13009, #10029, #10238, #19603, #20027, #26002, #29632, #38799, #39012, #23207, #9821, #470, #26640, #26430, #33258, #39647, #36242, #20233, #6426, #22787, #35611 ),
 ( #32406, #35823, #7062, #28991, #3236, #32615, #3447, #29416, #256, #10452, #39434, #13442, #3876, #16625, #16840, #9611, #23423, #39221, #679, #12803, #36451, #7271, #25794, #29840, #42006, #13232, #26215, #23001, #19399, #6842, #4088, #22579, #19813, #16195 ) ),
 .UNSPECIFIED., .F., .F., .F.,
 ( 4, 1, 1, 1, 1, 1, 3, 4 ),
 ( 4, 1, 1, 1, 1, 1, 1, 1, 1, 1, 1, 1, 1, 1, 1, 1, 1, 1, 1, 2, 1, 1, 1, 1, 1, 1, 1, 1, 1, 1, 4 ),
 ( 0.000000000000000000, 0.1666666666666666574, 0.2500000000000000000, 0.5000000000000000000, 0.5555555555555555802, 0.7500000000000000000, 1.000000000000000000, 1.010000000000000009 ),
 ( 0.000000000000000000, 0.02126250000000000015, 0.04252500000000000030, 0.06378749999999999698, 0.08505000000000000060, 0.1063125000000000042, 0.1275749999999999940, 0.1488374999999999837, 0.1701000000000000012, 0.1913624999999999909, 0.2126250000000000084, 0.2338874999999999704, 0.2551500000000000434, 0.2764124999999999499, 0.2870437499999999864, 0.2976749999999999674, 0.3083062500000000039, 0.3189375000000000404, 0.3295687499999999659, 0.3402000000000000024, 0.4226750000000000229, 0.5051499999999999879, 0.5876249999999998419, 0.6700999999999999179, 0.7525749999999999940, 0.7938125000000000320, 0.8350499999999999590, 0.8762874999999994419, 0.9175249999999994799, 0.9587624999999999620, 1.000000000000000000 ),
 .UNSPECIFIED. ) ;
#12635=CARTESIAN_POINT ( 'NONE',  ( -4.353257824593281811, 120.2039194668847699, 0.6262808803686856773 ) ) ;
#12637=CARTESIAN_POINT ( 'NONE',  ( 4.214263934994704641, 119.2415290214368042, -0.8241011934941718797 ) ) ;
#12638=CARTESIAN_POINT ( 'NONE',  ( 0.01051220311279016210, 117.9844940561907265, -0.5260736299896250356 ) ) ;
#12641=CARTESIAN_POINT ( 'NONE',  ( 16.04013775433281097, 147.3640369757652877, -0.6457813799431216806 ) ) ;
#12642=TOROIDAL_SURFACE ( 'NONE', #33727, 3.683000000000000718, 0.5080000000000000071 ) ;
#12644=CARTESIAN_POINT ( 'NONE',  ( -17.32761985034188967, 148.7932787949812905, -2.272318092294528746 ) ) ;
#12645=CARTESIAN_POINT ( 'NONE',  ( 3.509229686425914707, -14.99732357267335914, 1.369000748440630799 ) ) ;
#12646=FACE_OUTER_BOUND ( 'NONE', #24442, .T. ) ;
#12647=EDGE_CURVE ( 'NONE', #34334, #27898, #27401, .T. ) ;
#12650=CARTESIAN_POINT ( 'NONE',  ( -4.946322907344598896, 117.6258885912828447, 0.7621993455528004446 ) ) ;
#12651=CARTESIAN_POINT ( 'NONE',  ( 15.64494829320024749, 134.9797526104055123, 2.135645317121837916 ) ) ;
#12652=CARTESIAN_POINT ( 'NONE',  ( 0.4746723515649934888, 24.68197512780947278, 4.609222710213416896 ) ) ;
#12653=CARTESIAN_POINT ( 'NONE',  ( 9.153275543502777722, 153.8946005065304803, 0.4698995960908564640 ) ) ;
#12664=CARTESIAN_POINT ( 'NONE',  ( -10.78032506485383735, 157.9328640892066460, 0.04097195671286549268 ) ) ;
#12665=AXIS2_PLACEMENT_3D ( 'NONE', #31757, #41144, #38370 ) ;
#12668=CARTESIAN_POINT ( 'NONE',  ( -6.001478514085576421, 121.4367562474741504, -0.1909425338979525433 ) ) ;
#12670=EDGE_LOOP ( 'NONE', ( #35770, #6614, #12379 ) ) ;
#12671=CARTESIAN_POINT ( 'NONE',  ( 2.827719281018770126, 115.7033332903982199, -1.571166250493931216 ) ) ;
#12672=CARTESIAN_POINT ( 'NONE',  ( -8.534567384671404966, 123.3353292868209365, -0.2519373819028135619 ) ) ;
#12673=CARTESIAN_POINT ( 'NONE',  ( 6.341500637990160172, -13.03620802017263536, 0.6512942508830525945 ) ) ;
#12674=CARTESIAN_POINT ( 'NONE',  ( -21.17434475962611629, 141.7209635633906259, 1.395834004474946877 ) ) ;
#12676=CARTESIAN_POINT ( 'NONE',  ( 22.64163882069503231, 150.6401102206664291, 0.6810593374908546771 ) ) ;
#12677=CARTESIAN_POINT ( 'NONE',  ( 6.510425706326285145, 121.7797257153627015, 0.2058816303559638794 ) ) ;
#12678=CARTESIAN_POINT ( 'NONE',  ( -3.174366308152012373, 71.97546620154574271, -0.06343139340882732180 ) ) ;
#12679=CARTESIAN_POINT ( 'NONE',  ( 0.5714185265493636479, 16.70905722793067838, 0.7929698740637279863 ) ) ;
#12680=CARTESIAN_POINT ( 'NONE',  ( -16.05840932322207948, 121.2308719818149712, -0.4813400273897940895 ) ) ;
#12684=CARTESIAN_POINT ( 'NONE',  ( -8.664938106414361130, 118.4189509008067205, 0.7014074343780984933 ) ) ;
#12687=CARTESIAN_POINT ( 'NONE',  ( 3.992970410919064683, 117.9114980025989752, 0.8736511219775318082 ) ) ;
#12688=CARTESIAN_POINT ( 'NONE',  ( 8.870548826841499590, 119.8693228481767932, -1.115469810106635373 ) ) ;
#12689=CARTESIAN_POINT ( 'NONE',  ( 6.778223571145144177, 14.38247674671404752, -5.057098040585858989 ) ) ;
#12690=CARTESIAN_POINT ( 'NONE',  ( -13.61640385012406718, 120.8017016962898396, -1.366196570323218173 ) ) ;
#12691=CARTESIAN_POINT ( 'NONE',  ( 4.640660607179467156, 117.9806668035938486, -0.7264285073009650873 ) ) ;
#12693=CARTESIAN_POINT ( 'NONE',  ( -15.26897697690612077, 148.0131224598485744, -0.1773810520481277353 ) ) ;
#12694=CARTESIAN_POINT ( 'NONE',  ( -16.55752258724323056, 151.1890201267100906, -2.396410905537823766 ) ) ;
#12696=CARTESIAN_POINT ( 'NONE',  ( 6.000997576644805598, -14.76005184138509740, 0.6970346396957283197 ) ) ;
#12697=CARTESIAN_POINT ( 'NONE',  ( 4.973583767373020770, 117.3966162183443203, 0.9753880922370259388 ) ) ;
#12702=CARTESIAN_POINT ( 'NONE',  ( 17.69102400252380392, 149.9241642446907292, 2.437100891716216022 ) ) ;
#12705=CARTESIAN_POINT ( 'NONE',  ( -0.9873284109327559177, 106.8474934270474392, 4.901623504225490535 ) ) ;
#12706=CARTESIAN_POINT ( 'NONE',  ( -5.323917895073306816, 23.39377214425099893, 6.572471397932490689 ) ) ;
#12707=CARTESIAN_POINT ( 'NONE',  ( 15.03094698176517063, 148.9283877096812034, 1.255086756411656346 ) ) ;
#12709=CARTESIAN_POINT ( 'NONE',  ( 20.24728863611164442, 152.4988772720997190, -0.6427007754482428892 ) ) ;
#12710=CARTESIAN_POINT ( 'NONE',  ( -4.981086618571428204, 117.5220611846079919, -0.8176168157337386777 ) ) ;
#12712=CARTESIAN_POINT ( 'NONE',  ( -6.900242392319385409, 117.1694300671557727, -0.09431812980450667017 ) ) ;
#12714=CARTESIAN_POINT ( 'NONE',  ( 8.255333662909492887, 120.4554161523990103, -1.101604304946436352 ) ) ;
#12715=CARTESIAN_POINT ( 'NONE',  ( 5.122005163076088330, -14.79606521185782420, 3.940588708504694004 ) ) ;
#12716=CARTESIAN_POINT ( 'NONE',  ( -9.525206088249191794, 124.2661852542617709, -0.6183897905712307796 ) ) ;
#12718=CARTESIAN_POINT ( 'NONE',  ( 22.83540780336915432, 150.4058779721138421, 0.4563057931615321361 ) ) ;
#12720=CARTESIAN_POINT ( 'NONE',  ( 0.3994026957563919789, 5.465888722076803319, 4.619092260001838923 ) ) ;
#12722=CARTESIAN_POINT ( 'NONE',  ( -5.000152259933599019, 117.4026936823171354, 0.8307266032655276078 ) ) ;
#12724=AXIS2_PLACEMENT_3D ( 'NONE', #110, #35886, #6696 ) ;
#12725=CARTESIAN_POINT ( 'NONE',  ( -4.580899860306842264, 27.87760619330545708, 0.5121266511161914892 ) ) ;
#12726=CARTESIAN_POINT ( 'NONE',  ( -6.910925206761728390, 120.7147707202812938, 0.8460832644243309053 ) ) ;
#12727=CARTESIAN_POINT ( 'NONE',  ( -0.5165578309945342284, 6.287656885725535716, -4.620190224396742984 ) ) ;
#12728=CARTESIAN_POINT ( 'NONE',  ( 0.3562832388056000332, 117.2097358735305050, 0.4069867078728328091 ) ) ;
#12731=CARTESIAN_POINT ( 'NONE',  ( 3.126689565637636115, 118.0390668470448929, -0.7034308075613265876 ) ) ;
#12732=CARTESIAN_POINT ( 'NONE',  ( 0.02375515148176195884, 10.92298121479113426, 4.626086752085273979 ) ) ;
#12733=CARTESIAN_POINT ( 'NONE',  ( -0.9824256172936188802, 116.9078805053781025, -0.3575799159885130196 ) ) ;
#12735=CARTESIAN_POINT ( 'NONE',  ( -14.56142545302310332, 139.1552669279217298, 0.4455586761712632127 ) ) ;
#12736=CARTESIAN_POINT ( 'NONE',  ( 3.788645186935202691, -14.89109417362534415, 5.282457547420531974 ) ) ;
#12737=B_SPLINE_CURVE_WITH_KNOTS ( 'NONE', 3,
 ( #12922, #9520, #25913, #168, #3141, #23117, #15898, #19514, #6753, #3786, #22698 ),
 .UNSPECIFIED., .F., .F.,
 ( 4, 1, 1, 1, 1, 1, 1, 1, 4 ),
 ( 0.000000000000000000, 0.1249999999999979600, 0.2500000000000013878, 0.3749999999999938383, 0.4999999999999972800, 0.6249999999999980016, 0.7499999999999986677, 0.8749999999999993339, 1.000000000000000000 ),
 .UNSPECIFIED. ) ;
#12738=CARTESIAN_POINT ( 'NONE',  ( -4.825036788391023457, 62.83146620154573014, -0.09641571798141691796 ) ) ;
#12740=CARTESIAN_POINT ( 'NONE',  ( -4.603470251916389699, 118.0397685500664977, -0.8063307618835234836 ) ) ;
#12741=CARTESIAN_POINT ( 'NONE',  ( 15.76285804746341235, 145.9067145067653541, 0.3149794173055769919 ) ) ;
#12743=VERTEX_POINT ( 'NONE', #36282 ) ;
#12744=CARTESIAN_POINT ( 'NONE',  ( 17.39176377602785095, 131.6241255656270255, 2.296140998891703866 ) ) ;
#12745=CARTESIAN_POINT ( 'NONE',  ( 3.009276887026297587, 50.13146620154573441, -1.210121013456480599 ) ) ;
#12747=CARTESIAN_POINT ( 'NONE',  ( -21.72212103179845855, 136.7703657609320658, 0.7093728523935391994 ) ) ;
#12748=CARTESIAN_POINT ( 'NONE',  ( 4.791775023904364161, 117.5371554061328396, -0.9879116434822770021 ) ) ;
#12750=CARTESIAN_POINT ( 'NONE',  ( 0.003746264460233156724, 116.6481217037470373, -0.1874783927187336774 ) ) ;
#12754=CARTESIAN_POINT ( 'NONE',  ( 1.846504947182619372, -15.27658449339085145, 5.385181725049428714 ) ) ;
#12757=CARTESIAN_POINT ( 'NONE',  ( -4.532961034026489422, 118.0666435962141776, 0.6407912481266496707 ) ) ;
#12760=CARTESIAN_POINT ( 'NONE',  ( 5.988741557545202987, 119.1892980795774122, -1.027262291578486808 ) ) ;
#12761=CARTESIAN_POINT ( 'NONE',  ( -5.366896802164640157, 117.1940586887245388, -0.8977625253398613392 ) ) ;
#12762=CARTESIAN_POINT ( 'NONE',  ( 4.700517274211256868, 117.9669807353441229, 0.8083373127690804960 ) ) ;
#12763=CARTESIAN_POINT ( 'NONE',  ( 3.162461164278121739, -14.57801340048104777, 3.369881103115548893 ) ) ;
#12764=CARTESIAN_POINT ( 'NONE',  ( -8.359771539777545613, 154.6912814427390970, -1.273680951853116916 ) ) ;
#12768=CARTESIAN_POINT ( 'NONE',  ( 3.079207415998468811, 107.8364052097302306, -4.350788137014372836 ) ) ;
#12769=CARTESIAN_POINT ( 'NONE',  ( -11.62460634082118283, 124.4569610989641859, -1.598101315089358154 ) ) ;
#12770=CARTESIAN_POINT ( 'NONE',  ( 15.56076557484939116, 120.7233670659557419, 0.3109411287493940024 ) ) ;
#12771=CARTESIAN_POINT ( 'NONE',  ( -0.004910662370487326248, 159.5928157220454295, 0.2457496255665023166 ) ) ;
#12773=CARTESIAN_POINT ( 'NONE',  ( -4.609222696788063622, 3.091975128091568159, 0.4746723485708761459 ) ) ;
#12774=CARTESIAN_POINT ( 'NONE',  ( 22.89058624538201059, 149.8162411397050278, 1.183733681586531139 ) ) ;
#12776=CARTESIAN_POINT ( 'NONE',  ( 5.314256983242547250, 105.1224655745845524, -0.4585143439917250818 ) ) ;
#12777=CARTESIAN_POINT ( 'NONE',  ( 3.848634119772940565, -15.36481979860233871, 1.996958912074897396 ) ) ;
#12778=CARTESIAN_POINT ( 'NONE',  ( -5.879203592408529744, 119.4106843418347950, 0.9594678464101260573 ) ) ;
#12779=CARTESIAN_POINT ( 'NONE',  ( 0.5559618826558695437, 1.427253112428326753, 0.7990736944121461516 ) ) ;
#12780=CARTESIAN_POINT ( 'NONE',  ( 0.6613080194379835630, -2.301230296243127693, 0.7179688673762391060 ) ) ;
#12785=CARTESIAN_POINT ( 'NONE',  ( 4.012272795662530811, 117.4230540797109938, 0.9751040681224721896 ) ) ;
#12786=CARTESIAN_POINT ( 'NONE',  ( -14.10444703556382784, 134.4521314832425389, 0.9547003412267364153 ) ) ;
#12787=CARTESIAN_POINT ( 'NONE',  ( 3.944052607038018632, -12.86033490357471543, 2.408110524499547100 ) ) ;
#12788=CARTESIAN_POINT ( 'NONE',  ( 11.89126842552443719, 124.3826620800890339, -1.187748846906861777 ) ) ;
#12789=CARTESIAN_POINT ( 'NONE',  ( -18.52749500581566622, 150.2488615152233820, -2.471439233876493002 ) ) ;
#12792=CARTESIAN_POINT ( 'NONE',  ( 8.264950646253613087, 120.1599520239500549, 1.449220757049815678 ) ) ;
#12793=CARTESIAN_POINT ( 'NONE',  ( -5.333451871256411181, 31.98409668703959596, 0.9349438309233621958 ) ) ;
#12794=CARTESIAN_POINT ( 'NONE',  ( 7.056912283644645179, 122.0434499869739540, -0.04958421841494434906 ) ) ;
#12795=ORIENTED_EDGE ( 'NONE', *, *, #21417, .F. ) ;
#12796=DIRECTION ( 'NONE',  ( 0.9998004120163609398, 0.000000000000000000, 0.01997839162482749342 ) ) ;
#12797=CARTESIAN_POINT ( 'NONE',  ( -6.437058721807690810E-14, 62.83146620154573014, 4.519164521849267879E-29 ) ) ;
#12800=CARTESIAN_POINT ( 'NONE',  ( 9.631798221454305420, 123.4354624054469980, 1.070950170652381406 ) ) ;
#12801=CARTESIAN_POINT ( 'NONE',  ( -6.682056005205734733E-14, 110.9644662015457328, 1.123945309419055369E-18 ) ) ;
#12802=CARTESIAN_POINT ( 'NONE',  ( 23.41930689910511276, 142.8308675865925181, 0.4425677471174261357 ) ) ;
#12803=CARTESIAN_POINT ( 'NONE',  ( -5.287753629968840130, 116.2229785614576798, 0.9666386099593878845 ) ) ;
#12806=CARTESIAN_POINT ( 'NONE',  ( -1.409143871925768288, 33.49361554382132766, 0.6725023500899659501 ) ) ;
#12807=CARTESIAN_POINT ( 'NONE',  ( 13.72122979561076228, 121.8522644830672590, 1.670245716993636664 ) ) ;
#12808=EDGE_CURVE ( 'NONE', #909, #14618, #25858, .T. ) ;
#12809=CARTESIAN_POINT ( 'NONE',  ( -0.5507456681092424144, 15.89564879194059799, -4.587442282481805300 ) ) ;
#12810=CARTESIAN_POINT ( 'NONE',  ( 2.619848522501802446, -13.46771402114085703, -8.002427727062926266 ) ) ;
#12811=CARTESIAN_POINT ( 'NONE',  ( -8.726771976265984776, 117.9763464038613279, -0.7462392337901883055 ) ) ;
#12812=CARTESIAN_POINT ( 'NONE',  ( -0.7402556297412126174, 119.5055576915191580, -0.7321893670752777084 ) ) ;
#12816=CARTESIAN_POINT ( 'NONE',  ( -2.261344858989663642, 104.6144662015478701, 4.834083701540023092 ) ) ;
#12817=CARTESIAN_POINT ( 'NONE',  ( 0.1710433496020407063, 14.98650505531991506, 4.637963194678765610 ) ) ;
#12818=CARTESIAN_POINT ( 'NONE',  ( 4.771326357444911181, 117.9394488565474859, 1.118182396071486506 ) ) ;
#12820=CARTESIAN_POINT ( 'NONE',  ( 2.906309357581933650, -13.72804873580029472, 0.7610837935892840189 ) ) ;
#12822=CARTESIAN_POINT ( 'NONE',  ( 0.8718816746734422418, 108.7514562038770976, -4.146788293844217321 ) ) ;
#12823=CARTESIAN_POINT ( 'NONE',  ( -1.919474982883727199, 116.7789519286944966, 0.2705014076049042648 ) ) ;
#12824=ORIENTED_EDGE ( 'NONE', *, *, #14746, .T. ) ;
#12828=CARTESIAN_POINT ( 'NONE',  ( 5.825557336981400880, -14.92341722037543406, 1.564612827344095569 ) ) ;
#12829=CARTESIAN_POINT ( 'NONE',  ( -13.44120003175033595, 122.0388263298542739, 1.206224284286116832 ) ) ;
#12830=CARTESIAN_POINT ( 'NONE',  ( 4.918710253154888967, 117.7409041207840090, -0.6764595669667287092 ) ) ;
#12831=ADVANCED_FACE ( 'NONE', ( #29760 ), #25207, .F. ) ;
#12832=CARTESIAN_POINT ( 'NONE',  ( 4.224370802630715183, -2.505441902618962935, 1.893578447770203566 ) ) ;
#12836=CARTESIAN_POINT ( 'NONE',  ( 0.3568539549765675778, 120.5507043431651510, 0.5637235919965009057 ) ) ;
#12837=CARTESIAN_POINT ( 'NONE',  ( -4.647465358394767598, 117.9312056069267669, 0.7793557571712189658 ) ) ;
#12838=CARTESIAN_POINT ( 'NONE',  ( -0.5597765207468382576, 119.9180165495073283, 0.4599786748625145361 ) ) ;
#12839=DIRECTION ( 'NONE',  ( -4.017660918040594346E-17, 1.000000000000000000, 2.376309959284834438E-19 ) ) ;
#12841=CARTESIAN_POINT ( 'NONE',  ( 11.72911894083922668, 122.8035986606355152, -1.269020613264101982 ) ) ;
#12843=CARTESIAN_POINT ( 'NONE',  ( -5.843718602766688086, 118.4234969239897453, -1.100938688348692018 ) ) ;
#12846=CARTESIAN_POINT ( 'NONE',  ( 4.596726809479003251, 118.0790520653858806, -0.5325700990769507426 ) ) ;
#12847=CARTESIAN_POINT ( 'NONE',  ( 2.723409340394662870, 120.7183352303693340, -0.2545450062501626309 ) ) ;
#12849=CARTESIAN_POINT ( 'NONE',  ( -11.09706570755290578, 123.3376105302527037, -1.576947150105312279 ) ) ;
#12850=CARTESIAN_POINT ( 'NONE',  ( 2.381491173306826248, -15.37068253093559811, 4.932168965620852497 ) ) ;
#12851=CARTESIAN_POINT ( 'NONE',  ( -2.738177118692914025, 105.1243822654267177, -4.587785415214179707 ) ) ;
#12853=CARTESIAN_POINT ( 'NONE',  ( -4.841216625639615856, 117.7365175972573610, 0.8492818512291455679 ) ) ;
#12854=CARTESIAN_POINT ( 'NONE',  ( 8.045112435069260215, 121.5393406094847819, 1.176871282714906375 ) ) ;
#12856=CARTESIAN_POINT ( 'NONE',  ( -1.648064503646425649, 29.87956589480163316, -4.325937074807028715 ) ) ;
#12857=CARTESIAN_POINT ( 'NONE',  ( 1.577167647222550650, 156.2580631240469415, 0.1709568888171393575 ) ) ;
#12859=ADVANCED_FACE ( 'NONE', ( #4266 ), #24847, .T. ) ;
#12863=CARTESIAN_POINT ( 'NONE',  ( -0.7152400940742318358, 118.1588900943969520, 0.8748708461251418766 ) ) ;
#12867=CARTESIAN_POINT ( 'NONE',  ( 3.456281358658134906, 50.63946620154572997, 1.847419665314800064 ) ) ;
#12870=CARTESIAN_POINT ( 'NONE',  ( -0.9174821693852864835, 116.5216256635990391, 0.1124321123350598417 ) ) ;
#12871=ORIENTED_EDGE ( 'NONE', *, *, #17483, .T. ) ;
#12873=CARTESIAN_POINT ( 'NONE',  ( 6.033788598149758542, 121.4449637489673677, 0.07283107479205253032 ) ) ;
#12876=CARTESIAN_POINT ( 'NONE',  ( 2.277049499775069652, 115.7026830795285690, -1.618583747791560778 ) ) ;
#12877=CARTESIAN_POINT ( 'NONE',  ( -15.52804360843209253, 147.5314071815517138, -0.4383331365498628340 ) ) ;
#12878=CARTESIAN_POINT ( 'NONE',  ( 3.788645186935202691, -14.89109417362534415, 5.282457547420531974 ) ) ;
#12879=CARTESIAN_POINT ( 'NONE',  ( -5.881556420379579819, 118.2031694463412634, 0.8113220510518369677 ) ) ;
#12881=CARTESIAN_POINT ( 'NONE',  ( 16.82892344227259329, 155.2408147041404050, 0.5439083615366223645 ) ) ;
#12883=CARTESIAN_POINT ( 'NONE',  ( 15.71945467201891766, 145.6824202290839025, 0.4486337225308515975 ) ) ;
#12884=CARTESIAN_POINT ( 'NONE',  ( 5.276629905794020026, 115.6909491485453145, -0.8098420342951175854 ) ) ;
#12885=CARTESIAN_POINT ( 'NONE',  ( 0.4552753346810295421, 10.21665217803766268, -0.8656630863528285147 ) ) ;
#12886=CARTESIAN_POINT ( 'NONE',  ( -13.41573142586496559, 156.9389434127184018, -0.3962193537810600463 ) ) ;
#12890=CARTESIAN_POINT ( 'NONE',  ( 8.615066246506550840, 118.4883731374293916, 1.081964075605263975 ) ) ;
#12891=ORIENTED_EDGE ( 'NONE', *, *, #8373, .T. ) ;
#12893=CARTESIAN_POINT ( 'NONE',  ( 15.28824200187825788, 154.8698957928756954, 2.015933685939941267 ) ) ;
#12894=CARTESIAN_POINT ( 'NONE',  ( 5.881924083617287913, 119.0696708348911699, -0.9594134845634215703 ) ) ;
#12895=CARTESIAN_POINT ( 'NONE',  ( -6.994280559954464849, 7.701067304790329082, -4.726517096957497444 ) ) ;
#12896=CARTESIAN_POINT ( 'NONE',  ( -21.80715381475374315, 148.2155681941778482, -2.148825447453798443 ) ) ;
#12897=CARTESIAN_POINT ( 'NONE',  ( 4.801507292439965546, 117.8464550438453529, -0.7717428139693086608 ) ) ;
#12900=CARTESIAN_POINT ( 'NONE',  ( -13.59242215834144751, 150.2357272821285221, -0.2218801189746051894 ) ) ;
#12901=CARTESIAN_POINT ( 'NONE',  ( -17.74096168611294289, 140.4837523222294351, -2.437162785362842143 ) ) ;
#12903=CARTESIAN_POINT ( 'NONE',  ( 4.157678856868515460, -15.71065181052187754, 4.128466586810772831 ) ) ;
#12906=VERTEX_POINT ( 'NONE', #18799 ) ;
#12907=CARTESIAN_POINT ( 'NONE',  ( 12.38071862475238660, 124.1810962131942517, 1.797420231217670139 ) ) ;
#12910=CARTESIAN_POINT ( 'NONE',  ( -2.292460607442647014, 118.3648483361698851, 0.7949187631362103490 ) ) ;
#12911=CARTESIAN_POINT ( 'NONE',  ( 4.673167956146812685, 25.32871407960522347, 7.020956665532097851 ) ) ;
#12912=CARTESIAN_POINT ( 'NONE',  ( 5.875838086862335885, 121.3091694753028520, 0.5415667612380998808 ) ) ;
#12913=CARTESIAN_POINT ( 'NONE',  ( 18.18789719519565296, 154.1160801429439857, -0.6523539814353513933 ) ) ;
#12915=B_SPLINE_CURVE_WITH_KNOTS ( 'NONE', 3,
 ( #18992, #31996, #40084, #3886, #23012, #20453, #897, #4310, #27076, #30060, #36040, #39445, #26652, #13454, #3671, #17057, #23867, #7493, #17476, #33480 ),
 .UNSPECIFIED., .F., .F.,
 ( 4, 2, 2, 2, 2, 2, 2, 2, 2, 4 ),
 ( -5.999999999764871059E-08, 0.0007881984188580538637, 0.001576456837716104986, 0.002364715256574156325, 0.003152973675432207881, 0.003941232094290259003, 0.004729490513148310558, 0.006306007350864415405, 0.009459041026296625965, 0.01261207470172883739 ),
 .UNSPECIFIED. ) ;
#12919=CARTESIAN_POINT ( 'NONE',  ( -22.75657594704724929, 137.3797884758947703, -0.4311216471409407558 ) ) ;
#12921=CARTESIAN_POINT ( 'NONE',  ( 6.528646965957701553, 120.3692086654437361, -0.8958864263995045540 ) ) ;
#12922=CARTESIAN_POINT ( 'NONE',  ( 23.36555825341164550, 148.7788340588663800, 0.4668994608413311043 ) ) ;
#12923=CARTESIAN_POINT ( 'NONE',  ( -15.47370139510886666, 143.5853813351167219, -1.046079274478293852 ) ) ;
#12924=CARTESIAN_POINT ( 'NONE',  ( 3.965039388734942882, -13.93407386435618989, 4.333124597978631698 ) ) ;
#12926=CARTESIAN_POINT ( 'NONE',  ( 23.11127252101355722, 149.9001116002701224, 0.4618182267416076070 ) ) ;
#12928=EDGE_LOOP ( 'NONE', ( #35022, #28610, #1608 ) ) ;
#12929=CARTESIAN_POINT ( 'NONE',  ( -2.707926769430928804, 11.08828375386998033, -3.745406074561137721 ) ) ;
#12930=CARTESIAN_POINT ( 'NONE',  ( 3.301553950842845531, 105.1237708183731172, 4.201341878287736087 ) ) ;
#12933=CARTESIAN_POINT ( 'NONE',  ( -7.864245281215539229, 122.2955428227499937, 0.4135678702982136246 ) ) ;
#12934=CARTESIAN_POINT ( 'NONE',  ( -2.426139246716550346, 10.07336736126799437, 3.943011612146583023 ) ) ;
#12935=CARTESIAN_POINT ( 'NONE',  ( 14.92386488306798675, 121.2513550155162960, 1.224273950129214805 ) ) ;
#12936=CARTESIAN_POINT ( 'NONE',  ( -0.07157677170311223247, 110.3683645023726569, 3.581994345755902032 ) ) ;
#12937=CARTESIAN_POINT ( 'NONE',  ( 3.177488185987922709, -14.13217061847354472, 2.003775387181677026 ) ) ;
#12938=CARTESIAN_POINT ( 'NONE',  ( 2.167900391131057702, 117.8876587302075194, -0.6265904732959521883 ) ) ;
#12939=CARTESIAN_POINT ( 'NONE',  ( -1.889208318266999198, 10.27326514537015534, 4.227218769941996968 ) ) ;
#12940=CARTESIAN_POINT ( 'NONE',  ( -22.60558431049205197, 149.7032342875954498, -1.528355188309250323 ) ) ;
#12942=CARTESIAN_POINT ( 'NONE',  ( -7.056912283644773964, 122.0434499869739540, 0.04958421841494448784 ) ) ;
#12943=CARTESIAN_POINT ( 'NONE',  ( 6.101987814473650573, -12.39306998090061640, 0.4902605208062851827 ) ) ;
#12947=CARTESIAN_POINT ( 'NONE',  ( 19.66043293732242603, 148.5147687316951135, 2.511426770373371031 ) ) ;
#12948=CARTESIAN_POINT ( 'NONE',  ( 3.527324519276021420, 50.63946620154572997, -1.707870599815379586 ) ) ;
#12950=CARTESIAN_POINT ( 'NONE',  ( -3.161282452094362316, 159.3671203531505114, 0.6484678655804385627 ) ) ;
#12952=CARTESIAN_POINT ( 'NONE',  ( 3.792432603185356133, 116.7736770086926867, -0.1904249565637310959 ) ) ;
#12953=CARTESIAN_POINT ( 'NONE',  ( -5.011781081284850003, 115.7029491485453576, -1.398622308649235979 ) ) ;
#12957=CARTESIAN_POINT ( 'NONE',  ( -4.973857814267949706, 117.3975374627346326, -0.9751189716041865907 ) ) ;
#12960=CARTESIAN_POINT ( 'NONE',  ( -4.537430495507082107, 118.0683159900091539, 0.6374709560671608655 ) ) ;
#12962=B_SPLINE_SURFACE_WITH_KNOTS ( 'NONE', 3, 3, ( 
 ( #4287, #34087, #13638, #24056, #17455, #30454, #4707, #876, #14053, #30036, #7262, #39637 ),
 ( #1298, #14254, #37071, #13848, #26847, #23414, #10650, #26630, #20851, #21061, #23846, #27057 ),
 ( #20641, #40065, #4916, #20432, #29832, #1508, #670, #4495, #20222, #33249, #4078, #36867 ),
 ( #39854, #7682, #27263, #40279, #11072, #23631, #33460, #14463, #17251, #7889, #8718, #28091 ),
 ( #38323, #14880, #41102, #1715, #34704, #21680, #9142, #11478, #11908, #5750, #15516, #41525 ),
 ( #21893, #24467, #40686, #5533, #22099, #34922, #37471, #28307, #2555, #31496, #40891, #28518 ),
 ( #38111, #18491, #8298, #25318, #21267, #24897, #35128, #14671, #2344, #18702, #17870, #34296 ),
 ( #15301, #41314, #8926, #12119, #5126, #30871, #18077, #37896, #27675, #31080, #25108, #31713 ),
 ( #1919, #5328, #12330, #27882, #11695, #24681, #37689, #8511, #21470, #34500, #18282, #31283 ),
 ( #2126, #15090, #20125, #4185, #3978, #10757, #33355, #29938, #16726, #23739, #12536, #32130 ),
 ( #16939, #9342, #15924, #776, #5955, #22305, #2961, #25728, #28922, #19922, #17148, #13753 ),
 ( #18914, #31924, #26748, #36353, #7167, #10554, #19124, #6953, #35329, #25525, #15716, #3767 ),
 ( #33151, #39759, #6156, #41940, #28720, #12740, #2761, #23523, #30149, #571, #29730, #38735 ),
 ( #13545, #990, #9543, #41731, #36550, #38525, #10345, #22513, #35544, #13955, #26536, #32938 ),
 ( #39539, #23316, #7370, #20328, #26953, #39966, #40788, #11801, #30562, #27574, #4810, #5016 ),
 ( #33777, #17761, #20539, #11379, #40582, #27988, #30347, #30761, #24571, #34391, #18179, #5225 ),
 ( #1196, #17359, #24366, #14986, #11589, #14156, #17976, #21365, #31181, #33569, #7792, #27159 ),
 ( #21159, #2022, #14777, #23952, #37373, #40173, #10965, #40380, #27777, #36759, #37577, #40996 ),
 ( #8404, #7578, #4403, #36970, #8190, #1611, #20753, #34190, #1401, #30974, #33982, #1814 ),
 ( #27369, #4605, #17561, #14569, #14357, #11175, #24160, #37169, #7991, #20961, #15199, #12441 ),
 ( #41209, #8827, #2451, #34814, #38223, #22414, #22206, #9250, #38434, #25435, #28202, #35237 ),
 ( #28836, #38006, #25219, #12011, #2240, #34603, #22004, #6062, #19022, #32029, #25004, #21787 ),
 ( #5648, #21576, #15828, #6266, #18812, #35036, #18606, #15617, #5856, #35441, #15411, #24790 ),
 ( #29035, #28622, #5431, #8612, #19236, #31821, #31612, #28416, #9039, #2659, #41634, #2868 ) ),
 .UNSPECIFIED., .F., .F., .F.,
 ( 4, 2, 2, 2, 2, 2, 2, 2, 2, 2, 2, 4 ),
 ( 4, 2, 1, 2, 1, 2, 4 ),
 ( 0.000000000000000000, 0.1320131134996915812, 0.1980196702495373717, 0.2640262269993831623, 0.3918780277393359990, 0.4558039281093124173, 0.5197298284792888357, 0.5807783984393792842, 0.6418269683994697328, 0.7639241083196507409, 0.8819620541598254260, 1.000000000000000000 ),
 ( 0.000000000000000000, 0.1250000000000000000, 0.2500000000000000000, 0.5000000000000000000, 0.7500000000000000000, 0.8750000000000000000, 1.000000000000000000 ),
 .UNSPECIFIED. ) ;
#12963=ORIENTED_EDGE ( 'NONE', *, *, #7169, .F. ) ;
#12965=CARTESIAN_POINT ( 'NONE',  ( -5.985785924374277478, 119.2914591321808189, -1.266711398467851746 ) ) ;
#12966=CARTESIAN_POINT ( 'NONE',  ( -5.733418603097514499, 118.4539739381501988, -0.6622650514401647870 ) ) ;
#12968=CARTESIAN_POINT ( 'NONE',  ( 4.815183644347338365, 117.8246314654618345, 0.8831286348090380267 ) ) ;
#12970=CARTESIAN_POINT ( 'NONE',  ( -4.434842451389515716, 120.7762672505206041, -0.5587804529453966884 ) ) ;
#12971=CARTESIAN_POINT ( 'NONE',  ( -1.943362973813288486, 115.7022440231138063, -1.718213888689203772 ) ) ;
#12974=CARTESIAN_POINT ( 'NONE',  ( 7.117363349590072552, 122.4243137415680280, 0.03262055675632266616 ) ) ;
#12975=CARTESIAN_POINT ( 'NONE',  ( -2.572680461994368173, 120.1437993944865354, -0.5932419562244880540 ) ) ;
#12977=CARTESIAN_POINT ( 'NONE',  ( -0.02400040557479403425, 156.7459281804771365, 1.201078436782489822 ) ) ;
#12978=CARTESIAN_POINT ( 'NONE',  ( -2.448307479368688977, 115.7029487053374623, 1.604658189596191109 ) ) ;
#12979=CARTESIAN_POINT ( 'NONE',  ( -0.0007138457988933175546, 156.3034662015457741, 0.03572376281290677580 ) ) ;
#12980=CARTESIAN_POINT ( 'NONE',  ( -2.646443841375008432, -8.127818987380491578, -3.789199236247322133 ) ) ;
#12981=CARTESIAN_POINT ( 'NONE',  ( 15.39807837497266618, 121.0727120035890323, 0.9152850519163395759 ) ) ;
#12983=CARTESIAN_POINT ( 'NONE',  ( 4.546337323837841282, 104.6144662015457527, -1.651695662123250807 ) ) ;
#12984=CARTESIAN_POINT ( 'NONE',  ( 2.120377039319510715, -15.39027815159008128, 5.169171589912422426 ) ) ;
#12985=CARTESIAN_POINT ( 'NONE',  ( -18.94087081963961694, 148.8558894138562039, 1.735487911102015168 ) ) ;
#12986=CARTESIAN_POINT ( 'NONE',  ( 0.2491751845298053603, 0.8914985761586250446, 0.9476022430964140542 ) ) ;
#12987=CARTESIAN_POINT ( 'NONE',  ( -6.905604733424429931, 117.2797055272990292, -0.4577529590079176258 ) ) ;
#12988=CARTESIAN_POINT ( 'NONE',  ( -0.4068859638909740339, 2.017459551269393359, -0.8868740919469698669 ) ) ;
#12989=ORIENTED_EDGE ( 'NONE', *, *, #17360, .F. ) ;
#12991=CARTESIAN_POINT ( 'NONE',  ( 3.839037681459631646, 115.3331674797404247, 1.733041430519539183 ) ) ;
#12993=CARTESIAN_POINT ( 'NONE',  ( -6.388910139315926884, 155.4084287100276072, 0.7748799927007739008 ) ) ;
#12994=CARTESIAN_POINT ( 'NONE',  ( 2.004955844419833877, -15.09631637516548075, 5.820374350103214134 ) ) ;
#12995=CARTESIAN_POINT ( 'NONE',  ( 15.71777585039850500, 134.9797526104055123, -1.508943449597504483 ) ) ;
#12996=CARTESIAN_POINT ( 'NONE',  ( -15.71367270535934857, 153.2725199748809928, -2.344280857665636209 ) ) ;
#12999=CARTESIAN_POINT ( 'NONE',  ( 7.851578091136403259, 122.2417759690833066, 0.7721127453851787115 ) ) ;
#13000=CARTESIAN_POINT ( 'NONE',  ( -0.9584988517251393780, 37.03984800159950908, 1.311833450704142034 ) ) ;
#13001=CARTESIAN_POINT ( 'NONE',  ( 15.81858318527952179, 146.5893318786020814, -0.01456738144011935666 ) ) ;
#13003=FACE_OUTER_BOUND ( 'NONE', #18932, .T. ) ;
#13008=CARTESIAN_POINT ( 'NONE',  ( 8.216694157412756994, 117.5064756823292385, 0.07510791844681398433 ) ) ;
#13009=CARTESIAN_POINT ( 'NONE',  ( -5.615711437771641279, 117.9270669303711117, 0.5242027053071315335 ) ) ;
#13010=AXIS2_PLACEMENT_3D ( 'NONE', #20718, #13714, #4147 ) ;
#13011=CARTESIAN_POINT ( 'NONE',  ( -4.262945350134766720, 117.9852873898591952, 0.8017283871570700660 ) ) ;
#13012=DIRECTION ( 'NONE',  ( -0.01997839162482761832, -1.040247600000950455E-18, 0.9998004120163610509 ) ) ;
#13013=CARTESIAN_POINT ( 'NONE',  ( -3.549018488562215801, 31.67372709507380790, 0.4994073303616778925 ) ) ;
#13014=CARTESIAN_POINT ( 'NONE',  ( 12.91357091396819357, 121.2479969211051127, 1.612259173617573316 ) ) ;
#13015=CARTESIAN_POINT ( 'NONE',  ( -3.199182136055901626, 19.34408232073488065, 3.339653329369344004 ) ) ;
#13016=CARTESIAN_POINT ( 'NONE',  ( -4.443900581410109574, 30.07671411637534931, -7.177485988639727310 ) ) ;
#13017=CARTESIAN_POINT ( 'NONE',  ( -2.173371897564630117, 116.7870940319093620, -0.5153656708244387374 ) ) ;
#13018=CARTESIAN_POINT ( 'NONE',  ( -2.096106201831416271, 122.9394440205640961, -0.1965313455681949872 ) ) ;
#13020=CIRCLE ( 'NONE', #30718, 5.080000000000006288 ) ;
#13022=CARTESIAN_POINT ( 'NONE',  ( 3.055547683721570262, 104.6144662015413047, 4.375596321116328014 ) ) ;
#13023=CIRCLE ( 'NONE', #36865, 0.5079999999999946780 ) ;
#13024=CARTESIAN_POINT ( 'NONE',  ( -0.5093740622119584671, 14.76157059199007016, 4.595130897425484306 ) ) ;
#13026=CARTESIAN_POINT ( 'NONE',  ( -0.7702531061077007024, 117.3993836066117353, -1.486315056237274890 ) ) ;
#13027=CARTESIAN_POINT ( 'NONE',  ( 3.025122737553283869, -13.62787997529110662, 1.286645544439679156 ) ) ;
#13029=ADVANCED_FACE ( 'NONE', ( #9027 ), #19082, .F. ) ;
#13030=CARTESIAN_POINT ( 'NONE',  ( 1.859996092182608640, 121.3688471916803451, -0.2894809034927952052 ) ) ;
#13031=CARTESIAN_POINT ( 'NONE',  ( -21.63859276624145878, 151.3813297165527274, 0.4067934712883242709 ) ) ;
#13032=ORIENTED_EDGE ( 'NONE', *, *, #2569, .T. ) ;
#13034=EDGE_LOOP ( 'NONE', ( #6667, #14960, #21486, #34133 ) ) ;
#13035=CARTESIAN_POINT ( 'NONE',  ( -2.880736501481947265, 31.22451072257329585, 0.7774695130801791976 ) ) ;
#13037=CARTESIAN_POINT ( 'NONE',  ( 6.120062074970366695, -14.59381343598747982, -0.2446369611249375742 ) ) ;
#13038=CARTESIAN_POINT ( 'NONE',  ( -19.84954981513673644, 141.2215177107240436, 1.686013488323441223 ) ) ;
#13039=CARTESIAN_POINT ( 'NONE',  ( 13.66011217756154394, 120.8017016962898396, -0.8211468655896803082 ) ) ;
#13040=CARTESIAN_POINT ( 'NONE',  ( 0.05711764529616595448, 0.5181683540770932739, -4.631227783250111862 ) ) ;
#13044=CARTESIAN_POINT ( 'NONE',  ( -0.002462548249366884514, 123.7646714092002611, 0.1232359841710926190 ) ) ;
#13045=( NAMED_UNIT ( * ) PLANE_ANGLE_UNIT ( ) SI_UNIT ( $, .RADIAN. ) );
#13046=CARTESIAN_POINT ( 'NONE',  ( -17.54876304911002194, 147.2926247242496345, 1.462364720961516040 ) ) ;
#13047=CARTESIAN_POINT ( 'NONE',  ( 12.22472920326790558, 122.9664497093790629, -1.310580005724927499 ) ) ;
#13048=CARTESIAN_POINT ( 'NONE',  ( -20.74782508767443900, 148.9555414352193168, -2.393722347598511657 ) ) ;
#13051=CARTESIAN_POINT ( 'NONE',  ( 4.556576186746449153, 118.1065164564682703, -0.4936797517044704819 ) ) ;
#13052=CARTESIAN_POINT ( 'NONE',  ( 15.06908741399238849, 148.9283877096812034, -0.6536164350837784243 ) ) ;
#13054=CARTESIAN_POINT ( 'NONE',  ( -17.14693169618197999, 148.7218176724978775, -2.218585656167707754 ) ) ;
#13055=CARTESIAN_POINT ( 'NONE',  ( 3.847030120444227208, -15.22745156820166912, 0.3463556848800000143 ) ) ;
#13056=CARTESIAN_POINT ( 'NONE',  ( -5.043483815839604922, 105.1217967216603029, -1.770462747484127242 ) ) ;
#13061=CARTESIAN_POINT ( 'NONE',  ( -4.784146136289919582, 117.6343108313606933, 0.9514533180737122509 ) ) ;
#13062=CARTESIAN_POINT ( 'NONE',  ( 8.120140396194329924, 121.3802920439979118, 1.244985559442681078 ) ) ;
#13064=CARTESIAN_POINT ( 'NONE',  ( 3.655561289726139140, 27.93047918286777076, -2.829280713513928180 ) ) ;
#13065=CARTESIAN_POINT ( 'NONE',  ( 5.931002064882541447, 121.5392726388429168, 0.1896088198168330019 ) ) ;
#13069=CARTESIAN_POINT ( 'NONE',  ( 8.798071512540863282, 117.6842349196870572, 0.1758064070670784795 ) ) ;
#13070=CARTESIAN_POINT ( 'NONE',  ( -5.078986093043186045, 87.97746620154572383, -0.1014902294541231709 ) ) ;
#13073=CARTESIAN_POINT ( 'NONE',  ( -8.557937876389182463, 118.7559978815208552, -1.194452831535397719 ) ) ;
#13080=CARTESIAN_POINT ( 'NONE',  ( -0.002426349801212479562, 116.5266044092193880, 0.1214244658147705380 ) ) ;
#13083=CARTESIAN_POINT ( 'NONE',  ( -6.055293159970121408, 121.4335270663578683, -0.1273889451180159893 ) ) ;
#13086=CARTESIAN_POINT ( 'NONE',  ( -0.6369907463662666247, 120.9735524437166561, -0.07606544612864242494 ) ) ;
#13087=CARTESIAN_POINT ( 'NONE',  ( 2.850627862023833892, -15.32561772411503220, 5.765353718581858189 ) ) ;
#13088=CARTESIAN_POINT ( 'NONE',  ( -13.73828690980685963, 121.6032371815301900, 1.070726600328922640 ) ) ;
#13089=CARTESIAN_POINT ( 'NONE',  ( -5.112263072780976358, 116.9830771656617827, -0.4445654250014547948 ) ) ;
#13091=CARTESIAN_POINT ( 'NONE',  ( 14.74522353080544157, 120.3062992333385921, 0.5208356519839252297 ) ) ;
#13092=CARTESIAN_POINT ( 'NONE',  ( 9.045801974870443019, 124.1535288145754237, 0.2702127546846336825 ) ) ;
#13093=CARTESIAN_POINT ( 'NONE',  ( 5.276949677772993397, 115.6909491485453145, -0.8076138971160246038 ) ) ;
#13094=CARTESIAN_POINT ( 'NONE',  ( -0.5978751570792395498, 11.96162690172616294, -0.7744233872902203109 ) ) ;
#13095=CARTESIAN_POINT ( 'NONE',  ( -15.60991558517076605, 120.8175431576145940, -0.4704071646738434143 ) ) ;
#13096=DIRECTION ( 'NONE',  ( -0.9998004120163608288, -5.205824365704081956E-17, -0.01997839162482748995 ) ) ;
#13097=EDGE_CURVE ( 'NONE', #17493, #24980, #1661, .T. ) ;
#13100=CARTESIAN_POINT ( 'NONE',  ( 5.660275087203261002, 117.9280556746221293, 1.049642431879043158 ) ) ;
#13103=CARTESIAN_POINT ( 'NONE',  ( 12.26619010297299717, 120.4651188882986759, 1.462776157934944310 ) ) ;
#13104=CARTESIAN_POINT ( 'NONE',  ( 1.243168248768940831, 118.5604221528582372, -0.6402677339867957063 ) ) ;
#13105=CARTESIAN_POINT ( 'NONE',  ( 0.3859925973045487679, 4.674766832570296238, -0.8944012262243137279 ) ) ;
#13106=CARTESIAN_POINT ( 'NONE',  ( -3.896388542364412455, 10.26897056970580380, 7.485861278012786002 ) ) ;
#13107=CARTESIAN_POINT ( 'NONE',  ( -9.779442063456469825, 157.5983698538113629, -1.672576317993901274 ) ) ;
#13108=CARTESIAN_POINT ( 'NONE',  ( 4.803717081333231498, 117.8803964050671311, -0.6822223753014300396 ) ) ;
#13109=CARTESIAN_POINT ( 'NONE',  ( 7.326027964657929381, 123.0350022594044219, 0.2150643116641768604 ) ) ;
#13111=CARTESIAN_POINT ( 'NONE',  ( 7.221579903133987344, 121.4526873951801633, -0.6561908252823551724 ) ) ;
#13112=CARTESIAN_POINT ( 'NONE',  ( -5.308493528853332144, 121.3525139070573147, -0.1060763342189516428 ) ) ;
#13115=CARTESIAN_POINT ( 'NONE',  ( -10.15136974315543839, 155.5514087735115822, -2.139549497352468244 ) ) ;
#13116=CARTESIAN_POINT ( 'NONE',  ( 5.552702978602249040, -15.16724029374752547, 2.010675452401557095 ) ) ;
#13121=CARTESIAN_POINT ( 'NONE',  ( 0.4972808831007263231, 119.3183582894065893, 0.5800711753708563956 ) ) ;
#13122=CARTESIAN_POINT ( 'NONE',  ( -15.26262975083406381, 148.0175730703489592, -0.3049836654617371079 ) ) ;
#13123=EDGE_CURVE ( 'NONE', #34625, #37003, #25337, .T. ) ;
#13126=CARTESIAN_POINT ( 'NONE',  ( -4.551932963793476006, 124.4408722044843927, -0.07212455616362435651 ) ) ;
#13128=CARTESIAN_POINT ( 'NONE',  ( -6.340062920055459017, 30.52953040661039807, -5.581008500864042432 ) ) ;
#13129=CARTESIAN_POINT ( 'NONE',  ( 9.927929498514727058, 124.8826105625126530, 0.6426615136408517781 ) ) ;
#13130=CARTESIAN_POINT ( 'NONE',  ( 4.841477346015976124, 117.1414559920645644, -0.3963857013944135366 ) ) ;
#13134=CARTESIAN_POINT ( 'NONE',  ( -21.90617686096483396, 151.4314113202728436, -0.4124301881307765316 ) ) ;
#13137=CARTESIAN_POINT ( 'NONE',  ( 6.859376321155130185, 121.4516053872399226, -0.5286681357537772463 ) ) ;
#13139=CARTESIAN_POINT ( 'NONE',  ( -13.22128265123331481, 134.0707761029912035, -0.8398552229569320460 ) ) ;
#13140=CARTESIAN_POINT ( 'NONE',  ( 2.474817137005230983, -14.89163965485640340, 5.628581999208025266 ) ) ;
#13142=CARTESIAN_POINT ( 'NONE',  ( 23.42514220146282966, 142.8382549601284097, 0.4680900899253090941 ) ) ;
#13144=CARTESIAN_POINT ( 'NONE',  ( 4.087030650986479330, 6.990161447142720696, 2.163025551504125232 ) ) ;
#13145=CARTESIAN_POINT ( 'NONE',  ( -0.2924095564369283418, 116.4254662015451913, -0.005843038833676759622 ) ) ;
#13146=CARTESIAN_POINT ( 'NONE',  ( -13.43845804798116106, 156.9141898299356512, -0.2685323735513600041 ) ) ;
#13148=CARTESIAN_POINT ( 'NONE',  ( -6.019795697468436124, 120.5055318871546461, 0.7549818993857987381 ) ) ;
#13149=CARTESIAN_POINT ( 'NONE',  ( 4.577905313181523717, 13.52175256873284326, -0.6256056815880789435 ) ) ;
#13150=CARTESIAN_POINT ( 'NONE',  ( 21.93197806114481807, 150.5960492154097778, 1.608405794939391731 ) ) ;
#13153=CARTESIAN_POINT ( 'NONE',  ( 21.18042260023730705, 148.1333099715771766, -1.515480231459294114 ) ) ;
#13155=CARTESIAN_POINT ( 'NONE',  ( -1.792273654952471595, 16.32048121479114045, -4.264856162967389785 ) ) ;
#13156=CARTESIAN_POINT ( 'NONE',  ( -3.132853369507721197, 159.3671203531505114, -0.7742396785067983123 ) ) ;
#13159=ADVANCED_FACE ( 'NONE', ( #36963 ), #26792, .F. ) ;
#13160=B_SPLINE_CURVE_WITH_KNOTS ( 'NONE', 3,
 ( #15571, #32766, #41372, #12392 ),
 .UNSPECIFIED., .F., .F.,
 ( 4, 4 ),
 ( 0.001531465774898539082, 0.001759348651853699479 ),
 .UNSPECIFIED. ) ;
#13161=CARTESIAN_POINT ( 'NONE',  ( -10.49519746661490593, 153.0637448873655728, 0.1985316654307170414 ) ) ;
#13162=CARTESIAN_POINT ( 'NONE',  ( 5.767107246999573889, -13.94705323133380048, 2.761945726399152701 ) ) ;
#13163=DIRECTION ( 'NONE',  ( 4.017660918040594346E-17, -1.000000000000000000, -2.376309959284834438E-19 ) ) ;
#13165=CARTESIAN_POINT ( 'NONE',  ( -1.982805074603235296, 106.5591908312118221, -4.949216245379176371 ) ) ;
#13167=CARTESIAN_POINT ( 'NONE',  ( 12.48017577322008442, 122.5542284311838870, 1.820249166172293265 ) ) ;
#13170=CARTESIAN_POINT ( 'NONE',  ( -22.81445126409639812, 149.1304179266472261, 0.6239350898115072486 ) ) ;
#13171=EDGE_CURVE ( 'NONE', #9260, #3899, #19556, .T. ) ;
#13173=CARTESIAN_POINT ( 'NONE',  ( 15.22618061423887426, 120.7148350616293300, -0.1140551857323334473 ) ) ;
#13174=FACE_OUTER_BOUND ( 'NONE', #6098, .T. ) ;
#13175=CIRCLE ( 'NONE', #18611, 3.175000000000001155 ) ;
#13181=CARTESIAN_POINT ( 'NONE',  ( -4.601497063313658487, 118.0406231673457853, 0.6544036431963192735 ) ) ;
#13185=CARTESIAN_POINT ( 'NONE',  ( -0.1700182685997659593, 118.7629491485454025, -1.279869737540616059 ) ) ;
#13186=CARTESIAN_POINT ( 'NONE',  ( 5.909374519815934867, 119.0059304655898131, -1.022020752696235935 ) ) ;
#13187=CARTESIAN_POINT ( 'NONE',  ( -2.481140172163744495, 107.2306503360107541, -4.727365043318366489 ) ) ;
#13188=CARTESIAN_POINT ( 'NONE',  ( 4.584301209864922733, 117.9735000374216440, 0.9263109292462509137 ) ) ;
#13190=CARTESIAN_POINT ( 'NONE',  ( -9.867978122178644895, 123.6875948057429895, -1.092113756099770017 ) ) ;
#13192=CARTESIAN_POINT ( 'NONE',  ( -1.824499746566420999, 115.7028212133603802, -1.722090710131633173 ) ) ;
#13193=CARTESIAN_POINT ( 'NONE',  ( -1.119363313351095846, 106.1653619527225629, 5.174161313809158891 ) ) ;
#13195=CARTESIAN_POINT ( 'NONE',  ( 7.669269000495035904, 124.9344662015457317, 0.1532502464757267702 ) ) ;
#13196=CARTESIAN_POINT ( 'NONE',  ( -17.14717842969347572, 147.4900653055648547, -2.050122926623737296 ) ) ;
#13197=CARTESIAN_POINT ( 'NONE',  ( 15.97340373827820947, 121.0409387471171101, 0.3191866212789526425 ) ) ;
#13198=CARTESIAN_POINT ( 'NONE',  ( -0.02615207601228260181, 159.0391464308674756, 1.308756824028193488 ) ) ;
#13199=CYLINDRICAL_SURFACE ( 'NONE', #2502, 5.588000000000006295 ) ;
#13200=CARTESIAN_POINT ( 'NONE',  ( -1.631653520256556744, 120.9961520629786094, 0.03448668289050316194 ) ) ;
#13201=CARTESIAN_POINT ( 'NONE',  ( 0.6989348986720191892, -4.029744825116962303, 4.573446973323917142 ) ) ;
#13202=CARTESIAN_POINT ( 'NONE',  ( 8.152918552588246826, 117.7057695168643932, 0.6423243676978417360 ) ) ;
#13206=CARTESIAN_POINT ( 'NONE',  ( 3.434117431421463973, -14.91634622600368587, 0.6670077989445850619 ) ) ;
#13208=CARTESIAN_POINT ( 'NONE',  ( -16.12483552447403312, 131.4332636412663931, 1.626400019052950618 ) ) ;
#13209=CARTESIAN_POINT ( 'NONE',  ( 0.9735350199255810022, 12.44701472381428609, 0.02964292050307446719 ) ) ;
#13210=CARTESIAN_POINT ( 'NONE',  ( -22.61937536341561383, 150.3405807453409579, -1.175526429919688365 ) ) ;
#13211=CARTESIAN_POINT ( 'NONE',  ( 0.9102147817015755482, -10.07290960004636737, -0.3509275504499672627 ) ) ;
#13212=EDGE_LOOP ( 'NONE', ( #35863, #37765, #21282, #22552 ) ) ;
#13215=CARTESIAN_POINT ( 'NONE',  ( 5.192700560040893976, 116.2637919873444190, 1.171650394069924994 ) ) ;
#13217=CARTESIAN_POINT ( 'NONE',  ( -14.80764902091328317, 139.2804412874323248, 0.6846718672572660314 ) ) ;
#13218=CARTESIAN_POINT ( 'NONE',  ( 3.936650548058306054, -12.34391569202568384, 1.586490187297609156 ) ) ;
#13219=CARTESIAN_POINT ( 'NONE',  ( 10.96277846527056532, 123.4376579628654014, -1.079141073574104270 ) ) ;
#13221=CARTESIAN_POINT ( 'NONE',  ( -6.391991208685121606, 157.5392376370035095, -1.942695856706931457 ) ) ;
#13223=CARTESIAN_POINT ( 'NONE',  ( 2.576299636888586875, -14.89815494326314571, 4.769281578164155100 ) ) ;
#13224=CARTESIAN_POINT ( 'NONE',  ( -4.217721592883738602, 33.55733840984517968, 3.057578620386037116 ) ) ;
#13225=CARTESIAN_POINT ( 'NONE',  ( 15.79579396213690679, 146.5797798787131399, 0.08547097745249054856 ) ) ;
#13231=CARTESIAN_POINT ( 'NONE',  ( 16.10770497005612611, 121.2391669109744186, 0.2160841345999988949 ) ) ;
#13232=CARTESIAN_POINT ( 'NONE',  ( -4.074523107743509343, 109.7948460773305897, 3.525254900318187889 ) ) ;
#13233=CARTESIAN_POINT ( 'NONE',  ( -0.2373459926208821014, 115.6909491485452435, 1.758351689424455966 ) ) ;
#13234=CARTESIAN_POINT ( 'NONE',  ( 5.078986093043054595, 72.99146620154573384, 0.1014902294541243921 ) ) ;
#13235=CARTESIAN_POINT ( 'NONE',  ( -4.449580246473387568, 31.68166237237402783, -0.1589607140948728348 ) ) ;
#13236=CARTESIAN_POINT ( 'NONE',  ( 17.27141581160015349, 128.5728276651957742, 2.069917288257624666 ) ) ;
#13237=CARTESIAN_POINT ( 'NONE',  ( -3.633452533992191036, 26.69063122243967712, -2.854640957048627747 ) ) ;
#13238=CARTESIAN_POINT ( 'NONE',  ( 8.390987441844862005, -15.30508105673078667, -0.4368898320763015541 ) ) ;
#13239=CARTESIAN_POINT ( 'NONE',  ( 5.512484162645947983, 117.2038984734866744, -0.5832805902496341899 ) ) ;
#13240=CARTESIAN_POINT ( 'NONE',  ( -3.315491766441375443, 124.7872298565087021, -0.07248898146901441852 ) ) ;
#13242=CARTESIAN_POINT ( 'NONE',  ( 4.660168586682497782, 113.7931333194828909, -2.025023631320468365 ) ) ;
#13243=CARTESIAN_POINT ( 'NONE',  ( -2.605357904536034663, 104.6144662015456959, 4.072382053397732626 ) ) ;
#13244=CARTESIAN_POINT ( 'NONE',  ( 4.585487687326599726, 17.13547844546973309, 0.5842699607688729424 ) ) ;
#13247=CARTESIAN_POINT ( 'NONE',  ( 3.115274840615241292, -13.78277351762104175, 1.693892316854531455 ) ) ;
#13248=CARTESIAN_POINT ( 'NONE',  ( 0.7241986523582714108, 107.9696733310005214, -4.463276061801070504 ) ) ;
#13249=CARTESIAN_POINT ( 'NONE',  ( -13.30049347609366528, 119.7426348059052685, 0.3046699512218789541 ) ) ;
#13250=ORIENTED_EDGE ( 'NONE', *, *, #5832, .T. ) ;
#13254=CARTESIAN_POINT ( 'NONE',  ( 3.081975983035755373, -15.74694164559999088, 5.217090789712465870 ) ) ;
#13255=CARTESIAN_POINT ( 'NONE',  ( -15.12798499870471325, 125.5446871707752763, 1.421763802809897115 ) ) ;
#13256=CARTESIAN_POINT ( 'NONE',  ( 15.47853073355907050, 123.0316835747794642, -0.9738675477772636979 ) ) ;
#13257=CARTESIAN_POINT ( 'NONE',  ( 4.523211737919912601, 7.414965188139293950, 0.9565071382433593117 ) ) ;
#13259=ORIENTED_EDGE ( 'NONE', *, *, #28787, .F. ) ;
#13261=CARTESIAN_POINT ( 'NONE',  ( 2.216013192100191542, 123.7320667226965867, 0.1296889073052086561 ) ) ;
#13263=CARTESIAN_POINT ( 'NONE',  ( -15.84185526851211634, 139.7295799824062499, 1.277977597745375782 ) ) ;
#13265=CARTESIAN_POINT ( 'NONE',  ( 14.54156464587782871, 128.5519869857110393, -1.481139062272948115 ) ) ;
#13266=CARTESIAN_POINT ( 'NONE',  ( -20.33492986670573188, 149.7738053052645171, -2.379138827545465684 ) ) ;
#13269=CARTESIAN_POINT ( 'NONE',  ( 4.514839441275080745, 118.1273531810763018, -0.5014787992856909460 ) ) ;
#13270=CARTESIAN_POINT ( 'NONE',  ( 6.293976855803866677, 155.3815620563194955, -0.6499927463934686012 ) ) ;
#13272=CARTESIAN_POINT ( 'NONE',  ( -10.97746297113260994, 123.2082810311540300, -1.564610664257708894 ) ) ;
#13273=CARTESIAN_POINT ( 'NONE',  ( 2.997986829609769366, -15.20712831582179980, 4.056362312997196184 ) ) ;
#13276=AXIS2_PLACEMENT_3D ( 'NONE', #1373, #28338, #15546 ) ;
#13277=CARTESIAN_POINT ( 'NONE',  ( -3.128764270554720728, 7.249652477310866594, -3.416742352092642321 ) ) ;
#13278=CARTESIAN_POINT ( 'NONE',  ( -0.02768739821015471850, 156.9833357668885014, 1.385590625008458865 ) ) ;
#13279=CARTESIAN_POINT ( 'NONE',  ( 3.005048127465709928, 39.20946620154573026, -0.9984965929130177331 ) ) ;
#13280=CARTESIAN_POINT ( 'NONE',  ( 8.141433899912401628, -11.15112405914982219, -2.164028758433363286 ) ) ;
#13281=CARTESIAN_POINT ( 'NONE',  ( 9.611064403080796126, 124.8310256250372277, 0.2802631513932195562 ) ) ;
#13284=CARTESIAN_POINT ( 'NONE',  ( 8.798540905981443672, 117.6856532891334979, 0.1377605412487556136 ) ) ;
#13285=DIRECTION ( 'NONE',  ( -0.01997839162482761832, -1.040247600000951803E-18, 0.9998004120163610509 ) ) ;
#13290=CARTESIAN_POINT ( 'NONE',  ( -4.074955089416341991, 118.2429491485453354, 0.1454234154749719787 ) ) ;
#13294=CARTESIAN_POINT ( 'NONE',  ( -0.002459401150367294953, 159.6023738651833810, 0.1230784904792620454 ) ) ;
#13297=CARTESIAN_POINT ( 'NONE',  ( 6.070073713991016362, 121.4399315956317054, 0.1168545408771763938 ) ) ;
#13300=CARTESIAN_POINT ( 'NONE',  ( -8.793090887881007234, 123.6850765633735421, -0.2090564433599596816 ) ) ;
#13301=CARTESIAN_POINT ( 'NONE',  ( 5.314795342858649185, -13.92002763284938638, 3.476347616104731753 ) ) ;
#13302=CARTESIAN_POINT ( 'NONE',  ( -13.59286959522826876, 121.6867650304669013, 1.114243377227002618 ) ) ;
#13303=CARTESIAN_POINT ( 'NONE',  ( 2.488009491785908800, 18.85968022696138391, -3.895047602898422223 ) ) ;
#13304=CARTESIAN_POINT ( 'NONE',  ( 22.75358200450888191, 150.3871190066015799, 0.9055542368224058780 ) ) ;
#13305=CARTESIAN_POINT ( 'NONE',  ( 7.761062069545141995, 154.6910982259716150, 0.3223645707746605193 ) ) ;
#13307=CARTESIAN_POINT ( 'NONE',  ( -0.6011478996571989475, -4.452122406214784611, 0.7678286701737500053 ) ) ;
#13308=CARTESIAN_POINT ( 'NONE',  ( -20.41771265994164608, 129.0384130229076334, -0.5332683426449598141 ) ) ;
#13309=CARTESIAN_POINT ( 'NONE',  ( -4.883848590450072358, 117.7607009110569862, 0.7127853619805604168 ) ) ;
#13311=ORIENTED_EDGE ( 'NONE', *, *, #25846, .F. ) ;
#13312=CIRCLE ( 'NONE', #13998, 0.5080000000000002292 ) ;
#13313=CARTESIAN_POINT ( 'NONE',  ( -5.551318956506019475, 117.0040208047680608, 0.4076684244378269151 ) ) ;
#13315=CARTESIAN_POINT ( 'NONE',  ( -14.06576283519511428, 128.5416456306063253, 1.400350009575090038 ) ) ;
#13317=CARTESIAN_POINT ( 'NONE',  ( 4.008523173341837165, 118.0179939250997023, 0.8984863180294773155 ) ) ;
#13318=CARTESIAN_POINT ( 'NONE',  ( 4.147108463826105762, 118.7489093234570561, -0.8374340306925341926 ) ) ;
#13319=CARTESIAN_POINT ( 'NONE',  ( -0.4197673533123916778, 5.974963139197415174, -0.8815698914671175057 ) ) ;
#13320=CARTESIAN_POINT ( 'NONE',  ( -3.949038439882312179, 117.6225627337916393, -0.7921763187007299090 ) ) ;
#13321=CARTESIAN_POINT ( 'NONE',  ( 4.730749274543958549, 117.9657169516164856, -0.6167170664779215716 ) ) ;
#13322=CARTESIAN_POINT ( 'NONE',  ( -6.442348895218290093E-14, 63.84746620154572838, 4.408874939877717575E-29 ) ) ;
#13323=CARTESIAN_POINT ( 'NONE',  ( 17.01014995307818722, 147.0740084267719396, -1.247012517048586622 ) ) ;
#13324=CARTESIAN_POINT ( 'NONE',  ( -0.6421132086019301077, 120.9975462804897433, 0.01250379197263697117 ) ) ;
#13325=VERTEX_POINT ( 'NONE', #7159 ) ;
#13326=CARTESIAN_POINT ( 'NONE',  ( -18.62504088965198434, 146.9271955717142930, -2.448500584228243682 ) ) ;
#13327=CARTESIAN_POINT ( 'NONE',  ( 3.756887254765235440, -15.74060793811991843, 4.623245420838687281 ) ) ;
#13328=CARTESIAN_POINT ( 'NONE',  ( -5.339075059129462453, 115.7029491485453718, 0.2008031272278917312 ) ) ;
#13331=ORIENTED_EDGE ( 'NONE', *, *, #8940, .F. ) ;
#13332=CARTESIAN_POINT ( 'NONE',  ( 11.35704730865796463, 122.8492764348241337, 1.683887364911069273 ) ) ;
#13333=CARTESIAN_POINT ( 'NONE',  ( -3.999880774356848523, 33.21692059697370070, 1.336717509662867398 ) ) ;
#13335=CARTESIAN_POINT ( 'NONE',  ( -1.795323270064466792, 111.6436615656963909, 3.008962535700986596 ) ) ;
#13336=CARTESIAN_POINT ( 'NONE',  ( -6.161128625374170831, 23.17997237347384853, 5.746845633999829950 ) ) ;
#13337=CARTESIAN_POINT ( 'NONE',  ( 5.891535241408099033, 121.4229528491920576, 0.4202535615248634837 ) ) ;
#13338=ADVANCED_FACE ( 'NONE', ( #27152 ), #28288, .T. ) ;
#13340=CARTESIAN_POINT ( 'NONE',  ( 5.853624122459038404, 117.3024554866451865, -0.4121555180536239926 ) ) ;
#13341=CARTESIAN_POINT ( 'NONE',  ( 4.850929972935443146, 117.7610086971114356, 0.9074237114610381738 ) ) ;
#13343=CARTESIAN_POINT ( 'NONE',  ( -5.781358041568783968, 116.9360814311326777, -0.07286664083783161994 ) ) ;
#13345=CARTESIAN_POINT ( 'NONE',  ( 5.100432878203172926, 120.2001702409422990, -0.6603920651319280521 ) ) ;
#13346=CARTESIAN_POINT ( 'NONE',  ( 6.167707869044355640, -13.99985869331082178, 1.617558169626257314 ) ) ;
#13347=CARTESIAN_POINT ( 'NONE',  ( -15.76219760562764094, 147.2673792861271522, -0.9072345144146883866 ) ) ;
#13348=CARTESIAN_POINT ( 'NONE',  ( 4.249299001760414640, -12.92553893317818847, 2.698699680779739207 ) ) ;
#13349=CARTESIAN_POINT ( 'NONE',  ( -14.96856157597592940, 121.5307057168427605, 0.7335553340177137782 ) ) ;
#13350=CARTESIAN_POINT ( 'NONE',  ( -5.152689475313444234, 116.8412042432202185, -0.1029630068797482562 ) ) ;
#13351=CARTESIAN_POINT ( 'NONE',  ( 23.21042342040053086, 149.6290410902582551, 0.5408589295980603673 ) ) ;
#13353=CARTESIAN_POINT ( 'NONE',  ( 3.728136974946417492, 6.765255174955887796, 2.739693761753763113 ) ) ;
#13355=CARTESIAN_POINT ( 'NONE',  ( -20.51686376604223128, 129.1072961674477710, -0.4099757654675940111 ) ) ;
#13357=CARTESIAN_POINT ( 'NONE',  ( 2.292992513364368268, 106.8193516554411531, 4.820700389358663962 ) ) ;
#13358=CARTESIAN_POINT ( 'NONE',  ( 7.873896660004363390, 122.1234394815680986, 0.8695851236811991125 ) ) ;
#13360=CARTESIAN_POINT ( 'NONE',  ( 2.854375549615681962, 5.100648791940559867, -3.633247542873777380 ) ) ;
#13361=CARTESIAN_POINT ( 'NONE',  ( 21.15273274666895276, 151.2337125027825095, 1.710087910014103985 ) ) ;
#13362=CARTESIAN_POINT ( 'NONE',  ( -0.09909826073589839135, 106.8097931225389630, 4.959282197179073925 ) ) ;
#13364=CARTESIAN_POINT ( 'NONE',  ( 15.00359386227399483, 154.7288491705591866, -1.534247969496847164 ) ) ;
#13365=CARTESIAN_POINT ( 'NONE',  ( 3.679437910380295218, 2.726752568732802917, 2.794697870780981752 ) ) ;
#13366=CARTESIAN_POINT ( 'NONE',  ( 0.006370369177271557534, 117.0014201992989058, -0.3187993231787206727 ) ) ;
#13367=ADVANCED_FACE ( 'NONE', ( #20454 ), #12634, .T. ) ;
#13368=AXIS2_PLACEMENT_3D ( 'NONE', #25299, #9123, #35111 ) ;
#13370=CARTESIAN_POINT ( 'NONE',  ( -3.009276887026423264, 44.28946620154572855, 1.210121013456480377 ) ) ;
#13371=AXIS2_PLACEMENT_3D ( 'NONE', #19717, #32737, #16529 ) ;
#13372=CARTESIAN_POINT ( 'NONE',  ( -7.065481736843254090, 122.0164807696326790, 0.1187983231582535742 ) ) ;
#13373=CARTESIAN_POINT ( 'NONE',  ( 3.833788745076180060, -15.06587152019073272, 5.274579322627055866 ) ) ;
#13375=CARTESIAN_POINT ( 'NONE',  ( -2.321297342765445748, 107.3035951680803635, -4.704727343862274758 ) ) ;
#13377=CARTESIAN_POINT ( 'NONE',  ( 6.111605970564418122, 157.2590385278250267, 1.959406070573513459 ) ) ;
#13381=CARTESIAN_POINT ( 'NONE',  ( -22.85738479169587123, 148.8343141121478652, 0.6244747819152592916 ) ) ;
#13382=CARTESIAN_POINT ( 'NONE',  ( 7.231359443275770182, 22.16797014818540745, 4.386519482779798196 ) ) ;
#13383=CARTESIAN_POINT ( 'NONE',  ( 15.62286502882988870, 121.0226940419799462, -0.1111101786179099632 ) ) ;
#13386=DIRECTION ( 'NONE',  ( 0.9998004120163609398, 0.000000000000000000, 0.01997839162482749342 ) ) ;
#13388=CARTESIAN_POINT ( 'NONE',  ( 1.819893491534947838, -15.08787143633222350, 5.611221046887520103 ) ) ;
#13391=CARTESIAN_POINT ( 'NONE',  ( -4.387617986301902917, 118.1845766253724150, 0.4238482731264395231 ) ) ;
#13393=AXIS2_PLACEMENT_3D ( 'NONE', #5822, #29427, #41818 ) ;
#13394=ORIENTED_EDGE ( 'NONE', *, *, #21517, .F. ) ;
#13396=CARTESIAN_POINT ( 'NONE',  ( -8.314269420833845459, 119.9197522654141750, -1.446063649029603715 ) ) ;
#13398=CARTESIAN_POINT ( 'NONE',  ( -6.073876170729706203, 119.5347744825833871, -0.5156133147040063980 ) ) ;
#13399=CARTESIAN_POINT ( 'NONE',  ( 4.441115804996636385, 118.1267861108847086, 0.7297787586869709520 ) ) ;
#13400=CARTESIAN_POINT ( 'NONE',  ( -6.488156926834150795, 121.4051597255373025, -0.7118474008431249223 ) ) ;
#13401=CARTESIAN_POINT ( 'NONE',  ( -2.487218026922475733, 115.7030328841145206, -1.696577405177432496 ) ) ;
#13403=CARTESIAN_POINT ( 'NONE',  ( 5.252825482164369397, 116.2501875120488393, -0.9643948023431453409 ) ) ;
#13404=CARTESIAN_POINT ( 'NONE',  ( -17.23725050067796616, 146.8699245690979751, -2.055247338431126725 ) ) ;
#13406=CARTESIAN_POINT ( 'NONE',  ( -0.02969037535081191920, 158.7301711276701894, 1.485827791648137497 ) ) ;
#13407=CARTESIAN_POINT ( 'NONE',  ( 8.060916924639187187, 121.3839393899244925, -0.8986322262796456739 ) ) ;
#13408=CARTESIAN_POINT ( 'NONE',  ( -15.38354879105530237, 147.8362818251703459, -0.1740999797858117648 ) ) ;
#13410=CARTESIAN_POINT ( 'NONE',  ( -4.478778176974229197, 3.316883148187759645, 1.141857468124592101 ) ) ;
#13411=CARTESIAN_POINT ( 'NONE',  ( 21.68922513019249010, 151.4054434770023363, 1.149106048033103011 ) ) ;
#13413=CARTESIAN_POINT ( 'NONE',  ( 1.863517626568274910, -15.41251410767331720, 5.374852164437769808 ) ) ;
#13414=CARTESIAN_POINT ( 'NONE',  ( -18.16172641238603802, 140.6071502257508143, 1.752259283733317519 ) ) ;
#13415=CARTESIAN_POINT ( 'NONE',  ( 0.9436776830090995993, 12.87300645547595046, -0.2395577073833762005 ) ) ;
#13416=CARTESIAN_POINT ( 'NONE',  ( -10.68516669180073286, 157.9381250348597234, -0.6779181152352149464 ) ) ;
#13419=CARTESIAN_POINT ( 'NONE',  ( 0.7508863055360318617, -11.68651920905074348, 0.6198408032357946018 ) ) ;
#13420=ORIENTED_EDGE ( 'NONE', *, *, #7115, .T. ) ;
#13423=CARTESIAN_POINT ( 'NONE',  ( 5.925882289753468868, 120.8604418758245487, 0.3792092984231499875 ) ) ;
#13425=CARTESIAN_POINT ( 'NONE',  ( -11.89914747278639950, 128.3619849303985632, 0.5991027734528264759 ) ) ;
#13426=CARTESIAN_POINT ( 'NONE',  ( 2.309263497243444263, -14.96449433386182193, 5.702862618531368888 ) ) ;
#13427=CARTESIAN_POINT ( 'NONE',  ( 17.39219791206827992, 147.8988302317391117, -1.461875531624039493 ) ) ;
#13429=CARTESIAN_POINT ( 'NONE',  ( -19.80203545474871518, 147.6055923437354238, -2.520003004638577515 ) ) ;
#13431=FACE_OUTER_BOUND ( 'NONE', #24787, .T. ) ;
#13432=CARTESIAN_POINT ( 'NONE',  ( 3.074000544403499902, -13.70685301784095600, 1.494313880732895283 ) ) ;
#13433=CARTESIAN_POINT ( 'NONE',  ( -6.430405882401983853, 30.45907221301710877, 0.4699959139286034593 ) ) ;
#13434=CARTESIAN_POINT ( 'NONE',  ( 0.6527697516717059223, 156.3069099058775748, -0.1169209421757346490 ) ) ;
#13437=CARTESIAN_POINT ( 'NONE',  ( -3.562848200393185838, 109.2372022974361698, 3.773768304531518236 ) ) ;
#13441=CARTESIAN_POINT ( 'NONE',  ( 8.060084350832182665, 158.6724238832827609, 0.05135189671889815732 ) ) ;
#13442=CARTESIAN_POINT ( 'NONE',  ( -5.966545996697778520, 118.9610140496397719, 0.3495452691818400348 ) ) ;
#13446=CARTESIAN_POINT ( 'NONE',  ( 0.3600194693791573530, 38.02539389153889005, -1.148431998888613359 ) ) ;
#13447=CARTESIAN_POINT ( 'NONE',  ( 4.941607502190644041, 118.3881331334009985, 1.039683250452205998 ) ) ;
#13448=CARTESIAN_POINT ( 'NONE',  ( -4.487480840803009130, 27.34045677879159442, -1.100063755011520872 ) ) ;
#13449=CARTESIAN_POINT ( 'NONE',  ( 7.636339006008190822, 27.50728337528610012, -3.595707551023701765 ) ) ;
#13450=CARTESIAN_POINT ( 'NONE',  ( -2.478289490271501805, 117.4827286966103941, -0.7432425970007181526 ) ) ;
#13451=CARTESIAN_POINT ( 'NONE',  ( -2.269084004857128800, 124.1308405194309188, -0.09931761310301590040 ) ) ;
#13452=B_SPLINE_CURVE_WITH_KNOTS ( 'NONE', 3,
 ( #24580, #11390, #14577, #14996, #21797, #31407, #15421, #15207, #37383, #34201 ),
 .UNSPECIFIED., .F., .F.,
 ( 4, 2, 2, 2, 4 ),
 ( 0.0001356198500382660844, 0.001295386987695697732, 0.002455154125353129109, 0.003614921263010560919, 0.004774688400667992730 ),
 .UNSPECIFIED. ) ;
#13454=CARTESIAN_POINT ( 'NONE',  ( -3.368418438749888111, 109.1383545882859778, -3.951708265540383014 ) ) ;
#13455=CARTESIAN_POINT ( 'NONE',  ( 3.054645280121299766, 105.1240653689918645, 4.374269570515916250 ) ) ;
#13456=CARTESIAN_POINT ( 'NONE',  ( -4.631227783250409402, 22.10816835407601744, -0.05711764529929251599 ) ) ;
#13459=CARTESIAN_POINT ( 'NONE',  ( 3.282182858002726356, -14.11059071864860570, 3.604430013830858037 ) ) ;
#13460=CARTESIAN_POINT ( 'NONE',  ( 2.162440637018669065, 123.3349985135950959, -0.07568789353404296871 ) ) ;
#13461=CARTESIAN_POINT ( 'NONE',  ( -20.72298665840535037, 132.2482564273973935, 0.5730191400310229444 ) ) ;
#13466=CYLINDRICAL_SURFACE ( 'NONE', #3623, 5.588000000000006295 ) ;
#13467=CARTESIAN_POINT ( 'NONE',  ( 5.836094479182562189, -14.94293577981173371, 0.6207079514943552034 ) ) ;
#13468=CARTESIAN_POINT ( 'NONE',  ( -19.50252919055214207, 149.6234262069624492, 1.702160239338572634 ) ) ;
#13469=CARTESIAN_POINT ( 'NONE',  ( 7.954494586186791061, 118.5968412048868288, -0.8561882949445157598 ) ) ;
#13471=CARTESIAN_POINT ( 'NONE',  ( 0.9679928046509989059, 27.93285725408814812, -0.1178628334679577422 ) ) ;
#13475=CARTESIAN_POINT ( 'NONE',  ( 0.1664298668078588450, 110.3683645023726427, 3.586750284817682211 ) ) ;
#13476=CARTESIAN_POINT ( 'NONE',  ( -4.645572480595541620, 117.9340260526530813, 0.7769932229682322555 ) ) ;
#13477=CARTESIAN_POINT ( 'NONE',  ( -8.784047514290692860, 154.8283212766472445, 1.235621501372049735 ) ) ;
#13480=CARTESIAN_POINT ( 'NONE',  ( 18.13417818756197519, 144.6555253171603397, -1.679261103697790913 ) ) ;
#13481=CARTESIAN_POINT ( 'NONE',  ( -13.21388725472906955, 155.5383117973235585, -2.112422614401994636 ) ) ;
#13485=CARTESIAN_POINT ( 'NONE',  ( 4.378236034317057879, 118.1843938197233683, -0.4336838323394221484 ) ) ;
#13486=CARTESIAN_POINT ( 'NONE',  ( 15.50313878892739972, 143.5853813351167219, -0.4270882868188063952 ) ) ;
#13488=CARTESIAN_POINT ( 'NONE',  ( -9.288997298956406468, 155.0893615026619159, -1.903066234436350701 ) ) ;
#13489=CARTESIAN_POINT ( 'NONE',  ( 2.352443540978347958, -15.20488079220741540, 4.935102241435597392 ) ) ;
#13493=CARTESIAN_POINT ( 'NONE',  ( 4.428293322310913993, 12.87204911218450576, 1.319288874004734158 ) ) ;
#13494=CARTESIAN_POINT ( 'NONE',  ( 17.19591734316806608, 148.1877419978735873, 2.150982665507991776 ) ) ;
#13495=CARTESIAN_POINT ( 'NONE',  ( 2.996590608344533280, 39.20946620154573026, -0.5752477518260917799 ) ) ;
#13496=CARTESIAN_POINT ( 'NONE',  ( 3.043391175932955495, 18.63480288530714191, -3.501419995799015528 ) ) ;
#13497=CARTESIAN_POINT ( 'NONE',  ( 12.91493749300776095, 133.8340822528099636, 0.3749514369420006155 ) ) ;
#13500=CARTESIAN_POINT ( 'NONE',  ( -2.182713281679669937, 116.1939960727429622, -0.1100263013286016944 ) ) ;
#13501=DIRECTION ( 'NONE',  ( -4.017660918040594346E-17, 1.000000000000000000, 2.376309959284834438E-19 ) ) ;
#13503=CARTESIAN_POINT ( 'NONE',  ( -6.034489779195991079E-14, 75.78546620154573077, 9.392091281095912196E-17 ) ) ;
#13510=CARTESIAN_POINT ( 'NONE',  ( -10.74909004363699161, 157.9381345072164038, 0.1376009798949089924 ) ) ;
#13513=CARTESIAN_POINT ( 'NONE',  ( 6.973621732378568971, 121.9497932120239199, 0.04315832297541429691 ) ) ;
#13516=CARTESIAN_POINT ( 'NONE',  ( -4.232597188052773518, 155.8470599587123502, -0.1762653075193722496 ) ) ;
#13517=CARTESIAN_POINT ( 'NONE',  ( 3.633732803939692335, -15.12841498804032270, 5.400629595854979037 ) ) ;
#13519=CARTESIAN_POINT ( 'NONE',  ( -4.984194916311549761, 158.4862278396301178, 1.425929471103634549 ) ) ;
#13520=CARTESIAN_POINT ( 'NONE',  ( -4.349660437102230048, 31.17966527223318707, -1.615541842050199461 ) ) ;
#13521=CARTESIAN_POINT ( 'NONE',  ( 4.777924661806521200, 116.8922783744782379, 0.3800144224740277243 ) ) ;
#13522=CARTESIAN_POINT ( 'NONE',  ( 15.76634901350801243, 146.5666095545782071, 0.5163113226649066467 ) ) ;
#13524=CARTESIAN_POINT ( 'NONE',  ( -0.9385480264228447389, -6.289884363042010484, -0.2871545319985167044 ) ) ;
#13525=CARTESIAN_POINT ( 'NONE',  ( -0.9036256862536363732, 116.4850453793277865, -0.1155468115323371875 ) ) ;
#13526=DIRECTION ( 'NONE',  ( -0.9998004120163608288, 0.000000000000000000, -0.01997839162482749342 ) ) ;
#13528=EDGE_LOOP ( 'NONE', ( #8762, #13250, #25957, #37937, #30193 ) ) ;
#13529=CARTESIAN_POINT ( 'NONE',  ( 2.225071688287161287, 116.2692689860753603, 0.1766109378387185069 ) ) ;
#13530=VERTEX_POINT ( 'NONE', #33887 ) ;
#13531=CARTESIAN_POINT ( 'NONE',  ( -18.15383854178437417, 147.5382818419693649, 1.618175512470155342 ) ) ;
#13533=CARTESIAN_POINT ( 'NONE',  ( 18.77683424009538626, 152.0234722879370111, 2.226617664588433243 ) ) ;
#13534=CARTESIAN_POINT ( 'NONE',  ( 2.527692779614272744, 158.0185616612000956, -1.624164342510254988 ) ) ;
#13535=CARTESIAN_POINT ( 'NONE',  ( -0.8880852245287531588, 7.049514723814470862, -0.3999422104893632923 ) ) ;
#13536=CARTESIAN_POINT ( 'NONE',  ( -14.46681479972627926, 121.7426775721902175, -1.517288920005034791 ) ) ;
#13537=CARTESIAN_POINT ( 'NONE',  ( 4.621803021457706606, 118.0614903755723049, -0.5437508832788947588 ) ) ;
#13538=CARTESIAN_POINT ( 'NONE',  ( 5.032151674051235979, 104.6144662015512381, 1.777523892075001388 ) ) ;
#13539=CARTESIAN_POINT ( 'NONE',  ( 16.48541106618845831, 147.8801373804967341, -1.108338632072817243 ) ) ;
#13540=CARTESIAN_POINT ( 'NONE',  ( -1.563936845556568089, 156.2577446057484281, -0.001723203835320021677 ) ) ;
#13541=ORIENTED_EDGE ( 'NONE', *, *, #29947, .F. ) ;
#13542=CARTESIAN_POINT ( 'NONE',  ( -6.601024023181220279, 120.1594786313440011, -1.214938174674062621 ) ) ;
#13543=CARTESIAN_POINT ( 'NONE',  ( 5.240434970354078459, -15.39321860721029545, 1.015353449650246764 ) ) ;
#13544=DIRECTION ( 'NONE',  ( 4.017660918040594346E-17, -1.000000000000000000, -2.376309959284834438E-19 ) ) ;
#13545=CARTESIAN_POINT ( 'NONE',  ( -4.600069725331597859, 118.0596821417892954, -0.7231468346112266410 ) ) ;
#13548=CARTESIAN_POINT ( 'NONE',  ( 10.38552121992528399, 122.0805278159965610, 1.592441429402150055 ) ) ;
#13549=CYLINDRICAL_SURFACE ( 'NONE', #15455, 0.5080000000000002292 ) ;
#13550=CIRCLE ( 'NONE', #16944, 3.683000000000001162 ) ;
#13551=CARTESIAN_POINT ( 'NONE',  ( 1.794468298957800689, 116.4672891243423578, 0.03585774721038192947 ) ) ;
#13552=CARTESIAN_POINT ( 'NONE',  ( 0.01634572621781915994, 29.22912819268679030, -8.429653881604959764 ) ) ;
#13553=CARTESIAN_POINT ( 'NONE',  ( 4.372087114477248626, 155.8497297829079571, 0.6179351164228052973 ) ) ;
#13554=CARTESIAN_POINT ( 'NONE',  ( 2.899870334229791791, 116.9538966677400254, -0.3598414239652114044 ) ) ;
#13558=CARTESIAN_POINT ( 'NONE',  ( 0.1700004239520251370, 118.7629491485454025, 1.279869604491548296 ) ) ;
#13559=CARTESIAN_POINT ( 'NONE',  ( -20.69945920510674142, 152.5542719854981044, -0.3887601451951301912 ) ) ;
#13561=CARTESIAN_POINT ( 'NONE',  ( 6.724651104264945722, 120.8999252434172291, -0.7604862180030697028 ) ) ;
#13562=CARTESIAN_POINT ( 'NONE',  ( 6.475684456959278634, -13.49251406434824574, 0.1304084665236045215 ) ) ;
#13563=CARTESIAN_POINT ( 'NONE',  ( -4.292261259499774440, 155.8363458669846864, -0.4108933393057503380 ) ) ;
#13564=CARTESIAN_POINT ( 'NONE',  ( 3.919216764667305064, -12.20455369412110080, 1.363517133079271026 ) ) ;
#13565=CARTESIAN_POINT ( 'NONE',  ( -19.81309253913748947, 152.3633698111425758, 1.013446639353942968 ) ) ;
#13567=CARTESIAN_POINT ( 'NONE',  ( 16.27462974253330685, 121.4070763266325628, 0.3766275504196341939 ) ) ;
#13569=VERTEX_POINT ( 'NONE', #14264 ) ;
#13570=CARTESIAN_POINT ( 'NONE',  ( 4.586363120317823672, -1.655842793181455663, -0.6244342276643227718 ) ) ;
#13571=CARTESIAN_POINT ( 'NONE',  ( -15.73471677569744287, 120.8416612192341972, -0.3144170877231854955 ) ) ;
#13572=DIRECTION ( 'NONE',  ( -0.01997839162482761832, -1.040247600000950455E-18, 0.9998004120163610509 ) ) ;
#13573=CARTESIAN_POINT ( 'NONE',  ( 2.780396738703073911, 107.4069940011556383, 4.543958154617097733 ) ) ;
#13574=CARTESIAN_POINT ( 'NONE',  ( 8.061196390534837164, 121.1687499546863336, 1.293492009120990716 ) ) ;
#13575=AXIS2_PLACEMENT_3D ( 'NONE', #1018, #805, #1433 ) ;
#13576=CARTESIAN_POINT ( 'NONE',  ( 2.901706292870370518, -4.507343114274551255, -3.632229383212865592 ) ) ;
#13577=CARTESIAN_POINT ( 'NONE',  ( 15.68124023389185240, 122.9504679175852573, 1.501494826411870154 ) ) ;
#13578=CARTESIAN_POINT ( 'NONE',  ( 15.26262975083392170, 148.0175730703490160, 0.3049836654617371079 ) ) ;
#13580=CARTESIAN_POINT ( 'NONE',  ( 9.025716902755924309, 119.5326672034033777, -1.052790416315139144 ) ) ;
#13581=CARTESIAN_POINT ( 'NONE',  ( 2.198398128136354934, 2.077049112184502278, 4.064154346441791965 ) ) ;
#13582=CARTESIAN_POINT ( 'NONE',  ( -2.899385524442621875, 117.0242007548465608, -0.5112881796358939024 ) ) ;
#13583=ORIENTED_EDGE ( 'NONE', *, *, #42077, .T. ) ;
#13584=CARTESIAN_POINT ( 'NONE',  ( -4.305249565653826771, 155.8363458669846864, 0.2390946120805821085 ) ) ;
#13585=CARTESIAN_POINT ( 'NONE',  ( 5.253367374056280070, -14.88852847978991356, 3.689182801501961428 ) ) ;
#13587=CARTESIAN_POINT ( 'NONE',  ( -0.1908661700457686961, 105.7852372209750200, -5.338925892754766700 ) ) ;
#13588=ORIENTED_EDGE ( 'NONE', *, *, #41797, .F. ) ;
#13589=CARTESIAN_POINT ( 'NONE',  ( 9.864431837517868118, 120.7895603300898699, 1.595968683908904007 ) ) ;
#13592=CARTESIAN_POINT ( 'NONE',  ( -20.00278215841964524, 152.4248492066682559, 0.8711105393690440346 ) ) ;
#13593=CARTESIAN_POINT ( 'NONE',  ( 8.378134419073882455, 22.78949214230337006, 1.148743996083190888 ) ) ;
#13595=CARTESIAN_POINT ( 'NONE',  ( 16.02795213054438506, 143.8376908863262997, 1.609587254066635387 ) ) ;
#13596=CIRCLE ( 'NONE', #40127, 5.080000000000006288 ) ;
#13597=CARTESIAN_POINT ( 'NONE',  ( 1.900581966505874076, 116.7132768022172797, -0.2320997050762015623 ) ) ;
#13603=CARTESIAN_POINT ( 'NONE',  ( -4.496964070084271903, 118.1160052686005457, 0.5628395517699180672 ) ) ;
#13605=B_SPLINE_CURVE_WITH_KNOTS ( 'NONE', 3,
 ( #21069, #14887, #8304, #37696, #18499, #24271, #21274, #11079, #40897, #11701, #27272, #33885, #34304, #28097, #24904, #8725, #37903, #41109, #17668, #30668, #24688, #5133, #21686, #4922, #40287, #1516, #37276, #5334, #8518, #21476, #18289, #34508, #34094, #17877, #11915, #30880, #34711, #1721, #14677, #27683, #24474, #35551, #41322, #2562, #25115, #32344, #35336, #22522, #15934 ),
 .UNSPECIFIED., .F., .F.,
 ( 4, 1, 1, 1, 1, 1, 1, 1, 1, 1, 1, 1, 1, 1, 1, 1, 1, 1, 1, 1, 1, 1, 1, 1, 1, 1, 1, 1, 1, 1, 1, 1, 1, 1, 1, 1, 1, 1, 1, 1, 1, 1, 1, 1, 1, 1, 4 ),
 ( 0.000000000000000000, 0.007812500000000000000, 0.01562500000000000000, 0.02343750000000000000, 0.03125000000000000000, 0.04687500000000000000, 0.06250000000000000000, 0.07812500000000000000, 0.09375000000000000000, 0.1093750000000000000, 0.1250000000000000000, 0.1406250000000000000, 0.1562500000000000000, 0.1875000000000000000, 0.2187500000000000000, 0.2500000000000000000, 0.2812500000000000000, 0.3125000000000000000, 0.3281250000000000000, 0.3437500000000000000, 0.3750000000000000000, 0.4062500000000000000, 0.4375000000000000000, 0.4687500000000000000, 0.5000000000000000000, 0.5312500000000000000, 0.5625000000000000000, 0.5937500000000000000, 0.6250000000000000000, 0.6562500000000000000, 0.6718750000000000000, 0.6875000000000000000, 0.7187500000000000000, 0.7500000000000000000, 0.7812500000000000000, 0.8125000000000000000, 0.8437500000000000000, 0.8750000000000000000, 0.8906250000000000000, 0.9062500000000000000, 0.9218750000000000000, 0.9375000000000000000, 0.9531250000000000000, 0.9687500000000000000, 0.9765625000000000000, 0.9843750000000000000, 1.000000000000000000 ),
 .UNSPECIFIED. ) ;
#13609=CARTESIAN_POINT ( 'NONE',  ( -8.283754562202487293, 120.0681802063006671, -1.449964621888376159 ) ) ;
#13610=CARTESIAN_POINT ( 'NONE',  ( -6.667064533335244292, 121.2389289720308199, -0.3413157713140473892 ) ) ;
#13611=CARTESIAN_POINT ( 'NONE',  ( 4.547318138317117509, 118.0745339805481109, 0.7854269464174529203 ) ) ;
#13612=CARTESIAN_POINT ( 'NONE',  ( -12.19070665030426071, 151.9982576965888654, -1.154562729007634569 ) ) ;
#13614=CARTESIAN_POINT ( 'NONE',  ( 4.811878810637661097, 117.9496053154559689, -0.9251022342672158283 ) ) ;
#13615=CARTESIAN_POINT ( 'NONE',  ( 7.328771362700555514, 123.0350022594044219, 0.07777345538051000373 ) ) ;
#13616=CARTESIAN_POINT ( 'NONE',  ( -13.72925640114938872, 131.0408573235120571, -1.723107598632782844 ) ) ;
#13617=CARTESIAN_POINT ( 'NONE',  ( -0.002459394113084579191, 156.3065584682211124, 0.1230781383047673677 ) ) ;
#13618=CARTESIAN_POINT ( 'NONE',  ( 7.882738460396603308, 122.2119657951149918, -0.4812898729222590544 ) ) ;
#13619=CARTESIAN_POINT ( 'NONE',  ( -9.096994273319783275, 153.9681518559695803, -0.06573532333832052266 ) ) ;
#13620=CARTESIAN_POINT ( 'NONE',  ( -4.515506726787251068, -6.291224493951820484, 1.111903093310195212 ) ) ;
#13621=CARTESIAN_POINT ( 'NONE',  ( 5.832486214875661545, 117.3024554866451865, 0.6456718139904971121 ) ) ;
#13623=CARTESIAN_POINT ( 'NONE',  ( 3.134532381368876575, -15.16579696257060128, 3.749817985361381112 ) ) ;
#13624=CARTESIAN_POINT ( 'NONE',  ( -13.18164045127540440, 153.9517556018257096, 1.734949727869876002 ) ) ;
#13625=CARTESIAN_POINT ( 'NONE',  ( 0.9708619386763404080, 12.65153173543952470, -0.1022289352641109206 ) ) ;
#13626=CARTESIAN_POINT ( 'NONE',  ( -22.96526709448186310, 149.8455236008688303, -1.052246632350672506 ) ) ;
#13627=CARTESIAN_POINT ( 'NONE',  ( -0.8940008744714061928, 26.26452439613007428, -0.3861867617640990513 ) ) ;
#13631=CARTESIAN_POINT ( 'NONE',  ( 7.618479139564604985, 124.9344662015457317, 0.1522353441811855612 ) ) ;
#13632=CARTESIAN_POINT ( 'NONE',  ( -4.498274173886023242, 155.8822484669112214, 0.6329996689149903766 ) ) ;
#13633=CARTESIAN_POINT ( 'NONE',  ( 3.392078256862109953, -14.39927144874259035, 5.014931565121842461 ) ) ;
#13634=CARTESIAN_POINT ( 'NONE',  ( 9.055011062051939064, 121.9018297702777858, -0.9711463333382074348 ) ) ;
#13635=CARTESIAN_POINT ( 'NONE',  ( -7.562035183886322898, 119.9600249249614592, -1.380075063195379093 ) ) ;
#13636=CARTESIAN_POINT ( 'NONE',  ( -0.2157595710058203831, 104.6144662015457243, 4.831689807522736579 ) ) ;
#13637=CARTESIAN_POINT ( 'NONE',  ( 3.025122737553283869, -13.62787997529110662, 1.286645544439679156 ) ) ;
#13638=CARTESIAN_POINT ( 'NONE',  ( -4.967168320455268571, 117.4023968188195681, -1.002192383175803503 ) ) ;
#13639=CARTESIAN_POINT ( 'NONE',  ( 0.002459394112955782911, 156.3065584682211124, -0.1230781383047671457 ) ) ;
#13642=CARTESIAN_POINT ( 'NONE',  ( -4.555615850703588876, 110.9173261774677712, 2.841647770357901504 ) ) ;
#13643=CARTESIAN_POINT ( 'NONE',  ( 2.278431206749268245, 107.0260912999229390, 4.818171318492614041 ) ) ;
#13644=DIRECTION ( 'NONE',  ( 4.017660918040594346E-17, -1.000000000000000000, -2.376309959284834438E-19 ) ) ;
#13645=CIRCLE ( 'NONE', #24514, 5.588000000000006295 ) ;
#13647=CARTESIAN_POINT ( 'NONE',  ( 4.745947329130571823, 116.7839080817633430, -0.02307940527355892280 ) ) ;
#13649=CARTESIAN_POINT ( 'NONE',  ( -5.946884660761687869, 118.9717589635377664, 0.3494607991981762418 ) ) ;
#13652=CARTESIAN_POINT ( 'NONE',  ( -6.507153519498132566E-14, 76.29346620154572634, 3.067795752821199360E-29 ) ) ;
#13654=CARTESIAN_POINT ( 'NONE',  ( -4.399413851824025556, 32.38558793863810337, 0.9715087743876699156 ) ) ;
#13655=CARTESIAN_POINT ( 'NONE',  ( 20.10299018766027146, 141.3454246894093274, 2.438971827487009580 ) ) ;
#13656=CARTESIAN_POINT ( 'NONE',  ( -4.596079559025361583, 18.26954911218466648, 0.4757704999388879807 ) ) ;
#13657=CARTESIAN_POINT ( 'NONE',  ( 0.8142577860443056537, 14.98675861574836077, 8.418590528086960845 ) ) ;
#13658=CARTESIAN_POINT ( 'NONE',  ( 5.509788357450847940, 117.4222437278462223, -0.6928894233252995694 ) ) ;
#13659=CARTESIAN_POINT ( 'NONE',  ( -2.216013192100319884, 123.7320667226965867, -0.1296889073052085173 ) ) ;
#13660=CARTESIAN_POINT ( 'NONE',  ( 4.810181142648978891, 117.4081489754564274, 1.190371033444491244 ) ) ;
#13662=CARTESIAN_POINT ( 'NONE',  ( -0.003073426022617897335, 123.4679809879534247, 0.1538068059577180902 ) ) ;
#13663=CARTESIAN_POINT ( 'NONE',  ( 1.790774717077139089, 25.13178105314743860, 4.274281468382033822 ) ) ;
#13665=CARTESIAN_POINT ( 'NONE',  ( -23.45208337669106058, 146.8499405025503961, -0.4686284387228000226 ) ) ;
#13666=CARTESIAN_POINT ( 'NONE',  ( 1.878022632408997250, -15.11918648689831990, 5.509382895440600336 ) ) ;
#13667=CARTESIAN_POINT ( 'NONE',  ( 3.706399805698057826, 113.7286232773062125, -2.153009399082070452 ) ) ;
#13668=CARTESIAN_POINT ( 'NONE',  ( -20.86923087398519172, 132.2939277659177151, 0.4710007621541096867 ) ) ;
#13669=ADVANCED_FACE ( 'NONE', ( #34306 ), #27274, .T. ) ;
#13671=ORIENTED_EDGE ( 'NONE', *, *, #17305, .F. ) ;
#13673=EDGE_LOOP ( 'NONE', ( #21861, #21305 ) ) ;
#13674=CARTESIAN_POINT ( 'NONE',  ( -2.803395127021860223, 31.26063551530791074, 0.8708390753670086637 ) ) ;
#13675=CARTESIAN_POINT ( 'NONE',  ( 5.293312112441732609, -15.32963308811979886, 0.4416779358531437993 ) ) ;
#13676=CARTESIAN_POINT ( 'NONE',  ( -0.4598942929540284497, 118.4074432378348689, 0.5883637925338035535 ) ) ;
#13677=CARTESIAN_POINT ( 'NONE',  ( 15.22748671137934551, 123.1171956318823533, -1.061527106655570707 ) ) ;
#13678=CARTESIAN_POINT ( 'NONE',  ( 4.560443952884764229, -11.68867000232777542, 0.6947937212093100445 ) ) ;
#13681=CARTESIAN_POINT ( 'NONE',  ( -4.810636611593423595, 117.4081599864878598, -1.190287313834438532 ) ) ;
#13682=CARTESIAN_POINT ( 'NONE',  ( 0.08587196332404170573, 108.5751225745497806, 4.267111774705385052 ) ) ;
#13684=B_SPLINE_SURFACE_WITH_KNOTS ( 'NONE', 3, 3, ( 
 ( #40350, #17528, #20929, #7961, #7544, #4569, #14326, #14541, #30735, #27338, #30529, #26915, #27550, #33953, #24131, #40556, #33533, #33320, #39929, #17325, #4784, #24543, #953, #24340, #37344, #27125, #1159, #8164, #21132, #7334, #4988, #30948, #1788, #27751 ),
 ( #40761, #13921, #20292, #14124, #37976, #5405, #8801, #38195, #28175, #18997, #11772, #15384, #2633, #41824, #5620, #1995, #21548, #41180, #21760, #12416, #32001, #34365, #18361, #28808, #11983, #8374, #28389, #9221, #31795, #18576, #12200, #35008, #15592, #38410 ),
 ( #22179, #21339, #2840, #15799, #41395, #24763, #34578, #37761, #34786, #24977, #14958, #31585, #28597, #31156, #35209, #2423, #6036, #27959, #9011, #31367, #25191, #15169, #41606, #25408, #21976, #5828, #12618, #37550, #2210, #18783, #5198, #18152, #40968, #8585 ),
 ( #274, #16429, #16857, #19209, #6655, #13460, #23227, #39451, #9629, #32632, #13030, #6239, #29435, #3893, #29649, #60, #22596, #26020, #19833, #6442, #36260, #22387, #38818, #36047, #33062, #39029, #32847, #3679, #12822, #13248, #29007, #32217, #29218, #16641 ),
 ( #487, #695, #3253, #39236, #26232, #9837, #19619, #35628, #10046, #35411, #19417, #20044, #3050, #32423, #22803, #23018, #29857, #10254, #6861, #35840, #25605, #16008, #16213, #3467, #26448, #7080, #38614, #42024, #25809, #9419, #36678, #33488, #23658, #27082 ),
 ( #7915, #23873, #30480, #11099, #33906, #14491, #17484, #23439, #26872, #14079, #904, #33275, #39879, #21089, #26659, #4317, #20880, #13878, #10676, #36468, #4521, #4734, #24291, #40306, #7711, #10885, #7499, #1324, #20459, #14281, #27291, #7287, #17686, #17899 ),
 ( #40090, #17064, #20249, #17281, #30067, #36893, #30270, #20673, #1112, #11306, #1536, #33697, #24087, #4104, #37097, #30686, #27504, #40512, #37296, #8115, #34113, #4940, #30902, #13667, #39666, #10471, #2584, #11934, #34953, #31740, #14907, #8324, #18310, #9170 ),
 ( #37499, #24926, #15544, #41554, #28546, #27910, #8747, #31312, #24495, #5564, #22126, #5776, #2156, #40917, #15116, #38143, #24710, #12362, #40712, #11723, #12147, #35156, #28119, #8956, #21923, #31111, #18521, #5151, #21295, #5357, #18730, #18945, #41128, #25350 ),
 ( #15329, #31527, #37924, #21709, #37715, #2371, #11508, #8538, #38353, #34323, #21498, #34733, #41345, #5982, #1741, #25139, #28336, #14700, #18106, #34531, #27705, #1948, #432, #32795, #38557, #32161, #15955, #12768, #9576, #41969, #3195, #29599, #25552, #16375 ),
 ( #29380, #9991, #3626, #35783, #41765, #2995, #32367, #19156, #9370, #28951, #39398, #2790, #22545, #26179, #25758, #38765, #12565, #22751, #22963, #13403, #220, #25967, #29162, #35574, #6597, #6392, #19566, #32575, #22334, #35992, #36205, #3407, #28752, #8 ),
 ( #13195, #19362, #39182, #6806, #19775, #12974, #16158, #38975, #9783, #35357, #6187, #16591, #26393, #10200, #23171, #7027, #31951, #15747, #7864, #20404, #646, #40462, #40252, #20826, #30220, #11046, #33851, #33224, #26605, #36626, #27446, #20198, #36420, #17636 ),
 ( #4679, #4051, #27031, #7446, #13615, #23816, #11252, #24031, #33434, #17012, #4261, #14230, #850, #30638, #16804, #30011, #30427, #24236, #17224, #27238, #37047, #7238, #36837, #23388, #39612, #23605, #1481, #37246, #1060, #14437, #19994, #13824, #33012, #3840 ) ),
 .UNSPECIFIED., .F., .F., .F.,
 ( 4, 1, 1, 1, 1, 1, 3, 4 ),
 ( 4, 1, 1, 1, 1, 1, 1, 1, 1, 1, 1, 1, 1, 1, 1, 1, 1, 1, 1, 2, 1, 1, 1, 1, 1, 1, 1, 1, 1, 1, 4 ),
 ( 0.000000000000000000, 0.1666666666666666574, 0.2500000000000000000, 0.5000000000000000000, 0.5555555555555555802, 0.7500000000000000000, 1.000000000000000000, 1.010000000000000009 ),
 ( 0.000000000000000000, 0.02126250000000000015, 0.04252500000000000030, 0.06378749999999999698, 0.08505000000000000060, 0.1063125000000000042, 0.1275749999999999940, 0.1488374999999999837, 0.1701000000000000012, 0.1913624999999999909, 0.2126250000000000084, 0.2338874999999999704, 0.2551500000000000434, 0.2764124999999999499, 0.2870437499999999864, 0.2976749999999999674, 0.3083062500000000039, 0.3189375000000000404, 0.3295687499999999659, 0.3402000000000000024, 0.4226750000000000229, 0.5051499999999999879, 0.5876249999999998419, 0.6700999999999999179, 0.7525749999999999940, 0.7938125000000000320, 0.8350499999999999590, 0.8762874999999994419, 0.9175249999999994799, 0.9587624999999999620, 1.000000000000000000 ),
 .UNSPECIFIED. ) ;
#13685=CARTESIAN_POINT ( 'NONE',  ( -17.03734119261612889, 146.7604995623492243, 1.248076303867124093 ) ) ;
#13687=CARTESIAN_POINT ( 'NONE',  ( 18.71424449056243233, 147.4429432625130119, -1.699796950208447788 ) ) ;
#13689=CARTESIAN_POINT ( 'NONE',  ( -7.783141725463827321, 119.0983413489662297, -1.312215641098251950 ) ) ;
#13691=ORIENTED_EDGE ( 'NONE', *, *, #20230, .F. ) ;
#13692=CARTESIAN_POINT ( 'NONE',  ( 4.429221712000376954, 118.1654444364263128, -0.4667334324146756863 ) ) ;
#13693=EDGE_CURVE ( 'NONE', #1790, #6660, #12529, .T. ) ;
#13694=CARTESIAN_POINT ( 'NONE',  ( 9.185752227574047524, 123.6526633469202920, -0.3199782652467453303 ) ) ;
#13696=CARTESIAN_POINT ( 'NONE',  ( 2.867866294591228993, -15.05265924143639467, 4.220695585399262484 ) ) ;
#13699=CARTESIAN_POINT ( 'NONE',  ( -4.556395268149300293, 8.773967715207941609, 0.7749943352582737699 ) ) ;
#13700=CARTESIAN_POINT ( 'NONE',  ( 4.324763564747695632, 120.2039194668847699, 0.7996884002708145589 ) ) ;
#13701=CARTESIAN_POINT ( 'NONE',  ( 2.988133089223356187, 39.20946620154573026, -0.1519989107391659100 ) ) ;
#13702=AXIS2_PLACEMENT_3D ( 'NONE', #34339, #11526, #14505 ) ;
#13704=CARTESIAN_POINT ( 'NONE',  ( 1.111903444298625754, 15.29877551736591812, 4.515507465039587665 ) ) ;
#13705=CARTESIAN_POINT ( 'NONE',  ( 3.737471135337817607, 121.0798372856833538, 0.1416028149587414686 ) ) ;
#13706=CARTESIAN_POINT ( 'NONE',  ( -4.522151473809593369, 110.7919029432140974, 2.894729270667253829 ) ) ;
#13708=CARTESIAN_POINT ( 'NONE',  ( -8.784945553904831783, 117.7269525811338013, -0.3943082114503992930 ) ) ;
#13709=CARTESIAN_POINT ( 'NONE',  ( -1.028573857428271010, 117.3993836102140449, 1.440221441096896315 ) ) ;
#13710=AXIS2_PLACEMENT_3D ( 'NONE', #35504, #22894, #6958 ) ;
#13712=CARTESIAN_POINT ( 'NONE',  ( -5.078986093043186045, 81.62746620154572952, -0.1014902294541231709 ) ) ;
#13714=DIRECTION ( 'NONE',  ( -5.206863593109713661E-17, 1.000000000000000000, -1.077750396879097183E-30 ) ) ;
#13718=CARTESIAN_POINT ( 'NONE',  ( -18.44111676445476888, 125.1790410860780298, 0.1047302884851513127 ) ) ;
#13721=CARTESIAN_POINT ( 'NONE',  ( 7.791856601383843284, 122.6038259070386687, 0.04541553377301332101 ) ) ;
#13723=CARTESIAN_POINT ( 'NONE',  ( 3.653205933764129831, 115.7029491755316712, -1.478537451617223386 ) ) ;
#13724=CARTESIAN_POINT ( 'NONE',  ( -15.76280660274407808, 145.9085485750152316, -0.3664889719343313867 ) ) ;
#13725=CARTESIAN_POINT ( 'NONE',  ( 4.840206765044483994, -15.05961300585426166, 4.264492456498921946 ) ) ;
#13727=CARTESIAN_POINT ( 'NONE',  ( -11.93281433870470742, 156.4809912657682673, 1.479000486392927138 ) ) ;
#13728=CARTESIAN_POINT ( 'NONE',  ( 3.655561289726139140, 27.93047918286777076, -2.829280713513928180 ) ) ;
#13729=CARTESIAN_POINT ( 'NONE',  ( 21.82265835376359675, 151.4369626909183637, 0.8820245880042207887 ) ) ;
#13730=CARTESIAN_POINT ( 'NONE',  ( 12.76659075803674348, 133.6868103333486602, 0.4399761219218703556 ) ) ;
#13732=CARTESIAN_POINT ( 'NONE',  ( 0.9340445150430609633, -0.5783478219614121008, -0.2901879621234355056 ) ) ;
#13733=CARTESIAN_POINT ( 'NONE',  ( -0.3088162040007921827, 116.5752054743899038, -0.1648661904198056027 ) ) ;
#13737=CARTESIAN_POINT ( 'NONE',  ( 2.232464228204602996, 116.2826474796002287, 0.1929315044139254531 ) ) ;
#13738=CARTESIAN_POINT ( 'NONE',  ( -13.85609184427570995, 152.5163154464351294, 1.589750347114884166 ) ) ;
#13740=CARTESIAN_POINT ( 'NONE',  ( 21.26307135201298948, 148.5140355411650717, 2.311892396764664070 ) ) ;
#13741=CARTESIAN_POINT ( 'NONE',  ( 4.169621149806018501, 118.9132445967212419, -0.8414384147219282628 ) ) ;
#13742=CARTESIAN_POINT ( 'NONE',  ( 0.7725557299734273631, -15.30006921971679112, -0.5871674697799584841 ) ) ;
#13743=AXIS2_PLACEMENT_3D ( 'NONE', #30886, #7486, #4927 ) ;
#13744=CARTESIAN_POINT ( 'NONE',  ( -20.53318969041758635, 136.3738900553462372, -2.061127768630951707 ) ) ;
#13745=CARTESIAN_POINT ( 'NONE',  ( 4.652316817438794772, 118.0213487410945845, -0.6399539048371912786 ) ) ;
#13747=CARTESIAN_POINT ( 'NONE',  ( 6.515494676151939224, 155.4519854478747902, -0.9200225795255460026 ) ) ;
#13748=CARTESIAN_POINT ( 'NONE',  ( -9.049782359939607446, 124.0675141969884692, -0.1808361888366264991 ) ) ;
#13750=CARTESIAN_POINT ( 'NONE',  ( -9.495519422240835894, 121.2752502669211339, -1.536911970732435462 ) ) ;
#13751=CARTESIAN_POINT ( 'NONE',  ( 1.959965285483297404, -15.65532139403495648, 5.519319896091174904 ) ) ;
#13752=CARTESIAN_POINT ( 'NONE',  ( -4.559029627764906500, 31.49133049583777932, -0.6947656260690758812 ) ) ;
#13753=CARTESIAN_POINT ( 'NONE',  ( -4.584608287924823777, 117.9735455925265768, -0.9262146779261964946 ) ) ;
#13755=CARTESIAN_POINT ( 'NONE',  ( 4.065926199369043204, 118.2429491485453354, 0.3080910687088499467 ) ) ;
#13756=CARTESIAN_POINT ( 'NONE',  ( 5.042934966769523797, 119.7208665877771665, 1.041708725922360523 ) ) ;
#13758=CARTESIAN_POINT ( 'NONE',  ( 18.63504953328963154, 154.1157618415863624, 0.3723726386282266709 ) ) ;
#13759=CARTESIAN_POINT ( 'NONE',  ( 4.559522851259544041, 6.111780172613243245, 7.100340242056582873 ) ) ;
#13760=CARTESIAN_POINT ( 'NONE',  ( 4.509850150708832217, 121.0527503406816123, 0.3565835012282698169 ) ) ;
#13761=CARTESIAN_POINT ( 'NONE',  ( 3.898136962790617943, 117.1932757116604762, -0.4670938640342005010 ) ) ;
#13762=CARTESIAN_POINT ( 'NONE',  ( -6.501940248589056060E-14, 66.13346620154574396, -9.529289869050788486E-18 ) ) ;
#13764=CARTESIAN_POINT ( 'NONE',  ( 1.378659152591106274, 115.6909491485452719, 1.738311037673413662 ) ) ;
#13766=CARTESIAN_POINT ( 'NONE',  ( -23.11138188961087891, 149.8995197111492814, -0.3848215369211049897 ) ) ;
#13768=CARTESIAN_POINT ( 'NONE',  ( -8.019101373013308276, 121.3809242941630373, -1.222737436254428545 ) ) ;
#13771=CARTESIAN_POINT ( 'NONE',  ( -11.96402413561931155, 151.9649008058812569, -0.7942868072307402993 ) ) ;
#13772=CARTESIAN_POINT ( 'NONE',  ( 2.933303798676236696, -14.66982100897798524, 5.370674165220748364 ) ) ;
#13773=CARTESIAN_POINT ( 'NONE',  ( -22.10195095183553349, 148.8299554149626260, 1.146864445019731393 ) ) ;
#13774=DIRECTION ( 'NONE',  ( -4.017660918040594346E-17, 1.000000000000000000, 2.376309959284834438E-19 ) ) ;
#13775=CARTESIAN_POINT ( 'NONE',  ( 20.46883641438825308, 129.0748834149669904, 0.4693348210411831811 ) ) ;
#13776=ORIENTED_EDGE ( 'NONE', *, *, #21226, .F. ) ;
#13777=CARTESIAN_POINT ( 'NONE',  ( -1.214995109038484067, 0.9429784454696930052, -4.460028654918597901 ) ) ;
#13778=CARTESIAN_POINT ( 'NONE',  ( -22.83540780336928577, 150.4058779721138421, -0.4563057931615319140 ) ) ;
#13780=AXIS2_PLACEMENT_3D ( 'NONE', #17981, #30978, #24576 ) ;
#13781=LINE ( 'NONE', #24192, #16967 ) ;
#13782=CARTESIAN_POINT ( 'NONE',  ( -5.034331710563058948, 119.1737376751357118, 0.9019231717209493793 ) ) ;
#13783=CARTESIAN_POINT ( 'NONE',  ( -2.900346660479264482, -2.445871450894649968, -3.618988008572288972 ) ) ;
#13784=CARTESIAN_POINT ( 'NONE',  ( 20.95410280040430351, 151.1643092826112138, 1.845047842948928762 ) ) ;
#13787=CARTESIAN_POINT ( 'NONE',  ( 18.13891979603522486, 131.7244750738095149, -1.506900917850658050 ) ) ;
#13788=CARTESIAN_POINT ( 'NONE',  ( -3.339653329301207840, -2.245917679271888900, -3.199182135983138053 ) ) ;
#13789=CARTESIAN_POINT ( 'NONE',  ( -12.90531570856127175, 156.9034992427187376, -1.273604633583561796 ) ) ;
#13790=VERTEX_POINT ( 'NONE', #1094 ) ;
#13791=CARTESIAN_POINT ( 'NONE',  ( -7.620757776630488145, 122.3831840716419066, 0.1218999176909029841 ) ) ;
#13792=CARTESIAN_POINT ( 'NONE',  ( 3.639791848495840476, -15.36872039720094207, 5.326864320309495859 ) ) ;
#13794=AXIS2_PLACEMENT_3D ( 'NONE', #9227, #5411, #19003 ) ;
#13795=FACE_OUTER_BOUND ( 'NONE', #11295, .T. ) ;
#13797=CARTESIAN_POINT ( 'NONE',  ( 6.251746415250003963, 157.3995435888475072, 1.956906209352898829 ) ) ;
#13798=DIRECTION ( 'NONE',  ( -4.017660918040594346E-17, 1.000000000000000000, 2.376309959284834438E-19 ) ) ;
#13800=AXIS2_PLACEMENT_3D ( 'NONE', #16096, #6329, #3136 ) ;
#13801=CARTESIAN_POINT ( 'NONE',  ( -1.353295744334297224, 159.4649289425152858, 0.7236632733165272446 ) ) ;
#13802=CARTESIAN_POINT ( 'NONE',  ( 0.09500447679424951775, 1.427469433126556053, 8.421719372511704549 ) ) ;
#13803=CARTESIAN_POINT ( 'NONE',  ( -0.01887828017123771920, 156.5412816204240301, 0.9447463363288814975 ) ) ;
#13806=CARTESIAN_POINT ( 'NONE',  ( 6.917230302148959176, 117.3903047926647787, -0.3126493885886559854 ) ) ;
#13807=DIRECTION ( 'NONE',  ( 0.9998004120163608288, 5.205824365704082573E-17, 0.01997839162482763914 ) ) ;
#13810=CARTESIAN_POINT ( 'NONE',  ( 3.496333745419838657, 108.2590522130000323, -4.019922511746928606 ) ) ;
#13813=CARTESIAN_POINT ( 'NONE',  ( -4.464873506718732621, 118.1580953083285692, 0.4253042567280939101 ) ) ;
#13816=CARTESIAN_POINT ( 'NONE',  ( 6.137199031469663169, 119.5145805505420924, -1.013644267285056966 ) ) ;
#13817=CARTESIAN_POINT ( 'NONE',  ( -6.530233653229074342, 120.6338824379019172, -0.3959831657380195047 ) ) ;
#13819=CARTESIAN_POINT ( 'NONE',  ( 4.599842283008522159, 118.0596567094243596, 0.7232788779925730660 ) ) ;
#13820=CARTESIAN_POINT ( 'NONE',  ( -16.01418025823793911, 147.7157881801689427, -1.429122529412921061 ) ) ;
#13822=CARTESIAN_POINT ( 'NONE',  ( -1.665825627024804634, 115.7029491485453434, -1.727339162086583890 ) ) ;
#13823=CARTESIAN_POINT ( 'NONE',  ( 2.753590479458230433, 118.1651001943547925, -0.7052533925992238162 ) ) ;
#13824=CARTESIAN_POINT ( 'NONE',  ( 0.8832484628481780398, 105.9424719104300436, -5.282093952356136768 ) ) ;
#13825=CARTESIAN_POINT ( 'NONE',  ( -13.16414530391302584, 152.2904283036577908, -1.902647459344306347 ) ) ;
#13826=CARTESIAN_POINT ( 'NONE',  ( -5.332935397695335311, 104.6144662015457385, -0.1065647409268299373 ) ) ;
#13827=CARTESIAN_POINT ( 'NONE',  ( -3.525175246668108109, 31.21832863748435472, -0.5828980424257260706 ) ) ;
#13828=CARTESIAN_POINT ( 'NONE',  ( 8.511289907599318028, 119.1972314554220276, -1.000383355283308129 ) ) ;
#13829=CARTESIAN_POINT ( 'NONE',  ( -7.997804479448351600, 122.8474177855006246, -0.03617150109717347239 ) ) ;
#13831=CARTESIAN_POINT ( 'NONE',  ( 0.3303419930533891824, 116.8490449975401617, 0.2909865916005164310 ) ) ;
#13833=CARTESIAN_POINT ( 'NONE',  ( 1.824651611884654967, -15.33505462125983598, 5.392305443003406751 ) ) ;
#13834=CARTESIAN_POINT ( 'NONE',  ( -19.30447918735904622, 147.3692480224366079, 1.738561774106543778 ) ) ;
#13835=CARTESIAN_POINT ( 'NONE',  ( -0.2718671964776636085, -13.46374167387040366, -0.9358251418597670623 ) ) ;
#13836=CARTESIAN_POINT ( 'NONE',  ( -23.06197264524096724, 149.2510847660714148, -1.189562549516614443 ) ) ;
#13838=CARTESIAN_POINT ( 'NONE',  ( 0.9522911014763013604, -10.27702741150894994, -0.2247348558088197723 ) ) ;
#13841=CARTESIAN_POINT ( 'NONE',  ( 5.292905998138358825, 116.9650601603920279, 0.9543338394691548432 ) ) ;
#13842=CARTESIAN_POINT ( 'NONE',  ( -0.6112472438487006610, 120.6441756478195089, 0.2446543754660638059 ) ) ;
#13843=CARTESIAN_POINT ( 'NONE',  ( 3.798736437616232919, -14.27876630094554500, 4.860596070177301442 ) ) ;
#13844=CARTESIAN_POINT ( 'NONE',  ( 7.347594966877624145, 120.9764928074160082, -0.8683198564056585633 ) ) ;
#13845=CARTESIAN_POINT ( 'NONE',  ( -8.661198069469564942, 120.2102557752085232, -1.489220423754913369 ) ) ;
#13846=CARTESIAN_POINT ( 'NONE',  ( 4.531670475907399798, 115.7029491485453434, 1.515581646943963356 ) ) ;
#13847=CARTESIAN_POINT ( 'NONE',  ( 2.967701212693483193, -13.54563334627871463, 1.070011838909553425 ) ) ;
#13848=CARTESIAN_POINT ( 'NONE',  ( -4.948335771857875542, 117.4718462369176137, -1.024210282226911684 ) ) ;
#13849=CARTESIAN_POINT ( 'NONE',  ( 7.846345427436761000, 154.6110463214094182, -0.1182179892959121792 ) ) ;
#13851=CARTESIAN_POINT ( 'NONE',  ( -3.892802331515536007, 109.0594729580251254, 3.652645560113729761 ) ) ;
#13852=CARTESIAN_POINT ( 'NONE',  ( 3.936408729728400058, 109.5187069194626872, 3.609317897251677287 ) ) ;
#13854=CARTESIAN_POINT ( 'NONE',  ( -13.70496720263922619, 119.6480011847203002, -0.2738578607179661395 ) ) ;
#13855=ADVANCED_FACE ( 'NONE', ( #40074, #31505 ), #9151, .F. ) ;
#13857=CARTESIAN_POINT ( 'NONE',  ( 5.742584425896265721, 159.1207877133979309, 0.01316620519284362155 ) ) ;
#13859=DIRECTION ( 'NONE',  ( -0.9998004120163609398, 0.000000000000000000, -0.01997839162482749689 ) ) ;
#13861=CARTESIAN_POINT ( 'NONE',  ( 1.692908751855406679, -15.45794499411305623, 5.831830892034441050 ) ) ;
#13863=CARTESIAN_POINT ( 'NONE',  ( -6.580517660824093636E-14, 85.69146620154573668, -4.881702850681514412E-18 ) ) ;
#13864=EDGE_CURVE ( 'NONE', #18999, #24610, #15669, .T. ) ;
#13865=CARTESIAN_POINT ( 'NONE',  ( 19.97852701226055316, 149.8444905389382882, 2.417717604095676265 ) ) ;
#13867=CARTESIAN_POINT ( 'NONE',  ( -8.379105243356219646, 21.88232641057985361, -0.8402904295462267914 ) ) ;
#13868=CARTESIAN_POINT ( 'NONE',  ( 5.545307748665752712, 117.8092076766180867, -0.8261742690153465185 ) ) ;
#13869=CARTESIAN_POINT ( 'NONE',  ( -1.726955742647845460, 108.8931014686503289, -4.100893600158903141 ) ) ;
#13870=AXIS2_PLACEMENT_3D ( 'NONE', #16683, #6482, #26705 ) ;
#13873=CARTESIAN_POINT ( 'NONE',  ( -5.314273266013044505, 104.6144662015457527, 0.4583182832411464291 ) ) ;
#13874=CARTESIAN_POINT ( 'NONE',  ( 4.440276399826426967, -1.430929408009915083, -1.287880193523989636 ) ) ;
#13876=CARTESIAN_POINT ( 'NONE',  ( 0.1066493941974573784, 105.7853621660184444, -5.332931186019219005 ) ) ;
#13877=CARTESIAN_POINT ( 'NONE',  ( 2.491201389814710065, -14.86453887000410745, 4.964479704013470496 ) ) ;
#13878=CARTESIAN_POINT ( 'NONE',  ( 3.201024870707998016, 118.2446163226072713, -0.7148959180058853669 ) ) ;
#13879=CARTESIAN_POINT ( 'NONE',  ( -15.64055365641546835, 121.4606353739761744, 0.3859511643760805133 ) ) ;
#13880=CARTESIAN_POINT ( 'NONE',  ( 4.828635879361813821, 117.4024293536648855, -1.010132067140149026 ) ) ;
#13881=CARTESIAN_POINT ( 'NONE',  ( -3.682264917456322895, 69.43546620154573645, -0.07358041635423923088 ) ) ;
#13883=LINE ( 'NONE', #29225, #29456 ) ;
#13885=CARTESIAN_POINT ( 'NONE',  ( 2.989574797431095554, -15.77888062423098070, 5.070590765341169259 ) ) ;
#13886=CARTESIAN_POINT ( 'NONE',  ( -6.603547431282940749, 157.6773268839678508, 1.653176294384505640 ) ) ;
#13887=CARTESIAN_POINT ( 'NONE',  ( -0.6053885369530382921, 31.17761759867932980, -0.7634260365338448873 ) ) ;
#13890=CARTESIAN_POINT ( 'NONE',  ( -6.513165593194060347E-14, 68.92746620154572668, -8.865348866426607246E-18 ) ) ;
#13891=CARTESIAN_POINT ( 'NONE',  ( 1.032349031751431445, 124.2655319029901335, 0.08020592950830184031 ) ) ;
#13893=CARTESIAN_POINT ( 'NONE',  ( -15.87656987697871891, 149.2064892436030163, 1.252469198948042761 ) ) ;
#13895=CARTESIAN_POINT ( 'NONE',  ( 18.67487979129049336, 147.7499600834086948, -1.698815563122507699 ) ) ;
#13896=CARTESIAN_POINT ( 'NONE',  ( -20.40332572169753433, 149.1468970683199586, -2.432323357318188606 ) ) ;
#13899=ORIENTED_EDGE ( 'NONE', *, *, #26607, .T. ) ;
#13900=CARTESIAN_POINT ( 'NONE',  ( 4.415132207561733857, 118.1795667174292532, -0.3921168564559623371 ) ) ;
#13901=CARTESIAN_POINT ( 'NONE',  ( 15.74292597311039898, 147.5983985311728759, -0.4089823612135939368 ) ) ;
#13902=ORIENTED_EDGE ( 'NONE', *, *, #21380, .F. ) ;
#13903=CARTESIAN_POINT ( 'NONE',  ( 2.709380901426776678, -15.26748983718428931, 4.527680251005613776 ) ) ;
#13906=CARTESIAN_POINT ( 'NONE',  ( -4.324967070706027705, -0.5217348546298695711, 1.653223044864502222 ) ) ;
#13907=CARTESIAN_POINT ( 'NONE',  ( 15.02674521555423581, 134.7883251604851580, 1.951091898071899200 ) ) ;
#13908=CARTESIAN_POINT ( 'NONE',  ( -2.960856320778833428, 31.17411798999470918, 0.6378382452821284021 ) ) ;
#13909=CARTESIAN_POINT ( 'NONE',  ( 3.700881553190929374, 8.714383148187751615, -2.768892949411812854 ) ) ;
#13910=CARTESIAN_POINT ( 'NONE',  ( 8.506011814013298533, 123.3280575159016905, 0.2025880313713111225 ) ) ;
#13913=CARTESIAN_POINT ( 'NONE',  ( 5.560813481388145796, 116.7424064675562505, -0.1180550052279501078 ) ) ;
#13914=CARTESIAN_POINT ( 'NONE',  ( 3.682264917456193665, 63.84746620154572838, 0.07358041635423968885 ) ) ;
#13917=CARTESIAN_POINT ( 'NONE',  ( -3.174366308152013705, 97.37546620154573418, -0.06343139340882732180 ) ) ;
#13918=CARTESIAN_POINT ( 'NONE',  ( 1.223683442775902463, 5.461509463947571419, 8.358860550006438572 ) ) ;
#13921=CARTESIAN_POINT ( 'NONE',  ( 0.4234688608138943988, 124.8375573595198063, -0.002553167718423972939 ) ) ;
#13922=CARTESIAN_POINT ( 'NONE',  ( -21.27466159042558758, 132.4531229209162575, 0.1171209876626085472 ) ) ;
#13926=CARTESIAN_POINT ( 'NONE',  ( 6.988932177366979026, 121.9539960043768616, 0.09502985394448600076 ) ) ;
#13929=CARTESIAN_POINT ( 'NONE',  ( -15.72575858332452015, 145.6903699455376113, -0.3657738730356400181 ) ) ;
#13930=CARTESIAN_POINT ( 'NONE',  ( 6.002709446384779213, -13.95775275001606630, 2.224537231649871494 ) ) ;
#13931=CARTESIAN_POINT ( 'NONE',  ( -17.75928342660610681, 128.5843929717815115, 1.279242276855531379 ) ) ;
#13932=CARTESIAN_POINT ( 'NONE',  ( -3.562413952978887632, 23.18266144714348798, 2.948169924785601470 ) ) ;
#13933=CARTESIAN_POINT ( 'NONE',  ( 22.49834027909111356, 137.1624432810789358, 0.8864494676080415525 ) ) ;
#13934=CARTESIAN_POINT ( 'NONE',  ( 2.137372358784370263, -15.62272051899096859, 5.517997703402476084 ) ) ;
#13936=CARTESIAN_POINT ( 'NONE',  ( -0.5845540250341307864, -7.254922367050685494, -0.7839501960785225654 ) ) ;
#13937=CARTESIAN_POINT ( 'NONE',  ( -1.410028229074622219, 159.6020224343070026, -0.1582310832764448894 ) ) ;
#13938=CARTESIAN_POINT ( 'NONE',  ( -3.174366308152013705, 104.6144662015457243, -0.06343139340882732180 ) ) ;
#13939=CARTESIAN_POINT ( 'NONE',  ( 8.754061279740081858, 117.8557914870123682, 0.6177215411034930881 ) ) ;
#13940=CARTESIAN_POINT ( 'NONE',  ( -0.01023306027096490718, 119.5380416804913324, 0.5121041807152045822 ) ) ;
#13942=CARTESIAN_POINT ( 'NONE',  ( 9.459309661781043488, 157.4068808874136209, 1.850812122078211441 ) ) ;
#13943=CARTESIAN_POINT ( 'NONE',  ( 19.53500017296053670, 148.0998626603252148, -1.736236475658778033 ) ) ;
#13944=CARTESIAN_POINT ( 'NONE',  ( 0.6087277426107279288, -8.065848283227245119, 0.7602462886992925606 ) ) ;
#13945=CARTESIAN_POINT ( 'NONE',  ( -12.26619010297312684, 120.4651188882986759, -1.462776157934944310 ) ) ;
#13948=CARTESIAN_POINT ( 'NONE',  ( 4.553366535382863844, 104.6144662015457243, 1.608775678008367516 ) ) ;
#13949=CARTESIAN_POINT ( 'NONE',  ( 0.7532517793758595204, 156.4767055779393559, -0.8130599351363748672 ) ) ;
#13950=CARTESIAN_POINT ( 'NONE',  ( -13.59117098933512580, 150.2425924485890505, -0.2715839415562138481 ) ) ;
#13952=CARTESIAN_POINT ( 'NONE',  ( -11.26837603645374131, 123.0403929720162495, -1.648478483780370318 ) ) ;
#13953=CARTESIAN_POINT ( 'NONE',  ( 5.315755633098069310, -15.26259334675766866, -0.1387823706055290596 ) ) ;
#13954=LINE ( 'NONE', #16938, #2727 ) ;
#13955=CARTESIAN_POINT ( 'NONE',  ( -4.512940082713024381, 118.0696988386537214, -0.8149125216352793855 ) ) ;
#13958=CARTESIAN_POINT ( 'NONE',  ( 13.99859221269040432, 128.5416456306063253, 1.961142612884885450 ) ) ;
#13960=CARTESIAN_POINT ( 'NONE',  ( 5.757472737270592944, 159.1136035536173097, 0.1150480073142623738 ) ) ;
#13961=CARTESIAN_POINT ( 'NONE',  ( 6.431785950458272616, 8.712657024569978148, -5.436233950049250474 ) ) ;
#13962=CARTESIAN_POINT ( 'NONE',  ( 6.479751845157252887, 121.6679077367135591, 0.4493306481243478645 ) ) ;
#13963=CARTESIAN_POINT ( 'NONE',  ( 15.15503192428636581, 121.4505734225448066, -0.6300967139502822167 ) ) ;
#13965=CARTESIAN_POINT ( 'NONE',  ( -22.98521553460867750, 150.1595482613961110, -0.3823759483556143368 ) ) ;
#13966=CIRCLE ( 'NONE', #13276, 0.5080000000000002292 ) ;
#13969=CARTESIAN_POINT ( 'NONE',  ( 6.787014259399680505, 121.1158114507673531, -0.6846564350370034635 ) ) ;
#13970=CARTESIAN_POINT ( 'NONE',  ( -8.796322004575976905, 117.7098159678576224, 0.02677737093239071497 ) ) ;
#13973=CARTESIAN_POINT ( 'NONE',  ( -8.994301780669152535, 123.6974368934138226, -0.4925676131310582351 ) ) ;
#13974=CARTESIAN_POINT ( 'NONE',  ( 3.467186027297813666, -14.69398785160878873, 5.340258725024584763 ) ) ;
#13975=CARTESIAN_POINT ( 'NONE',  ( -14.35401710045877799, 121.2650221238243944, 0.8333810220845707661 ) ) ;
#13977=CARTESIAN_POINT ( 'NONE',  ( 4.732570698819401400, 116.7698466342620378, 0.1749797587976940905 ) ) ;
#13979=CARTESIAN_POINT ( 'NONE',  ( -4.515506726787251068, -6.291224493951820484, 1.111903093310195212 ) ) ;
#13980=CARTESIAN_POINT ( 'NONE',  ( -22.75563279970867470, 137.3797884758947703, -0.4783205966563212619 ) ) ;
#13984=CARTESIAN_POINT ( 'NONE',  ( -4.401808571117955537, 118.5828793204378115, 0.8681470107976926309 ) ) ;
#13986=CARTESIAN_POINT ( 'NONE',  ( -0.3558933743640902425, 1.202427940091101100, 4.626034787239965418 ) ) ;
#13987=CARTESIAN_POINT ( 'NONE',  ( 21.19929070476245059, 136.5942649496780632, 1.819607900871525796 ) ) ;
#13989=CARTESIAN_POINT ( 'NONE',  ( 16.52101850268826055, 153.5550899668227203, -1.581448849539220269 ) ) ;
#13990=CARTESIAN_POINT ( 'NONE',  ( 3.951836011467571907, -5.044640503713330837, -2.394960105287299523 ) ) ;
#13991=CARTESIAN_POINT ( 'NONE',  ( -2.005144469771080740, 117.2046888992736200, -0.5340627965622030127 ) ) ;
#13992=EDGE_CURVE ( 'NONE', #38547, #39868, #10491, .T. ) ;
#13994=CARTESIAN_POINT ( 'NONE',  ( -9.248842176950111238, 124.1957968681474824, -0.02334546025992350476 ) ) ;
#13995=CARTESIAN_POINT ( 'NONE',  ( 6.166227012738786151, -13.75546675568918609, 1.699147612634045235 ) ) ;
#13997=CARTESIAN_POINT ( 'NONE',  ( -5.045173026404576433, 113.8198996840133930, -1.826729658900504649 ) ) ;
#13998=AXIS2_PLACEMENT_3D ( 'NONE', #20155, #27190, #4007 ) ;
#14000=CARTESIAN_POINT ( 'NONE',  ( 19.51070465195328651, 147.4874203640471535, 2.520207112597399934 ) ) ;
#14001=FACE_OUTER_BOUND ( 'NONE', #33867, .T. ) ;
#14002=CARTESIAN_POINT ( 'NONE',  ( 3.682264917456192332, 95.34346620154573770, 0.07358041635423968885 ) ) ;
#14003=CARTESIAN_POINT ( 'NONE',  ( -2.024878990865745187, 117.2046888992736200, 0.4535333368958822109 ) ) ;
#14004=CARTESIAN_POINT ( 'NONE',  ( 7.114778624005384522, 4.676967889965610858, -4.534447634950107719 ) ) ;
#14005=CARTESIAN_POINT ( 'NONE',  ( 10.62861998609533742, 124.7671305375842934, 1.166658412819147950 ) ) ;
#14007=CARTESIAN_POINT ( 'NONE',  ( 4.817281438370265789, 117.0090399748681875, -0.3002870190743004986 ) ) ;
#14013=CARTESIAN_POINT ( 'NONE',  ( -4.503997341962783452, 118.1168880179826175, 0.5560608495562332498 ) ) ;
#14014=CARTESIAN_POINT ( 'NONE',  ( 0.3948153568139246561, 105.8845321910897042, -5.327123519515836847 ) ) ;
#14015=B_SPLINE_SURFACE_WITH_KNOTS ( 'NONE', 5, 5, ( 
 ( #29259, #36090, #3721, #32889, #41487, #13069 ),
 ( #41275, #22842, #26488, #29684, #39070, #528 ),
 ( #25069, #18455, #35882, #6692, #317, #13284 ),
 ( #35097, #26269, #13500, #26059, #18881, #38286 ),
 ( #22070, #12294, #105, #10298, #16256, #5494 ),
 ( #2304, #31890, #2726, #39279, #19661, #38072 ),
 ( #8888, #32675, #27115, #4355, #7745, #23911 ),
 ( #23693, #30306, #29895, #33943, #732, #33311 ),
 ( #4140, #20494, #1359, #27329, #23479, #20079 ),
 ( #40547, #11134, #40130, #39919, #10921, #40341 ),
 ( #7325, #30519, #14317, #11345, #13913, #20712 ),
 ( #33523, #10713, #17316, #3933, #36927, #943 ),
 ( #17101, #36712, #33736, #7533, #36504, #20920 ),
 ( #1149, #20283, #33102, #30104, #4559, #4774 ),
 ( #13708, #26906, #14118, #17519, #36302, #24121 ),
 ( #37131, #7951, #17723, #30726, #7124, #1575 ),
 ( #14531, #27541, #16892, #26702, #39707, #10509 ),
 ( #17936, #34152, #15375, #8577, #27950, #30939 ),
 ( #14950, #11975, #5190, #1988, #2415, #15160 ),
 ( #25185, #31147, #24754, #34570, #37968, #31359 ),
 ( #14739, #40959, #24968, #41387, #11765, #4979 ),
 ( #18353, #15584, #1778, #41171, #31785, #11549 ),
 ( #27742, #37541, #18775, #40752, #21331, #37753 ),
 ( #21540, #8793, #5397, #24532, #2202, #8364 ),
 ( #34358, #21751, #34999, #38185, #18143, #28166 ),
 ( #34778, #41597, #5612, #18568, #31575, #28380 ),
 ( #12192, #28589, #9002, #21969, #5819, #2625 ),
 ( #24330, #37336, #8154, #21124, #10037, #35830 ),
 ( #6646, #12609, #41813, #22170, #32414, #38604 ),
 ( #12811, #22587, #9410, #25801, #39227, #28799 ),
 ( #9619, #29640, #32208, #35402, #3668, #15791 ),
 ( #28998, #35201, #16633, #3041, #13239, #42015 ),
 ( #23009, #265, #38807, #19200, #15999, #25596 ),
 ( #26223, #35619, #29424, #32838, #36037, #6433 ),
 ( #22795, #22376, #6852, #31993, #38401, #19407 ),
 ( #3244, #26011, #51, #6229, #16203, #29208 ),
 ( #19821, #18989, #13017, #39020, #9828, #19610 ),
 ( #3456, #32623, #9213, #2831, #12407, #25399 ),
 ( #16418, #6027, #4512, #20240, #13658, #36883 ),
 ( #17677, #33266, #14069, #4307, #894, #36669 ),
 ( #1102, #20870, #24076, #4095, #17054, #10876 ),
 ( #20034, #26438, #10666, #33477, #23647, #27073 ),
 ( #16848, #30056, #7490, #36249, #40296, #7070 ),
 ( #686, #39656, #26862, #7701, #33688, #29848 ),
 ( #33053, #4725, #17473, #17270, #13868, #30261 ),
 ( #39870, #26648, #20662, #30471, #477, #20450 ),
 ( #40081, #23864, #1315, #10460, #14272, #10245 ),
 ( #37088, #23216, #23430, #27282, #11089, #7906 ),
 ( #33894, #36459, #13450, #7278, #39442, #3883 ),
 ( #41335, #31516, #37286, #30891, #14690, #11499 ),
 ( #15106, #14898, #24485, #37490, #28109, #21285 ),
 ( #8738, #2361, #34521, #40502, #1732, #31100 ),
 ( #8105, #21489, #28327, #11925, #21914, #24917 ),
 ( #17889, #11297, #8529, #27695, #15320, #1939 ),
 ( #34944, #12138, #8313, #27900, #40908, #2147 ),
 ( #40703, #21079, #34314, #31302, #5554, #5143 ),
 ( #5768, #18097, #25130, #11713, #24700, #38132 ),
 ( #37706, #5347, #18301, #41119, #37914, #8947 ),
 ( #18511, #21699, #34723, #30678, #1526, #14482 ),
 ( #27494, #24281, #34104, #4931, #25341, #22538 ),
 ( #2782, #9362, #32152, #35774, #13186, #15536 ),
 ( #35984, #3187, #2985, #12557, #25546, #16149 ),
 ( #22956, #38549, #3399, #15947, #22325, #32566 ),
 ( #26171, #39175, #16366, #12353, #28538, #9776 ),
 ( #35350, #38344, #28944, #6178, #6383, #41756 ),
 ( #38966, #9567, #18722, #19557, #19147, #41961 ),
 ( #32359, #25749, #28743, #9162, #12760, #19353 ),
 ( #38757, #41545, #9983, #35565, #29372, #29153 ),
 ( #31732, #5973, #22742, #35148, #2575, #42161 ),
 ( #6589, #12965, #25959, #18936, #211, #22119 ),
 ( #31944, #15738, #30004, #36830, #4465, #20606 ),
 ( #20398, #36620, #23164, #36414, #844, #426 ),
 ( #13396, #3834, #7020, #16798, #33217, #14018 ),
 ( #36199, #32788, #26385, #11039, #23809, #10617 ),
 ( #23599, #10827, #26599, #19988, #1054, #27025 ),
 ( #39606, #33426, #7439, #7232, #13816, #33006 ),
 ( #16583, #29799, #4255, #7650, #23381, #29592 ),
 ( #10409, #33638, #20192, #640, #17422, #30420 ),
 ( #13609, #4044, #17005, #26815, #1267, #39823 ),
 ( #27231, #14223, #17217, #30214, #40033, #40245 ),
 ( #39392, #3618, #24022, #6799, #19767, #10194 ),
 ( #24435, #31046, #30630, #34674, #1473, #34054 ),
 ( #4883, #21234, #2094, #28058, #24229, #20818 ),
 ( #41281, #11878, #40859, #40653, #11661, #41068 ),
 ( #8057, #31253, #15058, #12087, #14639, #8481 ),
 ( #37439, #1885, #21031, #37657, #4672, #17838 ),
 ( #17629, #30836, #8262, #5299, #27640, #21437 ),
 ( #11244, #34263, #1685, #33844, #11446, #34466 ),
 ( #37863, #14430, #37239, #5092, #18045, #37039 ),
 ( #14847, #27852, #24647, #18247, #24867, #7857 ),
 ( #21649, #8687, #5503, #18462, #27438, #31467 ),
 ( #2310, #15271, #28276, #40454, #19305, #25288 ),
 ( #34889, #2935, #9110, #38920, #25500, #35304 ),
 ( #38500, #9730, #41494, #25912, #22278, #167 ),
 ( #5924, #16320, #31682, #9316, #15687, #12714 ),
 ( #6132, #19095, #22074, #32104, #22697, #12299 ),
 ( #15897, #25075, #2732, #18887, #29323, #28486 ),
 ( #22486, #38292, #35101, #2524, #28899, #38081 ),
 ( #41914, #32522, #31895, #29107, #28693, #8895 ),
 ( #21863, #16102, #41702, #25704, #12510, #38709 ),
 ( #9519, #35514, #18675, #6335, #12921, #35728 ),
 ( #32310, #3140, #42125, #6539, #19513, #3353 ),
 ( #5719, #15487, #10146, #13345, #23116, #39557 ),
 ( #4201, #379, #39130, #32740, #17376, #30164 ),
 ( #16745, #16954, #17165, #32958, #26334, #7385 ),
 ( #30366, #3785, #26765, #29953, #13561, #7186 ),
 ( #13768, #22906, #39341, #7594, #35940, #36152 ),
 ( #23547, #29750, #39774, #26551, #29544, #10362 ),
 ( #9936, #6969, #10569, #23756, #13969, #19721 ),
 ( #19940, #4418, #3573, #36778, #589, #26973 ),
 ( #6752, #20345, #793, #33369, #39984, #36568 ),
 ( #16534, #20556, #33586, #10775, #23333, #36369 ),
 ( #20145, #33168, #3996, #1005, #13137, #26128 ),
 ( #24386, #10987, #30992, #8008, #1630, #11191 ),
 ( #1832, #4830, #1420, #28006, #14585, #11823 ),
 ( #5037, #24812, #27387, #34000, #27590, #18198 ),
 ( #40192, #24177, #34623, #33794, #37807, #20979 ),
 ( #17782, #23969, #37599, #17994, #21384, #2042 ),
 ( #36988, #14377, #40599, #30581, #20770, #34209 ),
 ( #24592, #5450, #8425, #40397, #37186, #7808 ),
 ( #30781, #15007, #11399, #37391, #8209, #21181 ),
 ( #14796, #27799, #40807, #11608, #34410, #4622 ),
 ( #8632, #5243, #17577, #31199, #41015, #21594 ),
 ( #18410, #1215, #14174, #27178, #35465, #5670 ),
 ( #19045, #28223, #22435, #22026, #25457, #18627 ),
 ( #32267, #31842, #28856, #25023, #12463, #19259 ),
 ( #3097, #15434, #38454, #18838, #12032, #35258 ),
 ( #6288, #22229, #16058, #38025, #41229, #2259 ),
 ( #32050, #41869, #12668, #38869, #2682, #25657 ),
 ( #9272, #15639, #9061, #8846, #35055, #29060 ),
 ( #5875, #42080, #9681, #12873, #38244, #25862 ),
 ( #28644, #35681, #41655, #22647, #6082, #2887 ),
 ( #15221, #6490, #31417, #21810, #34836, #31632 ),
 ( #15850, #38664, #2473, #9472, #28437, #41443 ),
 ( #12248, #25241, #10312, #23706, #20296, #26284 ),
 ( #29698, #33117, #26502, #29490, #9885, #39292 ),
 ( #16906, #35895, #6705, #26075, #13513, #10726 ),
 ( #36317, #26919, #19674, #23492, #32689, #36726 ),
 ( #16270, #10521, #10098, #39506, #3523, #23281 ),
 ( #19888, #29908, #13083, #539, #7338, #17116 ),
 ( #16484, #7136, #6919, #119, #20093, #39934 ),
 ( #30117, #39083, #331, #13297, #23071, #3735 ),
 ( #36519, #36104, #3305, #22858, #19468, #33324 ),
 ( #32904, #3946, #4153, #16693, #746, #13721 ),
 ( #32475, #26715, #39723, #957, #13926, #29272 ),
 ( #8749, #17329, #20725, #2586, #30319, #4574 ),
 ( #18523, #27911, #21711, #8539, #23924, #34532 ),
 ( #33537, #33749, #5567, #18732, #8958, #14128 ),
 ( #17532, #30533, #25352, #34735, #37926, #4369 ),
 ( #40918, #2158, #36940, #11936, #21926, #21499 ) ),
 .UNSPECIFIED., .F., .F., .F.,
 ( 6, 4, 4, 4, 4, 4, 4, 4, 4, 4, 4, 4, 4, 4, 4, 4, 4, 4, 4, 4, 4, 4, 4, 4, 4, 4, 4, 4, 4, 4, 4, 4, 4, 4, 4, 4, 4, 6 ),
 ( 6, 6 ),
 ( 0.000000000000000000, 0.01562500000000000000, 0.02343750000000000000, 0.03125000000000000000, 0.04687500000000000000, 0.06250000000000000000, 0.09375000000000000000, 0.1093750000000000000, 0.1171875000000000000, 0.1250000000000000000, 0.1875000000000000000, 0.2187500000000000000, 0.2500000000000000000, 0.3125000000000000000, 0.3750000000000000000, 0.4062500000000000000, 0.4218750000000000000, 0.4375000000000000000, 0.4687500000000000000, 0.4843750000000000000, 0.4921875000000000000, 0.5000000000000000000, 0.5312500000000000000, 0.5468750000000000000, 0.5625000000000000000, 0.6250000000000000000, 0.6875000000000000000, 0.7500000000000000000, 0.8125000000000000000, 0.8437500000000000000, 0.8750000000000000000, 0.9062500000000000000, 0.9375000000000000000, 0.9531250000000000000, 0.9687500000000000000, 0.9765625000000000000, 0.9843750000000000000, 1.000000000000000000 ),
 ( 0.000000000000000000, 1.000000000000000000 ),
 .UNSPECIFIED. ) ;
#14018=CARTESIAN_POINT ( 'NONE',  ( 8.365669025111728274, 119.9184419981384906, -1.112736592547703962 ) ) ;
#14019=CARTESIAN_POINT ( 'NONE',  ( -7.474242191267291169, 123.6620266863018855, -0.1838331482465496713 ) ) ;
#14020=CARTESIAN_POINT ( 'NONE',  ( 4.506509836442742944, 118.1222450895864142, 0.6634770384556544220 ) ) ;
#14021=CARTESIAN_POINT ( 'NONE',  ( -8.116318325016218083, 154.6259123219959690, -0.9857874811295549433 ) ) ;
#14022=CARTESIAN_POINT ( 'NONE',  ( 0.03519895179119666290, 115.7029491485446613, -1.761499482103947800 ) ) ;
#14023=CARTESIAN_POINT ( 'NONE',  ( 2.601312006192598947, 117.9496052548661282, -1.235025137275671536 ) ) ;
#14025=DIRECTION ( 'NONE',  ( -4.017660918040594346E-17, 1.000000000000000000, 2.376309959284834438E-19 ) ) ;
#14026=CARTESIAN_POINT ( 'NONE',  ( -5.138962689587368793, 120.6777149489875569, -0.7548553450424396738 ) ) ;
#14030=CARTESIAN_POINT ( 'NONE',  ( 8.709803600792051625, 118.1821829479768411, -0.5645179937760026467 ) ) ;
#14031=CARTESIAN_POINT ( 'NONE',  ( -6.068413115653235046, 121.4395679061438500, -0.1212613406838785185 ) ) ;
#14034=CARTESIAN_POINT ( 'NONE',  ( 22.80589948333479455, 149.4631731099488832, 1.425235564609340644 ) ) ;
#14036=CARTESIAN_POINT ( 'NONE',  ( 3.040187153003802933, -14.59799761600802448, -0.3075781077882258630 ) ) ;
#14037=CARTESIAN_POINT ( 'NONE',  ( -8.398523874639556297, 120.8878392079396065, 1.065324388190682869 ) ) ;
#14038=CARTESIAN_POINT ( 'NONE',  ( -0.6988831915142799112, -0.7227331674307564402, 0.6786060147580050828 ) ) ;
#14039=CARTESIAN_POINT ( 'NONE',  ( -14.89898862929395307, 156.1361208441215922, -1.045442070961571712 ) ) ;
#14040=CARTESIAN_POINT ( 'NONE',  ( 0.1793159252905947298, -3.154364953387045034, 0.9593126492898319535 ) ) ;
#14044=CARTESIAN_POINT ( 'NONE',  ( 4.746159770738230144, 112.7696648386057632, 2.567419849205245796 ) ) ;
#14046=CARTESIAN_POINT ( 'NONE',  ( -5.231962949222473291, 121.1607713875043117, 0.2380388119251650447 ) ) ;
#14047=CARTESIAN_POINT ( 'NONE',  ( 4.143153066788715755, -13.73528615761443561, 4.025237717645509861 ) ) ;
#14048=CARTESIAN_POINT ( 'NONE',  ( 13.47719143446456158, 152.3772590505219569, -1.474657383304484037 ) ) ;
#14050=CARTESIAN_POINT ( 'NONE',  ( -17.77132669990263381, 135.5811125208551857, -2.431814553008901481 ) ) ;
#14051=CARTESIAN_POINT ( 'NONE',  ( 4.696425917067753808, 104.6144662015457811, 1.156094417770676230 ) ) ;
#14052=CARTESIAN_POINT ( 'NONE',  ( 2.770737963896511946, -14.84290363635286347, 4.452025088638788652 ) ) ;
#14053=CARTESIAN_POINT ( 'NONE',  ( -4.810636611593423595, 117.4081599864878598, -1.190287313834438532 ) ) ;
#14054=CARTESIAN_POINT ( 'NONE',  ( 6.023029630344915120, 155.3544091381320982, -0.1360875627331026294 ) ) ;
#14055=ORIENTED_EDGE ( 'NONE', *, *, #16267, .T. ) ;
#14057=CARTESIAN_POINT ( 'NONE',  ( 1.982478559079971836, 106.5598271223885973, 4.949040049329130220 ) ) ;
#14058=DIRECTION ( 'NONE',  ( -5.206863593109713045E-17, 1.000000000000000000, -1.077750396879097359E-30 ) ) ;
#14061=CARTESIAN_POINT ( 'NONE',  ( 15.55989727259145816, 120.8127473925414108, 0.08007127899889542044 ) ) ;
#14063=CARTESIAN_POINT ( 'NONE',  ( 1.674296855365971837, -15.41063152441347839, 5.809694019739205295 ) ) ;
#14065=CARTESIAN_POINT ( 'NONE',  ( -1.606566256928685599, 32.19982401495065716, 1.077694121983207021 ) ) ;
#14066=CARTESIAN_POINT ( 'NONE',  ( 1.110739552455571877, 158.5855360310326319, 1.562719372149667496 ) ) ;
#14068=CARTESIAN_POINT ( 'NONE',  ( -5.777836206968382626, 13.68815862607732825, 6.147148275823971275 ) ) ;
#14069=CARTESIAN_POINT ( 'NONE',  ( -2.234004830793105967, 117.0010803218221440, -0.5995543873723633288 ) ) ;
#14070=CARTESIAN_POINT ( 'NONE',  ( -5.704032853997477837, 123.8402959710505087, -0.1558735912124264156 ) ) ;
#14071=CARTESIAN_POINT ( 'NONE',  ( 4.770616296362242714, 117.4047743977180431, 1.204058524662376728 ) ) ;
#14073=CARTESIAN_POINT ( 'NONE',  ( -5.219876558649859888, 104.6144662015479554, 1.151217749705495397 ) ) ;
#14075=CARTESIAN_POINT ( 'NONE',  ( 4.574821423538755205, -2.080616851812391310, 0.6590154617212384824 ) ) ;
#14078=CARTESIAN_POINT ( 'NONE',  ( 3.402052537932679588, -13.50846463298115196, 2.481730329246660371 ) ) ;
#14079=CARTESIAN_POINT ( 'NONE',  ( 3.788670433418564354, 121.1194860566822626, -0.2213384591549590330 ) ) ;
#14080=CARTESIAN_POINT ( 'NONE',  ( -19.68299761936910741, 128.7577553591919752, 0.4435077540095087589 ) ) ;
#14082=CARTESIAN_POINT ( 'NONE',  ( 0.6436272176209127949, 34.89395232701851768, 2.967994052886136824 ) ) ;
#14087=CARTESIAN_POINT ( 'NONE',  ( 4.747814429275453385, -15.55672444834840817, 1.946379828023123482 ) ) ;
#14088=CARTESIAN_POINT ( 'NONE',  ( -2.589082543892896826, 158.1729697732556588, 1.607049804855985808 ) ) ;
#14089=CARTESIAN_POINT ( 'NONE',  ( 4.529186081025091681, -11.15152372915077095, -0.9203776863585164669 ) ) ;
#14091=ORIENTED_EDGE ( 'NONE', *, *, #39751, .F. ) ;
#14094=CARTESIAN_POINT ( 'NONE',  ( 0.7422006451357222589, 119.7070660435176279, 0.6877902101425066306 ) ) ;
#14095=CARTESIAN_POINT ( 'NONE',  ( -0.007600002268431407110, 120.2037396364829505, 0.3803351912374560162 ) ) ;
#14097=CARTESIAN_POINT ( 'NONE',  ( 5.764372972839492348, 156.8407539676644546, -1.669942767410473872 ) ) ;
#14098=CARTESIAN_POINT ( 'NONE',  ( -19.36210883413068728, 150.5708382285403388, -2.397539767985719994 ) ) ;
#14100=CARTESIAN_POINT ( 'NONE',  ( 4.317686572074536322, 118.2120815337069502, -0.3237342310324874961 ) ) ;
#14102=CARTESIAN_POINT ( 'NONE',  ( 0.009747742627749139341, 156.3581291470199233, -0.4878169013068171522 ) ) ;
#14104=CARTESIAN_POINT ( 'NONE',  ( 3.275654002680270960, -14.73162568742410272, 0.7099577593494145189 ) ) ;
#14105=CARTESIAN_POINT ( 'NONE',  ( -5.007446857918051109, 117.4001727933947450, 0.7824604973016788811 ) ) ;
#14107=CARTESIAN_POINT ( 'NONE',  ( -2.651420880294951488, 7.049774601622781134, -3.792306073587544901 ) ) ;
#14108=CARTESIAN_POINT ( 'NONE',  ( 7.970993357304747562, 121.6949282028273132, 1.099362369368162007 ) ) ;
#14109=ADVANCED_FACE ( 'NONE', ( #13174 ), #23385, .F. ) ;
#14110=CARTESIAN_POINT ( 'NONE',  ( 2.324208648641447272, 36.38269483203109189, 0.7534968369120438325 ) ) ;
#14111=CARTESIAN_POINT ( 'NONE',  ( -3.253275476659364784, 108.9521120498200730, 3.903703133364782030 ) ) ;
#14112=CARTESIAN_POINT ( 'NONE',  ( -4.374560056058969693, 13.03735028915297534, 1.504755201125916875 ) ) ;
#14113=CARTESIAN_POINT ( 'NONE',  ( 10.40089755570032359, 153.1126597504080280, 0.2539288847195829701 ) ) ;
#14114=CARTESIAN_POINT ( 'NONE',  ( -0.6577828486943301245, 105.8200195939415238, 5.299418820073016789 ) ) ;
#14118=CARTESIAN_POINT ( 'NONE',  ( -2.159211318501875976, 116.3154634562797156, -0.2664370011832097873 ) ) ;
#14120=CARTESIAN_POINT ( 'NONE',  ( -5.377075248297400911, 4.191758615746518757, 6.528609652590111168 ) ) ;
#14121=EDGE_CURVE ( 'NONE', #10570, #27965, #34307, .T. ) ;
#14124=CARTESIAN_POINT ( 'NONE',  ( 0.4165637647020300482, 124.3520329708341023, -0.05485040398408827511 ) ) ;
#14125=CARTESIAN_POINT ( 'NONE',  ( -20.20614143541417107, 128.9119615565081176, -0.01722291150864733306 ) ) ;
#14128=CARTESIAN_POINT ( 'NONE',  ( 7.786259072927051328, 122.6240336679672964, 0.1181640080994604408 ) ) ;
#14129=VERTEX_POINT ( 'NONE', #26162 ) ;
#14131=CARTESIAN_POINT ( 'NONE',  ( -5.300740673260492031, 121.3529869156830046, -0.1337733589788158428 ) ) ;
#14132=CARTESIAN_POINT ( 'NONE',  ( 4.211475536325941071, -15.04083557003654903, 4.983330352733777779 ) ) ;
#14133=CARTESIAN_POINT ( 'NONE',  ( -21.33845497820667347, 148.5140355411650717, 1.460612514688959473 ) ) ;
#14134=CARTESIAN_POINT ( 'NONE',  ( 2.814065556059444528, 116.6946238705719594, 0.3036003272628904348 ) ) ;
#14135=CARTESIAN_POINT ( 'NONE',  ( 1.552363575376712435, 156.2629490296457107, 0.1466332841606040882 ) ) ;
#14136=CARTESIAN_POINT ( 'NONE',  ( -0.3239230800893593276, 29.42979164457532804, -4.628216972995994993 ) ) ;
#14137=CARTESIAN_POINT ( 'NONE',  ( -0.6378939814135665687, 2.446253604616882349, -0.7403349100440516084 ) ) ;
#14138=CARTESIAN_POINT ( 'NONE',  ( -23.16647984970260765, 149.6103952014060212, -0.7935852015942146398 ) ) ;
#14139=CARTESIAN_POINT ( 'NONE',  ( -4.645572480595541620, 117.9340260526530813, 0.7769932229682322555 ) ) ;
#14140=FACE_OUTER_BOUND ( 'NONE', #20678, .T. ) ;
#14142=CARTESIAN_POINT ( 'NONE',  ( -2.222944194728036393, 116.2580020178152438, 0.07250321285308233832 ) ) ;
#14143=CARTESIAN_POINT ( 'NONE',  ( -2.489404145489931608, 119.6096776070104681, 0.6201668936895532447 ) ) ;
#14145=CARTESIAN_POINT ( 'NONE',  ( 19.37548274631721057, 145.1342744731992127, -1.755133555010167434 ) ) ;
#14146=CARTESIAN_POINT ( 'NONE',  ( 0.7725963012898818816, -15.30024676335969325, -0.5870848125168374176 ) ) ;
#14147=CARTESIAN_POINT ( 'NONE',  ( -13.21493909911912823, 121.0513591912305316, -1.522979426720440843 ) ) ;
#14149=CARTESIAN_POINT ( 'NONE',  ( 4.504358764033148610, 104.6144662015500444, 2.878036670428496091 ) ) ;
#14150=CARTESIAN_POINT ( 'NONE',  ( 3.575420174883959135, 120.5283240077024800, -0.4162329711438421675 ) ) ;
#14151=CARTESIAN_POINT ( 'NONE',  ( -5.959810334499720419, 155.3892724211786742, -0.1190911940436165245 ) ) ;
#14153=CARTESIAN_POINT ( 'NONE',  ( -18.35242356974476863, 147.0160646422468744, -2.398428600884452866 ) ) ;
#14154=CARTESIAN_POINT ( 'NONE',  ( 3.166528004143551289, -15.72052770450255110, 4.635360722337766859 ) ) ;
#14155=CARTESIAN_POINT ( 'NONE',  ( -5.078986093043186933, 100.6774662015457409, -0.1014902294541231709 ) ) ;
#14156=CARTESIAN_POINT ( 'NONE',  ( -4.481907290720103632, 118.1292030818244996, -0.6917001881693495280 ) ) ;
#14160=CARTESIAN_POINT ( 'NONE',  ( 17.63007963961410240, 148.6960320134204210, 2.325091492104032653 ) ) ;
#14161=CARTESIAN_POINT ( 'NONE',  ( 0.02537255736346701387, 39.20946620154573736, -1.269746523260778970 ) ) ;
#14162=CARTESIAN_POINT ( 'NONE',  ( 14.90010799439742861, 120.3262451489332818, 0.2810636626631670132 ) ) ;
#14163=CARTESIAN_POINT ( 'NONE',  ( -8.420209349088564110, 12.38497237326411415, -0.2929423126682718648 ) ) ;
#14164=CARTESIAN_POINT ( 'NONE',  ( 11.96402413561918188, 151.9649008058812569, 0.7942868072307405214 ) ) ;
#14165=CARTESIAN_POINT ( 'NONE',  ( 5.484805557156704481, 159.0107326448372191, -0.7391455978106865610 ) ) ;
#14168=CARTESIAN_POINT ( 'NONE',  ( 5.586884702347365561, 72.99146620154573384, 0.1116392523995368286 ) ) ;
#14169=EDGE_CURVE ( 'NONE', #3481, #2591, #6561, .T. ) ;
#14171=CARTESIAN_POINT ( 'NONE',  ( -1.419391870195790162, 159.6052071245950970, 0.01540741456718481076 ) ) ;
#14174=CARTESIAN_POINT ( 'NONE',  ( -5.935837797515413072, 121.3959224772089129, -0.2928876704554002619 ) ) ;
#14175=CARTESIAN_POINT ( 'NONE',  ( -8.663704466952724559, 118.4235366968212730, 0.7034480781449566900 ) ) ;
#14178=CARTESIAN_POINT ( 'NONE',  ( -5.248704524870183796, 121.2670714900434206, -0.3264022214948025247 ) ) ;
#14179=CARTESIAN_POINT ( 'NONE',  ( 4.980517673276738222, -11.70649569897110709, 0.6972323075040541829 ) ) ;
#14181=CARTESIAN_POINT ( 'NONE',  ( -1.320630737124576903, 159.3505072347868747, 0.9467419726141096392 ) ) ;
#14183=CARTESIAN_POINT ( 'NONE',  ( 13.42863190281024011, 156.9273374874128137, 0.3327859972200289396 ) ) ;
#14185=CARTESIAN_POINT ( 'NONE',  ( 0.6989348986720191892, -4.029744825116962303, 4.573446973323917142 ) ) ;
#14186=CARTESIAN_POINT ( 'NONE',  ( -9.819578298036041986, 117.9942579372833933, -0.2115136170467757371 ) ) ;
#14190=CARTESIAN_POINT ( 'NONE',  ( -6.548379015483123844, 119.7817990349845587, 0.9906393647722963047 ) ) ;
#14191=CARTESIAN_POINT ( 'NONE',  ( -2.488979065607898722, -9.142725400274830605, 3.900846118434742493 ) ) ;
#14192=CARTESIAN_POINT ( 'NONE',  ( 22.06201951068898737, 142.1041199125429557, 1.893492075525809115 ) ) ;
#14194=CARTESIAN_POINT ( 'NONE',  ( 13.26531225419051729, 121.8780043825237982, -1.199064809579205360 ) ) ;
#14195=CARTESIAN_POINT ( 'NONE',  ( 0.6256056815405413030, -8.068247431453825058, 4.577905309659676014 ) ) ;
#14196=CARTESIAN_POINT ( 'NONE',  ( -7.599585376671227799, 158.5456267226934131, -1.164890904197547039 ) ) ;
#14198=CARTESIAN_POINT ( 'NONE',  ( -15.42372963437265376, 147.8340308814284754, 0.02010286832636639515 ) ) ;
#14200=CARTESIAN_POINT ( 'NONE',  ( 5.820489720963992752, -14.55473177801069795, 2.572867947693331381 ) ) ;
#14201=TOROIDAL_SURFACE ( 'NONE', #15539, 3.683000000000000718, 0.5080000000000000071 ) ;
#14205=CARTESIAN_POINT ( 'NONE',  ( 13.91666582400468677, 125.7699432187419575, 2.002145485623347376 ) ) ;
#14206=CARTESIAN_POINT ( 'NONE',  ( 4.946784285683848204, 117.5302610941451178, 0.9662579091233235440 ) ) ;
#14208=CARTESIAN_POINT ( 'NONE',  ( -17.61824099940339750, 125.1652531886817172, 0.6886689253619218132 ) ) ;
#14209=CARTESIAN_POINT ( 'NONE',  ( 7.425401986171529245, 12.64277321918224040, 4.020893088955488359 ) ) ;
#14210=CARTESIAN_POINT ( 'NONE',  ( 4.456531362648481043, 120.8671296916768227, 0.5026912216012411339 ) ) ;
#14212=CARTESIAN_POINT ( 'NONE',  ( 22.91960207526958726, 149.8162411397050278, -0.2683370967508545424 ) ) ;
#14214=CARTESIAN_POINT ( 'NONE',  ( -3.682264917456324671, 101.1854662015457365, -0.07358041635423923088 ) ) ;
#14218=CARTESIAN_POINT ( 'NONE',  ( -4.507460450193894630, 118.1171274854782212, 0.5525917382868535954 ) ) ;
#14219=CARTESIAN_POINT ( 'NONE',  ( 0.3831223070221896343, 105.9763118359730214, -5.290145194802176043 ) ) ;
#14220=ORIENTED_EDGE ( 'NONE', *, *, #18525, .T. ) ;
#14223=CARTESIAN_POINT ( 'NONE',  ( -6.121904736440446193, 119.5860228115829358, -1.252076594595966652 ) ) ;
#14225=CARTESIAN_POINT ( 'NONE',  ( -0.6661646497577808912, 105.9485402691003060, -5.310688274649121077 ) ) ;
#14226=CARTESIAN_POINT ( 'NONE',  ( 4.455728184749551346, 118.1125308307683355, 0.7544055872226939075 ) ) ;
#14227=CARTESIAN_POINT ( 'NONE',  ( -15.86545709684700256, 148.0001117310855250, -1.424070646214982139 ) ) ;
#14228=CARTESIAN_POINT ( 'NONE',  ( -0.9216814595139277699, 115.7029463646975245, -1.750463915914598934 ) ) ;
#14230=CARTESIAN_POINT ( 'NONE',  ( 5.966545996697649734, 118.9610140496397719, -0.3495452691818399238 ) ) ;
#14231=CARTESIAN_POINT ( 'NONE',  ( -7.189601074672337333, 121.4526873951801633, -0.9441605179235378342 ) ) ;
#14233=CARTESIAN_POINT ( 'NONE',  ( -5.260208640450895423, 116.0444662015457595, -1.274361246762516942 ) ) ;
#14235=CARTESIAN_POINT ( 'NONE',  ( 8.663704466952500738, 118.4235366968211736, -0.7034480781449402587 ) ) ;
#14236=CARTESIAN_POINT ( 'NONE',  ( -0.6427210712090456468, 156.3034662015459446, 0.05863295770775731747 ) ) ;
#14238=CARTESIAN_POINT ( 'NONE',  ( 13.19686234056486640, 119.7880570645780978, 0.9111371353940663775 ) ) ;
#14240=CARTESIAN_POINT ( 'NONE',  ( 2.997986829609769366, -15.20712831582179980, 4.056362312997196184 ) ) ;
#14241=CARTESIAN_POINT ( 'NONE',  ( -5.876330432687375982, 119.7498067647950961, 0.9241301181796095499 ) ) ;
#14242=CARTESIAN_POINT ( 'NONE',  ( 0.05045227420522335748, 0.5774631391966889016, 0.9751023907654918776 ) ) ;
#14243=CARTESIAN_POINT ( 'NONE',  ( -14.97360968503865131, 156.1447123740162226, -0.9344295344441083673 ) ) ;
#14244=CARTESIAN_POINT ( 'NONE',  ( 0.4410767147925211407, 14.17415678908661469, -0.8685042294053136880 ) ) ;
#14245=ORIENTED_EDGE ( 'NONE', *, *, #35752, .T. ) ;
#14247=CARTESIAN_POINT ( 'NONE',  ( 7.301789825441145965, 123.0387167848234355, 0.2146691528375952174 ) ) ;
#14248=CARTESIAN_POINT ( 'NONE',  ( -10.17757484390040545, 124.8647468421599598, 0.4356504197092354591 ) ) ;
#14249=CARTESIAN_POINT ( 'NONE',  ( 3.112015045868556928, -14.86597822091932564, 5.561823117377171499 ) ) ;
#14250=CARTESIAN_POINT ( 'NONE',  ( 1.968159265821130877, 156.7095495334699535, -1.232728320231046837 ) ) ;
#14251=ORIENTED_EDGE ( 'NONE', *, *, #2235, .T. ) ;
#14252=CARTESIAN_POINT ( 'NONE',  ( 4.497658079560046041, 104.6144662015457243, 1.758835774636801963 ) ) ;
#14253=CARTESIAN_POINT ( 'NONE',  ( 3.036083976128487016, -13.30543680819082297, 1.158518541688273729 ) ) ;
#14254=CARTESIAN_POINT ( 'NONE',  ( -4.960352205898358235, 117.4682330514041553, -0.9861013956279517378 ) ) ;
#14255=CARTESIAN_POINT ( 'NONE',  ( 15.73538347863339482, 145.6958675726371553, 0.1858358763210238851 ) ) ;
#14258=CARTESIAN_POINT ( 'NONE',  ( 4.088037439073622714, 118.5849532427036905, 0.9900007573961082663 ) ) ;
#14263=CARTESIAN_POINT ( 'NONE',  ( 20.37188742667021657, 129.0035756037533758, 0.2165721192533108241 ) ) ;
#14264=CARTESIAN_POINT ( 'NONE',  ( 4.825036788390894671, 63.33946620154573282, 0.09641571798141751470 ) ) ;
#14265=CARTESIAN_POINT ( 'NONE',  ( 1.854099703272072519, -15.70493002892270340, 5.640771195865757370 ) ) ;
#14267=CARTESIAN_POINT ( 'NONE',  ( -4.986976911676294755, 117.3993830381834726, -0.9021275479513909401 ) ) ;
#14268=CARTESIAN_POINT ( 'NONE',  ( 19.16059698253082999, 135.9655892003723636, 2.351238754465550862 ) ) ;
#14269=ORIENTED_EDGE ( 'NONE', *, *, #22929, .T. ) ;
#14270=CARTESIAN_POINT ( 'NONE',  ( -7.287282906664737325, 21.23368160547805061, -4.223004820119153457 ) ) ;
#14271=B_SPLINE_CURVE_WITH_KNOTS ( 'NONE', 3,
 ( #41729, #32335, #32544, #6155 ),
 .UNSPECIFIED., .F., .F.,
 ( 4, 4 ),
 ( 0.000000000000000000, 1.000000000000000000 ),
 .UNSPECIFIED. ) ;
#14272=CARTESIAN_POINT ( 'NONE',  ( 5.564818521742781243, 117.9257778791303934, -0.8576562958995672670 ) ) ;
#14273=CARTESIAN_POINT ( 'NONE',  ( -1.673685645604704231, 111.6436615656963909, -3.078281589618439451 ) ) ;
#14277=CARTESIAN_POINT ( 'NONE',  ( -0.9211762648548540433, 10.43857344512876040, -4.529598961101950927 ) ) ;
#14279=CARTESIAN_POINT ( 'NONE',  ( -4.844532766435863280, 115.6909491485453003, 1.283482262965630838 ) ) ;
#14280=CARTESIAN_POINT ( 'NONE',  ( 3.301452709780442252, -13.00349394711965090, 1.536261971075179478 ) ) ;
#14281=CARTESIAN_POINT ( 'NONE',  ( 1.341555883842814101, 107.4826764677166864, -4.621745984720207368 ) ) ;
#14283=CARTESIAN_POINT ( 'NONE',  ( 1.963896995744959684, 39.20946620154573026, 1.309496863130310329 ) ) ;
#14285=ORIENTED_EDGE ( 'NONE', *, *, #35816, .T. ) ;
#14286=CARTESIAN_POINT ( 'NONE',  ( -4.689376690405532067, 104.6144662015456959, -1.152304354653030716 ) ) ;
#14287=CARTESIAN_POINT ( 'NONE',  ( 2.110750219194173827, -15.67940412490098723, 5.433654451060461632 ) ) ;
#14288=CARTESIAN_POINT ( 'NONE',  ( -19.88689915616629378, 147.6055923437354238, 1.726923636697636599 ) ) ;
#14289=CARTESIAN_POINT ( 'NONE',  ( -1.504723661876595786, -8.552649586842417051, -4.374500482163298898 ) ) ;
#14292=CARTESIAN_POINT ( 'NONE',  ( -4.468667403750213651, 27.88063884994054220, 0.5133561255362272258 ) ) ;
#14293=CARTESIAN_POINT ( 'NONE',  ( 1.585818144368541960, 119.1892773189224783, 0.7268676395674206203 ) ) ;
#14294=CARTESIAN_POINT ( 'NONE',  ( -10.91797240702851290, 124.6990478933366404, 0.8611562105571396453 ) ) ;
#14295=CARTESIAN_POINT ( 'NONE',  ( -6.484670282503085616E-14, 71.97546620154574271, 3.533028205012241021E-29 ) ) ;
#14296=CARTESIAN_POINT ( 'NONE',  ( 12.23061257473121088, 124.2599011343719155, -1.262879005329815341 ) ) ;
#14297=CARTESIAN_POINT ( 'NONE',  ( -13.40750253236534917, 122.4565580348552913, -1.800089891214285531 ) ) ;
#14299=CARTESIAN_POINT ( 'NONE',  ( 4.269133473500895448, 118.2238350903788131, -0.2888805705710837946 ) ) ;
#14300=CARTESIAN_POINT ( 'NONE',  ( 14.89139266796658845, 148.8756053271976327, -0.4181552259878849598 ) ) ;
#14302=CARTESIAN_POINT ( 'NONE',  ( 3.047145566129288330, -14.72663143740328806, 3.823360744794035870 ) ) ;
#14306=CARTESIAN_POINT ( 'NONE',  ( 4.471266627501615076, -5.469457446779734333, -1.220754042301255948 ) ) ;
#14307=CARTESIAN_POINT ( 'NONE',  ( 15.77815547270811791, 139.7295799824062499, 1.909820663798255325 ) ) ;
#14308=CARTESIAN_POINT ( 'NONE',  ( -3.521685918548247418, 29.33394459973516888, 3.031038535435704340 ) ) ;
#14309=CARTESIAN_POINT ( 'NONE',  ( -4.039333660417916860, 117.0582680968029905, 0.9406562914258045360 ) ) ;
#14312=CARTESIAN_POINT ( 'NONE',  ( -1.756104463947763206, 14.33678105357426702, 4.288642365192034234 ) ) ;
#14313=CARTESIAN_POINT ( 'NONE',  ( 0.6411011158478991945, 120.9975462804897433, 0.03814546805551061875 ) ) ;
#14317=CARTESIAN_POINT ( 'NONE',  ( -2.169587742970651156, 116.2588381394661354, -0.2119676221548945638 ) ) ;
#14318=CARTESIAN_POINT ( 'NONE',  ( 0.003073426023161661153, 123.4679809879534247, -0.1538068059577044622 ) ) ;
#14320=CARTESIAN_POINT ( 'NONE',  ( -2.100979515209699944, 106.6614287958282858, 4.900381384812394714 ) ) ;
#14323=CARTESIAN_POINT ( 'NONE',  ( 8.429690783291841072, 7.639065531857588631, 0.01617727833786941974 ) ) ;
#14326=CARTESIAN_POINT ( 'NONE',  ( 0.003073426022489101923, 123.4679809879534247, -0.1538068059577179236 ) ) ;
#14327=CARTESIAN_POINT ( 'NONE',  ( -22.40468623258675507, 137.0915487549672491, 0.1281257692620775268 ) ) ;
#14328=ORIENTED_EDGE ( 'NONE', *, *, #11061, .F. ) ;
#14334=CARTESIAN_POINT ( 'NONE',  ( -15.78437780952707215, 146.2378312303354448, -0.3154094333657934679 ) ) ;
#14335=CARTESIAN_POINT ( 'NONE',  ( 5.122375111755775201, -14.64399685039916044, 3.991980633533394052 ) ) ;
#14336=CARTESIAN_POINT ( 'NONE',  ( -20.96550312372672664, 148.3608207065297222, 1.563628808460498787 ) ) ;
#14337=CARTESIAN_POINT ( 'NONE',  ( 15.50334291652339580, 121.0440340969820596, 0.8284681841690884063 ) ) ;
#14338=CARTESIAN_POINT ( 'NONE',  ( 12.83198513809769636, 156.8686255264331635, -0.8772202223719092196 ) ) ;
#14340=CARTESIAN_POINT ( 'NONE',  ( 0.002459401150240396027, 159.6023738651833810, -0.1230784904792617679 ) ) ;
#14343=CARTESIAN_POINT ( 'NONE',  ( 5.562407744872148285, 116.6996333493949436, 0.1111501445372547886 ) ) ;
#14344=CARTESIAN_POINT ( 'NONE',  ( -4.309327875669019647, 119.9149831030956932, 0.7077533764146595185 ) ) ;
#14346=CARTESIAN_POINT ( 'NONE',  ( 18.61143607275140965, 150.2488615152233820, -1.729315005182988196 ) ) ;
#14347=CARTESIAN_POINT ( 'NONE',  ( -4.583145339711863109, 27.87760190725156662, 0.5120832130453706332 ) ) ;
#14348=CARTESIAN_POINT ( 'NONE',  ( -10.72975491961958383, 119.6772744462923157, -1.366487948980413147 ) ) ;
#14351=CARTESIAN_POINT ( 'NONE',  ( 16.52109770691737722, 146.2355833862463328, -0.9494891650916719161 ) ) ;
#14352=CARTESIAN_POINT ( 'NONE',  ( -15.72385166996626715, 146.8976323831864477, -0.3141999770531619940 ) ) ;
#14353=ORIENTED_EDGE ( 'NONE', *, *, #19378, .T. ) ;
#14354=CARTESIAN_POINT ( 'NONE',  ( -15.37772490044532070, 131.3329289045130679, -2.176645470406190608 ) ) ;
#14355=CARTESIAN_POINT ( 'NONE',  ( 4.438132741721911856, -15.66483130081081043, 3.040968155030625120 ) ) ;
#14357=CARTESIAN_POINT ( 'NONE',  ( -4.291595391187098762, 118.2137919694442019, -0.5063013721726838945 ) ) ;
#14360=CARTESIAN_POINT ( 'NONE',  ( 4.112379816251298337, 118.2429491485453354, 0.3456808358118761970 ) ) ;
#14361=CARTESIAN_POINT ( 'NONE',  ( -0.01023306027097531379, 119.5380416804913324, 0.5121041807152043601 ) ) ;
#14362=FACE_OUTER_BOUND ( 'NONE', #38499, .T. ) ;
#14364=CARTESIAN_POINT ( 'NONE',  ( 18.86374853661768825, 125.3403196291361610, 0.3769425889880998470 ) ) ;
#14365=EDGE_CURVE ( 'NONE', #30834, #19419, #16530, .T. ) ;
#14366=CARTESIAN_POINT ( 'NONE',  ( 4.103208822911150300, 18.85939590645278585, -7.354229849909827088 ) ) ;
#14367=CARTESIAN_POINT ( 'NONE',  ( 6.089391457280314945, 155.3491548655973133, 0.5861119247043798941 ) ) ;
#14368=CARTESIAN_POINT ( 'NONE',  ( 22.76023949468076069, 146.4845460041848355, -0.7370798038890573611 ) ) ;
#14371=CARTESIAN_POINT ( 'NONE',  ( 3.195221254476268591, 115.6909491485452435, 1.660623339098961093 ) ) ;
#14374=CARTESIAN_POINT ( 'NONE',  ( -23.35954322469569178, 148.8716009884483071, -0.3896314068422417898 ) ) ;
#14377=CARTESIAN_POINT ( 'NONE',  ( -6.873076553849402082, 121.7066554103861620, -0.6264859833759695018 ) ) ;
#14379=VERTEX_POINT ( 'NONE', #832 ) ;
#14380=CARTESIAN_POINT ( 'NONE',  ( 4.459091033076425070, 115.6909491485368306, -1.361484950952978279 ) ) ;
#14381=CARTESIAN_POINT ( 'NONE',  ( -10.44459398727727262, 153.0728660266736370, -0.5066767128784233076 ) ) ;
#14382=CARTESIAN_POINT ( 'NONE',  ( 4.035643413487081332, -14.09208526182970189, 4.581805149448960002 ) ) ;
#14384=CARTESIAN_POINT ( 'NONE',  ( -21.39260515875404778, 150.3702682424204511, 1.149856210633945830 ) ) ;
#14386=AXIS2_PLACEMENT_3D ( 'NONE', #16478, #26067, #20086 ) ;
#14387=CARTESIAN_POINT ( 'NONE',  ( 18.76446887325675661, 125.2887878443791294, 0.4910110098351363472 ) ) ;
#14388=CARTESIAN_POINT ( 'NONE',  ( 1.558509422354653839, 156.2601852824606681, 0.06968051580646485166 ) ) ;
#14389=VERTEX_POINT ( 'NONE', #4871 ) ;
#14390=CARTESIAN_POINT ( 'NONE',  ( 0.8728101606606677443, 18.85996454746999618, -0.4358653558870161926 ) ) ;
#14391=CARTESIAN_POINT ( 'NONE',  ( -23.34271727006419539, 149.0672090665632936, -0.4921983935722529235 ) ) ;
#14396=CARTESIAN_POINT ( 'NONE',  ( 4.555470457886838354, 118.7543979957781488, 1.067760081256754034 ) ) ;
#14397=CARTESIAN_POINT ( 'NONE',  ( -3.769861741716944881, -2.021032284792064093, -2.673854242032364326 ) ) ;
#14398=CARTESIAN_POINT ( 'NONE',  ( 2.976591712665050515, 117.3922842568077698, 0.6615242749010382672 ) ) ;
#14400=CARTESIAN_POINT ( 'NONE',  ( 19.52548538990935612, 136.0480396440595996, -1.529100095608182608 ) ) ;
#14401=CARTESIAN_POINT ( 'NONE',  ( -4.540528814728789442, -1.371322978654152092, -0.8806307088788817294 ) ) ;
#14402=CARTESIAN_POINT ( 'NONE',  ( -6.873244579178622082, 117.6856483911789581, -0.8154597436780148811 ) ) ;
#14405=CARTESIAN_POINT ( 'NONE',  ( -14.24343488940578162, 138.9464670490549452, -0.05414037600900920011 ) ) ;
#14406=EDGE_CURVE ( 'NONE', #10361, #40008, #24802, .T. ) ;
#14407=CARTESIAN_POINT ( 'NONE',  ( 4.690731670358166738, -15.11132977793584686, 4.439372980131230939 ) ) ;
#14408=CARTESIAN_POINT ( 'NONE',  ( 5.012350601733652766, 115.6909491485453145, 1.400347971660041990 ) ) ;
#14409=EDGE_CURVE ( 'NONE', #38197, #4283, #36404, .T. ) ;
#14410=CARTESIAN_POINT ( 'NONE',  ( 0.01782677789211616418, 118.1651005001175889, -0.8921251404964753995 ) ) ;
#14412=CARTESIAN_POINT ( 'NONE',  ( 3.256054338613350474, 118.9727644790723531, 0.9029027703446365072 ) ) ;
#14416=CARTESIAN_POINT ( 'NONE',  ( -22.39452804842998646, 149.5981344557702641, 0.8550856607202137472 ) ) ;
#14417=CARTESIAN_POINT ( 'NONE',  ( 4.653112868187331941, 2.303567304790777648, 7.043327697551765354 ) ) ;
#14418=CARTESIAN_POINT ( 'NONE',  ( 14.76847666019552463, 139.2804412874323248, 1.275673245633013542 ) ) ;
#14420=EDGE_CURVE ( 'NONE', #18326, #8589, #40643, .T. ) ;
#14421=CARTESIAN_POINT ( 'NONE',  ( 1.919474982883598191, 116.7789519286944966, -0.2705014076049041538 ) ) ;
#14423=( NAMED_UNIT ( * ) PLANE_ANGLE_UNIT ( ) SI_UNIT ( $, .RADIAN. ) );
#14426=CARTESIAN_POINT ( 'NONE',  ( -4.172365507229960357, 118.2392283616613042, 0.2172622651388938786 ) ) ;
#14427=CARTESIAN_POINT ( 'NONE',  ( 2.005054034524792694, 106.7498038803853291, -4.871448594665350740 ) ) ;
#14428=ORIENTED_EDGE ( 'NONE', *, *, #5832, .F. ) ;
#14430=CARTESIAN_POINT ( 'NONE',  ( -6.231363852629784539, 119.8171196943256405, -1.230295645515693481 ) ) ;
#14431=CARTESIAN_POINT ( 'NONE',  ( -5.166232791442098460, 115.4535745449993982, -1.513138011745335909 ) ) ;
#14432=CARTESIAN_POINT ( 'NONE',  ( 4.388083867990050457, 118.1817479911534861, 0.5768821283915082088 ) ) ;
#14433=CARTESIAN_POINT ( 'NONE',  ( 0.01341678693497577735, 156.4123495908283985, -0.6714308817992609146 ) ) ;
#14435=CARTESIAN_POINT ( 'NONE',  ( 5.772319165917887851, 116.9338547871927858, 0.1153446742911717476 ) ) ;
#14437=CARTESIAN_POINT ( 'NONE',  ( 2.184544675937996061, 106.6795586461009009, -4.886581511092879637 ) ) ;
#14438=CARTESIAN_POINT ( 'NONE',  ( -3.555938004931326724, 120.5283240077024800, -0.5587344792657804593 ) ) ;
#14443=CARTESIAN_POINT ( 'NONE',  ( -12.77395747310483642, 133.6867917047960930, -0.07034420110178993268 ) ) ;
#14445=CARTESIAN_POINT ( 'NONE',  ( 4.811924804297746938, 117.0737178285515654, 0.5427311436463463368 ) ) ;
#14447=CARTESIAN_POINT ( 'NONE',  ( 2.567065079198288746, -15.08448375773686934, 4.691402903081304920 ) ) ;
#14448=CARTESIAN_POINT ( 'NONE',  ( 21.81117068996439556, 146.0876064316611860, -1.285479812297503743 ) ) ;
#14449=CARTESIAN_POINT ( 'NONE',  ( -3.371641211477255151, 119.4525916976722897, 0.7211689390744321360 ) ) ;
#14450=CARTESIAN_POINT ( 'NONE',  ( 0.3265437062995015238, -4.820036860806069967, -0.9201843903956486992 ) ) ;
#14451=CARTESIAN_POINT ( 'NONE',  ( -2.866641708098142338, 116.8851979753409580, -0.4370437109847168378 ) ) ;
#14453=CARTESIAN_POINT ( 'NONE',  ( -0.4694259674403166716, 18.92165170904731397, 0.8533247626313392731 ) ) ;
#14456=CARTESIAN_POINT ( 'NONE',  ( -5.892782515047567671, 121.3091694753028520, 0.3064017138515003902 ) ) ;
#14457=CARTESIAN_POINT ( 'NONE',  ( 4.939475803799734166, -12.60685243851100701, 2.184682653711520040 ) ) ;
#14458=CARTESIAN_POINT ( 'NONE',  ( 3.514252322483260471, 120.2313485970928326, -0.5318214084310806111 ) ) ;
#14460=CARTESIAN_POINT ( 'NONE',  ( 1.647191010927073762, 104.6144662015456532, 4.545328324975800527 ) ) ;
#14462=CARTESIAN_POINT ( 'NONE',  ( 3.250423480262735421, -14.11372661294146802, 3.006569077614236196 ) ) ;
#14463=CARTESIAN_POINT ( 'NONE',  ( -4.804485507087670193, 117.6428313260155960, -1.111657494208010188 ) ) ;
#14464=CARTESIAN_POINT ( 'NONE',  ( 7.558302675500184087, 122.4263405438208991, 0.1204446389788525473 ) ) ;
#14465=AXIS2_PLACEMENT_3D ( 'NONE', #38595, #22367, #6221 ) ;
#14468=CARTESIAN_POINT ( 'NONE',  ( 1.082660538731414990, 158.4310823543925721, 1.603207764552047054 ) ) ;
#14469=CARTESIAN_POINT ( 'NONE',  ( 3.583481579166091446, 109.6950698699342865, 3.736516032388299546 ) ) ;
#14473=CARTESIAN_POINT ( 'NONE',  ( 9.797860116729928848, 118.0024801742749929, 0.05693907317356660530 ) ) ;
#14474=DIRECTION ( 'NONE',  ( -4.017660918040594346E-17, 1.000000000000000000, 2.376309959284834438E-19 ) ) ;
#14475=CIRCLE ( 'NONE', #32870, 3.175000000000001155 ) ;
#14476=CARTESIAN_POINT ( 'NONE',  ( 2.041957097679553801, -15.35386704983179840, 5.998528387730076794 ) ) ;
#14479=CARTESIAN_POINT ( 'NONE',  ( -4.801861765505079482, 117.8465146159224588, 0.7715805027661067905 ) ) ;
#14481=CARTESIAN_POINT ( 'NONE',  ( -7.546363725996330984, 11.73557930518083303, -3.739946900464478752 ) ) ;
#14482=CARTESIAN_POINT ( 'NONE',  ( 8.455193764574449489, 119.4765705532822722, -1.058376901205021259 ) ) ;
#14483=CARTESIAN_POINT ( 'NONE',  ( -2.616318351458581937, 112.7379566594982663, -2.676765618731039797 ) ) ;
#14484=CARTESIAN_POINT ( 'NONE',  ( 4.744914421628031675, 117.7318590736328758, 1.087530422288184528 ) ) ;
#14486=CARTESIAN_POINT ( 'NONE',  ( -4.808149584360944750, 104.6144662015457527, 0.4147572885131461939 ) ) ;
#14487=CARTESIAN_POINT ( 'NONE',  ( -4.550674770548566173, 2.667180226961371137, -0.8080508602523945871 ) ) ;
#14489=CARTESIAN_POINT ( 'NONE',  ( -5.277380552522624946, 115.6909491485453003, 0.8071570353046304547 ) ) ;
#14490=CARTESIAN_POINT ( 'NONE',  ( 3.093634585129180881, -14.37226628243755400, 4.703574289890697813 ) ) ;
#14491=CARTESIAN_POINT ( 'NONE',  ( 4.257294657327800103, 122.9893884486272526, -0.03029934543357437962 ) ) ;
#14492=CARTESIAN_POINT ( 'NONE',  ( 0.2644822807012546795, 35.23508677173605719, 3.013287348562808443 ) ) ;
#14493=CARTESIAN_POINT ( 'NONE',  ( -2.065088524322160612, 115.7028725816649057, 1.634879246183956081 ) ) ;
#14495=FACE_OUTER_BOUND ( 'NONE', #7462, .T. ) ;
#14496=CARTESIAN_POINT ( 'NONE',  ( 2.260827880841108417, -15.68886294521955271, 5.354637041555423416 ) ) ;
#14497=CARTESIAN_POINT ( 'NONE',  ( -12.76794581240270254, 122.4237789811383550, 1.308419224297318051 ) ) ;
#14498=CARTESIAN_POINT ( 'NONE',  ( -0.8176680875534481086, 23.83313504737664346, 0.5327793711180701663 ) ) ;
#14501=CARTESIAN_POINT ( 'NONE',  ( -4.469853575504566301, 31.48943071249222214, -0.6923489671027511783 ) ) ;
#14502=CARTESIAN_POINT ( 'NONE',  ( -0.02647280040265726289, 106.0860833631645193, 5.252669131072540409 ) ) ;
#14503=SHAPE_REPRESENTATION_RELATIONSHIP ( 'NONE' , 'NONE' ,  #19076, #22381 ) ;
#14504=CARTESIAN_POINT ( 'NONE',  ( -2.657114488131365970, 120.4390018212493914, 0.3871174720959881244 ) ) ;
#14505=DIRECTION ( 'NONE',  ( -0.9998004120163609398, 0.000000000000000000, -0.01997839162482749689 ) ) ;
#14507=CARTESIAN_POINT ( 'NONE',  ( 4.623422138725822528, 118.0605935606111672, -0.5413340251631463262 ) ) ;
#14508=CARTESIAN_POINT ( 'NONE',  ( 2.165411683282626232, 157.1282018749678002, -1.500011447693321065 ) ) ;
#14510=CARTESIAN_POINT ( 'NONE',  ( -6.672308397275299896, 157.8130281244853279, -1.874701415657104242 ) ) ;
#14511=FACE_BOUND ( 'NONE', #13673, .T. ) ;
#14514=CARTESIAN_POINT ( 'NONE',  ( 4.411902438606213117, 118.1805500072961337, -0.3959976634185874422 ) ) ;
#14516=CARTESIAN_POINT ( 'NONE',  ( 9.094799215789642233, 123.6795089456687577, -0.2292421281602768091 ) ) ;
#14518=CARTESIAN_POINT ( 'NONE',  ( 3.198896590522081862, -14.38863201745455100, 2.123570546440393780 ) ) ;
#14519=CARTESIAN_POINT ( 'NONE',  ( -4.997723913362575487, 117.4043970260275813, 0.8231665828273773133 ) ) ;
#14522=CARTESIAN_POINT ( 'NONE',  ( -4.627572956979934204, -1.171460759993483647, -0.2796867628226345492 ) ) ;
#14523=CARTESIAN_POINT ( 'NONE',  ( 17.23442203377886628, 146.5563353440282981, 2.056614067264090906 ) ) ;
#14524=CARTESIAN_POINT ( 'NONE',  ( -1.788360971357598750, 31.32134090374974633, 3.767248576702360907 ) ) ;
#14525=CARTESIAN_POINT ( 'NONE',  ( -4.753511127315711349, 115.8251506319059843, 1.256829922054842008 ) ) ;
#14527=CARTESIAN_POINT ( 'NONE',  ( 1.068493265602401987, 5.690783753869971484, 4.496582723949734017 ) ) ;
#14528=CARTESIAN_POINT ( 'NONE',  ( 9.566940353391197860, 124.8108731098830049, 0.2265937611309802591 ) ) ;
#14531=CARTESIAN_POINT ( 'NONE',  ( -8.781393967084220264, 117.7409677532042735, -0.4282185732264804368 ) ) ;
#14532=DIRECTION ( 'NONE',  ( 4.017660918040594346E-17, -1.000000000000000000, -2.376309959284834438E-19 ) ) ;
#14535=CARTESIAN_POINT ( 'NONE',  ( -0.1058213901578662491, 105.9761915687788587, 5.295735085525936192 ) ) ;
#14537=CARTESIAN_POINT ( 'NONE',  ( -8.022552064266685434, 3.315157024569945765, 2.561087356634513590 ) ) ;
#14540=CARTESIAN_POINT ( 'NONE',  ( 1.824654213811243819, -15.25386490109567639, 5.420715704377902178 ) ) ;
#14541=CARTESIAN_POINT ( 'NONE',  ( 0.003708075273124115685, 123.1683257372384901, -0.1855672496570449914 ) ) ;
#14542=CARTESIAN_POINT ( 'NONE',  ( -0.004913308686094480619, 116.7872217978203224, 0.2458820580207660422 ) ) ;
#14543=ORIENTED_EDGE ( 'NONE', *, *, #2714, .T. ) ;
#14547=CARTESIAN_POINT ( 'NONE',  ( -12.85860202769644545, 133.7716054015561156, -0.2569454702854386263 ) ) ;
#14548=CARTESIAN_POINT ( 'NONE',  ( 5.819126084642364916, -14.14507005385615201, 2.709888076677010371 ) ) ;
#14549=CARTESIAN_POINT ( 'NONE',  ( -20.91036014055508829, 148.6614476615901594, 1.563091210272363307 ) ) ;
#14551=CARTESIAN_POINT ( 'NONE',  ( 22.60445334873316270, 148.5212373274837319, -0.8566365145943198867 ) ) ;
#14552=CARTESIAN_POINT ( 'NONE',  ( -2.029258473809828711, 23.83235028914373288, 4.157303687431403993 ) ) ;
#14553=CARTESIAN_POINT ( 'NONE',  ( -8.021187395864899372, 158.6806155330135084, -0.3964977924059485126 ) ) ;
#14555=ORIENTED_EDGE ( 'NONE', *, *, #11284, .F. ) ;
#14557=CARTESIAN_POINT ( 'NONE',  ( -11.89126842552456509, 124.3826620800890339, 1.187748846906861777 ) ) ;
#14559=CARTESIAN_POINT ( 'NONE',  ( 18.94087081963948549, 148.8558894138562039, -1.735487911102014946 ) ) ;
#14560=TOROIDAL_SURFACE ( 'NONE', #303, 5.080000000000005400, 0.5080000000000000071 ) ;
#14561=CARTESIAN_POINT ( 'NONE',  ( -6.809904206821648209, 118.2876074772933492, -1.086328812139342848 ) ) ;
#14564=CARTESIAN_POINT ( 'NONE',  ( 2.684237737021673453, 120.5579296053302727, -0.3360084551914348516 ) ) ;
#14566=CARTESIAN_POINT ( 'NONE',  ( -18.05261769607656319, 144.6555253171603397, -2.402359405240794832 ) ) ;
#14567=CARTESIAN_POINT ( 'NONE',  ( 4.028426573186930426, -15.65323953938244017, 3.316845843096514201 ) ) ;
#14569=CARTESIAN_POINT ( 'NONE',  ( -4.296542858503126006, 118.2130224152798945, -0.5011208106148314911 ) ) ;
#14572=CARTESIAN_POINT ( 'NONE',  ( 10.13131171838191413, 122.2967958330617648, 1.512676856611740783 ) ) ;
#14573=CARTESIAN_POINT ( 'NONE',  ( 3.682264917456192777, 82.13546620154573930, 0.07358041635423970273 ) ) ;
#14574=CARTESIAN_POINT ( 'NONE',  ( 0.2965531742115425917, 116.4333835968663919, -0.03207532894271091645 ) ) ;
#14575=CARTESIAN_POINT ( 'NONE',  ( 3.113543590025587005, -0.1312883392403825233, -7.836836066719057747 ) ) ;
#14576=CARTESIAN_POINT ( 'NONE',  ( 11.46436990449499760, 128.2561452373498980, 0.7395913538610451310 ) ) ;
#14577=CARTESIAN_POINT ( 'NONE',  ( 3.879144173866336143, 118.0219252979734677, -0.8163251714509417445 ) ) ;
#14579=CARTESIAN_POINT ( 'NONE',  ( 1.176010826768138173, 105.9617161350778787, -5.207309035134176867 ) ) ;
#14580=CARTESIAN_POINT ( 'NONE',  ( -8.060487153020286399, 121.1729579957945901, -1.292971159565753148 ) ) ;
#14582=CARTESIAN_POINT ( 'NONE',  ( -14.84180086987441172, 120.3134675335783754, -0.1939203138368897072 ) ) ;
#14585=CARTESIAN_POINT ( 'NONE',  ( 6.878842811470913254, 121.5723321815868871, -0.4547243280587507375 ) ) ;
#14586=CARTESIAN_POINT ( 'NONE',  ( -7.819596425554085073, 122.5025573185424435, 0.1851470016872596713 ) ) ;
#14588=CARTESIAN_POINT ( 'NONE',  ( 0.4158179766845868097, 118.7629491485454025, -1.264088747447795980 ) ) ;
#14589=CARTESIAN_POINT ( 'NONE',  ( -9.737435037572492291, 124.8671652961716489, -0.4371131421146304818 ) ) ;
#14590=CARTESIAN_POINT ( 'NONE',  ( 2.601617458372238900, -15.08031326607275879, 5.801161347629554044 ) ) ;
#14591=CARTESIAN_POINT ( 'NONE',  ( -12.29982474031040596, 156.6574886424908470, 1.289654987246354079 ) ) ;
#14593=CARTESIAN_POINT ( 'NONE',  ( 16.10347893962645216, 121.2391669109744186, 0.4275719782727096518 ) ) ;
#14594=CARTESIAN_POINT ( 'NONE',  ( 7.544955551308853536, 122.4259255053487436, 0.1906877313379402028 ) ) ;
#14595=ORIENTED_EDGE ( 'NONE', *, *, #39114, .F. ) ;
#14596=CARTESIAN_POINT ( 'NONE',  ( 0.9036657058557058253, 17.56215383894848614, 0.3677562154327245758 ) ) ;
#14597=CARTESIAN_POINT ( 'NONE',  ( -15.54780490071038024, 120.7212560704218589, -0.3275748350740994019 ) ) ;
#14603=CARTESIAN_POINT ( 'NONE',  ( 8.390685855369055091, 119.5507258284018093, 1.408871319322181792 ) ) ;
#14604=CARTESIAN_POINT ( 'NONE',  ( 3.174366308151880034, 97.37546620154573418, 0.06343139340882766875 ) ) ;
#14605=CARTESIAN_POINT ( 'NONE',  ( 2.957233306982478105, 159.1263692740743068, 1.212116333074086283 ) ) ;
#14607=CARTESIAN_POINT ( 'NONE',  ( 17.80465198604232313, 131.6735282812448986, -1.559227381006986990 ) ) ;
#14608=CARTESIAN_POINT ( 'NONE',  ( -8.365627035046871995, 27.56796056798338057, -1.282220400777004388 ) ) ;
#14609=CARTESIAN_POINT ( 'NONE',  ( -3.104962560943469896, 159.3365417412370562, -0.8543937160244109430 ) ) ;
#14610=CARTESIAN_POINT ( 'NONE',  ( 4.942462214789340891, 117.6285031199090412, -0.7735160008196966253 ) ) ;
#14613=CARTESIAN_POINT ( 'NONE',  ( -0.003550340867792285433, 156.3099534201614631, 0.1776735749810083032 ) ) ;
#14614=CARTESIAN_POINT ( 'NONE',  ( 4.127870218248371970, -15.50624122109489633, 4.747786349039386344 ) ) ;
#14616=CARTESIAN_POINT ( 'NONE',  ( -0.3814255583757257817, 118.1651003383654768, -0.8943798372417751663 ) ) ;
#14618=VERTEX_POINT ( 'NONE', #15479 ) ;
#14620=CARTESIAN_POINT ( 'NONE',  ( 0.9722352627952559612, 157.7941190989783991, 1.644571785473256220 ) ) ;
#14621=DIRECTION ( 'NONE',  ( 0.9998004120163608288, 0.000000000000000000, 0.01997839162482749342 ) ) ;
#14623=CARTESIAN_POINT ( 'NONE',  ( -1.626581124784322929, 119.3928400758114918, 0.6183738137425960346 ) ) ;
#14624=CARTESIAN_POINT ( 'NONE',  ( 6.022233187337456606, 12.22246943312702427, 5.887876567768997482 ) ) ;
#14625=CARTESIAN_POINT ( 'NONE',  ( 8.219871311007414860, 154.6505398758502849, 1.119353551822957149 ) ) ;
#14628=CARTESIAN_POINT ( 'NONE',  ( 15.52406334459478465, 121.0440340969820596, -0.2084667659489262137 ) ) ;
#14630=DIRECTION ( 'NONE',  ( -5.206863593109713661E-17, 1.000000000000000000, -1.077750396879097183E-30 ) ) ;
#14634=CARTESIAN_POINT ( 'NONE',  ( 2.071654280177505303, -15.34349575202162974, 5.977339193430268871 ) ) ;
#14635=CARTESIAN_POINT ( 'NONE',  ( -4.313832278175046220, 118.2128970912768438, 0.3282138498878479638 ) ) ;
#14636=ORIENTED_EDGE ( 'NONE', *, *, #20675, .F. ) ;
#14639=CARTESIAN_POINT ( 'NONE',  ( 6.198907113810094849, 119.6457338356565430, -1.000577012762424944 ) ) ;
#14640=CARTESIAN_POINT ( 'NONE',  ( -6.937169949972989080, 121.8132169909553966, -0.2949249740950673493 ) ) ;
#14641=CARTESIAN_POINT ( 'NONE',  ( 4.252925440392405498, 118.2240520237851626, 0.4605658090341683275 ) ) ;
#14642=CARTESIAN_POINT ( 'NONE',  ( -3.037839899926094489, 156.1243923452879017, -0.6481072647156851385 ) ) ;
#14646=CARTESIAN_POINT ( 'NONE',  ( -1.932895124392534303, 20.38400505531995321, -4.219463811995566083 ) ) ;
#14647=CARTESIAN_POINT ( 'NONE',  ( -16.29178962149237009, 143.9496486471311698, -1.781768755694404849 ) ) ;
#14649=CARTESIAN_POINT ( 'NONE',  ( -3.148524768479886937, 30.89467502894792972, -0.4672404312464801812 ) ) ;
#14651=CARTESIAN_POINT ( 'NONE',  ( 6.989538638170239793, 121.9084849004810138, 0.3647075761099029534 ) ) ;
#14652=DIRECTION ( 'NONE',  ( -0.01997839162482761832, -1.040247600000950455E-18, 0.9998004120163610509 ) ) ;
#14653=CARTESIAN_POINT ( 'NONE',  ( 22.71086789718616572, 148.5871737753741115, 1.637050152828072314 ) ) ;
#14655=CARTESIAN_POINT ( 'NONE',  ( 3.117629155811438402, -14.23119940253145188, 1.544136867890079090 ) ) ;
#14656=CARTESIAN_POINT ( 'NONE',  ( 5.066682439019537298, 158.5910778905036977, -1.349075717862105561 ) ) ;
#14657=CARTESIAN_POINT ( 'NONE',  ( -6.663576545388717243, 119.9895581359321994, 0.9799952387295398637 ) ) ;
#14658=CARTESIAN_POINT ( 'NONE',  ( -0.6014681082635296994, -0.5174402789662015945, 0.7683055774679631300 ) ) ;
#14659=CARTESIAN_POINT ( 'NONE',  ( -22.23561040172140579, 150.7043692363948537, -1.289434558007279685 ) ) ;
#14660=CARTESIAN_POINT ( 'NONE',  ( -0.7801697309092696653, 18.27050645547500451, 0.5824522774875325881 ) ) ;
#14664=CARTESIAN_POINT ( 'NONE',  ( -9.384706802269613846, 123.8909350679826815, 0.3250447036211730478 ) ) ;
#14665=CARTESIAN_POINT ( 'NONE',  ( 3.194768752100229925, -14.65262985833884457, 5.377959301279905624 ) ) ;
#14666=CARTESIAN_POINT ( 'NONE',  ( 0.008945177887880035456, 119.9096241394016715, -0.4476532798976761707 ) ) ;
#14668=CARTESIAN_POINT ( 'NONE',  ( 0.3866447666624587276, 115.7034473292545584, 1.763797082902897495 ) ) ;
#14670=CARTESIAN_POINT ( 'NONE',  ( 3.154677723130417277, -14.38507846778283650, 3.622984934187011952 ) ) ;
#14671=CARTESIAN_POINT ( 'NONE',  ( -4.760401155226894332, 117.7660915045744190, -1.056044474819750834 ) ) ;
#14672=CARTESIAN_POINT ( 'NONE',  ( 9.614588335866148583, 124.8310256250372277, 0.1039111448415540317 ) ) ;
#14674=CARTESIAN_POINT ( 'NONE',  ( 20.31017440411229202, 148.4497675966422889, 2.477828910454907607 ) ) ;
#14677=CARTESIAN_POINT ( 'NONE',  ( 0.01341678693497577735, 156.4123495908283985, -0.6714308817992609146 ) ) ;
#14679=CARTESIAN_POINT ( 'NONE',  ( 22.59814275696091812, 137.2245694613254443, 0.1355511068837784994 ) ) ;
#14682=CARTESIAN_POINT ( 'NONE',  ( 2.099639488158107081, -15.34085824818334842, 5.967397557607278635 ) ) ;
#14684=CARTESIAN_POINT ( 'NONE',  ( -4.957032329879782040, 117.5911933634104543, -0.8969954988694857079 ) ) ;
#14685=CARTESIAN_POINT ( 'NONE',  ( -4.623803002916879734, 117.9758317316280198, 0.7387004689016926084 ) ) ;
#14688=CARTESIAN_POINT ( 'NONE',  ( 4.854633716284414646, 115.7029491485453292, -1.279498648767039448 ) ) ;
#14689=EDGE_CURVE ( 'NONE', #29613, #11330, #29414, .T. ) ;
#14690=CARTESIAN_POINT ( 'NONE',  ( 5.606335446380697363, 118.1214203281341781, -0.9042019091217482485 ) ) ;
#14691=CARTESIAN_POINT ( 'NONE',  ( -2.486440349385922843, 120.2382744777187611, -0.5044468955786924891 ) ) ;
#14692=CARTESIAN_POINT ( 'NONE',  ( 4.830107420232238269, 117.5457777486666089, 1.145229895618746774 ) ) ;
#14694=CARTESIAN_POINT ( 'NONE',  ( -0.1065646865916158176, 105.8844662015456919, 5.332932678536313809 ) ) ;
#14695=CARTESIAN_POINT ( 'NONE',  ( 4.326043401919948295, 8.289558097378858292, -1.648119079657388353 ) ) ;
#14698=CARTESIAN_POINT ( 'NONE',  ( -0.4455429663221430192, 105.8200183450921941, -5.321466673365036648 ) ) ;
#14699=CARTESIAN_POINT ( 'NONE',  ( 3.944052607038018632, -12.86033490357471543, 2.408110524499547100 ) ) ;
#14700=CARTESIAN_POINT ( 'NONE',  ( 5.282628607151995226, 116.7267603939287426, -0.8077565746219077525 ) ) ;
#14701=CARTESIAN_POINT ( 'NONE',  ( -3.938977128594350230, 28.07268674286775578, 0.7495841607770368231 ) ) ;
#14702=CARTESIAN_POINT ( 'NONE',  ( -2.050006216300763739, 115.7029491482434622, 1.635993916937294568 ) ) ;
#14703=CARTESIAN_POINT ( 'NONE',  ( -1.287880193524239658, 20.15907059199006923, -4.440276399826991849 ) ) ;
#14704=ORIENTED_EDGE ( 'NONE', *, *, #7896, .F. ) ;
#14705=CARTESIAN_POINT ( 'NONE',  ( -4.835487464103170652, 104.6144662015457527, 0.09712566206071873709 ) ) ;
#14706=CARTESIAN_POINT ( 'NONE',  ( 3.179180861052679052, -15.64967171142420099, 4.365151252316144870 ) ) ;
#14707=CARTESIAN_POINT ( 'NONE',  ( -1.263959281924281752, 118.7146927282448132, 0.6429003683496403720 ) ) ;
#14709=CARTESIAN_POINT ( 'NONE',  ( -0.9756124605737610533, 22.95965383878278843, 0.006055453616918176837 ) ) ;
#14710=EDGE_LOOP ( 'NONE', ( #39754, #15436, #39640 ) ) ;
#14712=CARTESIAN_POINT ( 'NONE',  ( -6.707568152035292797E-14, 117.3144662015457271, 2.632902133564923224E-18 ) ) ;
#14713=CARTESIAN_POINT ( 'NONE',  ( 4.134812325681913592, 122.5143120247930142, 0.2378952825278687622 ) ) ;
#14715=CARTESIAN_POINT ( 'NONE',  ( -1.496072496114464911, 120.3785564700922492, 0.3614901595391031286 ) ) ;
#14718=CARTESIAN_POINT ( 'NONE',  ( 4.590055535865089631, 118.0156062071498297, -0.6989146611030767620 ) ) ;
#14719=CARTESIAN_POINT ( 'NONE',  ( 0.9532528233479417024, 157.3234082283764792, -1.521469375400507307 ) ) ;
#14720=CARTESIAN_POINT ( 'NONE',  ( -18.81387422072304361, 135.8679125664981484, -2.390408806419126009 ) ) ;
#14723=CARTESIAN_POINT ( 'NONE',  ( 4.115781193554201245, 118.2429491485453354, -0.1890479318226853389 ) ) ;
#14724=CARTESIAN_POINT ( 'NONE',  ( 9.339416610757361070, 123.9819092696984910, -0.2335442159362872416 ) ) ;
#14727=CARTESIAN_POINT ( 'NONE',  ( 3.205116352530840373, -14.62692654125133451, 3.000134484400556190 ) ) ;
#14728=CARTESIAN_POINT ( 'NONE',  ( 4.942575927434568861, 117.5943726187274194, 0.9708222732221650775 ) ) ;
#14730=CARTESIAN_POINT ( 'NONE',  ( -1.722957355399680202, -2.895624787512894649, -4.295268622497145472 ) ) ;
#14731=CARTESIAN_POINT ( 'NONE',  ( 17.21112184089930963, 146.3482411845097886, 2.056990446313781362 ) ) ;
#14732=CARTESIAN_POINT ( 'NONE',  ( 0.9496290232869858405, 34.46945342146898383, 2.665853779434302684 ) ) ;
#14733=CARTESIAN_POINT ( 'NONE',  ( -3.998592866256331035, 116.4303826247378026, 1.177299868075282641 ) ) ;
#14735=CARTESIAN_POINT ( 'NONE',  ( -4.476207883417873568, -7.053342675672244155, -1.178223045331058705 ) ) ;
#14736=CARTESIAN_POINT ( 'NONE',  ( 5.939593986634037925, 121.5467800236367424, 0.1471147542197156211 ) ) ;
#14737=CARTESIAN_POINT ( 'NONE',  ( 7.154006291674216200, 2.952895779142483246, 4.500751621275830061 ) ) ;
#14739=CARTESIAN_POINT ( 'NONE',  ( -8.771200022011038655, 117.7827218713625115, -0.5098789378553986174 ) ) ;
#14742=LINE ( 'NONE', #5821, #35528 ) ;
#14744=CARTESIAN_POINT ( 'NONE',  ( -5.871471797037544071, 31.01275966357848901, 2.875548327037550589 ) ) ;
#14745=CARTESIAN_POINT ( 'NONE',  ( 6.515560366292186600, -0.8950661730705262720, -5.416678580889517924 ) ) ;
#14746=EDGE_CURVE ( 'NONE', #13325, #10933, #29537, .T. ) ;
#14747=CARTESIAN_POINT ( 'NONE',  ( 1.940878836488825643, 118.1588881878910939, 0.8639920667537415166 ) ) ;
#14751=CARTESIAN_POINT ( 'NONE',  ( -3.811114225546910816, 116.8316721669309572, 0.2429903670874780930 ) ) ;
#14757=CARTESIAN_POINT ( 'NONE',  ( -5.318614220644641399, 121.3518964346359468, -0.06992023047444935469 ) ) ;
#14758=CARTESIAN_POINT ( 'NONE',  ( 3.388119949408427978, -15.58183483456807039, 5.324763925812813881 ) ) ;
#14759=CARTESIAN_POINT ( 'NONE',  ( -0.4390033025491983376, 118.1045761740670201, 0.5613618447453817550 ) ) ;
#14760=CARTESIAN_POINT ( 'NONE',  ( 3.102616959202278757, 159.2904672602661549, -0.8345756338990467649 ) ) ;
#14761=CARTESIAN_POINT ( 'NONE',  ( 2.584458374606236841, 15.83607344512877368, 3.832284875798456447 ) ) ;
#14762=CARTESIAN_POINT ( 'NONE',  ( -9.754222058523323469, 118.0373187826741486, -0.4689489433136687646 ) ) ;
#14764=CARTESIAN_POINT ( 'NONE',  ( -8.796213517692432760, 117.7094638964744320, -0.009884658790045439819 ) ) ;
#14766=CARTESIAN_POINT ( 'NONE',  ( -3.718565865972091267, 156.7231754051992425, 1.451222330515915093 ) ) ;
#14768=CARTESIAN_POINT ( 'NONE',  ( 1.305241956589648034, 119.0230276286704054, -0.6306560096549495009 ) ) ;
#14769=CARTESIAN_POINT ( 'NONE',  ( -13.68454576465616590, 121.6032371815301900, -1.618700059879337072 ) ) ;
#14771=AXIS2_PLACEMENT_3D ( 'NONE', #6931, #36738, #26934 ) ;
#14773=CARTESIAN_POINT ( 'NONE',  ( 0.005430166084257035536, 120.5648899400503069, -0.2717477157510631014 ) ) ;
#14775=CARTESIAN_POINT ( 'NONE',  ( -12.61679319894190598, 153.7453525671159298, -2.178569956567484756 ) ) ;
#14776=CARTESIAN_POINT ( 'NONE',  ( 3.308369008328103433, -15.71782228035249673, 4.479361047165574483 ) ) ;
#14777=CARTESIAN_POINT ( 'NONE',  ( -4.439283198886601944, 118.1598961654773632, -0.6091820576028420531 ) ) ;
#14781=CARTESIAN_POINT ( 'NONE',  ( 11.36144155339839656, 123.3954635094115702, 1.633191427152098418 ) ) ;
#14782=FACE_OUTER_BOUND ( 'NONE', #35086, .T. ) ;
#14783=CARTESIAN_POINT ( 'NONE',  ( 2.068261358883969780, 0.06400946394871305511, -8.190863557276260920 ) ) ;
#14784=CARTESIAN_POINT ( 'NONE',  ( 13.22128265123318691, 134.0707761029912035, 0.8398552229569322680 ) ) ;
#14787=ORIENTED_EDGE ( 'NONE', *, *, #1891, .F. ) ;
#14788=CARTESIAN_POINT ( 'NONE',  ( 3.104280510418153671, 107.6125246504606281, -4.328335581088759376 ) ) ;
#14789=CARTESIAN_POINT ( 'NONE',  ( 1.060420246909465236, 118.7629491485454025, 1.261316868433438376 ) ) ;
#14790=AXIS2_PLACEMENT_3D ( 'NONE', #6050, #38211, #19012 ) ;
#14793=CARTESIAN_POINT ( 'NONE',  ( -22.53108783561251371, 150.7873321363286152, -0.2974592429706744423 ) ) ;
#14796=CARTESIAN_POINT ( 'NONE',  ( -7.846638837763108221, 122.2680111424683957, -0.7500643504151511820 ) ) ;
#14797=CARTESIAN_POINT ( 'NONE',  ( -7.991391493690929160, 121.7106681566311579, 0.7744224044266007079 ) ) ;
#14799=CARTESIAN_POINT ( 'NONE',  ( 2.253168137283801276, 115.6909491485452577, -1.622715864987487544 ) ) ;
#14800=CARTESIAN_POINT ( 'NONE',  ( -1.586003330670630485, 156.2604006213118453, -0.2328413704193781908 ) ) ;
#14801=CARTESIAN_POINT ( 'NONE',  ( 2.771648496353774860, -15.01054376081380148, 5.729243832102374867 ) ) ;
#14802=CARTESIAN_POINT ( 'NONE',  ( -0.008945125900505456612, 117.5133074443058945, 0.4476506782301717946 ) ) ;
#14804=DIRECTION ( 'NONE',  ( -4.017660918040594346E-17, 1.000000000000000000, 2.376309959284834438E-19 ) ) ;
#14805=CARTESIAN_POINT ( 'NONE',  ( 11.68195978820569536, 118.7263634577040676, 0.3785536984881910372 ) ) ;
#14806=CARTESIAN_POINT ( 'NONE',  ( 15.64207015331054862, 147.2204672151589193, 0.3125657877211908686 ) ) ;
#14808=CARTESIAN_POINT ( 'NONE',  ( 0.6634555152105963138, 29.00466287695533296, -0.7151348822165174424 ) ) ;
#14809=CARTESIAN_POINT ( 'NONE',  ( -23.28768492013425018, 149.3500807853454546, -0.5424486132203800715 ) ) ;
#14810=FACE_OUTER_BOUND ( 'NONE', #31197, .T. ) ;
#14814=CARTESIAN_POINT ( 'NONE',  ( 5.927595846997289364, 118.6114240595178018, 1.195360803812330452 ) ) ;
#14816=CARTESIAN_POINT ( 'NONE',  ( 14.57523308444390686, 121.8773232776577942, 1.525373117076484153 ) ) ;
#14818=CARTESIAN_POINT ( 'NONE',  ( 19.90609901365546364, 149.5711785761137662, -1.665592367946398422 ) ) ;
#14819=CARTESIAN_POINT ( 'NONE',  ( 1.173990663012069113, -13.46572784750561880, -4.469126434461346165 ) ) ;
#14820=CARTESIAN_POINT ( 'NONE',  ( -16.15135472115380111, 155.1612327564137388, -1.525667687477715084 ) ) ;
#14821=CARTESIAN_POINT ( 'NONE',  ( 4.947454507184974482, 117.6245515869850919, -0.7568747717558176324 ) ) ;
#14823=CARTESIAN_POINT ( 'NONE',  ( -9.177823364990569388, 124.0935018032023436, -0.02293427522457971990 ) ) ;
#14824=CARTESIAN_POINT ( 'NONE',  ( 0.01147819631900381422, 118.8623374019222894, -0.5744158801423950855 ) ) ;
#14825=CARTESIAN_POINT ( 'NONE',  ( 2.462693652799142541, -15.54209007114785912, 5.820364621994587040 ) ) ;
#14827=CARTESIAN_POINT ( 'NONE',  ( -1.083479109511653826, 117.9496054725919123, -1.389487458230839190 ) ) ;
#14829=CARTESIAN_POINT ( 'NONE',  ( 6.637665810843221159, 119.8184877057495754, 1.268479684707346511 ) ) ;
#14830=CARTESIAN_POINT ( 'NONE',  ( -5.586884702347496123, 98.39146620154573952, -0.1116392523995361624 ) ) ;
#14832=CARTESIAN_POINT ( 'NONE',  ( -2.686747594420624718, 118.0959492836583422, -0.9542362816721940977 ) ) ;
#14833=CARTESIAN_POINT ( 'NONE',  ( -2.504607545376518640, 120.2382744777187611, 0.4047138806074999096 ) ) ;
#14834=CARTESIAN_POINT ( 'NONE',  ( -3.184215270518052421, -12.39116543543024562, -7.798991864805400631 ) ) ;
#14835=CARTESIAN_POINT ( 'NONE',  ( 16.14702439603928141, 146.0959698922748942, 1.294960982472433741 ) ) ;
#14836=CARTESIAN_POINT ( 'NONE',  ( -4.800388046790427410, 115.6909491485453003, -1.474219336065222041 ) ) ;
#14837=CARTESIAN_POINT ( 'NONE',  ( 1.937878880890121058, 116.8467566806161386, -0.3061478142745880371 ) ) ;
#14842=CARTESIAN_POINT ( 'NONE',  ( 2.037655544652285933, -15.20941935993469940, 5.943311982828842766 ) ) ;
#14843=CARTESIAN_POINT ( 'NONE',  ( -4.119060676135726240, 118.2429491485453354, 0.1854733653491233702 ) ) ;
#14844=CARTESIAN_POINT ( 'NONE',  ( 4.686997755226863127, 113.9923204192467523, -1.949621542610482372 ) ) ;
#14845=ORIENTED_EDGE ( 'NONE', *, *, #17814, .F. ) ;
#14847=CARTESIAN_POINT ( 'NONE',  ( -8.226885276541187508, 120.3464503904280321, -1.440290466561924498 ) ) ;
#14848=DIRECTION ( 'NONE',  ( 0.9998004120163608288, 0.000000000000000000, 0.01997839162482749342 ) ) ;
#14849=CARTESIAN_POINT ( 'NONE',  ( 4.223530570022107966, 118.2238270089485184, 0.4905371497760634969 ) ) ;
#14850=CARTESIAN_POINT ( 'NONE',  ( -1.530927031713913866, 120.6610732671444595, -0.3086461854719843578 ) ) ;
#14851=CARTESIAN_POINT ( 'NONE',  ( -4.618747647011250734, 118.0632304573675810, 0.5484251646978447470 ) ) ;
#14854=ORIENTED_EDGE ( 'NONE', *, *, #27682, .F. ) ;
#14855=CARTESIAN_POINT ( 'NONE',  ( -3.562413952978887632, 23.18266144714348798, 2.948169924785601470 ) ) ;
#14856=CARTESIAN_POINT ( 'NONE',  ( -16.54853992722335931, 147.5857818452174115, -1.770514083359864044 ) ) ;
#14860=CARTESIAN_POINT ( 'NONE',  ( -6.066676402028498671, 121.4189492134451029, 0.06607077281897212606 ) ) ;
#14862=CARTESIAN_POINT ( 'NONE',  ( 4.064150447026247726, 23.66704930264554818, -2.198397014704132513 ) ) ;
#14863=CARTESIAN_POINT ( 'NONE',  ( 5.835170694357040055, 117.3723397083485622, 0.6929373658347461884 ) ) ;
#14864=CARTESIAN_POINT ( 'NONE',  ( 1.757780374235184739, 104.6144662015457243, -4.503817898648089901 ) ) ;
#14865=CARTESIAN_POINT ( 'NONE',  ( 3.198896590522081862, -14.38863201745455100, 2.123570546440393780 ) ) ;
#14866=CARTESIAN_POINT ( 'NONE',  ( 20.65103440377610866, 150.0789294893613999, -1.463288793709878632 ) ) ;
#14867=CARTESIAN_POINT ( 'NONE',  ( -14.85905242749878497, 128.5561590274816126, 1.519445497462470485 ) ) ;
#14869=CARTESIAN_POINT ( 'NONE',  ( -3.633452533992191036, 26.69063122243967712, -2.854640957048627747 ) ) ;
#14870=CARTESIAN_POINT ( 'NONE',  ( -18.16683071450857412, 125.1529741258727597, -1.044517495177846422 ) ) ;
#14871=CARTESIAN_POINT ( 'NONE',  ( -0.9510052327539034733, 17.61975311242802533, 0.2078495401503242801 ) ) ;
#14874=CARTESIAN_POINT ( 'NONE',  ( -16.08279055836844051, 146.6973543426590254, 0.5313625374031881732 ) ) ;
#14875=CARTESIAN_POINT ( 'NONE',  ( 5.114911232981273592, -13.88689734646693452, 3.682185042294812582 ) ) ;
#14876=CARTESIAN_POINT ( 'NONE',  ( 14.11650378654203664, 131.1061190467503934, -1.279305142450559707 ) ) ;
#14878=CARTESIAN_POINT ( 'NONE',  ( 1.071098897595643473, 115.7029399971135319, 1.745873157700803757 ) ) ;
#14879=CARTESIAN_POINT ( 'NONE',  ( 3.236250843111535769, -14.18372432684703099, 3.165927027233770286 ) ) ;
#14880=CARTESIAN_POINT ( 'NONE',  ( -4.899907873566092142, 117.6566817052388245, -0.9515826219193989077 ) ) ;
#14881=EDGE_CURVE ( 'NONE', #6467, #24193, #513, .T. ) ;
#14882=CARTESIAN_POINT ( 'NONE',  ( 9.191399985966370423, 124.2403664864748549, 0.1492717680338160047 ) ) ;
#14883=ORIENTED_EDGE ( 'NONE', *, *, #8685, .T. ) ;
#14884=CARTESIAN_POINT ( 'NONE',  ( 20.38365538121562892, 147.8414448467482600, 2.482674703111231285 ) ) ;
#14885=CARTESIAN_POINT ( 'NONE',  ( 0.6412933796112577634, 156.3034662015457741, 0.01281456791805622546 ) ) ;
#14887=CARTESIAN_POINT ( 'NONE',  ( 0.0002734175338603746100, 159.6054662015457382, -0.01368293144939978188 ) ) ;
#14888=CARTESIAN_POINT ( 'NONE',  ( 15.48609530480946894, 120.8153160915142337, -0.009749853210865230824 ) ) ;
#14890=CARTESIAN_POINT ( 'NONE',  ( 0.09221630143774380006, 107.6766875080336376, -4.614880812453306724 ) ) ;
#14891=CARTESIAN_POINT ( 'NONE',  ( 1.759666435841401810, -15.35400245117242513, 5.409080988316447680 ) ) ;
#14894=CARTESIAN_POINT ( 'NONE',  ( -4.704233533693831681, 117.8349189730105309, 0.8529071958809373299 ) ) ;
#14896=ORIENTED_EDGE ( 'NONE', *, *, #9552, .T. ) ;
#14897=CARTESIAN_POINT ( 'NONE',  ( -5.078986093043186045, 94.83546620154572793, -0.1014902294541231709 ) ) ;
#14898=CARTESIAN_POINT ( 'NONE',  ( -5.583873019120129122, 118.2001624726323854, -1.144883371530341254 ) ) ;
#14899=CARTESIAN_POINT ( 'NONE',  ( -4.531575537552095412, 119.7344140837147819, -0.5249638875923485770 ) ) ;
#14900=CARTESIAN_POINT ( 'NONE',  ( 4.943796685340839936, 117.5327713888434431, 0.9784953665843204584 ) ) ;
#14901=CARTESIAN_POINT ( 'NONE',  ( -4.731399709915055318, 117.6315807060625929, -1.144721263631117703 ) ) ;
#14902=CARTESIAN_POINT ( 'NONE',  ( -0.4040709798586945567, 123.7646714092001190, 0.1152108919326052111 ) ) ;
#14906=CARTESIAN_POINT ( 'NONE',  ( 3.514454466653502251, -13.37942318924494067, 2.559657187549406299 ) ) ;
#14907=CARTESIAN_POINT ( 'NONE',  ( 1.225173952871632332, 106.6134986179334589, -4.982835752217485314 ) ) ;
#14909=CARTESIAN_POINT ( 'NONE',  ( -3.890668369019033790, 28.55756886444901710, 1.917437575001415651 ) ) ;
#14910=CARTESIAN_POINT ( 'NONE',  ( -1.199145814505997665, 115.7029469948677018, 1.697500384976515564 ) ) ;
#14911=CARTESIAN_POINT ( 'NONE',  ( -2.406711483539481389, 4.503775517365914638, 3.979180414515509412 ) ) ;
#14912=ORIENTED_EDGE ( 'NONE', *, *, #18525, .F. ) ;
#14913=CARTESIAN_POINT ( 'NONE',  ( 3.957041461616310762, 104.6144662015457811, -2.768236986571138480 ) ) ;
#14914=CARTESIAN_POINT ( 'NONE',  ( 1.897852064921616622, -15.54654116324019597, 5.408738352340563438 ) ) ;
#14915=CARTESIAN_POINT ( 'NONE',  ( -19.86924145434966960, 147.9128418260961837, 1.725515945229960657 ) ) ;
#14916=CARTESIAN_POINT ( 'NONE',  ( -0.6881565663083963891, 18.49284505249605459, 0.6899137464212180548 ) ) ;
#14917=CARTESIAN_POINT ( 'NONE',  ( -0.9731698936423014423, 13.46246454747003618, 0.06867709314994872860 ) ) ;
#14921=DIRECTION ( 'NONE',  ( -4.017660918040594346E-17, 1.000000000000000000, 2.376309959284834438E-19 ) ) ;
#14922=CARTESIAN_POINT ( 'NONE',  ( 2.416298757281802434, 119.8248006784163380, 0.5703471319689770169 ) ) ;
#14925=CARTESIAN_POINT ( 'NONE',  ( -10.06202586252270770, 123.8737202207250618, 0.7052144931501602709 ) ) ;
#14927=FACE_OUTER_BOUND ( 'NONE', #39173, .T. ) ;
#14929=CARTESIAN_POINT ( 'NONE',  ( 3.297440819997984107, -14.19009280176566890, 4.446257544676719853 ) ) ;
#14930=CARTESIAN_POINT ( 'NONE',  ( 18.08730999440950882, 147.8422069945528108, -1.617706263729447702 ) ) ;
#14931=CARTESIAN_POINT ( 'NONE',  ( -19.70389350229454095, 149.1964539096042870, -2.489783701940901484 ) ) ;
#14933=CARTESIAN_POINT ( 'NONE',  ( -6.497774333512897904, 30.00467535414699327, 0.6616146369854277731 ) ) ;
#14934=CARTESIAN_POINT ( 'NONE',  ( 8.172795105213573663, 122.8283871457973362, -0.1257892658093056615 ) ) ;
#14935=ORIENTED_EDGE ( 'NONE', *, *, #40941, .T. ) ;
#14936=CARTESIAN_POINT ( 'NONE',  ( 2.667920334613889555, -13.82128762729334426, -0.01087480101406306660 ) ) ;
#14937=EDGE_CURVE ( 'NONE', #31748, #35799, #19256, .T. ) ;
#14940=CARTESIAN_POINT ( 'NONE',  ( 4.571311019248293306, -6.119132638730012452, 0.7325351754658009362 ) ) ;
#14941=CARTESIAN_POINT ( 'NONE',  ( 16.67506696845903846, 147.9788754379930822, 1.914365833524547478 ) ) ;
#14942=CARTESIAN_POINT ( 'NONE',  ( -1.655660646363030786, 31.15378821692802802, 3.245565323402777480 ) ) ;
#14943=CARTESIAN_POINT ( 'NONE',  ( -3.444826702830499965, 112.1633951907056996, 2.719597167543061467 ) ) ;
#14944=CARTESIAN_POINT ( 'NONE',  ( 4.440276399826426967, -1.430929408009915083, -1.287880193523989636 ) ) ;
#14945=CARTESIAN_POINT ( 'NONE',  ( 15.21351360038791789, 143.4186079242267340, 0.3040022078858843346 ) ) ;
#14946=AXIS2_PLACEMENT_3D ( 'NONE', #32396, #19807, #7056 ) ;
#14947=EDGE_CURVE ( 'NONE', #14129, #27965, #35587, .T. ) ;
#14948=CARTESIAN_POINT ( 'NONE',  ( -8.308456333890557488, -0.7205321100333081930, 1.466575456822119206 ) ) ;
#14950=CARTESIAN_POINT ( 'NONE',  ( -8.775520152584638467, 117.7647785482566576, -0.4778187140148553724 ) ) ;
#14953=CARTESIAN_POINT ( 'NONE',  ( -6.446885413170102552, 29.42808026494702389, 0.2842954123359194840 ) ) ;
#14954=CARTESIAN_POINT ( 'NONE',  ( -8.418590987418564708, -6.603242653765095227, 0.8142584484527041200 ) ) ;
#14958=CARTESIAN_POINT ( 'NONE',  ( 0.8647483397478292755, 121.9014879524050343, -0.2897378433829551625 ) ) ;
#14959=CARTESIAN_POINT ( 'NONE',  ( -7.966904459259942506, 158.6775731370129279, 0.2701962758350455185 ) ) ;
#14960=ORIENTED_EDGE ( 'NONE', *, *, #730, .T. ) ;
#14962=( BOUNDED_SURFACE ( )  B_SPLINE_SURFACE ( 3, 2, ( 
 ( #37758, #21973, #40758 ),
 ( #41176, #9008, #34363 ),
 ( #40964, #41392, #2630 ),
 ( #1993, #5617, #5824 ),
 ( #27956, #24759, #11555 ),
 ( #12197, #18780, #9218 ),
 ( #15165, #11769, #2420 ),
 ( #21545, #37547, #15380 ),
 ( #38407, #2207, #18573 ),
 ( #31581, #28172, #28594 ),
 ( #35206, #8798, #15589 ),
 ( #31791, #12413, #34575 ),
 ( #8370, #5402, #14747 ),
 ( #25405, #18358, #21336 ),
 ( #28386, #25189, #22175 ),
 ( #38192, #37973, #6032 ),
 ( #35005, #18994, #1785 ),
 ( #11980, #31364, #5195 ),
 ( #24974, #24539, #31153 ),
 ( #19829, #12818, #25806 ) ),
 .UNSPECIFIED., .F., .F., .T. ) 
 B_SPLINE_SURFACE_WITH_KNOTS ( ( 4, 2, 2, 2, 2, 2, 2, 2, 2, 4 ),
 ( 3, 3 ),
 ( -3.903127820947815962E-18, 0.0002906707827382450766, 0.0004360061741073695393, 0.0005813415654764940562, 0.0008720123482147429817, 0.001162683130952992016, 0.002325366261905987934, 0.002906707827382486002, 0.003488049392858983636, 0.004650732523811979338 ),
 ( 0.000000000000000000, 0.7006112354927811481 ),
 .UNSPECIFIED. ) 
 GEOMETRIC_REPRESENTATION_ITEM ( )  RATIONAL_B_SPLINE_SURFACE ( (
 ( 1.000000000000000000, 0.8321377275423429420, 0.8994878432830558657),
 ( 1.000000000000000000, 0.8321377275423429420, 0.8994878432830558657),
 ( 1.000000000000000000, 0.8321378623915750561, 0.8994879240277457999),
 ( 1.000000000000000000, 0.8321376435713845332, 0.8994877930031328628),
 ( 1.000000000000000000, 0.8321373692613844852, 0.8994876287524689040),
 ( 1.000000000000000000, 0.8321375004543833942, 0.8994877073078884067),
 ( 1.000000000000000000, 0.8321376855588478172, 0.8994878181442822473),
 ( 1.000000000000000000, 0.8321378848318423671, 0.8994879374644735304),
 ( 1.000000000000000000, 0.8321377198722352819, 0.8994878386903677470),
 ( 1.000000000000000000, 0.8321377383289947360, 0.8994878497418605789),
 ( 1.000000000000000000, 0.8321377253651141004, 0.8994878419793801427),
 ( 1.000000000000000000, 0.8321377372094624914, 0.8994878490715096930),
 ( 1.000000000000000000, 0.8321377976487042138, 0.8994878852611696285),
 ( 1.000000000000000000, 0.8321376953121012443, 0.8994878239843113743),
 ( 1.000000000000000000, 0.8321372635390859029, 0.8994875654483320826),
 ( 1.000000000000000000, 0.8321371748454207129, 0.8994875123405583484),
 ( 1.000000000000000000, 0.8321377042314352934, 0.8994878293250081480),
 ( 1.000000000000000000, 0.8321377726643398587, 0.8994878703010936727),
 ( 1.000000000000000000, 0.8321377275429439058, 0.8994878432834155779),
 ( 1.000000000000000000, 0.8321377275429439058, 0.8994878432834155779) ) ) 
 REPRESENTATION_ITEM ( '' )  SURFACE ( )  );
#14965=CARTESIAN_POINT ( 'NONE',  ( -0.6412933796113865492, 156.3034662015457741, -0.01281456791805603290 ) ) ;
#14966=CARTESIAN_POINT ( 'NONE',  ( 6.104261451579751530, -14.47397795074312299, 1.449478640324443290 ) ) ;
#14967=CARTESIAN_POINT ( 'NONE',  ( -20.99182874412630184, 148.0559997909317644, 1.564581863923973470 ) ) ;
#14968=CARTESIAN_POINT ( 'NONE',  ( 17.77240244235137112, 153.9999837190418930, -1.018827867329159531 ) ) ;
#14969=CARTESIAN_POINT ( 'NONE',  ( -4.544942180623752215, 12.81246518813932589, 0.8472608254572608910 ) ) ;
#14970=CARTESIAN_POINT ( 'NONE',  ( -3.764301891765764463, 116.7207137014398626, -0.2841661138181404977 ) ) ;
#14974=CARTESIAN_POINT ( 'NONE',  ( 5.555698890664002576, 116.7273188082384081, 0.2769282034075690180 ) ) ;
#14976=CARTESIAN_POINT ( 'NONE',  ( -8.163394002857751630, 121.3802920439979118, 0.9196017894915151647 ) ) ;
#14978=CARTESIAN_POINT ( 'NONE',  ( 1.064682733363894407, 157.9544661020348997, -1.608744340525367633 ) ) ;
#14980=CARTESIAN_POINT ( 'NONE',  ( -21.10297322700582257, 148.1333099715771766, -2.360403108977008557 ) ) ;
#14982=CARTESIAN_POINT ( 'NONE',  ( 7.149839403334782517, 121.7184703992695773, -0.4778388566947553984 ) ) ;
#14983=ORIENTED_EDGE ( 'NONE', *, *, #38817, .F. ) ;
#14984=CARTESIAN_POINT ( 'NONE',  ( -13.99859221269053222, 128.5416456306063253, -1.961142612884885450 ) ) ;
#14985=CARTESIAN_POINT ( 'NONE',  ( 4.167245103190982292, -15.48560191675932352, 1.819225864046467356 ) ) ;
#14986=CARTESIAN_POINT ( 'NONE',  ( -4.500643392528203890, 118.1244706977970793, -0.6706124182329965544 ) ) ;
#14988=AXIS2_PLACEMENT_3D ( 'NONE', #23649, #40298, #24079 ) ;
#14990=CARTESIAN_POINT ( 'NONE',  ( -4.865551005416930863, 117.4776490099701505, 0.9870761551034079595 ) ) ;
#14991=CARTESIAN_POINT ( 'NONE',  ( 17.64033768477175101, 147.6919162452172145, 2.236185705752640640 ) ) ;
#14992=CARTESIAN_POINT ( 'NONE',  ( -6.505112547751767921E-14, 75.78546620154573077, -1.207165459009924652E-19 ) ) ;
#14993=TOROIDAL_SURFACE ( 'NONE', #18394, 3.683000000000000718, 0.5080000000000000071 ) ;
#14994=CARTESIAN_POINT ( 'NONE',  ( -1.112825283668275045, 5.041181605477844663, 8.348645504544187190 ) ) ;
#14995=CARTESIAN_POINT ( 'NONE',  ( 0.6635084510828398452, 156.3292479207028407, 0.3574603001491371002 ) ) ;
#14996=CARTESIAN_POINT ( 'NONE',  ( 3.108425975021062992, 118.0774503567615028, -0.8384703576004943759 ) ) ;
#14998=ORIENTED_EDGE ( 'NONE', *, *, #7896, .T. ) ;
#14999=CARTESIAN_POINT ( 'NONE',  ( -4.812631915126818427, 117.9394518360245172, 0.9265897817142734194 ) ) ;
#15004=CARTESIAN_POINT ( 'NONE',  ( -13.40764007945161218, 156.9487217736090940, -0.07645926402191043081 ) ) ;
#15007=CARTESIAN_POINT ( 'NONE',  ( -6.881936038377706844, 121.7539469809695873, -0.5834300994894434655 ) ) ;
#15008=CARTESIAN_POINT ( 'NONE',  ( -8.207314164617301344, 120.6877426416252490, 1.076149196205786085 ) ) ;
#15010=CARTESIAN_POINT ( 'NONE',  ( 0.5120572057462492443, 118.7629491485454025, -1.259108956518884881 ) ) ;
#15011=CARTESIAN_POINT ( 'NONE',  ( 0.004910621514677531059, 156.3161161488371533, -0.2457475809811480449 ) ) ;
#15012=CARTESIAN_POINT ( 'NONE',  ( 5.306636623844629419, -13.66766582561489152, 3.280230747366464694 ) ) ;
#15013=CARTESIAN_POINT ( 'NONE',  ( -17.54374246740532683, 153.9260871938423065, 1.166327135487699618 ) ) ;
#15015=CARTESIAN_POINT ( 'NONE',  ( 3.288660796955097609, 159.4686222989141697, 0.1587487428767535014 ) ) ;
#15016=CARTESIAN_POINT ( 'NONE',  ( 9.081988434275306332, 124.1603627706468842, 0.2262077945552918301 ) ) ;
#15018=CARTESIAN_POINT ( 'NONE',  ( -0.6497956273327881727, 21.66276798020532013, -0.7290388503713802759 ) ) ;
#15019=CARTESIAN_POINT ( 'NONE',  ( -22.53260066761450631, 150.7862151120626777, -0.5269028172337438809 ) ) ;
#15023=CARTESIAN_POINT ( 'NONE',  ( 5.825538371254951997, 118.3804061813496276, 1.156786149343531411 ) ) ;
#15025=CARTESIAN_POINT ( 'NONE',  ( 1.253347288035624674, 159.2526592949493534, 1.130111582746273990 ) ) ;
#15027=CARTESIAN_POINT ( 'NONE',  ( 3.179094171403590963, 118.3302933575512412, -0.7469981754565536702 ) ) ;
#15028=CARTESIAN_POINT ( 'NONE',  ( 8.327223946240280839, 23.24253473731531727, -1.329248712143314748 ) ) ;
#15029=CARTESIAN_POINT ( 'NONE',  ( -14.51227343941619274, 121.4416029531759591, -1.418621967605989909 ) ) ;
#15030=CARTESIAN_POINT ( 'NONE',  ( 4.880012207426760895, 117.7310911472439017, -0.7975209570774519641 ) ) ;
#15032=CARTESIAN_POINT ( 'NONE',  ( 5.366896802164511371, 117.1940586887245388, 0.8977625253398615612 ) ) ;
#15034=CARTESIAN_POINT ( 'NONE',  ( -9.048378227557902775, 123.9859359328134190, -0.09628433740681502373 ) ) ;
#15035=CARTESIAN_POINT ( 'NONE',  ( -5.003445044761956950, 119.2220797256985350, -1.100019038710256192 ) ) ;
#15036=CARTESIAN_POINT ( 'NONE',  ( 4.578653272329702872, -15.42525073102989097, 4.254151796826286969 ) ) ;
#15037=AXIS2_PLACEMENT_3D ( 'NONE', #16566, #32341, #3170 ) ;
#15041=CARTESIAN_POINT ( 'NONE',  ( 12.01154561878600546, 123.1955650103826798, 1.772196977085516378 ) ) ;
#15042=CARTESIAN_POINT ( 'NONE',  ( -5.276425599434919178, 115.6909491485453003, 0.8138454675774937641 ) ) ;
#15043=CARTESIAN_POINT ( 'NONE',  ( -0.1065646865916159425, 105.8844662015457203, 5.332932678536313809 ) ) ;
#15044=CARTESIAN_POINT ( 'NONE',  ( 4.050812540078617019, -7.421221357003889629, 7.384888961799156881 ) ) ;
#15045=CARTESIAN_POINT ( 'NONE',  ( 1.710293758672529751, 156.3676537730497387, 0.7734167093480265320 ) ) ;
#15047=CARTESIAN_POINT ( 'NONE',  ( 15.52007106302753492, 121.3130774642648220, -0.3850180365863630216 ) ) ;
#15050=DIRECTION ( 'NONE',  ( 4.017660918040594346E-17, -1.000000000000000000, -2.376309959284834438E-19 ) ) ;
#15052=B_SPLINE_CURVE_WITH_KNOTS ( 'NONE', 3,
 ( #28954, #12770, #10, #13197, #38356, #5984, #25760, #31953, #28754, #15749, #25969, #41767, #38977, #12568 ),
 .UNSPECIFIED., .F., .F.,
 ( 4, 1, 1, 1, 2, 1, 1, 1, 1, 1, 4 ),
 ( 0.2031000000004874739, 0.2063375000004613602, 0.2095750000004352187, 0.2128125000004091050, 0.2160500000003829635, 0.2667374999999738705, 0.3174249999995648053, 0.3681124999991557400, 0.4187999999987466193, 0.5201749999979283778, 0.6215499999971101364 ),
 .UNSPECIFIED. ) ;
#15054=CARTESIAN_POINT ( 'NONE',  ( -4.172034051875796123, 118.2392512717115665, 0.2176196316604530057 ) ) ;
#15055=CARTESIAN_POINT ( 'NONE',  ( -23.42514220146296111, 142.8382549601284097, -0.4680900899253088721 ) ) ;
#15058=CARTESIAN_POINT ( 'NONE',  ( -4.035982701929945016, 119.1815125624980425, -0.9242715903990733617 ) ) ;
#15059=CARTESIAN_POINT ( 'NONE',  ( -4.333424916720135300, 104.6144662015457243, 3.954443799498177370 ) ) ;
#15060=AXIS2_PLACEMENT_3D ( 'NONE', #27064, #7059, #39218 ) ;
#15061=CARTESIAN_POINT ( 'NONE',  ( 4.301387610206993450, 118.2120950049252315, 0.4959387244165239794 ) ) ;
#15062=CARTESIAN_POINT ( 'NONE',  ( -15.56852431296078976, 143.6313904367523833, -1.174399326838564184 ) ) ;
#15066=CARTESIAN_POINT ( 'NONE',  ( 3.465721614298269415, 18.43485028915299750, -3.064284189100199729 ) ) ;
#15071=CARTESIAN_POINT ( 'NONE',  ( -6.996998182677447886, 121.8717014067360651, 0.1556392694547679423 ) ) ;
#15072=CARTESIAN_POINT ( 'NONE',  ( -4.556403025205056245, 17.84477460162305107, -0.8067276567318153457 ) ) ;
#15073=CARTESIAN_POINT ( 'NONE',  ( 1.957152676258774981, 116.9869758084673208, 0.4489687564533214603 ) ) ;
#15075=CARTESIAN_POINT ( 'NONE',  ( 2.568134854143032442, -15.02010252187911554, 4.714990346623905815 ) ) ;
#15076=CARTESIAN_POINT ( 'NONE',  ( 0.009931510163619200818, 117.7854482299006378, -0.4970133802592049954 ) ) ;
#15077=CARTESIAN_POINT ( 'NONE',  ( -18.32188643113677884, 147.9371514012413229, 1.660510838394361866 ) ) ;
#15078=CARTESIAN_POINT ( 'NONE',  ( 0.6341690014321406110, -14.98600045789189394, -0.7374838701073263003 ) ) ;
#15079=CARTESIAN_POINT ( 'NONE',  ( -18.03394523526743143, 125.1493905788104684, -1.135097528960560265 ) ) ;
#15080=CARTESIAN_POINT ( 'NONE',  ( 0.3717569628964236816, 23.89034148085472964, -0.9007439114964531646 ) ) ;
#15083=CARTESIAN_POINT ( 'NONE',  ( -15.94455450784152895, 146.9815093338748966, 0.4077454470555677002 ) ) ;
#15084=CARTESIAN_POINT ( 'NONE',  ( 3.797208283716756227, -14.50848223276941873, 5.080264250175951624 ) ) ;
#15085=CARTESIAN_POINT ( 'NONE',  ( 3.484775907859185562, 120.0787590019544098, -0.5801956493991065056 ) ) ;
#15087=CARTESIAN_POINT ( 'NONE',  ( 1.824384274485360447, 115.7028213362407456, 1.722094561094771326 ) ) ;
#15090=CARTESIAN_POINT ( 'NONE',  ( -4.720466306959788305, 117.9455647699196561, -0.8231657741585700627 ) ) ;
#15091=CARTESIAN_POINT ( 'NONE',  ( 9.234582554329392678, 124.2544328994657405, 0.09881537413615872067 ) ) ;
#15093=CARTESIAN_POINT ( 'NONE',  ( -0.01133701039344599780, 118.4098733054621277, 0.5673503590873753000 ) ) ;
#15095=DIRECTION ( 'NONE',  ( -4.017660918040594346E-17, 1.000000000000000000, 2.376309959284834438E-19 ) ) ;
#15097=CARTESIAN_POINT ( 'NONE',  ( 15.14699153459420877, 156.1345691653134509, 0.01578391296358650636 ) ) ;
#15098=VECTOR ( 'NONE', #31788, 1000.000000000000000 ) ;
#15099=CARTESIAN_POINT ( 'NONE',  ( 0.1058213901577000071, 105.9761915687834772, -5.295735085524063024 ) ) ;
#15100=CARTESIAN_POINT ( 'NONE',  ( 1.702391130740982028, -15.21670867692809281, 5.525181492016910667 ) ) ;
#15101=CARTESIAN_POINT ( 'NONE',  ( 4.936888680085094627, 117.4097579285739954, 1.082126315060445876 ) ) ;
#15103=CARTESIAN_POINT ( 'NONE',  ( -4.720046991804483838, 117.9726138801407274, 0.6354067178298792307 ) ) ;
#15104=ORIENTED_EDGE ( 'NONE', *, *, #15920, .F. ) ;
#15105=DIRECTION ( 'NONE',  ( -4.017660918040594346E-17, 1.000000000000000000, 2.376309959284834438E-19 ) ) ;
#15106=CARTESIAN_POINT ( 'NONE',  ( -8.541944604652830009, 118.8311428792084712, -1.223721217923770199 ) ) ;
#15107=CARTESIAN_POINT ( 'NONE',  ( -4.699507673534897734, 115.8251506319059843, -1.445723734630263824 ) ) ;
#15108=CARTESIAN_POINT ( 'NONE',  ( 4.876145371826403618, 117.7132259977969539, 0.9242780742304819164 ) ) ;
#15109=CARTESIAN_POINT ( 'NONE',  ( -4.612406548220088887, 117.9315729849519840, -0.9640725417016516863 ) ) ;
#15110=CARTESIAN_POINT ( 'NONE',  ( -0.4234688608140231847, 124.8375573595198063, 0.002553167718424102610 ) ) ;
#15111=CIRCLE ( 'NONE', #13794, 0.5080000000000002292 ) ;
#15112=CARTESIAN_POINT ( 'NONE',  ( -1.251853189678833411, -4.679435864505671283, 4.458631606201990394 ) ) ;
#15115=CARTESIAN_POINT ( 'NONE',  ( 3.292060170515798578, -12.34027101600769427, 0.7492661515550719242 ) ) ;
#15116=CARTESIAN_POINT ( 'NONE',  ( 5.007645675277571762, 117.8491495069952748, -0.5952962186315862159 ) ) ;
#15117=CARTESIAN_POINT ( 'NONE',  ( -17.14723838084594121, 144.2986879860016529, -2.167616513504174502 ) ) ;
#15118=CARTESIAN_POINT ( 'NONE',  ( 5.091522377831856794, 117.1430865926791967, -0.3977369347680486666 ) ) ;
#15119=CARTESIAN_POINT ( 'NONE',  ( -1.811248613112315553, 35.20749351892636980, 3.351885823999401381 ) ) ;
#15120=CARTESIAN_POINT ( 'NONE',  ( -1.218981586993044042, 115.7029483214412693, 1.696095298325300593 ) ) ;
#15121=CARTESIAN_POINT ( 'NONE',  ( -4.151662239014343392, 13.23730288530712862, 2.070234887608822572 ) ) ;
#15122=CARTESIAN_POINT ( 'NONE',  ( 16.90643861817980209, 122.6916909566506320, 0.7822879649369941513 ) ) ;
#15124=CARTESIAN_POINT ( 'NONE',  ( -1.823742538767885613, 105.1241012944524442, -5.023058958505786542 ) ) ;
#15125=CARTESIAN_POINT ( 'NONE',  ( 3.762885361805711870, -15.68952731832974656, 3.843115198823321865 ) ) ;
#15126=CARTESIAN_POINT ( 'NONE',  ( -18.33246729151856869, 150.1405190176936344, 1.740612831648467917 ) ) ;
#15127=CARTESIAN_POINT ( 'NONE',  ( 0.8451309169872193161, 21.29487494764119759, 0.4837088869917456346 ) ) ;
#15128=CARTESIAN_POINT ( 'NONE',  ( -0.9703616065139187841, 22.75662690174698355, -0.1248384507273650884 ) ) ;
#15129=ORIENTED_EDGE ( 'NONE', *, *, #14947, .F. ) ;
#15133=CARTESIAN_POINT ( 'NONE',  ( 3.156357112953781741, 123.6198120039584154, 0.1457842492014824465 ) ) ;
#15135=CARTESIAN_POINT ( 'NONE',  ( -16.75300165896971549, 146.9696287467501179, 1.108775417838743005 ) ) ;
#15136=CARTESIAN_POINT ( 'NONE',  ( -6.654617103318593247E-14, 104.6144662015457243, 1.534725424433578570E-31 ) ) ;
#15137=CARTESIAN_POINT ( 'NONE',  ( 3.514454466653502251, -13.37942318924494067, 2.559657187549406299 ) ) ;
#15138=CARTESIAN_POINT ( 'NONE',  ( 5.507840079722706506, 156.5946142756450570, -1.582329182567087766 ) ) ;
#15139=CARTESIAN_POINT ( 'NONE',  ( -10.11172965818669134, 120.4647147465577461, -1.576227610178517979 ) ) ;
#15141=EDGE_CURVE ( 'NONE', #909, #30579, #4312, .T. ) ;
#15142=CARTESIAN_POINT ( 'NONE',  ( -15.26262975079004569, 148.0175730704188481, -0.3049836654608575892 ) ) ;
#15143=CARTESIAN_POINT ( 'NONE',  ( -6.158966240078259879, 30.49883854570459718, 2.286114001711006871 ) ) ;
#15144=CARTESIAN_POINT ( 'NONE',  ( 3.695597174621954029, 120.9852966486377710, -0.1212977071129681950 ) ) ;
#15146=CARTESIAN_POINT ( 'NONE',  ( 2.671714809844681238, -14.97371442308345380, 4.574436322856921144 ) ) ;
#15147=FACE_OUTER_BOUND ( 'NONE', #41445, .T. ) ;
#15148=CARTESIAN_POINT ( 'NONE',  ( -3.748619050207897985, 28.91994025391836942, 2.520532616727765518 ) ) ;
#15150=EDGE_CURVE ( 'NONE', #20685, #39579, #9726, .T. ) ;
#15151=CARTESIAN_POINT ( 'NONE',  ( 3.793251108634954516, -14.54000584982637001, -2.652246991476435056 ) ) ;
#15152=CARTESIAN_POINT ( 'NONE',  ( 13.40915985073331562, 130.9706359334022920, 1.586196205478585419 ) ) ;
#15153=CARTESIAN_POINT ( 'NONE',  ( -2.549105041318592946, 30.42860202397990221, 3.618266982626868522 ) ) ;
#15154=CARTESIAN_POINT ( 'NONE',  ( -3.079207415998597153, 107.8364052097302306, 4.350788137014373724 ) ) ;
#15156=CARTESIAN_POINT ( 'NONE',  ( -1.825063964020108065, -4.879331645356781877, 4.256838567046823840 ) ) ;
#15157=CARTESIAN_POINT ( 'NONE',  ( 8.981069108608807028, 123.9698733229553937, 0.1794631345465902139 ) ) ;
#15158=CARTESIAN_POINT ( 'NONE',  ( 5.926391002875100789, -6.993723907645660098, 5.986726992520772228 ) ) ;
#15160=CARTESIAN_POINT ( 'NONE',  ( 8.787644062751441609, 117.7645083475051422, -0.1261381370569843452 ) ) ;
#15161=CARTESIAN_POINT ( 'NONE',  ( -0.4140400251256791120, 124.3520329708341023, -0.07144784443200472013 ) ) ;
#15164=CARTESIAN_POINT ( 'NONE',  ( -0.8828713250188725548, -8.991384785216279596, -8.412059017423759499 ) ) ;
#15165=CARTESIAN_POINT ( 'NONE',  ( 0.5456427185285884773, 117.3993834314738933, 1.492634212376517056 ) ) ;
#15167=CARTESIAN_POINT ( 'NONE',  ( -6.639407854763120941E-14, 101.6934662015457320, 3.307182826377456566E-30 ) ) ;
#15169=CARTESIAN_POINT ( 'NONE',  ( 0.7687070661361545820, 118.7604188656930120, -0.8775891873661259002 ) ) ;
#15170=CARTESIAN_POINT ( 'NONE',  ( -22.79600589338280514, 150.0845277111093310, 0.2694608383616130531 ) ) ;
#15175=FACE_OUTER_BOUND ( 'NONE', #29291, .T. ) ;
#15176=AXIS2_PLACEMENT_3D ( 'NONE', #37243, #36835, #4049 ) ;
#15177=CARTESIAN_POINT ( 'NONE',  ( -6.508431974736152092, 121.7798191570849440, -0.09215171978640852857 ) ) ;
#15178=CARTESIAN_POINT ( 'NONE',  ( 5.947420766284201576, -14.61438673846185488, 1.993024607196187459 ) ) ;
#15179=CARTESIAN_POINT ( 'NONE',  ( -14.68166051447203913, 123.3142630313093377, 1.213898157370195463 ) ) ;
#15181=CARTESIAN_POINT ( 'NONE',  ( 22.12005076447803731, 142.1041199125429557, -1.010629163944517517 ) ) ;
#15182=CARTESIAN_POINT ( 'NONE',  ( -3.640175008984333882, 11.51306413504884318, -2.862805987297033727 ) ) ;
#15183=CARTESIAN_POINT ( 'NONE',  ( -13.33768363058614881, 156.9675713949798421, -0.6438986485269783122 ) ) ;
#15187=CARTESIAN_POINT ( 'NONE',  ( 2.184484440002603556, 116.2008805095703963, 0.07056628417267586661 ) ) ;
#15189=CARTESIAN_POINT ( 'NONE',  ( -0.9105297513474850390, 157.1001331247151143, 1.431354397858309868 ) ) ;
#15191=CARTESIAN_POINT ( 'NONE',  ( 13.67124846526806614, 154.1626644387825991, -1.747499485815532161 ) ) ;
#15192=CARTESIAN_POINT ( 'NONE',  ( -13.72122979561089195, 121.8522644830672590, -1.670245716993636442 ) ) ;
#15195=CARTESIAN_POINT ( 'NONE',  ( 9.374368624788175453, 123.5785764018267514, -0.4819391486299055560 ) ) ;
#15196=ORIENTED_EDGE ( 'NONE', *, *, #18535, .F. ) ;
#15197=CARTESIAN_POINT ( 'NONE',  ( -14.87841870982569148, 131.2528086460777388, -2.073644862699850933 ) ) ;
#15198=CARTESIAN_POINT ( 'NONE',  ( 2.152540537132713538, -15.51301927577993034, 5.194954439406326507 ) ) ;
#15199=CARTESIAN_POINT ( 'NONE',  ( -4.264711614227720382, 118.2128497746131330, -0.5330956542091240813 ) ) ;
#15202=CARTESIAN_POINT ( 'NONE',  ( 5.349253755625428042, 156.5090806470891209, 1.752114854137454714 ) ) ;
#15203=DIRECTION ( 'NONE',  ( 4.017660918040594346E-17, -1.000000000000000000, -2.376309959284834438E-19 ) ) ;
#15204=CIRCLE ( 'NONE', #41745, 5.080000000000006288 ) ;
#15205=CARTESIAN_POINT ( 'NONE',  ( -2.857158067608712493, -4.877720491018326499, 7.942258620001617864 ) ) ;
#15206=CARTESIAN_POINT ( 'NONE',  ( 15.67344897587543251, 147.2319784351455780, 0.6427785636300454852 ) ) ;
#15207=CARTESIAN_POINT ( 'NONE',  ( 0.7907840460254358383, 118.1535584534380661, -0.8818625303437642726 ) ) ;
#15211=EDGE_CURVE ( 'NONE', #3899, #22816, #7588, .T. ) ;
#15212=CARTESIAN_POINT ( 'NONE',  ( -0.7495039368703291238, 117.9394521389051249, 1.374537209560392936 ) ) ;
#15214=CARTESIAN_POINT ( 'NONE',  ( -7.825995833725252204, 122.3857360859386461, -0.6413020235143477299 ) ) ;
#15218=CARTESIAN_POINT ( 'NONE',  ( -23.35661798279360113, 142.7586093370927074, -0.2368412396931507957 ) ) ;
#15221=CARTESIAN_POINT ( 'NONE',  ( -7.799325083925558566, 122.5293066583467834, -0.4363886786053240430 ) ) ;
#15225=CARTESIAN_POINT ( 'NONE',  ( 2.969299016715368111, 115.7030432460468177, -1.557441274767545680 ) ) ;
#15226=CARTESIAN_POINT ( 'NONE',  ( -4.562414174745367035, 121.1702857069421100, -0.2029539227048860195 ) ) ;
#15228=CARTESIAN_POINT ( 'NONE',  ( 2.095434763668091005, -15.29852786734210746, 5.959135360315205077 ) ) ;
#15229=CARTESIAN_POINT ( 'NONE',  ( -10.00431039430844038, 157.6892375622926181, 1.152258088200127872 ) ) ;
#15230=CARTESIAN_POINT ( 'NONE',  ( -3.743815577281074614, 31.31851751214970037, -0.6207396561878217867 ) ) ;
#15231=CARTESIAN_POINT ( 'NONE',  ( 1.414297571701309320, 159.6040221172770259, 0.1149235736256736529 ) ) ;
#15233=CARTESIAN_POINT ( 'NONE',  ( 0.6461735126227318160, 120.9973616882760723, 0.04597716564786796106 ) ) ;
#15235=CARTESIAN_POINT ( 'NONE',  ( -0.7403349074254782503, 24.03625360216656404, 0.6378939806667418555 ) ) ;
#15236=CARTESIAN_POINT ( 'NONE',  ( -22.73177750447378642, 137.3553536570635742, -0.5243227317837020340 ) ) ;
#15240=CARTESIAN_POINT ( 'NONE',  ( -6.235261774140225199, 119.1541313481671551, 1.003364376444240813 ) ) ;
#15241=DIRECTION ( 'NONE',  ( 0.9998004120163609398, 4.016384292689130894E-17, 0.01997839162482749689 ) ) ;
#15242=CARTESIAN_POINT ( 'NONE',  ( 21.77023485109854306, 148.7205309135917730, 2.145821470179948953 ) ) ;
#15243=CARTESIAN_POINT ( 'NONE',  ( 13.04666149862676860, 122.0079276396459704, -1.242691380407616286 ) ) ;
#15244=CARTESIAN_POINT ( 'NONE',  ( -4.534963259934312596, 26.26729952004485824, -7.114490783490484027 ) ) ;
#15245=CARTESIAN_POINT ( 'NONE',  ( -14.37796933089572171, 121.0470547900126519, -1.299527359048518793 ) ) ;
#15246=CARTESIAN_POINT ( 'NONE',  ( 4.924141663657016110, 117.6632128302819780, -0.7819755836232500368 ) ) ;
#15247=CARTESIAN_POINT ( 'NONE',  ( 0.6688473404177899262, 105.9455060897651748, 5.311925200740537534 ) ) ;
#15248=CARTESIAN_POINT ( 'NONE',  ( -12.91960671971527042, 133.8340822528099636, -0.1412842392263897739 ) ) ;
#15249=CARTESIAN_POINT ( 'NONE',  ( -5.835242038117813834, 119.5807162246413498, -1.179424802705185238 ) ) ;
#15250=CARTESIAN_POINT ( 'NONE',  ( 6.376069600431401696, -13.97715805579494130, 0.6469259796868158663 ) ) ;
#15254=CARTESIAN_POINT ( 'NONE',  ( 11.93340282868940960, 123.0912118827050108, 1.763528850166467432 ) ) ;
#15256=CARTESIAN_POINT ( 'NONE',  ( -1.527851852856435766, 118.1343055320472928, -0.9288516185665885994 ) ) ;
#15257=CARTESIAN_POINT ( 'NONE',  ( -1.979347617175880147, 122.1523088006674840, 0.1944583918105484699 ) ) ;
#15258=CARTESIAN_POINT ( 'NONE',  ( -6.116428202004375869, -11.74185255526443505, -5.788024375304219760 ) ) ;
#15259=CARTESIAN_POINT ( 'NONE',  ( 15.64597882779391114, 147.9168465093495399, 1.159024332450872663 ) ) ;
#15260=CARTESIAN_POINT ( 'NONE',  ( -4.770965495274668733, 118.5930653697794384, -0.9879445655740133336 ) ) ;
#15261=CARTESIAN_POINT ( 'NONE',  ( 10.59335592519045299, 157.9214973357695158, -0.4646299181629826580 ) ) ;
#15265=DIRECTION ( 'NONE',  ( 4.017660918040594346E-17, -1.000000000000000000, -2.376309959284834438E-19 ) ) ;
#15266=CARTESIAN_POINT ( 'NONE',  ( -4.293957123808202603, 118.2142473212576164, 0.3502411785888445150 ) ) ;
#15267=CARTESIAN_POINT ( 'NONE',  ( -20.51686376604223128, 129.1072961674477710, -0.4099757654675939000 ) ) ;
#15268=VERTEX_POINT ( 'NONE', #40184 ) ;
#15270=EDGE_CURVE ( 'NONE', #14618, #35734, #21807, .T. ) ;
#15271=CARTESIAN_POINT ( 'NONE',  ( -6.278307647342964870, 119.9169151369681430, -1.219481925155367907 ) ) ;
#15273=CARTESIAN_POINT ( 'NONE',  ( -5.218277051435869396, 121.1607713875043117, -0.4468594773273020793 ) ) ;
#15274=CARTESIAN_POINT ( 'NONE',  ( 4.999199951152328403, 117.4030387777868469, -0.8341129481215795449 ) ) ;
#15277=ORIENTED_EDGE ( 'NONE', *, *, #4825, .F. ) ;
#15278=CARTESIAN_POINT ( 'NONE',  ( -3.854280124997887746, 21.23357344512866973, -2.551540157904111261 ) ) ;
#15283=CARTESIAN_POINT ( 'NONE',  ( 7.790228995712999094, 122.5851452327640772, 0.3185712494481027224 ) ) ;
#15284=CARTESIAN_POINT ( 'NONE',  ( 2.264360804680111805, 21.29314879275315064, 4.027482774281332389 ) ) ;
#15285=CARTESIAN_POINT ( 'NONE',  ( 15.38653228232027992, 121.5363848317736739, 1.155577132538254670 ) ) ;
#15286=CARTESIAN_POINT ( 'NONE',  ( 2.051927835239828024, 104.6144662015457243, -4.377228190977056954 ) ) ;
#15287=CARTESIAN_POINT ( 'NONE',  ( 3.092642723064080279, -14.67800799544728285, 3.675123631970977911 ) ) ;
#15288=CARTESIAN_POINT ( 'NONE',  ( 2.147481372520596121, 117.7847241295267651, -0.6070331404035437250 ) ) ;
#15289=CARTESIAN_POINT ( 'NONE',  ( -12.44264023681993869, 124.1810962131942517, 1.301390444852660755 ) ) ;
#15290=CARTESIAN_POINT ( 'NONE',  ( 4.610398055573782905, 23.01736123548795021, -0.3254830233858732602 ) ) ;
#15291=CARTESIAN_POINT ( 'NONE',  ( -15.18175346423898198, 121.1469641333237917, -1.070035192906481081 ) ) ;
#15292=CARTESIAN_POINT ( 'NONE',  ( -0.9660709935815289251, 7.903159174923253261, 0.1333004412508401459 ) ) ;
#15295=CARTESIAN_POINT ( 'NONE',  ( -15.92043486079658088, 145.9828583539951126, 0.2780828054990249765 ) ) ;
#15296=CARTESIAN_POINT ( 'NONE',  ( 4.383797612528895549, -14.46967269938057044, 4.720428574551663203 ) ) ;
#15297=CARTESIAN_POINT ( 'NONE',  ( 3.430652046320601389, 156.3978305292817481, -1.152991164011112346 ) ) ;
#15299=CARTESIAN_POINT ( 'NONE',  ( 1.786958751275772306, 115.7029469026952029, 1.723307358492499830 ) ) ;
#15301=CARTESIAN_POINT ( 'NONE',  ( -4.815518961581000568, 117.8246686530165448, -0.8829384762845114976 ) ) ;
#15302=CARTESIAN_POINT ( 'NONE',  ( 5.945776936743700780, 121.5465042053001667, 0.1188107733588234516 ) ) ;
#15305=CARTESIAN_POINT ( 'NONE',  ( 19.26131898708108992, 149.3473233412102275, 2.496341295301664598 ) ) ;
#15306=CARTESIAN_POINT ( 'NONE',  ( -3.174366308152012817, 84.67546620154573134, -0.06343139340882732180 ) ) ;
#15309=CARTESIAN_POINT ( 'NONE',  ( 4.949796331672161820, 117.4773373787071193, -0.8984534372031296456 ) ) ;
#15310=CARTESIAN_POINT ( 'NONE',  ( 22.63314285866076858, 150.6357905964555925, 0.1239933314926730257 ) ) ;
#15313=CARTESIAN_POINT ( 'NONE',  ( 1.957116903647192263, -15.34957576579747140, 5.354569344195124536 ) ) ;
#15316=CARTESIAN_POINT ( 'NONE',  ( -4.678029067978729749, 117.8847919582286465, 0.8180832583663835145 ) ) ;
#15319=CARTESIAN_POINT ( 'NONE',  ( 4.850929972935443146, 117.7610086971114356, 0.9074237114610381738 ) ) ;
#15320=CARTESIAN_POINT ( 'NONE',  ( 5.722844102788878118, 118.5195176813615063, -0.9755545356960315662 ) ) ;
#15321=CARTESIAN_POINT ( 'NONE',  ( -1.025137579952785094, 106.6134986179334589, -5.027802332087124348 ) ) ;
#15322=CARTESIAN_POINT ( 'NONE',  ( 4.899053217361366563, 117.6324216922197365, 0.9917945611932356131 ) ) ;
#15324=CARTESIAN_POINT ( 'NONE',  ( -0.7690845662406576855, 119.7070660435176279, 0.6575911349602957534 ) ) ;
#15325=CARTESIAN_POINT ( 'NONE',  ( -1.504723661876595786, -8.552649586842417051, -4.374500482163298898 ) ) ;
#15328=CARTESIAN_POINT ( 'NONE',  ( 3.604966970014626959, -13.82400766246429136, 3.906450875976586801 ) ) ;
#15329=CARTESIAN_POINT ( 'NONE',  ( 7.618479139564604985, 124.9344662015457317, 0.1522353441811855612 ) ) ;
#15330=CARTESIAN_POINT ( 'NONE',  ( -8.888678185457033365, 122.0520977060996586, -1.259005013942402718 ) ) ;
#15332=CARTESIAN_POINT ( 'NONE',  ( 5.152689472752729039, 116.8412042436348912, 0.1029629964107459106 ) ) ;
#15333=CARTESIAN_POINT ( 'NONE',  ( -0.02244247360070318262, 39.09286639261657115, 1.286999615499952787 ) ) ;
#15335=CARTESIAN_POINT ( 'NONE',  ( -1.627051029834679419, 115.7027888630229171, 1.667098993452897693 ) ) ;
#15336=CARTESIAN_POINT ( 'NONE',  ( 1.068493265602401987, 5.690783753869971484, 4.496582723949734017 ) ) ;
#15337=CARTESIAN_POINT ( 'NONE',  ( 15.81407516854438100, 121.2341309109925334, 0.7422539548746110993 ) ) ;
#15339=CARTESIAN_POINT ( 'NONE',  ( 0.2402493194813784261, 105.1224165606177365, -5.340051935206860279 ) ) ;
#15340=CARTESIAN_POINT ( 'NONE',  ( 4.100156219318407125, -15.52122063102406813, 2.251114749721512709 ) ) ;
#15341=CARTESIAN_POINT ( 'NONE',  ( -12.31762543427507417, 122.6846661264431191, 1.317417697584883030 ) ) ;
#15342=CARTESIAN_POINT ( 'NONE',  ( 0.7093541224826089842, 23.24201423063343697, -0.6674325600367136957 ) ) ;
#15343=CARTESIAN_POINT ( 'NONE',  ( -0.7472855871240335901, 21.88424109716052612, -0.6269268744489370215 ) ) ;
#15344=ORIENTED_EDGE ( 'NONE', *, *, #25847, .T. ) ;
#15347=CARTESIAN_POINT ( 'NONE',  ( 1.486515533885975016, 107.1743931308027129, 4.786382923486936392 ) ) ;
#15349=CARTESIAN_POINT ( 'NONE',  ( -1.514956540612282021, 120.4980338609919386, 0.3173598453907558459 ) ) ;
#15350=CARTESIAN_POINT ( 'NONE',  ( 5.586884702347365561, 68.92746620154572668, 0.1116392523995368286 ) ) ;
#15351=CARTESIAN_POINT ( 'NONE',  ( 3.497624268394256219, -13.57517324819364291, 2.900746184505403669 ) ) ;
#15352=CARTESIAN_POINT ( 'NONE',  ( 18.00357552251023563, 146.8415343102147972, -1.578964580512862925 ) ) ;
#15353=CARTESIAN_POINT ( 'NONE',  ( -1.082660538731543776, 158.4310823543925721, -1.603207764552046832 ) ) ;
#15354=CARTESIAN_POINT ( 'NONE',  ( -5.586884702347496123, 79.34146620154574236, -0.1116392523995361624 ) ) ;
#15355=CARTESIAN_POINT ( 'NONE',  ( 3.047145566129288330, -14.72663143740328806, 3.823360744794035870 ) ) ;
#15356=CARTESIAN_POINT ( 'NONE',  ( -0.01632536679074420016, 38.84944212800221663, 1.323018725044088573 ) ) ;
#15357=CARTESIAN_POINT ( 'NONE',  ( 7.620757776630359359, 122.3831840716419066, -0.1218999176909028453 ) ) ;
#15359=CARTESIAN_POINT ( 'NONE',  ( -0.4436142255061583661, 106.0194232803738998, -5.281734587570124262 ) ) ;
#15364=CARTESIAN_POINT ( 'NONE',  ( -3.436282163690115077, 26.04026231355703658, -7.687665148811276161 ) ) ;
#15365=CARTESIAN_POINT ( 'NONE',  ( -0.02156534543299366835, 156.6359106937186709, 1.079218069903262744 ) ) ;
#15367=CARTESIAN_POINT ( 'NONE',  ( 15.52360445758504426, 120.7153972339879715, 0.2596658046059213687 ) ) ;
#15369=CARTESIAN_POINT ( 'NONE',  ( -1.571019246621560450, 106.2535611835979239, 5.108158685570669988 ) ) ;
#15370=CARTESIAN_POINT ( 'NONE',  ( -3.609430071560130848, 3.966570591990036032, 2.889066364458971137 ) ) ;
#15371=CARTESIAN_POINT ( 'NONE',  ( 15.77133435453283461, 146.5691041611200660, 0.3151487940933137555 ) ) ;
#15373=CARTESIAN_POINT ( 'NONE',  ( 3.135079784281773918, -3.970030566872769562, -7.817010796087090263 ) ) ;
#15375=CARTESIAN_POINT ( 'NONE',  ( -2.148722934776839288, 116.3868840314291475, -0.3193016367261526933 ) ) ;
#15376=CARTESIAN_POINT ( 'NONE',  ( -0.8285762425324525449, 121.5536190086353372, -0.3701497059917958632 ) ) ;
#15379=CARTESIAN_POINT ( 'NONE',  ( -0.3239230800893593276, 29.42979164457532804, -4.628216972995994993 ) ) ;
#15380=CARTESIAN_POINT ( 'NONE',  ( 0.6796407112084186242, 118.1588882304778423, 0.9027520341413136640 ) ) ;
#15383=EDGE_CURVE ( 'NONE', #17144, #17052, #9097, .T. ) ;
#15384=CARTESIAN_POINT ( 'NONE',  ( 0.3799753109754416269, 121.9236798544226730, -0.3295597595137199631 ) ) ;
#15385=CARTESIAN_POINT ( 'NONE',  ( -13.24393851483428719, 156.9672759736256467, 0.3459722171078645769 ) ) ;
#15390=CARTESIAN_POINT ( 'NONE',  ( -14.13522066970473112, 138.8284419781823829, -0.1497975941480006734 ) ) ;
#15391=CARTESIAN_POINT ( 'NONE',  ( 4.849545180983690251, -15.35966036743073637, 3.882997576023691444 ) ) ;
#15392=CARTESIAN_POINT ( 'NONE',  ( -20.72967856921748009, 148.2641884961211076, 1.615940018417327817 ) ) ;
#15393=CARTESIAN_POINT ( 'NONE',  ( 21.94752568715507834, 149.4141677464492091, -1.146579238551070468 ) ) ;
#15394=CARTESIAN_POINT ( 'NONE',  ( -3.130497002865707312, 23.39511390029671745, 3.426874451367011520 ) ) ;
#15396=CARTESIAN_POINT ( 'NONE',  ( -15.30459713313471681, 120.6995131204970875, -0.6235550965980859450 ) ) ;
#15401=CARTESIAN_POINT ( 'NONE',  ( 0.3665064675491350177, 121.9236798544226730, 0.3444762419765421968 ) ) ;
#15402=CARTESIAN_POINT ( 'NONE',  ( -5.134369219808014861, 120.3680889145531552, 0.6721547394862481539 ) ) ;
#15404=CARTESIAN_POINT ( 'NONE',  ( 11.73216920131852881, 154.7938929448963279, -1.733846838993656325 ) ) ;
#15405=CARTESIAN_POINT ( 'NONE',  ( -17.48279436891391114, 128.5781302034472162, -2.030760391889158800 ) ) ;
#15407=CARTESIAN_POINT ( 'NONE',  ( 12.35517153206324181, 152.0262389575480881, -0.8038591168380518903 ) ) ;
#15409=CARTESIAN_POINT ( 'NONE',  ( -0.8698789912703093208, 157.1975648536147787, -1.511617766987151334 ) ) ;
#15410=CARTESIAN_POINT ( 'NONE',  ( 4.433333709997448580, -15.52846643035468688, 1.874498299855786421 ) ) ;
#15411=CARTESIAN_POINT ( 'NONE',  ( -4.105428725848253357, 118.2429491485453070, -0.3529517962327167191 ) ) ;
#15414=CARTESIAN_POINT ( 'NONE',  ( -4.996941175475388519, 117.4672098027941303, 0.7805663078437622415 ) ) ;
#15415=CARTESIAN_POINT ( 'NONE',  ( -0.02874415600673332558, 157.0795416643300939, 1.438475106415294302 ) ) ;
#15419=CARTESIAN_POINT ( 'NONE',  ( -8.268995186617910775, -7.056286353048313309, -1.660136952399225319 ) ) ;
#15420=CARTESIAN_POINT ( 'NONE',  ( 10.39558336183860021, 126.0814211662656419, 0.4651924986760612724 ) ) ;
#15421=CARTESIAN_POINT ( 'NONE',  ( 1.563499521607991438, 118.1343052102891988, -0.8670908977950454455 ) ) ;
#15422=AXIS2_PLACEMENT_3D ( 'NONE', #1318, #10464, #30264 ) ;
#15425=CARTESIAN_POINT ( 'NONE',  ( -0.02812206017517816792, 117.9394518360233519, 1.407342955188501943 ) ) ;
#15431=CARTESIAN_POINT ( 'NONE',  ( -5.733252156539744071, 159.1225378944267845, 0.03759195597257692506 ) ) ;
#15434=CARTESIAN_POINT ( 'NONE',  ( -6.919813487662133333, 121.8949882256362827, -0.3984175079523645246 ) ) ;
#15435=CARTESIAN_POINT ( 'NONE',  ( -7.966529119767051803, 121.8269078720122565, 0.7202784793016417941 ) ) ;
#15436=ORIENTED_EDGE ( 'NONE', *, *, #37538, .T. ) ;
#15437=CARTESIAN_POINT ( 'NONE',  ( 1.232143138580572783, 115.7029489553663808, -1.695162972283317249 ) ) ;
#15438=CARTESIAN_POINT ( 'NONE',  ( -10.25892126925259085, 126.0184183664171655, -0.2980827979995013255 ) ) ;
#15439=CARTESIAN_POINT ( 'NONE',  ( 2.450443274655972559, -15.26395620497007855, 5.889056594049635329 ) ) ;
#15440=CARTESIAN_POINT ( 'NONE',  ( -5.066682439019665196, 158.5910778905036977, 1.349075717862105783 ) ) ;
#15441=DIRECTION ( 'NONE',  ( -0.1548639604663282210, -0.9876883405951374373, 0.02211098372092801939 ) ) ;
#15442=CARTESIAN_POINT ( 'NONE',  ( 0.9122582399080617632, 116.5216256635990391, 0.1489946802529018843 ) ) ;
#15444=CARTESIAN_POINT ( 'NONE',  ( 7.042656930656880476, 122.0730845385896544, 0.2183737125472967333 ) ) ;
#15446=CARTESIAN_POINT ( 'NONE',  ( -0.9542339719106045504, 13.68595756868040603, 0.2091889690632084686 ) ) ;
#15447=CARTESIAN_POINT ( 'NONE',  ( -3.725034515352510844, 116.6403000632267464, -0.1520601685204151510 ) ) ;
#15449=EDGE_CURVE ( 'NONE', #20737, #37727, #6378, .T. ) ;
#15452=CARTESIAN_POINT ( 'NONE',  ( -3.743659292024924756, 118.0176333062828320, 0.7744886050550696677 ) ) ;
#15454=CARTESIAN_POINT ( 'NONE',  ( 17.05973152613361066, 125.2153959547233910, 1.608365543201426773 ) ) ;
#15455=AXIS2_PLACEMENT_3D ( 'NONE', #7583, #26540, #26958 ) ;
#15456=CARTESIAN_POINT ( 'NONE',  ( 11.48785675552145591, 156.2473422840488979, -1.634126210350451469 ) ) ;
#15457=CARTESIAN_POINT ( 'NONE',  ( 3.518211725887771202, 24.73955407011506935, -7.658871095584262711 ) ) ;
#15458=CARTESIAN_POINT ( 'NONE',  ( -3.017629403179087788, 159.2229145144301867, -1.079859862993577391 ) ) ;
#15459=CARTESIAN_POINT ( 'NONE',  ( 4.781198548879745047, 117.7628531851493534, -0.8766415564179582676 ) ) ;
#15460=CARTESIAN_POINT ( 'NONE',  ( 5.928176885185626688, 118.9717589635377664, 0.5867527899620113008 ) ) ;
#15461=AXIS2_PLACEMENT_3D ( 'NONE', #12357, #25344, #19560 ) ;
#15462=CARTESIAN_POINT ( 'NONE',  ( -8.074187567049014191, 122.8559727437779827, -0.08249527776860599015 ) ) ;
#15463=CARTESIAN_POINT ( 'NONE',  ( -11.78639615006497365, 122.5845257805695923, -1.760937685738447334 ) ) ;
#15464=CARTESIAN_POINT ( 'NONE',  ( 6.422280156622033331, -13.89829431882434818, 0.3667318345078443564 ) ) ;
#15468=CARTESIAN_POINT ( 'NONE',  ( 16.55752258724309911, 151.1890201267100906, 2.396410905537823766 ) ) ;
#15469=DIRECTION ( 'NONE',  ( 0.9998004120163608288, 0.000000000000000000, 0.01997839162482749342 ) ) ;
#15473=CARTESIAN_POINT ( 'NONE',  ( -2.656358736808195342, 121.0686911241271702, 0.2846299364715212388 ) ) ;
#15475=CARTESIAN_POINT ( 'NONE',  ( 8.404578209848946102, -5.696077331678487177, -0.5057995593162113446 ) ) ;
#15476=CARTESIAN_POINT ( 'NONE',  ( 7.089475284343898842, 121.8675249661327626, 0.6210822171188468133 ) ) ;
#15478=CARTESIAN_POINT ( 'NONE',  ( 22.97084167624219475, 148.6798292920915117, -0.5140709287734970268 ) ) ;
#15479=CARTESIAN_POINT ( 'NONE',  ( 5.332935397695205637, 105.1224662015457199, 0.1065647409268305201 ) ) ;
#15484=DIRECTION ( 'NONE',  ( -5.206863593109713661E-17, 1.000000000000000000, -1.077750396879097183E-30 ) ) ;
#15487=CARTESIAN_POINT ( 'NONE',  ( -6.576985208878872946, 120.6005770300147049, -1.107357257247939764 ) ) ;
#15488=CARTESIAN_POINT ( 'NONE',  ( -6.442348895218290093E-14, 63.84746620154572838, 4.408874939877717575E-29 ) ) ;
#15489=CARTESIAN_POINT ( 'NONE',  ( -5.204851039068017826, 121.0999079655412203, -0.5006067476712319220 ) ) ;
#15491=CARTESIAN_POINT ( 'NONE',  ( 23.34271727006406394, 149.0672090665632936, 0.4921983935722531456 ) ) ;
#15492=EDGE_LOOP ( 'NONE', ( #8335, #17738 ) ) ;
#15493=CARTESIAN_POINT ( 'NONE',  ( 2.739727753987758252, 28.35525327666260864, -3.728201022356329553 ) ) ;
#15498=CARTESIAN_POINT ( 'NONE',  ( -7.795039456000409039, 122.5917715370820815, -0.009836026403675746793 ) ) ;
#15500=CARTESIAN_POINT ( 'NONE',  ( 8.098994982418634692, 117.9016134627522945, 0.8176261169560979924 ) ) ;
#15502=CARTESIAN_POINT ( 'NONE',  ( 4.002739386954954348, 110.9560952025013023, 3.257662289751307672 ) ) ;
#15503=CARTESIAN_POINT ( 'NONE',  ( 21.28061085028114618, 148.8133262010608462, -1.460188425234497878 ) ) ;
#15504=CARTESIAN_POINT ( 'NONE',  ( -5.091199858996015237, 119.8577235299091228, 0.8121313320900891419 ) ) ;
#15505=CARTESIAN_POINT ( 'NONE',  ( -0.001188813386588473625, -13.89074316258246000, -0.9734844304884215926 ) ) ;
#15506=CARTESIAN_POINT ( 'NONE',  ( -13.07250590169516613, 156.9444350391594014, -1.084824903291609521 ) ) ;
#15507=CARTESIAN_POINT ( 'NONE',  ( -0.3451692354163579113, -3.745485276186693469, -0.9107729336563508138 ) ) ;
#15510=CARTESIAN_POINT ( 'NONE',  ( -1.566048506583701316, 120.7946061759640486, 0.1772761409975700808 ) ) ;
#15511=CARTESIAN_POINT ( 'NONE',  ( 3.942998349758990440, -14.41637075870405482, 4.944918514907367779 ) ) ;
#15512=CARTESIAN_POINT ( 'NONE',  ( 11.50974670170843162, 153.2879862121713757, -1.252373795633383580 ) ) ;
#15514=CARTESIAN_POINT ( 'NONE',  ( 0.8281752705314345819, 115.7028553439171930, 1.753372524936649413 ) ) ;
#15515=AXIS2_PLACEMENT_3D ( 'NONE', #7630, #13798, #17406 ) ;
#15516=CARTESIAN_POINT ( 'NONE',  ( -4.734773379377719138, 117.6653775457820501, -1.128990523777680277 ) ) ;
#15517=CARTESIAN_POINT ( 'NONE',  ( 15.76486438913719468, 145.9085485750152316, 0.2635089261703657537 ) ) ;
#15519=CARTESIAN_POINT ( 'NONE',  ( 2.522816026436708992, 158.1729697732556588, 1.709197703933636348 ) ) ;
#15520=DIRECTION ( 'NONE',  ( -4.017660918040594346E-17, 1.000000000000000000, 2.376309959284834438E-19 ) ) ;
#15521=FACE_BOUND ( 'NONE', #2475, .T. ) ;
#15523=CARTESIAN_POINT ( 'NONE',  ( 4.900892916173488878, 117.4105777512120596, -0.9669312268769758578 ) ) ;
#15524=CARTESIAN_POINT ( 'NONE',  ( 23.14523085694525051, 149.5941399179437781, 0.009123583346248015716 ) ) ;
#15528=CARTESIAN_POINT ( 'NONE',  ( 1.797270874020278297, -15.24711907797275678, 5.420427335509073963 ) ) ;
#15531=CARTESIAN_POINT ( 'NONE',  ( -4.558937555069585201, 118.0891754523873942, 0.5799898687118973939 ) ) ;
#15534=CARTESIAN_POINT ( 'NONE',  ( 5.250303803498147737, 115.7029491485453150, -0.9234757868886493970 ) ) ;
#15536=CARTESIAN_POINT ( 'NONE',  ( 8.440428959602655823, 119.5498230060619278, -1.071212130833359977 ) ) ;
#15537=CARTESIAN_POINT ( 'NONE',  ( -1.237704251691503332, 106.3840144300045409, -5.116357776886615305 ) ) ;
#15538=CARTESIAN_POINT ( 'NONE',  ( 4.733981652075166302, 117.7614939300864023, 1.072079134280608192 ) ) ;
#15539=AXIS2_PLACEMENT_3D ( 'NONE', #8856, #15649, #40610 ) ;
#15540=CYLINDRICAL_SURFACE ( 'NONE', #15461, 5.334000000000001407 ) ;
#15541=CARTESIAN_POINT ( 'NONE',  ( -0.3780739950605601085, 121.2597428844643161, 0.4280417039577733007 ) ) ;
#15542=CARTESIAN_POINT ( 'NONE',  ( 4.114294302962228755, -10.72644468530807416, -2.136776772127288559 ) ) ;
#15544=CARTESIAN_POINT ( 'NONE',  ( 6.932344361571690428, 124.3275308867733600, 0.1272746869527294211 ) ) ;
#15545=CARTESIAN_POINT ( 'NONE',  ( -17.47633463031934298, 147.2926247242496345, -2.162249527696345375 ) ) ;
#15546=DIRECTION ( 'NONE',  ( -0.9998004120163608288, 0.000000000000000000, -0.01997839162482750383 ) ) ;
#15547=CARTESIAN_POINT ( 'NONE',  ( -5.892701309309134494, 29.15168417748227014, 1.983235083422884015 ) ) ;
#15549=CARTESIAN_POINT ( 'NONE',  ( -3.998286381996895233, 3.741657206818807424, 2.332027183294827832 ) ) ;
#15550=CARTESIAN_POINT ( 'NONE',  ( 15.11126220171598256, 120.7387302883610118, 0.8143899245520164198 ) ) ;
#15552=CARTESIAN_POINT ( 'NONE',  ( 2.873716936905370556, 105.1244232856616350, -4.504777322494160963 ) ) ;
#15553=CARTESIAN_POINT ( 'NONE',  ( 3.662106647173574370, -15.69883703644059381, 4.006612474821164227 ) ) ;
#15554=CARTESIAN_POINT ( 'NONE',  ( -9.920314382279082466, 120.7895603300898699, 1.200622369358214980 ) ) ;
#15555=CARTESIAN_POINT ( 'NONE',  ( 0.1924800537393606958, 19.99376482044840486, 0.9543378882872525226 ) ) ;
#15556=CARTESIAN_POINT ( 'NONE',  ( 0.9479787518424646064, 8.937585264489511516, -0.2400550011337005962 ) ) ;
#15558=ORIENTED_EDGE ( 'NONE', *, *, #41743, .T. ) ;
#15560=CARTESIAN_POINT ( 'NONE',  ( -0.1065646865916381331, 105.8844662015456777, 5.332932678536312032 ) ) ;
#15561=CARTESIAN_POINT ( 'NONE',  ( -7.796255004792742582, 122.1031240515655298, 0.5053261734565678287 ) ) ;
#15562=CARTESIAN_POINT ( 'NONE',  ( -14.16569067496504353, 138.8670163227227476, -0.2830642121559618363 ) ) ;
#15563=CARTESIAN_POINT ( 'NONE',  ( 2.715028358135622266, -14.64271907847003362, 5.065740987199049528 ) ) ;
#15564=CARTESIAN_POINT ( 'NONE',  ( 4.309327875668891750, 119.9149831030956932, -0.7077533764146594075 ) ) ;
#15565=CARTESIAN_POINT ( 'NONE',  ( -18.46656456646938693, 135.7714211226372640, -2.417028963773544259 ) ) ;
#15567=CARTESIAN_POINT ( 'NONE',  ( 7.974932797479802993, 121.6047494564416951, 1.136202016109667978 ) ) ;
#15568=CARTESIAN_POINT ( 'NONE',  ( -0.2616981356411257065, 38.12352966651759090, 1.602708108658221109 ) ) ;
#15569=CARTESIAN_POINT ( 'NONE',  ( 15.83367336760669097, 146.2622375132148989, -0.01472612784998089501 ) ) ;
#15571=CARTESIAN_POINT ( 'NONE',  ( 5.010184479710102501, 117.3993854065330851, 0.7504461923096029663 ) ) ;
#15576=CARTESIAN_POINT ( 'NONE',  ( -7.510622214715407807, 18.91685342841953954, 3.806420843228597306 ) ) ;
#15577=CARTESIAN_POINT ( 'NONE',  ( 10.10772093100550961, 154.1059161911440469, 1.650231108813019265 ) ) ;
#15579=CARTESIAN_POINT ( 'NONE',  ( 23.44551923343641064, 146.8400249081559537, 0.3912800906488115293 ) ) ;
#15580=CARTESIAN_POINT ( 'NONE',  ( -3.568456891169586420, 108.6786390861269922, 3.983803253449686110 ) ) ;
#15582=CARTESIAN_POINT ( 'NONE',  ( 2.884051542275651414, 156.0957788938021054, 0.05763021347587640730 ) ) ;
#15583=CARTESIAN_POINT ( 'NONE',  ( 5.670988759832523485, -4.508684804710943794, -6.293633234193930726 ) ) ;
#15584=CARTESIAN_POINT ( 'NONE',  ( -5.512364842945291166, 116.9397240910284239, -0.6180008233057252554 ) ) ;
#15585=CARTESIAN_POINT ( 'NONE',  ( 0.07157677170298341884, 110.3683645023726569, -3.581994345755902032 ) ) ;
#15588=CARTESIAN_POINT ( 'NONE',  ( -1.796629210684171918, -4.683219827815034542, 8.244768259809569955 ) ) ;
#15589=CARTESIAN_POINT ( 'NONE',  ( 1.067977723796545320, 118.1588881525931640, 0.8905038927680214433 ) ) ;
#15591=CARTESIAN_POINT ( 'NONE',  ( 1.831848720338793202, -15.17974794010013007, 5.463771816453670382 ) ) ;
#15592=CARTESIAN_POINT ( 'NONE',  ( 0.1289837059587395918, 106.1822392402443143, -5.211597877332949658 ) ) ;
#15593=CARTESIAN_POINT ( 'NONE',  ( -2.863213894092427658, 116.8186761214209213, 0.2817159656421849290 ) ) ;
#15598=FACE_OUTER_BOUND ( 'NONE', #26156, .T. ) ;
#15599=CARTESIAN_POINT ( 'NONE',  ( -5.953081049894649368, 155.3987518795295273, -0.06674817819388183249 ) ) ;
#15600=CARTESIAN_POINT ( 'NONE',  ( 3.006733222167471631, -15.59844357659602387, 5.538909454127313836 ) ) ;
#15601=CARTESIAN_POINT ( 'NONE',  ( -13.70042256496009614, 122.3361261571837986, 1.218568937077757264 ) ) ;
#15602=CARTESIAN_POINT ( 'NONE',  ( 15.72870526381831269, 122.9504679175852573, -0.8738493638518137763 ) ) ;
#15603=CARTESIAN_POINT ( 'NONE',  ( -3.158589313471108273, 4.191505055319898254, 3.400481138232230194 ) ) ;
#15605=ORIENTED_EDGE ( 'NONE', *, *, #12059, .F. ) ;
#15606=CARTESIAN_POINT ( 'NONE',  ( -0.008700780993364600618, 121.2597428844645293, 0.4354226598341946475 ) ) ;
#15608=CARTESIAN_POINT ( 'NONE',  ( -10.26617122093362333, 123.0849000269954701, 0.9769925898671679709 ) ) ;
#15610=CARTESIAN_POINT ( 'NONE',  ( 11.84733475906190314, 122.5845257805695923, -1.288679497020476905 ) ) ;
#15611=CARTESIAN_POINT ( 'NONE',  ( 0.02768730785345232051, 158.9256195073445213, -1.385586103196075447 ) ) ;
#15613=CARTESIAN_POINT ( 'NONE',  ( 9.485477581651457157, 123.8597080710187015, -0.4105858232041851852 ) ) ;
#15614=ORIENTED_EDGE ( 'NONE', *, *, #31641, .F. ) ;
#15615=CARTESIAN_POINT ( 'NONE',  ( -9.561780282765809602, 155.2307989660268959, -2.006535919638082088 ) ) ;
#15616=CARTESIAN_POINT ( 'NONE',  ( 3.866904830252686054, -15.34763638737450542, 1.784481441967298743 ) ) ;
#15617=CARTESIAN_POINT ( 'NONE',  ( -4.107451408814531746, 118.2429491485452928, -0.3509027312660569220 ) ) ;
#15620=CARTESIAN_POINT ( 'NONE',  ( -4.842027084325775554, 117.6755028110320183, 0.8981427047208370151 ) ) ;
#15621=CARTESIAN_POINT ( 'NONE',  ( -0.009931517865308202644, 119.6374844068871397, 0.4970137656763585210 ) ) ;
#15624=CARTESIAN_POINT ( 'NONE',  ( -2.614655561276646889, 23.60746518810343986, 3.812863311767609620 ) ) ;
#15625=CARTESIAN_POINT ( 'NONE',  ( 11.87576104716899117, 151.9737369308441544, 0.5463127210923327537 ) ) ;
#15627=B_SPLINE_CURVE_WITH_KNOTS ( 'NONE', 3,
 ( #30459, #40489, #37274, #20438, #13854, #23852, #27681 ),
 .UNSPECIFIED., .F., .F.,
 ( 4, 1, 1, 1, 4 ),
 ( 0.6462721360804385418, 0.7047636632187940231, 0.8031757754791960524, 0.9015878877395980817, 1.000000000000000000 ),
 .UNSPECIFIED. ) ;
#15630=CARTESIAN_POINT ( 'NONE',  ( -0.5995136777521792304, 117.9394517551924082, 1.384272192882745278 ) ) ;
#15633=CARTESIAN_POINT ( 'NONE',  ( -8.464895589923902008, 119.1960555687802525, -1.333724091418657220 ) ) ;
#15636=CARTESIAN_POINT ( 'NONE',  ( -10.81400209053381545, 157.9177219752764358, -0.09677702710655955443 ) ) ;
#15637=VERTEX_POINT ( 'NONE', #32561 ) ;
#15639=CARTESIAN_POINT ( 'NONE',  ( -6.939462325801320830, 121.9280307701022679, -0.3189346169104567141 ) ) ;
#15640=FACE_OUTER_BOUND ( 'NONE', #27071, .T. ) ;
#15641=ORIENTED_EDGE ( 'NONE', *, *, #38437, .T. ) ;
#15642=CARTESIAN_POINT ( 'NONE',  ( 2.027518441928002790, 115.7029486573731702, -1.637689744274474002 ) ) ;
#15643=CARTESIAN_POINT ( 'NONE',  ( -8.827910802435056326, 123.6950213215744583, -0.2595790122280455803 ) ) ;
#15644=CARTESIAN_POINT ( 'NONE',  ( 5.611934155553572445, -13.19144435144412064, 2.399925970747030846 ) ) ;
#15645=CARTESIAN_POINT ( 'NONE',  ( -5.880040083609346269, 118.0670013439590491, 0.7714800252663618352 ) ) ;
#15646=CARTESIAN_POINT ( 'NONE',  ( -5.071732749312718447, 117.1432901748061113, -0.6012547207297572749 ) ) ;
#15647=CARTESIAN_POINT ( 'NONE',  ( 23.18927481933079449, 149.6199392087789306, 0.6935230913228408456 ) ) ;
#15648=CARTESIAN_POINT ( 'NONE',  ( 0.6507712759201194075, 120.9971526617350577, 0.1121992020169609583 ) ) ;
#15649=DIRECTION ( 'NONE',  ( 4.017660918040594346E-17, -1.000000000000000000, -2.376309959284834438E-19 ) ) ;
#15650=CARTESIAN_POINT ( 'NONE',  ( -0.4721710868402241301, 14.98625149489145159, 0.8573358612705738180 ) ) ;
#15652=CARTESIAN_POINT ( 'NONE',  ( 0.0008202526017135117458, 159.6052337359418800, -0.04104879434819952433 ) ) ;
#15655=ORIENTED_EDGE ( 'NONE', *, *, #17045, .T. ) ;
#15656=CARTESIAN_POINT ( 'NONE',  ( 8.658023306739559999, 118.2891936209626778, 0.9762238836702761269 ) ) ;
#15658=CARTESIAN_POINT ( 'NONE',  ( 0.3865025759030094044, 117.6538564835029206, 0.5089310662413600861 ) ) ;
#15659=CARTESIAN_POINT ( 'NONE',  ( 20.17730036299072793, 147.7236477000422497, -1.702857440531004185 ) ) ;
#15660=CARTESIAN_POINT ( 'NONE',  ( -5.002256584969458686, 16.77047026005132224, -6.819937116506380903 ) ) ;
#15661=CARTESIAN_POINT ( 'NONE',  ( -3.924194517545539274, 117.4679918459733585, -0.7389123598820264149 ) ) ;
#15662=CARTESIAN_POINT ( 'NONE',  ( 4.726004515057145028, 117.8966366527547933, -0.7851610368387000882 ) ) ;
#15664=CARTESIAN_POINT ( 'NONE',  ( -9.119960873764156872, 153.9201329141909866, -0.06997149051007733878 ) ) ;
#15665=CARTESIAN_POINT ( 'NONE',  ( -18.87709319873820135, 147.8663216482595146, -2.479723349601893112 ) ) ;
#15666=CARTESIAN_POINT ( 'NONE',  ( 5.927515451590630313, -14.79481669900410701, -0.3156388015035426764 ) ) ;
#15667=CARTESIAN_POINT ( 'NONE',  ( 4.726250468511487668, 118.5931160184169073, 1.020578222860014872 ) ) ;
#15669=B_SPLINE_CURVE_WITH_KNOTS ( 'NONE', 3,
 ( #12128, #31293, #28316, #28529, #37906, #38332, #2137, #5759, #14890, #18293, #41534, #15099 ),
 .UNSPECIFIED., .F., .F.,
 ( 4, 1, 1, 1, 1, 1, 1, 1, 1, 4 ),
 ( 0.5426758968252777260, 0.5876249999999998419, 0.6700999999999999179, 0.7525749999999999940, 0.7938125000000000320, 0.8350499999999998479, 0.8762874999999994419, 0.9175249999999994799, 0.9587624999999999620, 0.9957666935384934526 ),
 .UNSPECIFIED. ) ;
#15672=B_SPLINE_SURFACE_WITH_KNOTS ( 'NONE', 3, 3, ( 
 ( #41212, #31401, #31183, #2453, #17765, #5227, #11803, #12013, #21790, #1614, #38008, #37375, #8192, #27576, #2025, #5653 ),
 ( #18608, #8830, #34818, #5018, #14990, #17979, #31614, #11382, #11591, #37789, #21161, #8616, #34394, #27991, #15414, #37580 ),
 ( #5434, #8407, #28418, #21367, #18390, #41424, #34194, #12231, #40584, #37171, #30976, #7995, #20963, #33984, #307, #35239 ),
 ( #9865, #13061, #25437, #18816, #6269, #26051, #22835, #39062, #12445, #25637, #35444, #38438, #3501, #12650, #29040, #42059 ),
 ( #19026, #3285, #22007, #31824, #22418, #32454, #15620, #16460, #2661, #19240, #28624, #41638, #16246, #35661, #9253, #28838 ),
 ( #25221, #29467, #9659, #38227, #9041, #35038, #29250, #32249, #12853, #22626, #25840, #35873, #6065, #32032, #22209, #15832 ),
 ( #16038, #6684, #41851, #2870, #38645, #3079, #6472, #19651, #94, #19447, #38848, #32667, #5858, #9451, #2358, #8524 ),
 ( #14894, #34311, #37283, #1936, #37485, #18298, #28322, #31095, #21694, #14479, #21075, #34720, #24480, #30887, #11708, #2143 ),
 ( #15316, #27897, #37910, #5550, #5139, #34101, #24911, #27490, #30675, #18507, #8102, #27692, #41331, #31512, #40904, #24696 ),
 ( #4928, #11495, #21483, #11921, #5765, #40700, #8944, #12133, #25125, #1728, #24278, #37702, #38127, #21910, #34941, #17885 ),
 ( #34516, #14685, #1523, #18092, #5342, #31297, #8733, #8310, #40498, #11293, #21281, #15103, #28105, #41115, #9977, #12348 ),
 ( #19551, #32147, #18931, #22532, #22736, #38544, #31941, #41752, #28535, #15943, #16145, #35767, #26168, #2980, #28939, #2777 ),
 ( #41541, #15733, #25338, #19347, #16361, #13181, #19143, #38752, #31728, #9561, #41956, #3395, #35978, #5969, #29147, #25954 ),
 ( #12757, #12960, #32560, #35561, #32354, #25743, #22320, #38341, #6377, #25542, #3182, #29367, #14851, #9772, #2572, #9158 ),
 ( #12553, #28738, #38961, #6584, #206, #39170, #22951, #18718, #15531, #35347, #22114, #35143, #9358, #6174, #36825, #26380 ),
 ( #4461, #7644, #7228, #20187, #13603, #14013, #14218, #17418, #7016, #6794, #27020, #3829, #16793, #33213, #1263, #23159 ),
 ( #39387, #32783, #10405, #19761, #16576, #634, #17213, #24017, #27227, #39819, #4038, #4250, #1050, #23594, #40240, #39602 ),
 ( #19984, #33001, #26811, #26594, #29794, #30210, #20602, #17000, #23377, #10612, #10822, #36410, #29999, #839, #29587, #13813 ),
 ( #23805, #11035, #36616, #7435, #20393, #33420, #421, #40029, #13391, #33634, #30415, #3613, #10190, #36195, #7853, #27847 ),
 ( #21645, #40854, #28271, #2090, #41063, #30832, #15266, #11657, #34259, #24641, #21433, #14635, #4879, #8257, #34669, #2306 ),
 ( #5499, #31042, #33839, #40648, #37234, #37653, #11874, #27636, #8053, #17834, #4667, #5088, #34461, #24863, #41277, #21229 ),
 ( #18040, #17624, #8477, #1679, #12083, #11442, #24225, #30626, #1469, #5294, #18458, #37035, #18243, #15054, #14426, #28054 ),
 ( #24430, #20813, #31248, #1880, #37859, #8681, #37435, #14843, #31462, #27433, #40449, #21026, #11240, #34049, #21859, #28690 ),
 ( #12296, #36097, #32896, #35888, #9878, #19881, #39499, #3516, #39285, #22848, #41698, #31678, #39076, #31891, #13290, #23273 ) ),
 .UNSPECIFIED., .F., .F., .F.,
 ( 4, 2, 2, 2, 2, 2, 2, 2, 2, 2, 2, 4 ),
 ( 4, 2, 2, 2, 2, 1, 1, 2, 4 ),
 ( 0.000000000000000000, 0.1320156187279754312, 0.1980234280919631606, 0.2640312374559508624, 0.3918846486443451349, 0.4558113542385422989, 0.5197380598327394630, 0.5807839412718216465, 0.6418298227109038301, 0.7639215855890681972, 0.8819607927945340986, 1.000000000000000000 ),
 ( 0.000000000000000000, 0.1250000000000000000, 0.2500000000000000000, 0.3750000000000000000, 0.5000000000000000000, 0.7500000000000000000, 0.8750000000000000000, 0.9375000000000000000, 1.000000000000000000 ),
 .UNSPECIFIED. ) ;
#15673=CARTESIAN_POINT ( 'NONE',  ( 18.29546242682543422, 149.1773161885088825, 2.457454238777247557 ) ) ;
#15675=VECTOR ( 'NONE', #7897, 1000.000000000000114 ) ;
#15677=CARTESIAN_POINT ( 'NONE',  ( -0.9965922269827753865, 107.7619142660649203, 4.530701086038176228 ) ) ;
#15678=CARTESIAN_POINT ( 'NONE',  ( 6.819937116507564845, -4.819529739946951885, -5.002256584970107056 ) ) ;
#15679=CARTESIAN_POINT ( 'NONE',  ( 16.02106284285049753, 145.8417561620165372, 1.176135107295965154 ) ) ;
#15681=CARTESIAN_POINT ( 'NONE',  ( 3.845766519666786287, 116.9593488885201538, -0.3368132424836104977 ) ) ;
#15685=CARTESIAN_POINT ( 'NONE',  ( -6.894732321505390615, 117.1676844715483270, -0.1377731603346601386 ) ) ;
#15687=CARTESIAN_POINT ( 'NONE',  ( 6.362922045609294308, 119.9956554345082935, -0.9575366525960410380 ) ) ;
#15688=CARTESIAN_POINT ( 'NONE',  ( -5.332935397695336199, 116.0444662015457311, -0.1065647409268299234 ) ) ;
#15689=CARTESIAN_POINT ( 'NONE',  ( -14.53200193279647223, 139.1552669279217298, -1.026914593849030943 ) ) ;
#15690=CARTESIAN_POINT ( 'NONE',  ( -5.064403469544192404, 117.2685460503076627, 0.4793543776217523145 ) ) ;
#15692=CARTESIAN_POINT ( 'NONE',  ( 23.36005780523110431, 148.8745345081378559, 0.4925575130201677032 ) ) ;
#15693=VERTEX_POINT ( 'NONE', #37036 ) ;
#15694=CARTESIAN_POINT ( 'NONE',  ( 0.1710433496020407063, 14.98650505531991506, 4.637963194678765610 ) ) ;
#15700=CARTESIAN_POINT ( 'NONE',  ( 6.103784187571975828, 121.1829703657862751, 0.6769658165800259697 ) ) ;
#15701=EDGE_CURVE ( 'NONE', #11376, #28135, #17625, .T. ) ;
#15702=CARTESIAN_POINT ( 'NONE',  ( 1.305078825605721526, 159.4185946040361728, 0.8784184817623138519 ) ) ;
#15703=CARTESIAN_POINT ( 'NONE',  ( 3.350153020191438014, 104.6144662015457385, -3.487106363639548512 ) ) ;
#15705=CARTESIAN_POINT ( 'NONE',  ( 11.79681931163863595, 156.4111399680655552, -1.533406117021610227 ) ) ;
#15707=CARTESIAN_POINT ( 'NONE',  ( -0.03066982525788228969, 157.3074135339440147, 1.534843470138540722 ) ) ;
#15708=CARTESIAN_POINT ( 'NONE',  ( 3.750385610654966229, 4.675867361267946443, -2.714424430587211834 ) ) ;
#15709=CARTESIAN_POINT ( 'NONE',  ( -14.81745968805125102, 156.1223461918646933, -1.150419650929870530 ) ) ;
#15710=ADVANCED_FACE ( 'NONE', ( #30627 ), #31020, .T. ) ;
#15713=CARTESIAN_POINT ( 'NONE',  ( -13.24427968334914851, 134.0707761029912035, 0.3110103029741254077 ) ) ;
#15714=CARTESIAN_POINT ( 'NONE',  ( 5.179289707447474633, -13.00434337860746581, 2.646125397160491222 ) ) ;
#15715=CARTESIAN_POINT ( 'NONE',  ( -0.03519895178523997636, 115.7029491485446613, 1.761499482104069703 ) ) ;
#15716=CARTESIAN_POINT ( 'NONE',  ( -4.558806136799320008, 118.0156478519566576, -0.8816215797218194261 ) ) ;
#15717=CARTESIAN_POINT ( 'NONE',  ( 12.85860202769631755, 133.7716054015561156, 0.2569454702854387373 ) ) ;
#15718=ORIENTED_EDGE ( 'NONE', *, *, #25394, .F. ) ;
#15719=CARTESIAN_POINT ( 'NONE',  ( 8.740007204533831953, 120.0394951565550343, 1.484413609726634942 ) ) ;
#15723=CARTESIAN_POINT ( 'NONE',  ( -22.08264656579488161, 150.6352520364973486, 0.6282006774575533692 ) ) ;
#15724=CARTESIAN_POINT ( 'NONE',  ( 4.851964763131728198, 117.4768176267210009, -0.9923522720269655206 ) ) ;
#15725=CARTESIAN_POINT ( 'NONE',  ( 0.9295402922911353283, 116.5712332538976455, -0.1496640007645968773 ) ) ;
#15727=TOROIDAL_SURFACE ( 'NONE', #39576, 3.683000000000000718, 0.5080000000000000071 ) ;
#15728=CARTESIAN_POINT ( 'NONE',  ( 5.295064810963916457, 115.6909491485453145, 0.7219800058539025400 ) ) ;
#15730=CARTESIAN_POINT ( 'NONE',  ( -4.812635773683934026, 117.4067914754907065, -1.196957445793439989 ) ) ;
#15733=CARTESIAN_POINT ( 'NONE',  ( -4.572877053309778006, 118.0343149336223831, 0.6783132061656282907 ) ) ;
#15735=ORIENTED_EDGE ( 'NONE', *, *, #32280, .T. ) ;
#15736=VERTEX_POINT ( 'NONE', #31043 ) ;
#15737=CARTESIAN_POINT ( 'NONE',  ( -1.967456252267424155, 118.7629491485468236, -1.232493637335213332 ) ) ;
#15738=CARTESIAN_POINT ( 'NONE',  ( -6.004173374711351485, 119.3322421624460077, -1.266279038469856122 ) ) ;
#15739=CARTESIAN_POINT ( 'NONE',  ( -2.208446607403949713, 108.4767889311100362, -4.246804138318780453 ) ) ;
#15740=CARTESIAN_POINT ( 'NONE',  ( 4.636258067987869325, 118.0184330405641333, 0.8097526809780418722 ) ) ;
#15743=CARTESIAN_POINT ( 'NONE',  ( -12.84263471596180928, 130.8243885708800747, -1.276791159582618018 ) ) ;
#15744=CARTESIAN_POINT ( 'NONE',  ( 1.360477052538118681, -3.804838552850991817, 4.419457122809256511 ) ) ;
#15747=CARTESIAN_POINT ( 'NONE',  ( 5.317809737553744753, 116.7000894413872629, -0.8094161617621952187 ) ) ;
#15748=CARTESIAN_POINT ( 'NONE',  ( -10.41670863957363302, 122.9580799906392343, -1.467069541016856826 ) ) ;
#15749=CARTESIAN_POINT ( 'NONE',  ( 21.68875320759051917, 132.7412702629105468, 0.4333929054516009183 ) ) ;
#15750=CARTESIAN_POINT ( 'NONE',  ( -5.307248809044878612, 31.23445644987117120, 3.607707940702756133 ) ) ;
#15752=CARTESIAN_POINT ( 'NONE',  ( -4.012847786888796620, 11.73797844546971270, -2.294585225469591983 ) ) ;
#15753=CARTESIAN_POINT ( 'NONE',  ( 7.852582050918188727, 158.6543443936584481, 0.7853876145049530910 ) ) ;
#15755=CARTESIAN_POINT ( 'NONE',  ( -1.944567074771800241, 104.6144662015455111, -4.425999150025703877 ) ) ;
#15756=CARTESIAN_POINT ( 'NONE',  ( 3.885490704569380060, -15.31119228946847777, 1.341400144935093630 ) ) ;
#15757=CARTESIAN_POINT ( 'NONE',  ( -5.880668475635614456, 119.2401804501882197, 0.9647153462086465181 ) ) ;
#15759=CARTESIAN_POINT ( 'NONE',  ( -0.8274880129334906131, 26.04165684986237039, -0.5117960016238547460 ) ) ;
#15760=AXIS2_PLACEMENT_3D ( 'NONE', #34159, #30946, #27122 ) ;
#15761=EDGE_CURVE ( 'NONE', #24980, #17144, #28484, .T. ) ;
#15762=CARTESIAN_POINT ( 'NONE',  ( 0.8097498057273965211, -0.1318080948593848278, -0.5455758836208917106 ) ) ;
#15767=CARTESIAN_POINT ( 'NONE',  ( 6.475519728870414049, 122.5560431351108974, 0.2403424393823896110 ) ) ;
#15768=CARTESIAN_POINT ( 'NONE',  ( -15.20409169301252739, 148.9716719698033387, 0.7946991634813627137 ) ) ;
#15769=FACE_OUTER_BOUND ( 'NONE', #1730, .T. ) ;
#15770=CARTESIAN_POINT ( 'NONE',  ( 2.584330390446285985, -14.72226154538576459, 5.166463236119047231 ) ) ;
#15771=CARTESIAN_POINT ( 'NONE',  ( 3.787250209144782165, 156.8112981010400802, -1.501541828261893086 ) ) ;
#15772=CARTESIAN_POINT ( 'NONE',  ( -4.978738709155277498, 118.8869175073591578, -1.099525347370199135 ) ) ;
#15774=CARTESIAN_POINT ( 'NONE',  ( 7.976738704924626333, 121.5955735554254602, 1.139979217470462158 ) ) ;
#15775=FACE_OUTER_BOUND ( 'NONE', #11037, .T. ) ;
#15776=CARTESIAN_POINT ( 'NONE',  ( 15.42372963437252587, 147.8340308814284754, -0.02010286832636620433 ) ) ;
#15779=CARTESIAN_POINT ( 'NONE',  ( 0.1066493941974573784, 105.7853621660184444, -5.332931186019219005 ) ) ;
#15780=CARTESIAN_POINT ( 'NONE',  ( 4.898459268277319367, 117.7581306180235288, -0.6108534173935511458 ) ) ;
#15781=CARTESIAN_POINT ( 'NONE',  ( -2.798479926918381544, 16.31753791307728818, -7.953355231451358698 ) ) ;
#15782=CARTESIAN_POINT ( 'NONE',  ( 6.488156926834022897, 121.4051597255373025, 0.7118474008431251443 ) ) ;
#15783=CARTESIAN_POINT ( 'NONE',  ( 3.682264917456192777, 84.67546620154573134, 0.07358041635424013294 ) ) ;
#15784=CARTESIAN_POINT ( 'NONE',  ( 17.27060146982319466, 122.7565812399420651, 0.2921901055230267108 ) ) ;
#15785=CARTESIAN_POINT ( 'NONE',  ( -7.643893061813611389, 124.7210964017841377, -0.1527835634684687749 ) ) ;
#15788=CARTESIAN_POINT ( 'NONE',  ( 8.041889123127029748, 122.8518031662551948, 0.1606960833125207766 ) ) ;
#15789=CARTESIAN_POINT ( 'NONE',  ( 19.44881300980840777, 136.0480396440595996, 2.307899331309748003 ) ) ;
#15790=CARTESIAN_POINT ( 'NONE',  ( 0.3193725800214416988, -13.04287899337829515, -8.422265478599168631 ) ) ;
#15791=CARTESIAN_POINT ( 'NONE',  ( 8.748550937609889999, 117.9820647352999003, -0.4023511751121509050 ) ) ;
#15792=CARTESIAN_POINT ( 'NONE',  ( -0.2949767777650753042, 114.7739974199301116, -2.049407731665748411 ) ) ;
#15795=CARTESIAN_POINT ( 'NONE',  ( 1.765626013768924807, -4.031643488171090972, 8.243228240708695864 ) ) ;
#15797=FACE_OUTER_BOUND ( 'NONE', #24156, .T. ) ;
#15798=CARTESIAN_POINT ( 'NONE',  ( 3.092642723064080279, -14.67800799544728285, 3.675123631970977911 ) ) ;
#15799=CARTESIAN_POINT ( 'NONE',  ( 1.034729067459722485, 124.2655319029901335, -0.03890078971358913035 ) ) ;
#15800=CARTESIAN_POINT ( 'NONE',  ( -0.009748065369249884343, 159.5507987164374981, 0.4878330526048098581 ) ) ;
#15802=ORIENTED_EDGE ( 'NONE', *, *, #22254, .F. ) ;
#15804=ADVANCED_FACE ( 'NONE', ( #37860 ), #10614, .T. ) ;
#15805=VERTEX_POINT ( 'NONE', #18548 ) ;
#15807=CARTESIAN_POINT ( 'NONE',  ( 3.361984464572039144, -15.63109852379819564, 5.271848418269179604 ) ) ;
#15808=CARTESIAN_POINT ( 'NONE',  ( -20.67621894907605196, 148.5655811199389689, 1.615315227278341537 ) ) ;
#15809=CARTESIAN_POINT ( 'NONE',  ( 12.49407882476840115, 156.7420262770442037, -1.161473977901223531 ) ) ;
#15811=CARTESIAN_POINT ( 'NONE',  ( -1.214995109038484067, 0.9429784454696930052, -4.460028654918597901 ) ) ;
#15815=CARTESIAN_POINT ( 'NONE',  ( 0.3588522330932212845, 120.9711055683163323, 0.4900691623393884644 ) ) ;
#15817=CARTESIAN_POINT ( 'NONE',  ( -17.27955699683406721, 146.3482411845097886, 1.367784599882192476 ) ) ;
#15819=CARTESIAN_POINT ( 'NONE',  ( 6.683041398157518742, 119.8184877057495754, -1.002300253150233411 ) ) ;
#15820=CARTESIAN_POINT ( 'NONE',  ( -7.819746389599830927, 118.9574329095587757, -1.279815391681077275 ) ) ;
#15824=CARTESIAN_POINT ( 'NONE',  ( 7.108627447324208148, 121.8675249661327626, -0.3373703349335457902 ) ) ;
#15825=ORIENTED_EDGE ( 'NONE', *, *, #23245, .F. ) ;
#15826=CARTESIAN_POINT ( 'NONE',  ( -10.86423259349712467, 154.4230204216147513, -2.019759596344636865 ) ) ;
#15827=CARTESIAN_POINT ( 'NONE',  ( 3.037377538037926428, -15.29769487807139328, 4.066060606540134792 ) ) ;
#15828=CARTESIAN_POINT ( 'NONE',  ( -4.112438057953108128, 118.2429491485453070, -0.3456707284627133503 ) ) ;
#15829=AXIS2_PLACEMENT_3D ( 'NONE', #36819, #21020, #34043 ) ;
#15832=CARTESIAN_POINT ( 'NONE',  ( -4.909535097854543118, 117.7132662139654684, 0.7284956952065094749 ) ) ;
#15833=CARTESIAN_POINT ( 'NONE',  ( 17.32761985034175822, 148.7932787949812905, 2.272318092294528746 ) ) ;
#15835=CARTESIAN_POINT ( 'NONE',  ( 0.2838385327444274964, 29.22985346960623332, -4.617364983570896086 ) ) ;
#15836=CARTESIAN_POINT ( 'NONE',  ( 15.27538331669044780, 143.4753230507764670, 0.6393389556987906230 ) ) ;
#15845=DIRECTION ( 'NONE',  ( 0.9998004120163608288, 0.000000000000000000, 0.01997839162482749342 ) ) ;
#15847=CARTESIAN_POINT ( 'NONE',  ( -16.81673201796769845, 155.2524275687165982, -0.03818847721824999292 ) ) ;
#15850=CARTESIAN_POINT ( 'NONE',  ( -7.796374419565617941, 122.5468937217193997, -0.4035712047578281503 ) ) ;
#15851=CARTESIAN_POINT ( 'NONE',  ( 5.152689472752729039, 116.8412042436348912, 0.1029629964107459106 ) ) ;
#15853=CARTESIAN_POINT ( 'NONE',  ( 1.626908944290321735, 115.7027889457816769, -1.667109174786431280 ) ) ;
#15854=CARTESIAN_POINT ( 'NONE',  ( -9.242391706085612668, 124.1957968681474824, -0.3461533994140003068 ) ) ;
#15855=CARTESIAN_POINT ( 'NONE',  ( 6.023256536641487635, -13.63339314725699225, 2.031454315062427796 ) ) ;
#15856=CARTESIAN_POINT ( 'NONE',  ( -13.26523119301606002, 121.0513591912305316, 0.9938426049807239648 ) ) ;
#15857=CARTESIAN_POINT ( 'NONE',  ( -5.124566020981691672, 116.9360569234986116, -0.3865489709985214795 ) ) ;
#15859=CARTESIAN_POINT ( 'NONE',  ( 22.81319227410996220, 150.4043717142618277, 0.6849243123989299242 ) ) ;
#15860=CARTESIAN_POINT ( 'NONE',  ( 8.877428936179040164, 123.9526547814713950, 0.3101401378828683164 ) ) ;
#15862=CARTESIAN_POINT ( 'NONE',  ( 0.9699771559235883522, 8.716109271805494885, -0.1015519487743763993 ) ) ;
#15863=CARTESIAN_POINT ( 'NONE',  ( -6.903663268456499580, 117.1865127098105575, -0.2656477445430289186 ) ) ;
#15867=CARTESIAN_POINT ( 'NONE',  ( -8.690633472767538947, 118.2864615337380485, 0.6276850432433955795 ) ) ;
#15870=CARTESIAN_POINT ( 'NONE',  ( 5.110479671343659547, 158.7070047875298826, 1.445852496635407824 ) ) ;
#15871=CARTESIAN_POINT ( 'NONE',  ( 4.124323422701878350, 118.5849532427036905, -0.8258982430451993206 ) ) ;
#15872=CARTESIAN_POINT ( 'NONE',  ( -7.300781474974964880, 17.39199087320084658, -4.267473507878162486 ) ) ;
#15873=CARTESIAN_POINT ( 'NONE',  ( -21.70861548485266113, 150.3096123636779566, -1.869307503447338314 ) ) ;
#15874=CARTESIAN_POINT ( 'NONE',  ( 4.749224635152644147, 117.9454780248063059, -0.6340590349429241490 ) ) ;
#15876=CARTESIAN_POINT ( 'NONE',  ( -15.81024248929847964, 146.2514283349100594, -0.08545504004084561456 ) ) ;
#15877=CARTESIAN_POINT ( 'NONE',  ( -3.283742410131533784, 119.1333808041459577, -0.8926212079385045239 ) ) ;
#15878=CARTESIAN_POINT ( 'NONE',  ( 5.620948709224020234, -15.12563517700941951, 1.754161952847088868 ) ) ;
#15880=CARTESIAN_POINT ( 'NONE',  ( 4.744456427932504994, 118.5931160184169073, 1.015333858321567861 ) ) ;
#15883=ORIENTED_EDGE ( 'NONE', *, *, #35752, .F. ) ;
#15884=CARTESIAN_POINT ( 'NONE',  ( 12.63334184343642796, 124.0847267554996591, 1.843480660383216563 ) ) ;
#15887=CARTESIAN_POINT ( 'NONE',  ( -3.075034626192941101, 115.9530684888725460, 1.465612804093755495 ) ) ;
#15888=CARTESIAN_POINT ( 'NONE',  ( -3.468545696377880461, 29.88095345675903403, -7.690089085670218871 ) ) ;
#15889=CARTESIAN_POINT ( 'NONE',  ( 13.85976170726103796, 150.2454140652271803, 1.103110692033626217 ) ) ;
#15890=CARTESIAN_POINT ( 'NONE',  ( 22.38075128446548234, 150.2360280492587776, -0.6257272249761318683 ) ) ;
#15892=TOROIDAL_SURFACE ( 'NONE', #28159, 3.683000000000000718, 0.5080000000000000071 ) ;
#15894=EDGE_CURVE ( 'NONE', #10310, #1073, #40113, .T. ) ;
#15895=CARTESIAN_POINT ( 'NONE',  ( -8.075779052176619288, 158.6620026115301698, -0.1430648235678988744 ) ) ;
#15896=ORIENTED_EDGE ( 'NONE', *, *, #30451, .T. ) ;
#15897=CARTESIAN_POINT ( 'NONE',  ( -8.196833826245901733, 120.4943603722682326, -1.426315956448065636 ) ) ;
#15898=CARTESIAN_POINT ( 'NONE',  ( 22.98488057257191741, 150.1591296352320910, 0.4592926148156237232 ) ) ;
#15900=CARTESIAN_POINT ( 'NONE',  ( -9.400309931224136051, 124.0858766813489780, -0.6109843400649569434 ) ) ;
#15901=CARTESIAN_POINT ( 'NONE',  ( -5.146090777129525229, 116.8856917068506220, 0.08017679380233867781 ) ) ;
#15902=CARTESIAN_POINT ( 'NONE',  ( 10.83330528665002923, 157.8980211815716928, 0.2164752214609689529 ) ) ;
#15905=CARTESIAN_POINT ( 'NONE',  ( -2.359559261509405204, 14.11188314818778267, 3.974389579228013503 ) ) ;
#15907=CARTESIAN_POINT ( 'NONE',  ( -5.008553077021508315, 117.3993868461436421, 0.7755932514345632578 ) ) ;
#15909=CARTESIAN_POINT ( 'NONE',  ( -6.431420355030265265E-14, 156.3034662015457172, 9.897580308537652682E-17 ) ) ;
#15910=CARTESIAN_POINT ( 'NONE',  ( -7.840345251802245841, 122.4018557723364040, 0.3085103408382670054 ) ) ;
#15911=CARTESIAN_POINT ( 'NONE',  ( 1.100877510726109954, 5.750359496286542971, -4.487862572965156005 ) ) ;
#15912=CARTESIAN_POINT ( 'NONE',  ( 10.25083424799698228, 157.8242135995235458, 1.281710951059998882 ) ) ;
#15913=DIRECTION ( 'NONE',  ( -0.9998004120163608288, 0.000000000000000000, -0.01997839162482749342 ) ) ;
#15914=CARTESIAN_POINT ( 'NONE',  ( 3.026662605148213725, -13.87242449132548217, 1.205013440933411228 ) ) ;
#15915=CARTESIAN_POINT ( 'NONE',  ( 13.46025642088307883, 121.5866728338796463, -1.110021706884414261 ) ) ;
#15916=CARTESIAN_POINT ( 'NONE',  ( 4.627658001546194555, 13.29687521248714610, 0.05192310334374634212 ) ) ;
#15917=CARTESIAN_POINT ( 'NONE',  ( -1.349732659538083190, 159.5224216140176168, -0.6194554754934779028 ) ) ;
#15920=EDGE_CURVE ( 'NONE', #32786, #34625, #11642, .T. ) ;
#15921=CARTESIAN_POINT ( 'NONE',  ( -12.05713894362187766, 151.9703418938154584, 0.4396675171196801069 ) ) ;
#15922=CARTESIAN_POINT ( 'NONE',  ( 6.231544205925810154, -13.28212530995504004, 1.212557631246017564 ) ) ;
#15924=CARTESIAN_POINT ( 'NONE',  ( -4.696919984883029642, 117.9693496385861380, -0.8143052264822483455 ) ) ;
#15925=CARTESIAN_POINT ( 'NONE',  ( 9.049782359939477772, 124.0675141969884692, 0.1808361888366266657 ) ) ;
#15926=ORIENTED_EDGE ( 'NONE', *, *, #30573, .T. ) ;
#15927=EDGE_CURVE ( 'NONE', #9488, #41007, #31976, .T. ) ;
#15928=CARTESIAN_POINT ( 'NONE',  ( 19.94553544501711428, 148.6304843473828043, 2.499072228797275308 ) ) ;
#15932=CARTESIAN_POINT ( 'NONE',  ( -19.39512251848563906, 128.7092500879292345, 0.6293422422100684033 ) ) ;
#15933=ADVANCED_FACE ( 'NONE', ( #19591 ), #10970, .T. ) ;
#15934=CARTESIAN_POINT ( 'NONE',  ( -6.431420355030265265E-14, 156.3034662015457172, 9.897580308537652682E-17 ) ) ;
#15935=CARTESIAN_POINT ( 'NONE',  ( 23.27509581586231491, 146.7258352529021863, -0.1368228026537801900 ) ) ;
#15936=CARTESIAN_POINT ( 'NONE',  ( -4.910976174659007043, 115.7029491485453576, -1.454476526932306113 ) ) ;
#15939=CARTESIAN_POINT ( 'NONE',  ( -4.757313731898603848, 117.4006812934349284, -1.206872148879561513 ) ) ;
#15940=EDGE_CURVE ( 'NONE', #32067, #33842, #13160, .T. ) ;
#15943=CARTESIAN_POINT ( 'NONE',  ( -4.652583246796857530, 118.0213927529021731, 0.6398161096456489449 ) ) ;
#15946=CARTESIAN_POINT ( 'NONE',  ( -0.6720308294796238924, 115.6909491485452435, -1.760267559040072483 ) ) ;
#15947=CARTESIAN_POINT ( 'NONE',  ( 3.456802958751930888, 118.5942819653431002, -0.7917318383961905459 ) ) ;
#15948=CARTESIAN_POINT ( 'NONE',  ( -6.868335724905657358, 121.8312213470058225, -0.2935230024867366838 ) ) ;
#15949=CARTESIAN_POINT ( 'NONE',  ( 4.798460879778644106, 117.8359694357527161, 0.9162085815312616122 ) ) ;
#15950=CARTESIAN_POINT ( 'NONE',  ( 3.075357915497110017, -13.94103813162880989, 1.416127232796946966 ) ) ;
#15951=CARTESIAN_POINT ( 'NONE',  ( -16.44150122627331001, 146.0252812507985141, -1.609049209688530935 ) ) ;
#15952=CARTESIAN_POINT ( 'NONE',  ( -1.787119016036921693, 115.7029469008264186, -1.723302017833900912 ) ) ;
#15953=CARTESIAN_POINT ( 'NONE',  ( -2.745631362450760893, 107.6373487222285235, 4.456378253842885329 ) ) ;
#15955=CARTESIAN_POINT ( 'NONE',  ( 3.556334529072911366, 108.6891572770382624, -3.980722479600265817 ) ) ;
#15956=CARTESIAN_POINT ( 'NONE',  ( -9.877803879600318027, 122.5082557396031291, -1.415055850893564227 ) ) ;
#15958=CARTESIAN_POINT ( 'NONE',  ( -0.3252752853362120833, 37.07821745674546321, 2.201007984806573337 ) ) ;
#15960=CARTESIAN_POINT ( 'NONE',  ( 4.440015753948663324, -2.305524871907271400, 1.325333094644747245 ) ) ;
#15961=CARTESIAN_POINT ( 'NONE',  ( 2.849674052733008889, 116.8186761214209213, 0.3958730627374474342 ) ) ;
#15964=CARTESIAN_POINT ( 'NONE',  ( 3.489657270499090025, -15.47349394630789732, 3.491754635552897668 ) ) ;
#15965=CARTESIAN_POINT ( 'NONE',  ( -12.68516923343336700, 122.7135068550949200, 1.328447112472142644 ) ) ;
#15966=CARTESIAN_POINT ( 'NONE',  ( -0.7381358996182917354, 6.602865006980263018, -0.6401951644792284180 ) ) ;
#15967=CARTESIAN_POINT ( 'NONE',  ( 0.8978640518332915432, -1.652899491467043180, 0.3817720442996600516 ) ) ;
#15971=CARTESIAN_POINT ( 'NONE',  ( 3.148404055479938624, 118.0279923103727242, 0.8990514348027990321 ) ) ;
#15972=CARTESIAN_POINT ( 'NONE',  ( -13.14213916796054349, 130.8944540161131442, 0.9043360416341286179 ) ) ;
#15973=CARTESIAN_POINT ( 'NONE',  ( 3.009276887026297587, 39.20946620154573736, -1.210121013456480599 ) ) ;
#15974=CARTESIAN_POINT ( 'NONE',  ( 2.810721824165392846, -14.60963343767143741, 5.218503737131710452 ) ) ;
#15975=CARTESIAN_POINT ( 'NONE',  ( 12.06094766868686463, 124.3217332413628640, -1.226997676231848855 ) ) ;
#15976=CARTESIAN_POINT ( 'NONE',  ( -19.13795181554008096, 149.5120288530235655, -2.492102325696694987 ) ) ;
#15978=CARTESIAN_POINT ( 'NONE',  ( 1.824654213811243819, -15.25386490109567639, 5.420715704377902178 ) ) ;
#15979=CARTESIAN_POINT ( 'NONE',  ( -0.02287401428062574640, 38.91018238071126945, -0.8096150143283803446 ) ) ;
#15980=CARTESIAN_POINT ( 'NONE',  ( 0.6320890182442912009, 120.8998192842950488, -0.1133706938477902909 ) ) ;
#15984=ADVANCED_FACE ( 'NONE', ( #2400 ), #17950, .T. ) ;
#15986=CARTESIAN_POINT ( 'NONE',  ( -0.006810764310409325381, 120.3493709785083183, 0.3408384964863779287 ) ) ;
#15988=CARTESIAN_POINT ( 'NONE',  ( 22.53566265713729422, 150.7862151120626777, 0.3736683405004933012 ) ) ;
#15989=EDGE_CURVE ( 'NONE', #2340, #40423, #23330, .T. ) ;
#15990=CARTESIAN_POINT ( 'NONE',  ( -4.047044637104160181, 109.8183322527596602, 3.518666775989008677 ) ) ;
#15992=DIRECTION ( 'NONE',  ( -5.206863593109713661E-17, 1.000000000000000000, -1.077750396879097183E-30 ) ) ;
#15993=DIRECTION ( 'NONE',  ( -0.01997839162482737546, -1.040247600000940825E-18, 0.9998004120163610509 ) ) ;
#15994=CARTESIAN_POINT ( 'NONE',  ( -4.460903749329073520, 31.58350409445925777, -0.5211678667172463530 ) ) ;
#15995=CARTESIAN_POINT ( 'NONE',  ( 9.341440546823472246, 157.3305555497073271, 1.901068499721875193 ) ) ;
#15997=CARTESIAN_POINT ( 'NONE',  ( -1.220754042303205500, 16.12054255322086860, -4.471266627502475721 ) ) ;
#15998=CARTESIAN_POINT ( 'NONE',  ( 4.725500162001525339, -13.89046571553399900, -6.993667195001821213 ) ) ;
#15999=CARTESIAN_POINT ( 'NONE',  ( 5.512123453640334070, 117.2133480785072521, -0.5884807297197708342 ) ) ;
#16000=CARTESIAN_POINT ( 'NONE',  ( 0.01254005783532663974, 120.1716774721351157, -0.6275557724548020966 ) ) ;
#16002=CARTESIAN_POINT ( 'NONE',  ( 2.745797790083741141, 107.6376760790657698, -4.456235498929850714 ) ) ;
#16003=CARTESIAN_POINT ( 'NONE',  ( -1.939848034429841217, 105.1240075698378575, 4.970163540756382226 ) ) ;
#16004=CARTESIAN_POINT ( 'NONE',  ( 2.889066315880882030, 25.55657059589919911, 3.609430016826872478 ) ) ;
#16006=CARTESIAN_POINT ( 'NONE',  ( -23.36555825341177339, 148.7788340588663800, -0.4668994608413308267 ) ) ;
#16007=CARTESIAN_POINT ( 'NONE',  ( 2.969447359227861405, -13.80100253337253946, 0.9847735008004718793 ) ) ;
#16008=CARTESIAN_POINT ( 'NONE',  ( 2.274554406286624975, 117.6064948828932444, -1.027890184761801384 ) ) ;
#16009=CARTESIAN_POINT ( 'NONE',  ( -15.52007106302766282, 121.3130774642648220, 0.3850180365863631327 ) ) ;
#16014=CARTESIAN_POINT ( 'NONE',  ( 2.394017677299879576, -15.71294128685811486, 5.613897423981592638 ) ) ;
#16015=CARTESIAN_POINT ( 'NONE',  ( -0.01111639779269613798, 118.2594330468507593, 0.5563100024230164253 ) ) ;
#16016=CARTESIAN_POINT ( 'NONE',  ( 10.00431039430831248, 157.6892375622926181, -1.152258088200127650 ) ) ;
#16017=CARTESIAN_POINT ( 'NONE',  ( 2.829288187452689396, 6.340478445469713620, 3.655570690059357197 ) ) ;
#16021=CARTESIAN_POINT ( 'NONE',  ( 0.3855071059147253676, 123.1683257372383054, 0.1933446952578523892 ) ) ;
#16024=CARTESIAN_POINT ( 'NONE',  ( -2.563812760316581674, 119.9929590031203901, 0.5332384965226231177 ) ) ;
#16026=CARTESIAN_POINT ( 'NONE',  ( 4.236690124160776172, 119.4047208153655646, -0.8054972593864422326 ) ) ;
#16027=CARTESIAN_POINT ( 'NONE',  ( -14.93032553133231310, 154.7288491705591866, -2.132398917750006451 ) ) ;
#16030=CARTESIAN_POINT ( 'NONE',  ( 4.493176929058669167, 118.1153340809138257, -0.5662424233016255526 ) ) ;
#16031=CARTESIAN_POINT ( 'NONE',  ( 4.488166000884652007, 120.9326014760084007, -0.2785428184686806752 ) ) ;
#16034=CARTESIAN_POINT ( 'NONE',  ( -0.5297590882382788857, 119.7690751942239729, -0.5117926329762007009 ) ) ;
#16035=CARTESIAN_POINT ( 'NONE',  ( 3.302563718500166612, -15.23312206205887342, 3.441858572223985391 ) ) ;
#16038=CARTESIAN_POINT ( 'NONE',  ( -4.737627528408766331, 117.7521883752312419, 0.9000133201668191196 ) ) ;
#16039=CARTESIAN_POINT ( 'NONE',  ( 15.36238541928142887, 134.8939017613128328, 2.058614936883395696 ) ) ;
#16040=CARTESIAN_POINT ( 'NONE',  ( -1.606566256928684933, 32.19982401495065716, 1.077694121983206799 ) ) ;
#16042=CARTESIAN_POINT ( 'NONE',  ( 5.678980076864418969, -10.27674996446047828, -6.244917620322217644 ) ) ;
#16043=CARTESIAN_POINT ( 'NONE',  ( 7.835359239711011448, 154.6110463214094182, 0.4315757689284727139 ) ) ;
#16046=CARTESIAN_POINT ( 'NONE',  ( -0.01811615190475213133, 118.1588900175948709, 0.9066062283863981497 ) ) ;
#16049=CARTESIAN_POINT ( 'NONE',  ( -8.198442868473685863, 120.4868523889126095, -1.425315046605219127 ) ) ;
#16054=CARTESIAN_POINT ( 'NONE',  ( -3.772649051595033498, 116.7207137014398626, 0.1335598970234345428 ) ) ;
#16058=CARTESIAN_POINT ( 'NONE',  ( -5.991689710969556160, 121.4334662389527466, -0.2049652515977599954 ) ) ;
#16060=CARTESIAN_POINT ( 'NONE',  ( 2.946371836444962256, 115.7030910448373788, -1.559712811386695819 ) ) ;
#16061=CARTESIAN_POINT ( 'NONE',  ( -10.32597032162043682, 126.0505730134521230, -0.3842079712423248639 ) ) ;
#16062=CARTESIAN_POINT ( 'NONE',  ( 3.036109343602874322, -15.28514977651167150, 5.695352409590039855 ) ) ;
#16063=CARTESIAN_POINT ( 'NONE',  ( -14.28818831795934230, 121.8555783441548073, 1.022170725131337665 ) ) ;
#16065=CARTESIAN_POINT ( 'NONE',  ( 18.58235751530886404, 154.1615476314759974, 0.6802042707109063890 ) ) ;
#16066=CARTESIAN_POINT ( 'NONE',  ( 14.67276854806925002, 148.8626603488974354, 0.4253145049176021986 ) ) ;
#16068=CARTESIAN_POINT ( 'NONE',  ( 0.3244192847266222923, 10.43846528477952340, -0.9201954171864650256 ) ) ;
#16069=CARTESIAN_POINT ( 'NONE',  ( -21.59686147024597247, 132.6646020023713959, -0.5653344646799387530 ) ) ;
#16072=CARTESIAN_POINT ( 'NONE',  ( 5.530566976517129696, 117.1577684187682564, 0.7355826452304826679 ) ) ;
#16075=CARTESIAN_POINT ( 'NONE',  ( 21.52700195390584526, 148.3057046726078170, 2.246165485461373290 ) ) ;
#16076=CARTESIAN_POINT ( 'NONE',  ( 2.589082543892768484, 158.1729697732556588, -1.607049804855985586 ) ) ;
#16077=CARTESIAN_POINT ( 'NONE',  ( -1.740095136297252543, 16.12223834230618635, -8.265420891812045312 ) ) ;
#16078=CARTESIAN_POINT ( 'NONE',  ( -3.006067730438063634, 117.5448765310053005, -0.7098943453401749260 ) ) ;
#16079=CARTESIAN_POINT ( 'NONE',  ( 4.827068429489758117, 117.7658018909618818, -0.8358721460697561279 ) ) ;
#16081=CARTESIAN_POINT ( 'NONE',  ( -12.88210196283061038, 133.7932622986943159, -0.2101989309002755546 ) ) ;
#16082=CARTESIAN_POINT ( 'NONE',  ( -18.01629081398026244, 149.0664087073519681, -2.421686302305671390 ) ) ;
#16083=CARTESIAN_POINT ( 'NONE',  ( 5.478045763647380717, -15.20773871853380044, 2.260320276039294640 ) ) ;
#16084=( BOUNDED_CURVE ( )  B_SPLINE_CURVE ( 3, ( #6881, #36278, #39684, #23671 ),
 .UNSPECIFIED., .F., .T. ) 
 B_SPLINE_CURVE_WITH_KNOTS ( ( 4, 4 ),
 ( 0.6486116422890977340, 0.6881516260757224446 ),
 .UNSPECIFIED. ) 
 CURVE ( )  GEOMETRIC_REPRESENTATION_ITEM ( )  RATIONAL_B_SPLINE_CURVE ( ( 0.5822367926346045941, 0.5608560245277020018, 0.5436443506017243354, 0.5306017708566714841 ) ) 
 REPRESENTATION_ITEM ( '' )  );
#16089=CARTESIAN_POINT ( 'NONE',  ( 0.5061634396315372042, 119.4440140289964774, 0.5640781084940280632 ) ) ;
#16090=CARTESIAN_POINT ( 'NONE',  ( -15.52687642492895037, 147.5330934759543879, -0.3102639428822864254 ) ) ;
#16092=CARTESIAN_POINT ( 'NONE',  ( -0.4402454045157814244, 106.4201689084969047, 5.104646014783341457 ) ) ;
#16093=CARTESIAN_POINT ( 'NONE',  ( -2.821688713678647709, 20.15627898171042176, -7.936949992814660071 ) ) ;
#16094=CARTESIAN_POINT ( 'NONE',  ( 1.656170893581987658, 156.3096136994911092, 0.5768031348127033997 ) ) ;
#16095=CARTESIAN_POINT ( 'NONE',  ( 22.08264656579475016, 150.6352520364973486, -0.6282006774575531471 ) ) ;
#16096=CARTESIAN_POINT ( 'NONE',  ( 3.682264917456192332, 91.02546620154572565, 0.07358041635424013294 ) ) ;
#16097=CARTESIAN_POINT ( 'NONE',  ( 6.485865538701863997, -14.69951297778787414, -0.2726410864842441772 ) ) ;
#16100=CARTESIAN_POINT ( 'NONE',  ( -6.896656464550618537, 117.1676486657671177, -0.1232935741316916883 ) ) ;
#16102=CARTESIAN_POINT ( 'NONE',  ( -6.449468943369818241, 120.2918880417729781, -1.168816612019687229 ) ) ;
#16105=CARTESIAN_POINT ( 'NONE',  ( -14.86280047924408798, 148.8756053271976327, -1.012714816113364558 ) ) ;
#16106=CARTESIAN_POINT ( 'NONE',  ( 4.273959209556542405, -12.80518358089995168, 2.504334382443756724 ) ) ;
#16108=CARTESIAN_POINT ( 'NONE',  ( 18.63504953328963154, 154.1157618415863624, 0.3723726386282266709 ) ) ;
#16110=CARTESIAN_POINT ( 'NONE',  ( -0.2084201458593382406, 5.265951782950084592, 4.622859108429906883 ) ) ;
#16111=CARTESIAN_POINT ( 'NONE',  ( -18.86374853661781970, 125.3403196291361610, -0.3769425889880998470 ) ) ;
#16112=CARTESIAN_POINT ( 'NONE',  ( -5.008987216415587973, 117.3966124399498199, 0.7756614673512686187 ) ) ;
#16116=CARTESIAN_POINT ( 'NONE',  ( 7.813248254659782788, 122.4491652087703670, 0.5620385025197442985 ) ) ;
#16117=CARTESIAN_POINT ( 'NONE',  ( 2.029292378383023898, 15.02103924000656043, -4.168288449772576065 ) ) ;
#16118=CARTESIAN_POINT ( 'NONE',  ( 1.978713825503164436, 117.0827246868714013, 0.4887249842031142766 ) ) ;
#16119=CARTESIAN_POINT ( 'NONE',  ( -0.06282972276541670675, 111.5577547982949227, 3.144256248693278355 ) ) ;
#16121=CARTESIAN_POINT ( 'NONE',  ( 13.94573646207659223, 122.0315337860429423, -1.127490061167130575 ) ) ;
#16122=CARTESIAN_POINT ( 'NONE',  ( 2.029292378383023898, 15.02103924000656043, -4.168288449772576065 ) ) ;
#16123=CARTESIAN_POINT ( 'NONE',  ( -14.85510260296675966, 121.0052616771249347, -1.128405194827190705 ) ) ;
#16124=ORIENTED_EDGE ( 'NONE', *, *, #32873, .F. ) ;
#16125=CARTESIAN_POINT ( 'NONE',  ( -9.317815699932426199, 124.0984330410602183, 0.1356161447201457426 ) ) ;
#16126=CARTESIAN_POINT ( 'NONE',  ( 4.669346286639404653, -14.72966438191931893, 4.552848284282712044 ) ) ;
#16128=CIRCLE ( 'NONE', #10702, 4.826000000000001400 ) ;
#16130=CARTESIAN_POINT ( 'NONE',  ( 19.42875987905491897, 141.0981142166620259, 2.503406319619450482 ) ) ;
#16131=CARTESIAN_POINT ( 'NONE',  ( -6.451606698686837575E-14, 65.62546620154573418, 4.217636114931141265E-29 ) ) ;
#16133=CARTESIAN_POINT ( 'NONE',  ( -14.88832262945836504, 121.0052616771249347, 0.5340607732653417372 ) ) ;
#16135=EDGE_CURVE ( 'NONE', #11942, #27588, #39698, .T. ) ;
#16138=CARTESIAN_POINT ( 'NONE',  ( 20.57623859521455856, 152.5775223076369400, -0.1637982859500252686 ) ) ;
#16144=CARTESIAN_POINT ( 'NONE',  ( -3.009276887026422820, 39.20946620154573736, 1.210121013456480377 ) ) ;
#16145=CARTESIAN_POINT ( 'NONE',  ( -4.665163707145283389, 118.0184243076322019, 0.6237975492375645858 ) ) ;
#16149=CARTESIAN_POINT ( 'NONE',  ( 8.429306250690459024, 119.6048990681906332, -1.079784194094564720 ) ) ;
#16150=CARTESIAN_POINT ( 'NONE',  ( -7.563243396832136867, 124.2956292408697863, -0.1602470646927416087 ) ) ;
#16151=CARTESIAN_POINT ( 'NONE',  ( 4.691553523908495116, 117.8976366721427098, 0.9736576180826594928 ) ) ;
#16152=CARTESIAN_POINT ( 'NONE',  ( 2.666490510518176649, -13.49855353256042712, 0.05227394649444803282 ) ) ;
#16153=CARTESIAN_POINT ( 'NONE',  ( -16.31317273256073719, 147.4903123243063590, -1.598834895054539018 ) ) ;
#16158=CARTESIAN_POINT ( 'NONE',  ( 6.920469006311881444, 121.8192184429722005, -0.01800753507563494088 ) ) ;
#16159=CARTESIAN_POINT ( 'NONE',  ( -16.52407570443684648, 148.2569838091642964, -1.909119861936069418 ) ) ;
#16161=CARTESIAN_POINT ( 'NONE',  ( -6.426369768295692736E-14, 159.6054662015457382, 1.032716915552223178E-16 ) ) ;
#16163=CARTESIAN_POINT ( 'NONE',  ( -4.637963820743935983, -6.603494994175692412, 0.1710436084038768345 ) ) ;
#16164=CARTESIAN_POINT ( 'NONE',  ( -0.008148259816616862383, 159.5682499516715040, 0.4077722408685187649 ) ) ;
#16166=CARTESIAN_POINT ( 'NONE',  ( 5.314256358595446983, 104.6144662015457527, -0.4585142901829573625 ) ) ;
#16167=CARTESIAN_POINT ( 'NONE',  ( 2.686089547800571964, -15.51909802064466248, 4.724564614977055044 ) ) ;
#16168=CARTESIAN_POINT ( 'NONE',  ( -19.29133405012203895, 147.6776069388173767, 1.737063910747457474 ) ) ;
#16169=CARTESIAN_POINT ( 'NONE',  ( 0.8777592251401162837, 3.590160258842859164, -0.4283581310676968790 ) ) ;
#16170=CARTESIAN_POINT ( 'NONE',  ( -3.254034125433686864, 159.4600617640778353, -0.3425454502237990639 ) ) ;
#16171=CARTESIAN_POINT ( 'NONE',  ( -0.02445332296907207215, 6.119348097484421878, 0.9755048060674135213 ) ) ;
#16173=ADVANCED_FACE ( 'NONE', ( #13795 ), #1929, .T. ) ;
#16177=CARTESIAN_POINT ( 'NONE',  ( 5.429077642219811928, 122.7706071131974994, 0.2216225483982832978 ) ) ;
#16179=CARTESIAN_POINT ( 'NONE',  ( -3.236331573563448583, 156.2293907256693331, 0.8668920366435202141 ) ) ;
#16180=CARTESIAN_POINT ( 'NONE',  ( 3.658150719587269784, -13.97641594243527408, 4.344832359604154703 ) ) ;
#16181=CARTESIAN_POINT ( 'NONE',  ( 13.85609184427558027, 152.5163154464351294, -1.589750347114883944 ) ) ;
#16182=CARTESIAN_POINT ( 'NONE',  ( -5.838901281334665683, 119.0696708348911699, -1.193623469369258894 ) ) ;
#16184=CARTESIAN_POINT ( 'NONE',  ( 2.350639260211558668, -15.10312717587823705, 4.966175652281853203 ) ) ;
#16185=CARTESIAN_POINT ( 'NONE',  ( -4.653079194867565604, 32.84790767926139665, 1.632299058096434496 ) ) ;
#16186=CARTESIAN_POINT ( 'NONE',  ( 4.553626923285095884, 121.1438296405421937, -0.06679122792761491012 ) ) ;
#16187=EDGE_LOOP ( 'NONE', ( #29961, #29669, #4722, #9999 ) ) ;
#16188=DIRECTION ( 'NONE',  ( -0.9998004120163609398, 0.000000000000000000, -0.01997839162482749689 ) ) ;
#16191=CARTESIAN_POINT ( 'NONE',  ( 5.036073817479851833, 117.3993844285031116, -0.5500234170841655779 ) ) ;
#16194=CARTESIAN_POINT ( 'NONE',  ( 1.817820247522382138, 116.4909138135563040, -0.03564457049243154735 ) ) ;
#16195=CARTESIAN_POINT ( 'NONE',  ( -0.1065646865916160396, 105.8844662015456777, 5.332932678536313809 ) ) ;
#16196=DIRECTION ( 'NONE',  ( -4.017660918040594346E-17, 1.000000000000000000, 2.376309959284834438E-19 ) ) ;
#16198=CARTESIAN_POINT ( 'NONE',  ( -4.843427198813659018, 31.50844634454021786, -0.7061668956633826433 ) ) ;
#16200=CARTESIAN_POINT ( 'NONE',  ( 18.56731909478072851, 131.8045874826418071, 2.147352672676718033 ) ) ;
#16201=CARTESIAN_POINT ( 'NONE',  ( 2.233585966345281282, 24.54162662436292308, -4.064490141941544898 ) ) ;
#16202=CARTESIAN_POINT ( 'NONE',  ( 8.391146056172745560, -15.30543149186461527, -0.4349570568239987667 ) ) ;
#16203=CARTESIAN_POINT ( 'NONE',  ( 5.510923006218381381, 117.2511638274202994, -0.6088136109206577773 ) ) ;
#16204=CARTESIAN_POINT ( 'NONE',  ( -0.5374927741466587472, 112.6282971158091470, -2.756357034314327326 ) ) ;
#16205=CARTESIAN_POINT ( 'NONE',  ( -22.53527615164659892, 150.7831677823004952, -0.4503084484864786075 ) ) ;
#16208=CARTESIAN_POINT ( 'NONE',  ( -0.9365507687766482237, 105.1228617213538570, 5.262462312604806236 ) ) ;
#16209=CARTESIAN_POINT ( 'NONE',  ( -2.029258473809828711, 23.83235028914373288, 4.157303687431403993 ) ) ;
#16211=CARTESIAN_POINT ( 'NONE',  ( -20.51686376604223128, 129.1072961674477710, -0.4099757654675940111 ) ) ;
#16212=CARTESIAN_POINT ( 'NONE',  ( 2.995043271588619493, -14.66878921821561299, 4.005342282345994320 ) ) ;
#16213=CARTESIAN_POINT ( 'NONE',  ( 2.226623034866197948, 116.5145642697238344, -1.365476420808193536 ) ) ;
#16214=CARTESIAN_POINT ( 'NONE',  ( -22.83860824214441720, 149.7823008822066697, 0.3949144739309159990 ) ) ;
#16218=EDGE_LOOP ( 'NONE', ( #10174, #38571, #39986, #38456 ) ) ;
#16220=CARTESIAN_POINT ( 'NONE',  ( 3.900291174488768053, -15.73247852219369847, 4.461464635514134969 ) ) ;
#16221=CARTESIAN_POINT ( 'NONE',  ( -0.4495176323323362699, 118.2558431149878402, 0.5768950177939178303 ) ) ;
#16222=CARTESIAN_POINT ( 'NONE',  ( 14.19262213114343929, 155.9232964860746620, -1.164639009528572799 ) ) ;
#16223=CARTESIAN_POINT ( 'NONE',  ( -0.5496829067194369811, 0.7180641350488168317, -4.598301960397928489 ) ) ;
#16226=CARTESIAN_POINT ( 'NONE',  ( 3.174366308151880922, 88.99346620154574339, 0.06343139340882768262 ) ) ;
#16227=CARTESIAN_POINT ( 'NONE',  ( -0.02135216056683805069, 118.1497763966934258, 1.068549427312529776 ) ) ;
#16229=CARTESIAN_POINT ( 'NONE',  ( -10.96277846527069322, 123.4376579628654014, 1.079141073574104492 ) ) ;
#16230=DIRECTION ( 'NONE',  ( -0.9998004120163609398, 0.000000000000000000, -0.01997839162482749689 ) ) ;
#16232=AXIS2_PLACEMENT_3D ( 'NONE', #13914, #26907, #7125 ) ;
#16233=CARTESIAN_POINT ( 'NONE',  ( 17.15907173562165156, 135.3907879583883869, -1.705144375702607240 ) ) ;
#16234=CARTESIAN_POINT ( 'NONE',  ( -11.58753624721098774, 156.3395478113760362, -2.047021040405474945 ) ) ;
#16238=CARTESIAN_POINT ( 'NONE',  ( 4.496748124183634232, 118.1159772194654352, -0.5629342433147717095 ) ) ;
#16239=CARTESIAN_POINT ( 'NONE',  ( 5.220694793870399586, 121.0999079655412203, -0.2922795305089893048 ) ) ;
#16241=CARTESIAN_POINT ( 'NONE',  ( -16.68865417205013912, 140.0893442862094673, -2.224985475129671375 ) ) ;
#16242=CARTESIAN_POINT ( 'NONE',  ( 3.885490704569380060, -15.31119228946847777, 1.341400144935093630 ) ) ;
#16243=CARTESIAN_POINT ( 'NONE',  ( -1.502787496059203809, 105.1237720616447007, -5.127625393460141900 ) ) ;
#16246=CARTESIAN_POINT ( 'NONE',  ( -4.930297673862535923, 117.6593853309075115, 0.7657671191340518213 ) ) ;
#16247=CARTESIAN_POINT ( 'NONE',  ( 17.14723838084580976, 144.2986879860016529, 2.167616513504174947 ) ) ;
#16249=CARTESIAN_POINT ( 'NONE',  ( -4.247245584637960647, 22.75789413176893206, 1.861891798430825862 ) ) ;
#16250=CARTESIAN_POINT ( 'NONE',  ( -0.002459394113082844901, 156.3065584682211124, 0.1230781383047674232 ) ) ;
#16251=CARTESIAN_POINT ( 'NONE',  ( 4.801216665947148243, 117.4032681888235459, -1.015537427445656782 ) ) ;
#16252=AXIS2_PLACEMENT_3D ( 'NONE', #40307, #27706, #11725 ) ;
#16256=CARTESIAN_POINT ( 'NONE',  ( 5.564921306486510844, 116.7072773883409837, -0.001268244569501262957 ) ) ;
#16257=CARTESIAN_POINT ( 'NONE',  ( 20.69909148798437926, 152.5508394022677692, 0.4136171090298765285 ) ) ;
#16259=DIRECTION ( 'NONE',  ( 0.9998004120163608288, 4.016384292689131511E-17, 0.01997839162482749342 ) ) ;
#16260=CARTESIAN_POINT ( 'NONE',  ( -8.158575919685375766, 120.6841143662035734, -1.398758167514821515 ) ) ;
#16262=DIRECTION ( 'NONE',  ( -5.206863593109713661E-17, 1.000000000000000000, -1.077750396879097183E-30 ) ) ;
#16266=CARTESIAN_POINT ( 'NONE',  ( -23.25537431167569835, 149.3282167461061931, -0.1335628131362693594 ) ) ;
#16267=EDGE_CURVE ( 'NONE', #15693, #24363, #39013, .T. ) ;
#16268=ORIENTED_EDGE ( 'NONE', *, *, #24786, .F. ) ;
#16270=CARTESIAN_POINT ( 'NONE',  ( -7.790237900701975526, 122.5851110379722257, -0.3184765188668609581 ) ) ;
#16273=CARTESIAN_POINT ( 'NONE',  ( -15.39298062464846240, 147.8297367799732456, -0.5361660792469025161 ) ) ;
#16274=CARTESIAN_POINT ( 'NONE',  ( 3.968318174290614397, -14.81366206205479763, 5.151173006574525814 ) ) ;
#16275=CARTESIAN_POINT ( 'NONE',  ( -19.13467844095171344, 131.8899703912256314, 1.275959715510669001 ) ) ;
#16277=CARTESIAN_POINT ( 'NONE',  ( 20.67395311655588941, 152.5754960671270055, 0.6363119977773277203 ) ) ;
#16278=CARTESIAN_POINT ( 'NONE',  ( 15.75762098209218465, 145.9019271191307610, 0.4493305750801200316 ) ) ;
#16280=CARTESIAN_POINT ( 'NONE',  ( 0.7678286665867425365, 17.13787758575863762, 0.6011479000593502597 ) ) ;
#16281=CARTESIAN_POINT ( 'NONE',  ( -11.68195978820582326, 118.7263634577040676, -0.3785536984881909262 ) ) ;
#16282=B_SPLINE_CURVE_WITH_KNOTS ( 'NONE', 1,
 ( #18232, #31234 ),
 .UNSPECIFIED., .F., .F.,
 ( 2, 2 ),
 ( 0.04444444444444391878, 0.9701209927381800879 ),
 .UNSPECIFIED. ) ;
#16285=ORIENTED_EDGE ( 'NONE', *, *, #23204, .F. ) ;
#16286=CARTESIAN_POINT ( 'NONE',  ( 5.604777855449654567, 117.7098723955010513, 0.9801559107764311607 ) ) ;
#16288=CARTESIAN_POINT ( 'NONE',  ( 5.078986093043053707, 85.69146620154573668, 0.1014902294541244060 ) ) ;
#16289=CARTESIAN_POINT ( 'NONE',  ( 2.895878334088767492, 159.0164033662945258, 1.329837440140976268 ) ) ;
#16290=CARTESIAN_POINT ( 'NONE',  ( 12.76794581240257287, 122.4237789811383550, -1.308419224297318051 ) ) ;
#16291=CARTESIAN_POINT ( 'NONE',  ( -0.7381358996182917354, 6.602865006980263018, -0.6401951644792284180 ) ) ;
#16292=CARTESIAN_POINT ( 'NONE',  ( -7.817010796087602742, 17.61996943312679775, -3.135079784279759085 ) ) ;
#16293=CARTESIAN_POINT ( 'NONE',  ( -19.25714749039855889, 152.1947311750261065, -2.059892502987373142 ) ) ;
#16294=CARTESIAN_POINT ( 'NONE',  ( 4.756981263701162810, 117.8474050189492459, -0.8188388414369660584 ) ) ;
#16296=CARTESIAN_POINT ( 'NONE',  ( 5.345964095105256497, 116.9256180743815179, 0.9586058045032991304 ) ) ;
#16299=CARTESIAN_POINT ( 'NONE',  ( 17.00728043862065419, 146.2370505443881257, -1.250989154318494334 ) ) ;
#16300=CARTESIAN_POINT ( 'NONE',  ( -15.38068278028571712, 147.8292851303062321, -0.2562860988859086975 ) ) ;
#16302=CARTESIAN_POINT ( 'NONE',  ( -5.834721624102832571, 119.7498067647950961, -1.158144809029191702 ) ) ;
#16304=CARTESIAN_POINT ( 'NONE',  ( 2.079639979227050350, -15.65372482070806548, 5.795360105834356013 ) ) ;
#16305=CARTESIAN_POINT ( 'NONE',  ( 4.770534990627869121, 118.5931160184169073, 0.9880304185510659920 ) ) ;
#16308=CARTESIAN_POINT ( 'NONE',  ( -0.03066982525788402442, 157.3074135339440147, 1.534843470138540500 ) ) ;
#16310=FACE_OUTER_BOUND ( 'NONE', #19438, .T. ) ;
#16311=CARTESIAN_POINT ( 'NONE',  ( -4.257294657327928000, 122.9893884486272526, 0.03029934543357451493 ) ) ;
#16312=CARTESIAN_POINT ( 'NONE',  ( 5.644239659282993316, 25.55377913558855596, 6.252972086369320337 ) ) ;
#16313=CARTESIAN_POINT ( 'NONE',  ( -0.003756957834558761079, 120.7746249494737896, 0.1880135328902411695 ) ) ;
#16314=CARTESIAN_POINT ( 'NONE',  ( 13.14342457437316192, 119.8381915656929380, -0.4562891928474252512 ) ) ;
#16316=DIRECTION ( 'NONE',  ( -0.9998004120163608288, 0.000000000000000000, -0.01997839162482749342 ) ) ;
#16318=CARTESIAN_POINT ( 'NONE',  ( -13.69580498508147137, 119.6466660129326272, -0.2573648061928515696 ) ) ;
#16320=CARTESIAN_POINT ( 'NONE',  ( -6.315404033698660768, 119.9964383445381344, -1.210168696518489462 ) ) ;
#16321=DIRECTION ( 'NONE',  ( -0.01997839162482749342, -1.040247600000944484E-18, 0.9998004120163608288 ) ) ;
#16322=CARTESIAN_POINT ( 'NONE',  ( -1.557716402914305798, 120.7946061759640486, -0.2396963980366530189 ) ) ;
#16323=CARTESIAN_POINT ( 'NONE',  ( 3.244298476066852732, -14.49340328532226785, 5.143112664727522265 ) ) ;
#16324=CARTESIAN_POINT ( 'NONE',  ( -5.152838217380527830, 116.8470107115679468, -0.02676777192457512403 ) ) ;
#16325=CARTESIAN_POINT ( 'NONE',  ( 21.90559427349690935, 151.4293160993575498, 0.4377259060014666026 ) ) ;
#16327=CARTESIAN_POINT ( 'NONE',  ( -3.998286381996895233, 3.741657206818807424, 2.332027183294827832 ) ) ;
#16328=CARTESIAN_POINT ( 'NONE',  ( -0.8838529761741459323, 116.4325158421065680, -0.01766148591713726304 ) ) ;
#16329=CARTESIAN_POINT ( 'NONE',  ( -4.999701296913731774, 117.4056873544018487, 0.8305309289140377915 ) ) ;
#16331=CARTESIAN_POINT ( 'NONE',  ( 6.946787401000980466, 121.0168171694836019, 1.036538389785776282 ) ) ;
#16332=( BOUNDED_SURFACE ( )  B_SPLINE_SURFACE ( 3, 2, ( 
 ( #21394, #1843, #8644 ),
 ( #24396, #41453, #5680 ),
 ( #11618, #31209, #2692 ),
 ( #31853, #5254, #37610 ) ),
 .UNSPECIFIED., .F., .F., .T. ) 
 B_SPLINE_SURFACE_WITH_KNOTS ( ( 4, 4 ),
 ( 3, 3 ),
 ( 0.001248090998549182236, 0.001439255081647348349 ),
 ( 0.000000000000000000, 0.2830925978542064847 ),
 .UNSPECIFIED. ) 
 GEOMETRIC_REPRESENTATION_ITEM ( )  RATIONAL_B_SPLINE_SURFACE ( (
 ( 1.000000000000000000, 0.9321727843773290889, 0.9027483341063369249),
 ( 1.000000000000000000, 0.9321727478157031399, 0.9027482816837362201),
 ( 1.000000000000000000, 0.9321727022987384981, 0.9027482164208384674),
 ( 1.000000000000000000, 0.9321727023713098914, 0.9027482165248924550) ) ) 
 REPRESENTATION_ITEM ( '' )  SURFACE ( )  );
#16333=CARTESIAN_POINT ( 'NONE',  ( -4.255528399684056495, 7.899375212487111497, -1.818898740287305138 ) ) ;
#16334=CARTESIAN_POINT ( 'NONE',  ( 1.323305960456815811, 159.4649289425152858, 0.7771481453362867331 ) ) ;
#16337=CARTESIAN_POINT ( 'NONE',  ( 20.59592450876350966, 149.8464234248869786, -1.516103928358539354 ) ) ;
#16338=CARTESIAN_POINT ( 'NONE',  ( -4.609865753310859127, 8.349128549105346409, -0.5081561704775721111 ) ) ;
#16339=CARTESIAN_POINT ( 'NONE',  ( -16.28621419528974101, 155.1963085991477271, -1.407434501154738449 ) ) ;
#16340=AXIS2_PLACEMENT_3D ( 'NONE', #34071, #30435, #8279 ) ;
#16342=CARTESIAN_POINT ( 'NONE',  ( -15.85793921209448243, 146.6055793175013093, 0.1365194753024331908 ) ) ;
#16343=CARTESIAN_POINT ( 'NONE',  ( 5.816378023188423896, -13.23522671163289388, 2.128111738716565338 ) ) ;
#16346=CARTESIAN_POINT ( 'NONE',  ( -1.770057497934276691, 106.3924174363319821, -5.031961110743496057 ) ) ;
#16348=CARTESIAN_POINT ( 'NONE',  ( 2.398927117898916883, 157.8629595415303584, 1.727538386417435401 ) ) ;
#16350=FACE_OUTER_BOUND ( 'NONE', #4384, .T. ) ;
#16351=CARTESIAN_POINT ( 'NONE',  ( -3.877771370679356622, 117.0975898859979054, 0.4181078409183316413 ) ) ;
#16353=CARTESIAN_POINT ( 'NONE',  ( 2.823947636868042288, 116.6946238705719594, -0.1909394059425170709 ) ) ;
#16356=CARTESIAN_POINT ( 'NONE',  ( -3.456281358658260583, 50.63946620154572997, -1.847419665314800508 ) ) ;
#16361=CARTESIAN_POINT ( 'NONE',  ( -4.592204290372686515, 118.0393302332859378, 0.6628552400479452711 ) ) ;
#16363=PRODUCT_DEFINITION_SHAPE ( 'NONE', 'NONE',  #37297 ) ;
#16365=CARTESIAN_POINT ( 'NONE',  ( -0.07233785497491922178, 118.7629491485454025, -1.278895185737845441 ) ) ;
#16366=CARTESIAN_POINT ( 'NONE',  ( -3.439708463638626590, 118.6150900816448797, -0.9303604156532724323 ) ) ;
#16367=CARTESIAN_POINT ( 'NONE',  ( -7.089375086750039578, 122.4291926079955317, -0.2513136963589432393 ) ) ;
#16369=CARTESIAN_POINT ( 'NONE',  ( 4.694918129094446613, 117.9582486484168982, 0.8614738248342319604 ) ) ;
#16371=CARTESIAN_POINT ( 'NONE',  ( -9.985636026282492139, 124.1433363813624311, -1.001463123883985729 ) ) ;
#16372=CARTESIAN_POINT ( 'NONE',  ( -3.627500158948379294, 115.7029588711417887, -1.619953353561904619 ) ) ;
#16375=CARTESIAN_POINT ( 'NONE',  ( 0.1065646865914870178, 105.8844662015456919, -5.332932678536313809 ) ) ;
#16376=CARTESIAN_POINT ( 'NONE',  ( 0.02400040557466870741, 156.7459281804771365, -1.201078436782489378 ) ) ;
#16378=CARTESIAN_POINT ( 'NONE',  ( -0.0008202526018428905668, 159.6052337359418800, 0.04104879434819971862 ) ) ;
#16379=CARTESIAN_POINT ( 'NONE',  ( -2.969549164036747957, 115.7030431952828735, 1.557416231888924196 ) ) ;
#16380=CARTESIAN_POINT ( 'NONE',  ( -1.560048624214163793, 156.2601855860432067, 0.007372770612580329189 ) ) ;
#16381=CARTESIAN_POINT ( 'NONE',  ( 1.398650104629075797, 0.06838872207683838189, -4.420329592304430122 ) ) ;
#16382=CARTESIAN_POINT ( 'NONE',  ( 22.91074218474003032, 142.4877946823990271, 1.320775467724695007 ) ) ;
#16385=CARTESIAN_POINT ( 'NONE',  ( 3.506097670019660217, -15.11506922876175452, 2.387495833752258267 ) ) ;
#16386=CARTESIAN_POINT ( 'NONE',  ( -13.98553986197822852, 125.7699432187419575, 1.444593012458400105 ) ) ;
#16387=CARTESIAN_POINT ( 'NONE',  ( 0.1179719058304127544, 10.27755972103446958, 0.9685762618712100425 ) ) ;
#16388=CARTESIAN_POINT ( 'NONE',  ( -13.35680032055093847, 119.7032035076741465, -0.7543780172957895713 ) ) ;
#16389=CARTESIAN_POINT ( 'NONE',  ( 0.9616503885695291132, 8.288457568681202758, 0.1719041247055087540 ) ) ;
#16393=CARTESIAN_POINT ( 'NONE',  ( 5.194452014863536249, 116.1170857923940787, 1.235891685093609915 ) ) ;
#16394=CARTESIAN_POINT ( 'NONE',  ( -10.90887028606303666, 153.1125297277760069, 0.8016274872379889338 ) ) ;
#16395=CARTESIAN_POINT ( 'NONE',  ( 3.097180478269691672, -14.43375334869456594, 4.992610980676636778 ) ) ;
#16396=CARTESIAN_POINT ( 'NONE',  ( 17.22187362939829214, 148.7218176724978775, -1.531815132551777037 ) ) ;
#16397=CARTESIAN_POINT ( 'NONE',  ( -19.60096582671588550, 145.2539617268756729, -2.527680105953240552 ) ) ;
#16398=CARTESIAN_POINT ( 'NONE',  ( 2.958531772299236362, 39.20946620154573736, 1.329372033065076231 ) ) ;
#16400=CARTESIAN_POINT ( 'NONE',  ( 2.768561164044480272, -13.57843041371762460, 0.3119852368007841603 ) ) ;
#16401=CARTESIAN_POINT ( 'NONE',  ( -0.5321123018419734452, 37.22158963861809156, -0.7300149017649122385 ) ) ;
#16402=CARTESIAN_POINT ( 'NONE',  ( 5.269990328701441129, 121.3020066425206807, -0.06069006697729611988 ) ) ;
#16406=AXIS2_PLACEMENT_3D ( 'NONE', #27836, #5486, #38278 ) ;
#16409=CARTESIAN_POINT ( 'NONE',  ( 13.42085051059965828, 156.9389434127184018, 0.1400394208249338968 ) ) ;
#16410=CARTESIAN_POINT ( 'NONE',  ( -6.130181428581336966, 119.5149100643186983, 0.2724793030934819504 ) ) ;
#16412=CARTESIAN_POINT ( 'NONE',  ( -1.447287616209143035, 115.6909491485452435, 1.681827335203893936 ) ) ;
#16413=CARTESIAN_POINT ( 'NONE',  ( 4.560362914109654220, -11.68884639558073069, 0.6953251057713033534 ) ) ;
#16414=CARTESIAN_POINT ( 'NONE',  ( -3.514327769487986419, 32.73121309073282958, 1.058241958670834704 ) ) ;
#16415=CARTESIAN_POINT ( 'NONE',  ( 13.26090510203103179, 121.6721647909590303, 1.681263517196597945 ) ) ;
#16416=CARTESIAN_POINT ( 'NONE',  ( 3.912982837994093188, 14.17146771520798332, -2.459658384584827218 ) ) ;
#16417=CARTESIAN_POINT ( 'NONE',  ( 8.129739676946041271, 26.40327925692461619, 2.337594602388961107 ) ) ;
#16418=CARTESIAN_POINT ( 'NONE',  ( -8.686247397591175812, 118.1594658427179780, -0.8950587481708219828 ) ) ;
#16419=CARTESIAN_POINT ( 'NONE',  ( -0.4574053846283027691, 111.1955024190080223, -3.269098021338873838 ) ) ;
#16422=CARTESIAN_POINT ( 'NONE',  ( 0.1701459486970862411, 105.9762159740997305, -5.294439841319366735 ) ) ;
#16423=CARTESIAN_POINT ( 'NONE',  ( -0.2157595709654898941, 104.6144662015456390, 4.831689808425918109 ) ) ;
#16424=AXIS2_PLACEMENT_3D ( 'NONE', #1678, #40647, #37434 ) ;
#16425=CARTESIAN_POINT ( 'NONE',  ( 3.465721614298269415, 18.43485028915299750, -3.064284189100199729 ) ) ;
#16428=CARTESIAN_POINT ( 'NONE',  ( 3.026662605148213725, -13.87242449132548217, 1.205013440933411228 ) ) ;
#16429=CARTESIAN_POINT ( 'NONE',  ( 2.328636301501455286, 124.8000875644994068, 0.03907356579384867884 ) ) ;
#16430=CARTESIAN_POINT ( 'NONE',  ( -21.01068656986065974, 132.3427885975763161, 0.3612206858233398821 ) ) ;
#16431=ORIENTED_EDGE ( 'NONE', *, *, #25895, .T. ) ;
#16432=CARTESIAN_POINT ( 'NONE',  ( 15.47023807670824525, 120.6682698389898576, 0.3091321738930620788 ) ) ;
#16433=VERTEX_POINT ( 'NONE', #3078 ) ;
#16434=CARTESIAN_POINT ( 'NONE',  ( -4.965295013367585497, 115.7029491485453576, 1.257100568209378988 ) ) ;
#16435=CARTESIAN_POINT ( 'NONE',  ( 5.949011718796170634, -14.81501284647598915, 0.9937821824230966827 ) ) ;
#16436=CARTESIAN_POINT ( 'NONE',  ( -12.82775609536344774, 122.1393999080170971, 1.276540306405074876 ) ) ;
#16437=CARTESIAN_POINT ( 'NONE',  ( 1.113991634874381020, 117.6437429425539420, -0.5281592773360502813 ) ) ;
#16438=CARTESIAN_POINT ( 'NONE',  ( -4.550674770548566173, 2.667180226961371137, -0.8080508602523945871 ) ) ;
#16443=CARTESIAN_POINT ( 'NONE',  ( 0.3557992751141359489, 119.2343925067223722, 0.8259638274389489165 ) ) ;
#16444=DIRECTION ( 'NONE',  ( -0.0004113621476973288913, 0.9999999153568039922, -8.219994698375953989E-06 ) ) ;
#16445=CARTESIAN_POINT ( 'NONE',  ( -10.67172107669508208, 123.8807653058400575, 0.9292482510779809246 ) ) ;
#16447=CARTESIAN_POINT ( 'NONE',  ( 12.44264023681980902, 124.1810962131942517, -1.301390444852660755 ) ) ;
#16448=CARTESIAN_POINT ( 'NONE',  ( -13.39049918543330975, 121.7711344121973411, -1.690880791723282428 ) ) ;
#16451=CARTESIAN_POINT ( 'NONE',  ( 4.552138684229567467, 118.1085559717327129, -0.4997336699443528651 ) ) ;
#16453=CARTESIAN_POINT ( 'NONE',  ( 15.82779737147842880, 147.6293441119438512, -0.5318544519934516046 ) ) ;
#16455=CARTESIAN_POINT ( 'NONE',  ( -14.65736332902334027, 131.2156652454908112, -2.020252246219832237 ) ) ;
#16456=CARTESIAN_POINT ( 'NONE',  ( 3.794293369880153310, -15.39696243832143452, 2.404174946430260196 ) ) ;
#16457=DIRECTION ( 'NONE',  ( -0.9998004120163609398, 0.000000000000000000, -0.01997839162482749689 ) ) ;
#16460=CARTESIAN_POINT ( 'NONE',  ( -4.858599712106120627, 117.6759678160989040, 0.8825250931707183666 ) ) ;
#16461=CARTESIAN_POINT ( 'NONE',  ( 5.258743330460715626, 156.4258374981641282, 1.697662213785431140 ) ) ;
#16462=CARTESIAN_POINT ( 'NONE',  ( -2.937855498725889802, 30.67129419150591829, -0.3884002086831440104 ) ) ;
#16463=CARTESIAN_POINT ( 'NONE',  ( -3.130497002865707312, 23.39511390029671745, 3.426874451367011520 ) ) ;
#16464=CARTESIAN_POINT ( 'NONE',  ( 9.132214679254509804, 153.9061766533773152, 0.3822102345680644109 ) ) ;
#16470=ORIENTED_EDGE ( 'NONE', *, *, #20593, .T. ) ;
#16471=DIRECTION ( 'NONE',  ( -4.017660918040594346E-17, 1.000000000000000000, 2.376309959284834438E-19 ) ) ;
#16474=FACE_BOUND ( 'NONE', #36335, .T. ) ;
#16475=CARTESIAN_POINT ( 'NONE',  ( -8.267082973024169945, 120.1495290627620847, -1.449466298147102483 ) ) ;
#16476=EDGE_CURVE ( 'NONE', #17174, #15268, #29497, .T. ) ;
#16478=CARTESIAN_POINT ( 'NONE',  ( -3.682264917456324227, 95.34346620154573770, -0.07358041635423923088 ) ) ;
#16481=CARTESIAN_POINT ( 'NONE',  ( -16.13169674176122115, 121.3783152868344075, -0.08747489889995958834 ) ) ;
#16484=CARTESIAN_POINT ( 'NONE',  ( -7.789231022850876762, 122.5917277006084447, -0.3009637317056043093 ) ) ;
#16485=ORIENTED_EDGE ( 'NONE', *, *, #19413, .T. ) ;
#16487=CARTESIAN_POINT ( 'NONE',  ( -9.075584820321632051, 124.0722828908287454, -0.2154388746608566219 ) ) ;
#16488=CARTESIAN_POINT ( 'NONE',  ( 6.168037961413951997, -13.40247527924742776, 1.492370457280242091 ) ) ;
#16489=CARTESIAN_POINT ( 'NONE',  ( -0.02768730785358111679, 158.9256195073445213, 1.385586103196075891 ) ) ;
#16492=CARTESIAN_POINT ( 'NONE',  ( 15.30459713313458892, 120.6995131204970875, 0.6235550965980859450 ) ) ;
#16494=CARTESIAN_POINT ( 'NONE',  ( 4.831639344160726601, 118.5266822147775940, -0.7488923974486405566 ) ) ;
#16495=CARTESIAN_POINT ( 'NONE',  ( -0.7366970693195243891, 2.667464547469879488, -0.6395729927624468347 ) ) ;
#16496=CARTESIAN_POINT ( 'NONE',  ( -1.414297571701438105, 159.6040221172770259, -0.1149235736256734586 ) ) ;
#16497=FACE_OUTER_BOUND ( 'NONE', #10824, .T. ) ;
#16499=VERTEX_POINT ( 'NONE', #32880 ) ;
#16500=CARTESIAN_POINT ( 'NONE',  ( 8.699452012065234996, 118.0993342392008714, 0.8513243511965803423 ) ) ;
#16502=CARTESIAN_POINT ( 'NONE',  ( -18.41704236485563584, 146.8095856830544790, 1.664602135862215615 ) ) ;
#16504=CARTESIAN_POINT ( 'NONE',  ( 10.62690833282000469, 119.8050749133877275, 1.415659332795228265 ) ) ;
#16505=CARTESIAN_POINT ( 'NONE',  ( 20.10795522872006913, 148.3334041379468715, -1.700709099906817512 ) ) ;
#16506=CARTESIAN_POINT ( 'NONE',  ( -0.09096679801628397566, 0.3556511065658448656, 0.9697834404811940257 ) ) ;
#16507=CARTESIAN_POINT ( 'NONE',  ( -21.06903215802097051, 150.2702755442954583, -2.120733010085479986 ) ) ;
#16508=CARTESIAN_POINT ( 'NONE',  ( 4.750401733383816882, 117.8973045592046986, -0.7610669662629643284 ) ) ;
#16509=CARTESIAN_POINT ( 'NONE',  ( 5.608813212978028595, 117.9149360781225937, 0.7492264055198125661 ) ) ;
#16511=CARTESIAN_POINT ( 'NONE',  ( 10.28583081752390349, 123.7737839053064022, -0.8195368008302434948 ) ) ;
#16512=CARTESIAN_POINT ( 'NONE',  ( -15.72486432277162649, 146.8976350983841144, -0.2628874744899974969 ) ) ;
#16513=ORIENTED_EDGE ( 'NONE', *, *, #15211, .F. ) ;
#16514=CARTESIAN_POINT ( 'NONE',  ( -0.4972808831008551644, 119.3183582894065893, -0.5800711753708561735 ) ) ;
#16515=CARTESIAN_POINT ( 'NONE',  ( 3.432040476525267891, -15.74971700692714904, 4.939269227581224442 ) ) ;
#16518=ORIENTED_EDGE ( 'NONE', *, *, #40126, .F. ) ;
#16519=CARTESIAN_POINT ( 'NONE',  ( 1.321503922127525765, 119.3298839580929638, 0.6528639922554047015 ) ) ;
#16520=DIRECTION ( 'NONE',  ( 0.01997839162482749689, 1.040247600000945640E-18, -0.9998004120163610509 ) ) ;
#16524=CARTESIAN_POINT ( 'NONE',  ( -2.458941639547564506, 111.1666841684333633, 3.140650435616773706 ) ) ;
#16525=CARTESIAN_POINT ( 'NONE',  ( 8.129739676946041271, 26.40327925692461619, 2.337594602388961107 ) ) ;
#16526=CARTESIAN_POINT ( 'NONE',  ( 2.749413646642089759, 120.8469057251343060, 0.2833394764088550399 ) ) ;
#16527=CARTESIAN_POINT ( 'NONE',  ( 16.42246607841793704, 155.2191194103077407, -0.6571739840263305377 ) ) ;
#16528=CARTESIAN_POINT ( 'NONE',  ( 4.708802384804349650, 117.9017870880961851, 0.9536527796915015287 ) ) ;
#16529=DIRECTION ( 'NONE',  ( -0.9998004120163610509, -4.016384292689131511E-17, -0.01997839162482749689 ) ) ;
#16530=CIRCLE ( 'NONE', #15829, 5.080000000000006288 ) ;
#16532=CARTESIAN_POINT ( 'NONE',  ( -3.715898061425088716, 116.6275173757784813, -0.03328880940299687452 ) ) ;
#16534=CARTESIAN_POINT ( 'NONE',  ( -7.937677187970164638, 121.7945880220786563, -1.052464246659149394 ) ) ;
#16535=CARTESIAN_POINT ( 'NONE',  ( 5.611662049521669360, -14.50861037526213160, 3.104497901075802702 ) ) ;
#16536=CARTESIAN_POINT ( 'NONE',  ( -5.232823448427346591, 121.2166884500396833, -0.3893023073710018545 ) ) ;
#16537=CARTESIAN_POINT ( 'NONE',  ( 3.526842715273949214, -14.30601272375732513, 4.884018970202873788 ) ) ;
#16539=CARTESIAN_POINT ( 'NONE',  ( -13.85601021432062652, 120.6843904051541898, 0.7167389240433507114 ) ) ;
#16541=CARTESIAN_POINT ( 'NONE',  ( 18.81533481972603283, 125.3161215262879580, 0.4318114027375014596 ) ) ;
#16543=CARTESIAN_POINT ( 'NONE',  ( 4.523211737919912601, 7.414965188139293950, 0.9565071382433593117 ) ) ;
#16544=CARTESIAN_POINT ( 'NONE',  ( -4.434004255332462563, 105.1217594994107003, 2.985252168657458238 ) ) ;
#16547=CARTESIAN_POINT ( 'NONE',  ( 8.005068693524716394, 121.4516396534798162, 1.199299645920925972 ) ) ;
#16548=CARTESIAN_POINT ( 'NONE',  ( -1.441504266290200897, 6.599927940091079748, -4.410093354674724964 ) ) ;
#16549=CARTESIAN_POINT ( 'NONE',  ( 21.78097984573138390, 150.5404744109896171, 1.730106343981699268 ) ) ;
#16551=CARTESIAN_POINT ( 'NONE',  ( -3.682264917456323339, 71.97546620154574271, -0.07358041635423968885 ) ) ;
#16552=CARTESIAN_POINT ( 'NONE',  ( 0.02874440110933674380, 158.8294072187990196, -1.438487372358303373 ) ) ;
#16554=CARTESIAN_POINT ( 'NONE',  ( -0.5507456681092424144, 15.89564879194059799, -4.587442282481805300 ) ) ;
#16555=CARTESIAN_POINT ( 'NONE',  ( -22.65971377182568602, 149.0844379882532849, -1.633711759839209243 ) ) ;
#16558=CARTESIAN_POINT ( 'NONE',  ( -2.954508604762049462, 156.0884104482065595, 0.2429312420959233720 ) ) ;
#16559=CARTESIAN_POINT ( 'NONE',  ( 5.673832624563095450, -13.47712647082498272, 2.605829897212420754 ) ) ;
#16560=CARTESIAN_POINT ( 'NONE',  ( -4.580899860306842264, 27.87760619330545708, 0.5121266511161914892 ) ) ;
#16562=CARTESIAN_POINT ( 'NONE',  ( -0.1714850630699969736, 105.9761014636842731, -5.301312858626547886 ) ) ;
#16563=ORIENTED_EDGE ( 'NONE', *, *, #33879, .T. ) ;
#16564=CARTESIAN_POINT ( 'NONE',  ( 17.37713502592712445, 151.5007859583534753, 2.430116715062250687 ) ) ;
#16566=CARTESIAN_POINT ( 'NONE',  ( -6.758592445694407663E-14, 130.0144662015457300, 5.650815781856659706E-18 ) ) ;
#16567=CARTESIAN_POINT ( 'NONE',  ( -1.973526102370684487, 116.9869758084673208, 0.3704244399607084515 ) ) ;
#16568=CARTESIAN_POINT ( 'NONE',  ( -5.424866478234207534, 26.46299946464603181, -6.465121161284864471 ) ) ;
#16569=CARTESIAN_POINT ( 'NONE',  ( 16.92419414914112608, 122.6916909566506320, -0.1062714098145888658 ) ) ;
#16572=CARTESIAN_POINT ( 'NONE',  ( -4.962679952929507365, 117.4046820319011033, -1.029671477350346809 ) ) ;
#16573=ADVANCED_FACE ( 'NONE', ( #6015 ), #8140, .T. ) ;
#16575=LINE ( 'NONE', #16144, #36184 ) ;
#16576=CARTESIAN_POINT ( 'NONE',  ( -4.477012829077108513, 118.1289466633855199, 0.5423931779833521816 ) ) ;
#16578=CIRCLE ( 'NONE', #31555, 3.175000000000001155 ) ;
#16580=CARTESIAN_POINT ( 'NONE',  ( -0.06585476185879614308, 115.6909491485452435, -1.765419769167920094 ) ) ;
#16583=CARTESIAN_POINT ( 'NONE',  ( -8.291374016806893010, 120.0310598864996479, -1.449589630850732114 ) ) ;
#16584=CARTESIAN_POINT ( 'NONE',  ( -4.994922087954134504, 114.3796182124986984, -1.954983995200229030 ) ) ;
#16585=CARTESIAN_POINT ( 'NONE',  ( 4.502580129441241752, 118.1162376777982956, 0.7114035020871308790 ) ) ;
#16587=CARTESIAN_POINT ( 'NONE',  ( -1.752245784495178649, 156.4219299504922844, -0.9069267871912082279 ) ) ;
#16589=CARTESIAN_POINT ( 'NONE',  ( -3.612350073381208393, 115.7029516324609233, -1.621358293364550063 ) ) ;
#16590=CARTESIAN_POINT ( 'NONE',  ( 5.586884702347364673, 85.69146620154573668, 0.1116392523995368424 ) ) ;
#16591=CARTESIAN_POINT ( 'NONE',  ( 5.946884660761559971, 118.9717589635377664, -0.3494607991981760753 ) ) ;
#16592=CARTESIAN_POINT ( 'NONE',  ( -6.954653016369137575, 155.6889469082406947, -1.616181084571816085 ) ) ;
#16593=CARTESIAN_POINT ( 'NONE',  ( -0.001367086239821354828, 156.3041635968983485, 0.06841458569046227067 ) ) ;
#16594=CARTESIAN_POINT ( 'NONE',  ( 8.796322004575774400, 117.7098159678576366, -0.02677737093245648181 ) ) ;
#16595=CARTESIAN_POINT ( 'NONE',  ( -15.72482850224671225, 145.6824189663691413, -0.1796683355943700655 ) ) ;
#16596=CARTESIAN_POINT ( 'NONE',  ( -0.8472427164685307766, -8.777537934218566207, -4.544909406875613733 ) ) ;
#16597=CARTESIAN_POINT ( 'NONE',  ( 9.660431270553193173, 118.1749183431956425, 0.7024802509354081126 ) ) ;
#16599=CARTESIAN_POINT ( 'NONE',  ( 3.141231902390079878, -14.40076222614043644, 1.273921468989656969 ) ) ;
#16601=CARTESIAN_POINT ( 'NONE',  ( -5.055620027408552986, 119.3892302351119810, 0.8859254200104713650 ) ) ;
#16602=CARTESIAN_POINT ( 'NONE',  ( 0.1234711523483410095, 5.102374915558315571, -0.9659065422363407594 ) ) ;
#16603=CARTESIAN_POINT ( 'NONE',  ( -23.20005416489669869, 148.7951734159264561, -1.060305963766562831 ) ) ;
#16604=CARTESIAN_POINT ( 'NONE',  ( -0.3677562164248854293, -4.027846162062824753, 0.9036657059391408620 ) ) ;
#16606=ORIENTED_EDGE ( 'NONE', *, *, #20652, .T. ) ;
#16608=CARTESIAN_POINT ( 'NONE',  ( 4.979866836074831937, 117.8491495069952748, 0.7948704875671747105 ) ) ;
#16610=CARTESIAN_POINT ( 'NONE',  ( -16.19917940306807935, 146.4165046419237228, 0.6472847106673342843 ) ) ;
#16611=CARTESIAN_POINT ( 'NONE',  ( 3.761132227337853351, -14.12294213130394027, 4.617837385609514733 ) ) ;
#16612=CARTESIAN_POINT ( 'NONE',  ( 5.322365003948895890, 156.4258374981641282, -1.486226487625613712 ) ) ;
#16613=CIRCLE ( 'NONE', #27509, 3.175000000000001155 ) ;
#16614=CARTESIAN_POINT ( 'NONE',  ( -10.99314024304357673, 156.0189320485970086, -2.156370349642058759 ) ) ;
#16616=CARTESIAN_POINT ( 'NONE',  ( 3.216637634036228821, -14.25892527173770752, 2.941440830758975888 ) ) ;
#16617=CARTESIAN_POINT ( 'NONE',  ( -4.975175664203050907, 32.06598106186588382, 0.7459204072935272656 ) ) ;
#16618=CARTESIAN_POINT ( 'NONE',  ( 2.930943089244447464, 156.0861408873597327, -0.1605890987591809260 ) ) ;
#16624=CARTESIAN_POINT ( 'NONE',  ( 23.43370484584237445, 146.8275480241000253, 0.3132885061830184004 ) ) ;
#16625=CARTESIAN_POINT ( 'NONE',  ( -5.634266555046488989, 117.9149360781225937, 0.5245629147119165170 ) ) ;
#16626=CARTESIAN_POINT ( 'NONE',  ( -2.051901798287135037, 115.6909491485452577, 1.638078500307909247 ) ) ;
#16628=CARTESIAN_POINT ( 'NONE',  ( 1.020007333917743342, 39.20946620154573026, -1.249871353326013068 ) ) ;
#16629=EDGE_CURVE ( 'NONE', #7830, #22451, #23672, .T. ) ;
#16630=CARTESIAN_POINT ( 'NONE',  ( -0.01051220311291895665, 117.9844940561907265, 0.5260736299896251467 ) ) ;
#16631=CARTESIAN_POINT ( 'NONE',  ( -4.024516124431025688, 26.91537645720152128, -2.298571904627217499 ) ) ;
#16632=CARTESIAN_POINT ( 'NONE',  ( 5.644239659282993316, 25.55377913558855596, 6.252972086369320337 ) ) ;
#16633=CARTESIAN_POINT ( 'NONE',  ( -2.163080554094883645, 116.7372139585571915, -0.4936440420418066743 ) ) ;
#16634=CARTESIAN_POINT ( 'NONE',  ( -0.6121664022497388391, 114.3327162918516962, -2.181662845130500461 ) ) ;
#16636=CARTESIAN_POINT ( 'NONE',  ( 3.603687985131259541, 104.6144662015326077, 3.947868320610233628 ) ) ;
#16637=CARTESIAN_POINT ( 'NONE',  ( -3.789191232057584902, 13.46218022696137773, 2.646434746401360893 ) ) ;
#16639=CARTESIAN_POINT ( 'NONE',  ( -0.3704417442436215291, 117.3993836136686326, -1.500862690023503587 ) ) ;
#16640=CARTESIAN_POINT ( 'NONE',  ( 3.114041961411902371, -14.44963006906317737, 3.768961988127400353 ) ) ;
#16641=CARTESIAN_POINT ( 'NONE',  ( 0.1065646865914870872, 105.8844662015456777, -5.332932678536313809 ) ) ;
#16642=CARTESIAN_POINT ( 'NONE',  ( -0.9959262657077846415, 116.9078805053781025, 0.3180477371503355744 ) ) ;
#16643=CARTESIAN_POINT ( 'NONE',  ( 5.008579095102096979, 117.3966161975143052, -0.7759206776167619779 ) ) ;
#16645=CARTESIAN_POINT ( 'NONE',  ( 5.586884702347364673, 98.39146620154573952, 0.1116392523995368424 ) ) ;
#16647=CARTESIAN_POINT ( 'NONE',  ( 3.009276887026297587, 39.20946620154573736, -1.210121013456480599 ) ) ;
#16648=CARTESIAN_POINT ( 'NONE',  ( 3.172349117095228710, -15.63690262102951323, 5.390679387232247599 ) ) ;
#16649=CARTESIAN_POINT ( 'NONE',  ( -19.78762832257856275, 149.1964539096042870, 1.700649111281397952 ) ) ;
#16650=CARTESIAN_POINT ( 'NONE',  ( 13.99438190394152493, 121.2764344996515717, -0.9244547817413870661 ) ) ;
#16651=CARTESIAN_POINT ( 'NONE',  ( 0.4398701176286285985, 29.43434963188315834, -0.8729469796826672123 ) ) ;
#16654=DIRECTION ( 'NONE',  ( 0.9998004120163608288, 0.000000000000000000, 0.01997839162482749342 ) ) ;
#16655=CARTESIAN_POINT ( 'NONE',  ( 0.9036232957555455636, 122.5862318000603182, 0.2430700419085215502 ) ) ;
#16656=PRESENTATION_STYLE_ASSIGNMENT (( #6878 ) ) ;
#16657=CARTESIAN_POINT ( 'NONE',  ( -2.594326071755724605, 120.1437993944865354, 0.4899928688880349492 ) ) ;
#16659=CARTESIAN_POINT ( 'NONE',  ( 5.875153347143252880, 119.9178398404649926, -0.8959128733076280326 ) ) ;
#16660=CARTESIAN_POINT ( 'NONE',  ( -17.27141581160028494, 128.5728276651957742, -2.069917288257624222 ) ) ;
#16663=CARTESIAN_POINT ( 'NONE',  ( 4.366462884195458471, 118.1827284966912686, -0.4455170831428560407 ) ) ;
#16664=CARTESIAN_POINT ( 'NONE',  ( 12.13795026801524024, 151.9817061558079274, -0.5567646394148115796 ) ) ;
#16666=CARTESIAN_POINT ( 'NONE',  ( -11.83432680469874221, 124.3826620800890339, -1.661842703385269626 ) ) ;
#16667=CARTESIAN_POINT ( 'NONE',  ( 1.824651611884654967, -15.33505462125983598, 5.392305443003406751 ) ) ;
#16669=CARTESIAN_POINT ( 'NONE',  ( 4.433447712847764066, 105.1217203547995069, -2.986091683647443595 ) ) ;
#16671=AXIS2_PLACEMENT_3D ( 'NONE', #5920, #16471, #25282 ) ;
#16672=CARTESIAN_POINT ( 'NONE',  ( -0.5832499861179958334, 10.72304255322087307, 4.598074068532726599 ) ) ;
#16673=CARTESIAN_POINT ( 'NONE',  ( 10.71484998910085551, 123.2317624570580534, 1.496280440855932037 ) ) ;
#16674=CARTESIAN_POINT ( 'NONE',  ( 1.398455114368189145, 34.89464803915915780, 0.3944493173928063090 ) ) ;
#16675=EDGE_CURVE ( 'NONE', #10681, #20793, #25947, .T. ) ;
#16676=CARTESIAN_POINT ( 'NONE',  ( -2.923568588381722844, 13.88697512809157786, 3.594856661414283394 ) ) ;
#16677=CARTESIAN_POINT ( 'NONE',  ( 4.248167858406068476, 155.8413357349917021, 0.2489887396171408807 ) ) ;
#16681=CARTESIAN_POINT ( 'NONE',  ( -0.2298130577371723104, 117.3993836757663729, 1.488868159487601872 ) ) ;
#16683=CARTESIAN_POINT ( 'NONE',  ( -6.513165593194060347E-14, 68.92746620154572668, -8.865348866426607246E-18 ) ) ;
#16690=CARTESIAN_POINT ( 'NONE',  ( -4.758755041967009269, 116.8068435238802465, 0.07043225793504331866 ) ) ;
#16693=CARTESIAN_POINT ( 'NONE',  ( 6.072382902230390123, 121.4395914931731113, 0.1186111012826013000 ) ) ;
#16694=EDGE_LOOP ( 'NONE', ( #32638, #1834, #35385 ) ) ;
#16696=CARTESIAN_POINT ( 'NONE',  ( -2.896036792256268644, 156.0891579660883508, -0.1428477814196378037 ) ) ;
#16697=CARTESIAN_POINT ( 'NONE',  ( 5.507117158935161072, -13.70471586423162336, 3.054220594615255191 ) ) ;
#16698=CARTESIAN_POINT ( 'NONE',  ( -20.03018601867076853, 150.7967616730061593, 1.468133569223299961 ) ) ;
#16699=CARTESIAN_POINT ( 'NONE',  ( -2.755274729907521980, 20.69627551736597226, -3.746277899328600558 ) ) ;
#16700=CARTESIAN_POINT ( 'NONE',  ( 3.781797959329852521, 116.7736770086926867, 0.3417761088697102712 ) ) ;
#16701=CARTESIAN_POINT ( 'NONE',  ( 15.25989735510956002, 148.0267574095444445, 0.5045397742221703341 ) ) ;
#16702=CARTESIAN_POINT ( 'NONE',  ( -3.685501180670149424, 30.72893705507438611, -2.802369389919810772 ) ) ;
#16703=CARTESIAN_POINT ( 'NONE',  ( -0.2306771026100957467, -3.802149480603859377, 0.9475509996518236555 ) ) ;
#16704=CARTESIAN_POINT ( 'NONE',  ( -23.37772998923903600, 142.7868430859564626, -0.6200176421473858612 ) ) ;
#16709=CARTESIAN_POINT ( 'NONE',  ( 8.725096631921111623, 117.9837440635962054, 0.7541645143275405028 ) ) ;
#16710=EDGE_LOOP ( 'NONE', ( #38234, #22704, #32660, #6357 ) ) ;
#16711=CARTESIAN_POINT ( 'NONE',  ( -17.58824906652093745, 148.8653046532945723, 1.619734885946522596 ) ) ;
#16713=CARTESIAN_POINT ( 'NONE',  ( 9.094277710717253882, 119.2843051134756536, 1.347562189204172034 ) ) ;
#16714=CARTESIAN_POINT ( 'NONE',  ( 2.330377461923264004, 118.7486697826011977, -0.7097125967482103004 ) ) ;
#16715=CARTESIAN_POINT ( 'NONE',  ( -0.3571511390000196573, -0.07365323586406080647, 0.9071407500242820721 ) ) ;
#16716=CARTESIAN_POINT ( 'NONE',  ( -6.827620370266043182, 118.1252062928739832, -1.028125137227138275 ) ) ;
#16717=CARTESIAN_POINT ( 'NONE',  ( 4.578866339686846310, 118.0740741925940256, -0.5988308625876450630 ) ) ;
#16718=DIRECTION ( 'NONE',  ( 0.9998004120163610509, 4.016384292689131511E-17, 0.01997839162482749689 ) ) ;
#16719=EDGE_CURVE ( 'NONE', #21134, #11121, #3981, .T. ) ;
#16720=CARTESIAN_POINT ( 'NONE',  ( 10.20798870728732410, 124.0743415861677903, -0.7134647857254746706 ) ) ;
#16721=CARTESIAN_POINT ( 'NONE',  ( -8.054407255016492684, 122.8529229587361442, -0.1293742239074501532 ) ) ;
#16722=ORIENTED_EDGE ( 'NONE', *, *, #40219, .T. ) ;
#16723=CARTESIAN_POINT ( 'NONE',  ( -4.224706347173693644, 119.5670751559891585, -0.9504096833562338809 ) ) ;
#16724=CARTESIAN_POINT ( 'NONE',  ( 5.328887433758706216, -15.24262819705347916, -0.4233796293290443269 ) ) ;
#16725=DIRECTION ( 'NONE',  ( 0.9998004120163608288, 0.000000000000000000, 0.01997839162482749342 ) ) ;
#16726=CARTESIAN_POINT ( 'NONE',  ( -4.624492705069667586, 117.9598748055318822, -0.9307939849546735811 ) ) ;
#16729=CARTESIAN_POINT ( 'NONE',  ( 4.144720667518057233, 118.2390924077483589, 0.4001709429842503218 ) ) ;
#16730=B_SPLINE_SURFACE_WITH_KNOTS ( 'NONE', 3, 3, ( 
 ( #25539, #23156, #19981, #31873, #6791, #32144 ),
 ( #12957, #32349, #2976, #25950, #15730, #15939 ),
 ( #35557, #16572, #6373, #39167, #35764, #9974 ),
 ( #22947, #28735, #32780, #8624, #8201, #630 ) ),
 .UNSPECIFIED., .F., .F., .F.,
 ( 4, 4 ),
 ( 4, 2, 4 ),
 ( 0.000000000000000000, 1.000000000000000000 ),
 ( 0.000000000000000000, 0.5000000000000000000, 1.000000000000000000 ),
 .UNSPECIFIED. ) ;
#16731=CARTESIAN_POINT ( 'NONE',  ( 18.01525633490669520, 148.5173242358814321, 2.382443637188214502 ) ) ;
#16733=CARTESIAN_POINT ( 'NONE',  ( 20.51686376604209983, 129.1072961674477710, 0.4099757654675941221 ) ) ;
#16734=CARTESIAN_POINT ( 'NONE',  ( -4.107119205180256749, 117.8719421043398370, 0.6926522829710091145 ) ) ;
#16735=CARTESIAN_POINT ( 'NONE',  ( 8.391066749008803782, -15.30525627429770097, -0.4359234444501501327 ) ) ;
#16736=CARTESIAN_POINT ( 'NONE',  ( 8.816380758798560535, 123.2701452714374568, 0.6637701367642926398 ) ) ;
#16738=CARTESIAN_POINT ( 'NONE',  ( 0.3479910049260485638, 116.9201722098172382, -0.3032510685202791101 ) ) ;
#16743=CARTESIAN_POINT ( 'NONE',  ( -8.217147260422519750, 117.5004391570743394, -0.1493243188240318264 ) ) ;
#16745=CARTESIAN_POINT ( 'NONE',  ( -8.061441164751348865, 121.1678581073247614, -1.290394762592997679 ) ) ;
#16747=CARTESIAN_POINT ( 'NONE',  ( -9.229671467331892032, 123.9961275534082148, -0.5040434471971627639 ) ) ;
#16748=CARTESIAN_POINT ( 'NONE',  ( 3.649535173467634674, -14.21384370944696407, 4.751373335446510637 ) ) ;
#16749=CARTESIAN_POINT ( 'NONE',  ( -18.94714202558217764, 128.6554162386474047, 0.8647899522199680167 ) ) ;
#16751=CARTESIAN_POINT ( 'NONE',  ( 16.85465591277202080, 155.2173118157008673, 0.4068649486066870935 ) ) ;
#16753=CARTESIAN_POINT ( 'NONE',  ( 4.560200836559435977, -11.68919918208664122, 0.6963878748952898601 ) ) ;
#16754=CARTESIAN_POINT ( 'NONE',  ( -2.432703290510899841, 105.1243935390225204, 4.756760888922076269 ) ) ;
#16757=CARTESIAN_POINT ( 'NONE',  ( -8.197999847188267353, 120.7315320437793531, 1.065923837117515260 ) ) ;
#16759=CARTESIAN_POINT ( 'NONE',  ( 4.506137822554599381, 3.376467715207942533, 1.027655576270160243 ) ) ;
#16760=CARTESIAN_POINT ( 'NONE',  ( 14.51227343941606485, 121.4416029531759591, 1.418621967605989909 ) ) ;
#16761=CARTESIAN_POINT ( 'NONE',  ( 15.72550100231830150, 145.6881679641598453, 0.3142329346387512934 ) ) ;
#16763=CARTESIAN_POINT ( 'NONE',  ( 18.41670328667946421, 131.7683309214445728, -1.453117541724253448 ) ) ;
#16764=CARTESIAN_POINT ( 'NONE',  ( -2.734508853367146219, 0.3528594962865297391, 3.724956791467788353 ) ) ;
#16765=CARTESIAN_POINT ( 'NONE',  ( -22.33788829447793489, 150.2360280492587776, -1.519312068210846078 ) ) ;
#16767=CARTESIAN_POINT ( 'NONE',  ( -7.869802931810743196, 122.7053923345238502, -0.1572573916676445194 ) ) ;
#16770=CARTESIAN_POINT ( 'NONE',  ( -12.13843755257585144, 130.5412724693565849, 0.1686832038582291304 ) ) ;
#16772=CARTESIAN_POINT ( 'NONE',  ( 5.747688368404943127, -13.35872296688338245, 2.372087187842143674 ) ) ;
#16775=CARTESIAN_POINT ( 'NONE',  ( -0.9968812942979460301, 106.0882118856391259, -5.244929698535035989 ) ) ;
#16776=EDGE_LOOP ( 'NONE', ( #24047, #1707, #15641, #23296 ) ) ;
#16777=CARTESIAN_POINT ( 'NONE',  ( 4.990993783036389964, 119.0545008048120366, 1.104648745759416295 ) ) ;
#16780=VECTOR ( 'NONE', #11117, 1000.000000000000000 ) ;
#16781=CARTESIAN_POINT ( 'NONE',  ( -14.74755344529033962, 121.0688405154646858, 0.6244351273456011375 ) ) ;
#16782=CARTESIAN_POINT ( 'NONE',  ( -5.272568914482754998, 19.56627864152888208, 6.568537450970175939 ) ) ;
#16783=CARTESIAN_POINT ( 'NONE',  ( 12.30032609686865186, 128.4316967252784991, 1.345898664372764175 ) ) ;
#16784=EDGE_CURVE ( 'NONE', #1073, #38342, #36028, .T. ) ;
#16785=CARTESIAN_POINT ( 'NONE',  ( 23.20995092461732057, 148.9919839608952827, -0.1323997120335723976 ) ) ;
#16793=CARTESIAN_POINT ( 'NONE',  ( -4.552334805148916530, 118.1085767403579467, 0.4996156392678010594 ) ) ;
#16795=AXIS2_PLACEMENT_3D ( 'NONE', #12195, #34781, #31362 ) ;
#16798=CARTESIAN_POINT ( 'NONE',  ( 3.813032422245561825, 118.9366574157493943, -0.7812632686729226172 ) ) ;
#16799=CARTESIAN_POINT ( 'NONE',  ( -3.406460098309205264, 108.6786390861269922, -4.123178694279357792 ) ) ;
#16800=CARTESIAN_POINT ( 'NONE',  ( 4.546980637774593603, 118.0358567185017762, 0.8570574294820361150 ) ) ;
#16801=CARTESIAN_POINT ( 'NONE',  ( -12.64766777886155857, 130.7634385742845780, -1.140803344710751288 ) ) ;
#16803=CARTESIAN_POINT ( 'NONE',  ( 0.8540871238041118918, 117.3993835805474362, -1.452928456153284698 ) ) ;
#16804=CARTESIAN_POINT ( 'NONE',  ( 5.516342712684529026, 117.4962825466697467, -0.6091453463174707483 ) ) ;
#16806=CARTESIAN_POINT ( 'NONE',  ( -1.917342111448811393, 156.7095495334699535, -1.310369884728256995 ) ) ;
#16807=CARTESIAN_POINT ( 'NONE',  ( 5.329288917532060132, 116.0444662015457453, 0.2890495193807575691 ) ) ;
#16809=CARTESIAN_POINT ( 'NONE',  ( 7.991391493690734649, 121.7106681566311579, -0.7744224044265761719 ) ) ;
#16810=CARTESIAN_POINT ( 'NONE',  ( -8.711945433812360307, 123.6715832479121673, -0.08701538749149796692 ) ) ;
#16811=CARTESIAN_POINT ( 'NONE',  ( -0.5496829067194369811, 0.7180641350488168317, -4.598301960397928489 ) ) ;
#16812=CARTESIAN_POINT ( 'NONE',  ( -0.01133159106151370929, 159.5297144918048673, 0.5670791535570577357 ) ) ;
#16814=CARTESIAN_POINT ( 'NONE',  ( 3.190981477959303980, -15.14443901668413517, 3.594454035019850835 ) ) ;
#16815=CARTESIAN_POINT ( 'NONE',  ( -16.91343413265456874, 151.2926467857828072, 1.744909534579184518 ) ) ;
#16816=CARTESIAN_POINT ( 'NONE',  ( -0.1559983344249278314, 9.848737885527594216, 0.9609112391775298523 ) ) ;
#16817=CARTESIAN_POINT ( 'NONE',  ( -3.798364743159273083, 116.8316721669309572, -0.3950458664356921168 ) ) ;
#16818=CIRCLE ( 'NONE', #27008, 3.175000000000001155 ) ;
#16819=CARTESIAN_POINT ( 'NONE',  ( -0.3022039251088723399, 24.96921649940425425, -0.9259629999792299282 ) ) ;
#16822=CARTESIAN_POINT ( 'NONE',  ( 6.667064533335116394, 121.2389289720308199, 0.3413157713140476113 ) ) ;
#16823=CARTESIAN_POINT ( 'NONE',  ( -6.293976855803995463, 155.3815620563194955, 0.6499927463934688232 ) ) ;
#16824=CARTESIAN_POINT ( 'NONE',  ( 4.181132250215417123, -13.15738584483822038, 3.071181452022354819 ) ) ;
#16825=CARTESIAN_POINT ( 'NONE',  ( 17.54876304910989049, 147.2926247242496345, -1.462364720961515818 ) ) ;
#16826=CARTESIAN_POINT ( 'NONE',  ( -17.10357040864165512, 151.3967157021085654, -2.430234537686703611 ) ) ;
#16827=CARTESIAN_POINT ( 'NONE',  ( 1.041310694851599550, 104.6144662015456817, 4.721824808304355692 ) ) ;
#16829=CARTESIAN_POINT ( 'NONE',  ( 3.205266406700632675, -14.32095172213143641, 3.103221849221895035 ) ) ;
#16830=CARTESIAN_POINT ( 'NONE',  ( 0.02537255736346739204, 39.20946620154573026, -1.269746523260778748 ) ) ;
#16831=CARTESIAN_POINT ( 'NONE',  ( 3.740144479511048559, 121.0798372856833538, 0.007817740762067634797 ) ) ;
#16834=CARTESIAN_POINT ( 'NONE',  ( -4.369275640764541002, 112.0482830817664137, 2.684166018868272552 ) ) ;
#16835=CARTESIAN_POINT ( 'NONE',  ( 1.038904431729710920, 105.9875614017122274, 5.236931198412617228 ) ) ;
#16838=CARTESIAN_POINT ( 'NONE',  ( 13.43120660244749942, 156.9273374874128137, 0.2039374989780119718 ) ) ;
#16840=CARTESIAN_POINT ( 'NONE',  ( -5.516342712684657812, 117.4962825466697467, 0.6091453463174709704 ) ) ;
#16841=AXIS2_PLACEMENT_3D ( 'NONE', #26993, #41621, #12000 ) ;
#16842=CARTESIAN_POINT ( 'NONE',  ( -2.215833297304112381, 118.7629491485454167, 1.137586326187810082 ) ) ;
#16843=DIRECTION ( 'NONE',  ( -5.206863593109713661E-17, 1.000000000000000000, -1.077750396879097183E-30 ) ) ;
#16844=CARTESIAN_POINT ( 'NONE',  ( -4.169593158777295194, 32.11536586671030591, 0.7217217036562449950 ) ) ;
#16845=CARTESIAN_POINT ( 'NONE',  ( 13.64080552068789487, 122.3361261571837986, 1.764911742735522537 ) ) ;
#16846=CARTESIAN_POINT ( 'NONE',  ( -1.535301415185580609, 19.99377045568717293, 4.360315235486975638 ) ) ;
#16847=CARTESIAN_POINT ( 'NONE',  ( 5.972130579385131810, 18.43406553185754504, -5.949252452957764170 ) ) ;
#16848=CARTESIAN_POINT ( 'NONE',  ( -8.629662989089693426, 118.4205806735777600, -1.047178699074468033 ) ) ;
#16849=CARTESIAN_POINT ( 'NONE',  ( -1.600579373210057055, 119.3928400758114918, -0.6828601607076613123 ) ) ;
#16853=CARTESIAN_POINT ( 'NONE',  ( 3.935102970030661673, 16.48578375386999539, 2.424025302511324309 ) ) ;
#16856=CARTESIAN_POINT ( 'NONE',  ( 2.843374750741399559, -13.00285448706176084, 0.5077109796929276664 ) ) ;
#16857=CARTESIAN_POINT ( 'NONE',  ( 2.312669815851102317, 124.5312663981120380, 0.02133033151766260474 ) ) ;
#16858=CARTESIAN_POINT ( 'NONE',  ( -3.862028650946987884, 117.0275016673472663, 0.3788463918649359052 ) ) ;
#16859=CARTESIAN_POINT ( 'NONE',  ( 4.854370033424973307, 117.4083523622822298, -0.9982548204258623326 ) ) ;
#16863=CARTESIAN_POINT ( 'NONE',  ( -6.784104592523965728E-14, 136.3644662015457527, 7.159772606002533724E-18 ) ) ;
#16864=CARTESIAN_POINT ( 'NONE',  ( 4.918313631922730522, -15.33159817589810281, -0.1794070962640156031 ) ) ;
#16865=CARTESIAN_POINT ( 'NONE',  ( -16.44572402506200248, 128.5611466799914240, 1.520858254922803354 ) ) ;
#16866=CARTESIAN_POINT ( 'NONE',  ( 10.89609060007105867, 119.5270080912504653, -0.8636533125102805464 ) ) ;
#16867=CARTESIAN_POINT ( 'NONE',  ( 4.560362914109654220, -11.68884639558073069, 0.6953251057713033534 ) ) ;
#16869=ORIENTED_EDGE ( 'NONE', *, *, #27165, .T. ) ;
#16871=CARTESIAN_POINT ( 'NONE',  ( 2.269084004857000458, 124.1308405194309188, 0.09931761310301601142 ) ) ;
#16872=CARTESIAN_POINT ( 'NONE',  ( -4.773351466264551313, 117.6315869056820418, 0.9547913690014270260 ) ) ;
#16873=CARTESIAN_POINT ( 'NONE',  ( -0.8386157876100502895, 156.7682548876429109, 1.206618248707300056 ) ) ;
#16874=CARTESIAN_POINT ( 'NONE',  ( -3.682264917456322895, 63.84746620154572838, -0.07358041635423923088 ) ) ;
#16875=CARTESIAN_POINT ( 'NONE',  ( 17.81946051592193925, 148.9562551477873740, -1.662425298156809284 ) ) ;
#16876=CARTESIAN_POINT ( 'NONE',  ( -10.35908644403310142, 120.1444133044471556, -1.518303869478637491 ) ) ;
#16877=FACE_BOUND ( 'NONE', #25379, .T. ) ;
#16878=ORIENTED_EDGE ( 'NONE', *, *, #26845, .F. ) ;
#16879=CARTESIAN_POINT ( 'NONE',  ( 4.514071185496203675, 118.1172072462845648, -0.5456106512196506886 ) ) ;
#16880=CARTESIAN_POINT ( 'NONE',  ( 10.74829939017195635, 126.1521286088116369, -0.3663887985317100804 ) ) ;
#16882=CARTESIAN_POINT ( 'NONE',  ( 3.411949332026259274, -14.94726182254324520, 2.206293558762954188 ) ) ;
#16883=CARTESIAN_POINT ( 'NONE',  ( 5.040103533774599853, 105.1217021379421084, -1.780561253959252577 ) ) ;
#16885=CARTESIAN_POINT ( 'NONE',  ( 0.02375515148176195884, 10.92298121479113426, 4.626086752085273979 ) ) ;
#16886=CARTESIAN_POINT ( 'NONE',  ( 4.298694136813140609, 120.0471566133196291, 0.8457497992440220491 ) ) ;
#16887=CARTESIAN_POINT ( 'NONE',  ( -2.817352878905182489, 30.99554970294005685, 0.7112045236633145473 ) ) ;
#16888=CARTESIAN_POINT ( 'NONE',  ( -0.2480930319908794535, 10.21371511114847053, -4.635561276548324727 ) ) ;
#16889=CARTESIAN_POINT ( 'NONE',  ( 15.73804366022553403, 146.9052959264698757, 0.5443085878246290976 ) ) ;
#16890=DIRECTION ( 'NONE',  ( 0.9998004120163608288, 0.000000000000000000, 0.01997839162482760791 ) ) ;
#16892=CARTESIAN_POINT ( 'NONE',  ( -2.153613147569079178, 116.3508512159758226, -0.2939559217719306949 ) ) ;
#16893=CARTESIAN_POINT ( 'NONE',  ( -0.02983097946891718685, 117.3993836135855418, 1.492864285907047561 ) ) ;
#16900=DIRECTION ( 'NONE',  ( 5.206863593109713661E-17, -1.000000000000000000, 1.077750396879097183E-30 ) ) ;
#16903=CARTESIAN_POINT ( 'NONE',  ( -16.78241155767117476, 155.2615993841311877, 0.07296080027729320849 ) ) ;
#16906=CARTESIAN_POINT ( 'NONE',  ( -7.792461912600263219, 122.5708967970961538, -0.3530462997155650595 ) ) ;
#16910=CARTESIAN_POINT ( 'NONE',  ( -8.959768907663441695, 123.9105667600146177, -0.2128205007565311946 ) ) ;
#16911=CARTESIAN_POINT ( 'NONE',  ( 6.089492611447847814, -14.32660765653466584, 1.811095812122764270 ) ) ;
#16913=CARTESIAN_POINT ( 'NONE',  ( -13.92608219098140232, 121.7708260186165177, 1.076920499313079871 ) ) ;
#16914=CARTESIAN_POINT ( 'NONE',  ( 1.141857472271699425, 24.90688314728938835, 4.478778191171412182 ) ) ;
#16915=CARTESIAN_POINT ( 'NONE',  ( 23.26560126724718813, 148.8247458934765461, 0.9199859812867274833 ) ) ;
#16916=CARTESIAN_POINT ( 'NONE',  ( 2.086111074717174940, -15.67854476527870489, 5.662254629584102972 ) ) ;
#16918=CARTESIAN_POINT ( 'NONE',  ( -0.9742996550080020857, -5.754034560434002188, 0.05241923913101136784 ) ) ;
#16919=CARTESIAN_POINT ( 'NONE',  ( -21.86057864824949704, 151.4416708234707301, -0.7622892283599552732 ) ) ;
#16923=CARTESIAN_POINT ( 'NONE',  ( -8.779664665387997502, 117.8111546309878293, 0.2055069415728331406 ) ) ;
#16924=CARTESIAN_POINT ( 'NONE',  ( -17.99030040960602506, 148.1388135707062474, 1.617688361210429804 ) ) ;
#16926=CARTESIAN_POINT ( 'NONE',  ( 21.20529034131888224, 148.8133262010608462, 2.309157841868048511 ) ) ;
#16927=CARTESIAN_POINT ( 'NONE',  ( 1.091998727716591455, 158.1148137021529578, -1.603323485041850072 ) ) ;
#16928=CARTESIAN_POINT ( 'NONE',  ( 0.6341690014321406110, -14.98600045789189394, -0.7374838701073263003 ) ) ;
#16929=CARTESIAN_POINT ( 'NONE',  ( -12.43770564682712632, 156.7420262770442037, -1.659670365993107133 ) ) ;
#16930=CARTESIAN_POINT ( 'NONE',  ( 4.719769988271771410, 117.9725737481287098, -0.6355710737933278898 ) ) ;
#16931=DIRECTION ( 'NONE',  ( 4.017660918040594346E-17, -1.000000000000000000, -2.376309959284834438E-19 ) ) ;
#16933=CARTESIAN_POINT ( 'NONE',  ( 9.755760200704601814, 153.9716628027005925, -0.9476658408544211820 ) ) ;
#16934=CARTESIAN_POINT ( 'NONE',  ( -9.191399985966498321, 124.2403664864748549, -0.1492717680338158659 ) ) ;
#16936=CARTESIAN_POINT ( 'NONE',  ( -8.426631749355234291, 120.7201681212196291, -1.435507493075423691 ) ) ;
#16937=CARTESIAN_POINT ( 'NONE',  ( 4.909888997889673590, -15.31669448615230422, -0.4577950299049654559 ) ) ;
#16938=CARTESIAN_POINT ( 'NONE',  ( 3.174366308151880922, 104.6144662015457243, 0.06343139340882769650 ) ) ;
#16939=CARTESIAN_POINT ( 'NONE',  ( -4.704478397100538167, 117.9644704501329784, -0.8020208166650271142 ) ) ;
#16942=CARTESIAN_POINT ( 'NONE',  ( 5.693059210196379283, 156.8407539676644546, 1.898889529600695791 ) ) ;
#16943=CARTESIAN_POINT ( 'NONE',  ( -2.579283729523311308, 34.63205429821886838, 0.7922911722492685938 ) ) ;
#16944=AXIS2_PLACEMENT_3D ( 'NONE', #30165, #27179, #4831 ) ;
#16945=CARTESIAN_POINT ( 'NONE',  ( 5.775410652799734201, 116.9337168780244696, 0.1011920919882985798 ) ) ;
#16946=CARTESIAN_POINT ( 'NONE',  ( 2.510961470319720501, 15.29743382693132148, 8.092466016612050339 ) ) ;
#16947=CARTESIAN_POINT ( 'NONE',  ( 3.666883307181533436, 120.9289264519876070, 0.3209655359951391063 ) ) ;
#16948=CARTESIAN_POINT ( 'NONE',  ( 22.42204277426964154, 149.9331680011685251, -0.7277228188736588610 ) ) ;
#16950=ORIENTED_EDGE ( 'NONE', *, *, #37873, .T. ) ;
#16952=CARTESIAN_POINT ( 'NONE',  ( -16.14921358636499704, 121.2501203052637493, -0.2714571880805007331 ) ) ;
#16953=ORIENTED_EDGE ( 'NONE', *, *, #21517, .T. ) ;
#16954=CARTESIAN_POINT ( 'NONE',  ( -6.632770492600033485, 120.7515164533844398, -1.069572372112960634 ) ) ;
#16955=DIRECTION ( 'NONE',  ( 0.9998004120163608288, 4.016384292689131511E-17, 0.01997839162482749342 ) ) ;
#16956=CARTESIAN_POINT ( 'NONE',  ( -9.178653662903588639, 123.9301100385560943, -0.5015510438870897092 ) ) ;
#16957=CARTESIAN_POINT ( 'NONE',  ( 2.228616319073483787, -14.90713850702725374, 5.562102343610016320 ) ) ;
#16958=CARTESIAN_POINT ( 'NONE',  ( -21.25505906629481245, 136.5942649496780632, 0.9712689567086304487 ) ) ;
#16959=CARTESIAN_POINT ( 'NONE',  ( -11.83539255247756117, 152.0195595274622349, -0.2364993098673504601 ) ) ;
#16960=CARTESIAN_POINT ( 'NONE',  ( -0.001319893060215945229, 116.4580521601689185, 0.06605284600166366760 ) ) ;
#16962=CARTESIAN_POINT ( 'NONE',  ( -3.178183004559932190, -7.902942162671289239, -3.366045245292264010 ) ) ;
#16963=CARTESIAN_POINT ( 'NONE',  ( 4.250140209130199409, 105.1218014449359117, 3.241604550325138501 ) ) ;
#16966=CARTESIAN_POINT ( 'NONE',  ( 8.238225305713989144, 120.2906795671698319, 1.445116664898250303 ) ) ;
#16967=VECTOR ( 'NONE', #40412, 1000.000000000000114 ) ;
#16968=CARTESIAN_POINT ( 'NONE',  ( 1.294644163514462987, -7.843371450943685375, 4.453423563430108700 ) ) ;
#16969=CARTESIAN_POINT ( 'NONE',  ( 14.92730792698318076, 121.5307057168427605, 1.330945954902035044 ) ) ;
#16972=CARTESIAN_POINT ( 'NONE',  ( 15.69714418277264123, 125.4375369430449609, -1.335551531390729130 ) ) ;
#16973=CARTESIAN_POINT ( 'NONE',  ( 1.583070580811935191, 1.852152477310867074, 4.353984577079609508 ) ) ;
#16974=CARTESIAN_POINT ( 'NONE',  ( -22.16805208646096403, 150.4821223471089411, -1.513879355785526348 ) ) ;
#16977=CARTESIAN_POINT ( 'NONE',  ( -11.92666644034625278, 151.9662372315928280, 0.1848526535252738023 ) ) ;
#16978=CARTESIAN_POINT ( 'NONE',  ( 4.841517317049865987, -14.78816330421856051, 4.356870016251622957 ) ) ;
#16980=DIRECTION ( 'NONE',  ( 0.9998004120163609398, 0.000000000000000000, 0.01997839162482749689 ) ) ;
#16983=CARTESIAN_POINT ( 'NONE',  ( 13.59052456474551640, 154.1626644387825991, 2.292254590369200873 ) ) ;
#16985=CARTESIAN_POINT ( 'NONE',  ( 4.756847264626144600, 117.4019737204766329, 1.206737312781331672 ) ) ;
#16986=CARTESIAN_POINT ( 'NONE',  ( -6.900334503690650934, 117.6856483911789581, 0.5402308543058539358 ) ) ;
#16987=CARTESIAN_POINT ( 'NONE',  ( -4.837940364245437941, 10.07446788996644038, 6.911991265526966188 ) ) ;
#16988=CARTESIAN_POINT ( 'NONE',  ( 9.867978122178516998, 123.6875948057429895, 1.092113756099770239 ) ) ;
#16989=DIRECTION ( 'NONE',  ( -0.9998004120163608288, 0.000000000000000000, -0.01997839162482749342 ) ) ;
#16992=CARTESIAN_POINT ( 'NONE',  ( 15.29680631459140017, 120.8527393138689376, -0.2092734171533191523 ) ) ;
#16996=CARTESIAN_POINT ( 'NONE',  ( 5.101394537142137864, 113.7221017772263423, -1.664686724803478679 ) ) ;
#17000=CARTESIAN_POINT ( 'NONE',  ( -4.429393387400064164, 118.1654609044154824, 0.4666533859188604083 ) ) ;
#17002=ORIENTED_EDGE ( 'NONE', *, *, #14689, .T. ) ;
#17005=CARTESIAN_POINT ( 'NONE',  ( -3.956238299408818104, 119.1072596976981686, -0.9222601227749728237 ) ) ;
#17006=CARTESIAN_POINT ( 'NONE',  ( -5.328278062783084579, 116.9387654363850260, -0.9571818161585842200 ) ) ;
#17007=CARTESIAN_POINT ( 'NONE',  ( 4.488792732110129968, 118.1174534351576710, 0.7255436720916952353 ) ) ;
#17008=CARTESIAN_POINT ( 'NONE',  ( -3.609032566395439012, 120.7384399880717467, -0.4518473439704069894 ) ) ;
#17009=CARTESIAN_POINT ( 'NONE',  ( -0.7314521050140387892, 115.7029491485454002, -1.756324785531854671 ) ) ;
#17011=CARTESIAN_POINT ( 'NONE',  ( 1.101716543613451726, 118.1651004027584122, -0.8326739446211146589 ) ) ;
#17012=CARTESIAN_POINT ( 'NONE',  ( 6.342742252399900416, 120.0627515544778134, -0.2010047130458858800 ) ) ;
#17013=CARTESIAN_POINT ( 'NONE',  ( -6.520514997712391292, 120.9817801663137971, -0.9553606176145342799 ) ) ;
#17014=CARTESIAN_POINT ( 'NONE',  ( -4.171990346301578612, 104.6144662015457385, -4.124402238216698713 ) ) ;
#17017=CARTESIAN_POINT ( 'NONE',  ( -1.558514902584574369, 156.2615677632183235, 0.04594967285455571482 ) ) ;
#17018=CARTESIAN_POINT ( 'NONE',  ( -3.174366308152012817, 95.34346620154573770, -0.06343139340882730792 ) ) ;
#17019=CARTESIAN_POINT ( 'NONE',  ( 22.14168286312773404, 150.6715983490228723, 1.403651840795991035 ) ) ;
#17021=CARTESIAN_POINT ( 'NONE',  ( 2.463764682325012778, -15.17880951736275108, 4.811303307383569816 ) ) ;
#17023=CARTESIAN_POINT ( 'NONE',  ( -6.683041398157647528, 119.8184877057495754, 1.002300253150233633 ) ) ;
#17024=CARTESIAN_POINT ( 'NONE',  ( -0.7316449863892299232, -12.60219034754442902, -0.6469547163463490458 ) ) ;
#17025=CARTESIAN_POINT ( 'NONE',  ( -22.25501949494962517, 137.0232865695268458, -1.151097374996565392 ) ) ;
#17026=CARTESIAN_POINT ( 'NONE',  ( -0.9739946362265716751, -5.975847910206034896, -0.08934465120823924245 ) ) ;
#17029=CARTESIAN_POINT ( 'NONE',  ( 4.902456202885992376, 117.5302216577071874, 0.8631654989601055261 ) ) ;
#17031=CARTESIAN_POINT ( 'NONE',  ( -13.98505335951055706, 150.2679186505038160, 0.6609695396245746091 ) ) ;
#17032=CARTESIAN_POINT ( 'NONE',  ( 4.970078376064472003, -11.71998231623441100, 0.7442660586517341192 ) ) ;
#17033=CARTESIAN_POINT ( 'NONE',  ( 7.187319939301631599, 155.7895407640516510, -1.441898956427383416 ) ) ;
#17034=CARTESIAN_POINT ( 'NONE',  ( -19.27109647334615161, 148.6897983921382433, -2.507318192549734537 ) ) ;
#17035=CARTESIAN_POINT ( 'NONE',  ( -4.780813784901702057, 104.6144662015457243, 0.7323647157448879286 ) ) ;
#17036=CARTESIAN_POINT ( 'NONE',  ( 2.237742905438162122, -15.06201634873256801, 5.120316289255383069 ) ) ;
#17038=CARTESIAN_POINT ( 'NONE',  ( 8.102825354745226250, 122.8525693413601800, 0.01624079103423765880 ) ) ;
#17044=CARTESIAN_POINT ( 'NONE',  ( -5.036351857865265735, 117.3993844875897139, 0.5494637324817667201 ) ) ;
#17045=EDGE_CURVE ( 'NONE', #5326, #3481, #24063, .T. ) ;
#17046=CARTESIAN_POINT ( 'NONE',  ( 16.85745507829906131, 155.2173118157008673, 0.2667832593600953928 ) ) ;
#17048=CARTESIAN_POINT ( 'NONE',  ( 1.889907755066986716, -15.70955065773127401, 5.776080436909005300 ) ) ;
#17051=CARTESIAN_POINT ( 'NONE',  ( 20.10333444936986069, 149.6821479856479300, 2.421853341415478589 ) ) ;
#17052=VERTEX_POINT ( 'NONE', #2135 ) ;
#17053=CARTESIAN_POINT ( 'NONE',  ( -2.203247880972440065, 24.02835216854757405, 8.161197317184477384 ) ) ;
#17054=CARTESIAN_POINT ( 'NONE',  ( 5.518253758338024895, 117.5767191514016758, -0.7526249397660861318 ) ) ;
#17055=CARTESIAN_POINT ( 'NONE',  ( -3.148404055480067409, 118.0279923103727242, -0.8990514348027989211 ) ) ;
#17057=CARTESIAN_POINT ( 'NONE',  ( -4.002141586467248047, 110.9560809575028912, -3.257691571474720771 ) ) ;
#17058=CARTESIAN_POINT ( 'NONE',  ( -4.573472120527176443, 105.1215731529328821, 2.768881509815038999 ) ) ;
#17059=CARTESIAN_POINT ( 'NONE',  ( 4.513502956352341222, 8.064680226961385756, -0.9949261897555528034 ) ) ;
#17062=CARTESIAN_POINT ( 'NONE',  ( -3.882979742979310700, 109.3893691838257354, -3.664566828557135114 ) ) ;
#17063=CARTESIAN_POINT ( 'NONE',  ( 2.870361413894247260, -14.70454541201141119, 4.341408117703424274 ) ) ;
#17064=CARTESIAN_POINT ( 'NONE',  ( 5.854232237047439114, 124.7508695889173111, 0.1141955550013107751 ) ) ;
#17065=CARTESIAN_POINT ( 'NONE',  ( -15.53115535783876489, 121.4967652112180048, 0.4657050394012309802 ) ) ;
#17067=CARTESIAN_POINT ( 'NONE',  ( 5.913343974131921144, 116.9636705803897456, 0.1181626845772993789 ) ) ;
#17070=CARTESIAN_POINT ( 'NONE',  ( -5.208855653336853742, 31.38455280743060527, -0.6720767434146609487 ) ) ;
#17071=CARTESIAN_POINT ( 'NONE',  ( 2.830806653267172734, -15.77471167405206032, 5.191726263073638492 ) ) ;
#17072=CARTESIAN_POINT ( 'NONE',  ( -20.31268976784564373, 148.7458375694471044, 1.664162616495830305 ) ) ;
#17074=CARTESIAN_POINT ( 'NONE',  ( -1.251853189678833411, -4.679435864505671283, 4.458631606201990394 ) ) ;
#17078=CARTESIAN_POINT ( 'NONE',  ( 1.788686868885968506, 120.9773948236336878, 0.4149341611056207579 ) ) ;
#17080=CARTESIAN_POINT ( 'NONE',  ( -17.00008652715119695, 148.0818255213264365, 1.363822447394349213 ) ) ;
#17082=CARTESIAN_POINT ( 'NONE',  ( 2.445625216771064814, 119.3768144667271542, -0.6598031440805111059 ) ) ;
#17084=CARTESIAN_POINT ( 'NONE',  ( -12.98660267081559105, 122.0079276396459704, -1.762897954238471954 ) ) ;
#17086=CARTESIAN_POINT ( 'NONE',  ( 4.117406091950198466, 118.2429491485453354, -0.1872858632366372345 ) ) ;
#17087=CARTESIAN_POINT ( 'NONE',  ( 16.01386893308418635, 146.3393691146323761, -0.4087692286948388376 ) ) ;
#17089=CARTESIAN_POINT ( 'NONE',  ( 2.102798109511007318, -15.25784609616889753, 5.176374340497880588 ) ) ;
#17090=CARTESIAN_POINT ( 'NONE',  ( 0.1605948352954452707, 105.1223807299189588, -5.342326028501328317 ) ) ;
#17092=CARTESIAN_POINT ( 'NONE',  ( -4.027482788729651375, -0.2968512080594384317, 2.264360808822050597 ) ) ;
#17093=CARTESIAN_POINT ( 'NONE',  ( 11.37357585002882843, 124.5424752485109963, 1.510439678823544574 ) ) ;
#17094=CARTESIAN_POINT ( 'NONE',  ( 2.744290041233341970, 37.36458345705863593, -0.9092844709908223244 ) ) ;
#17096=CARTESIAN_POINT ( 'NONE',  ( 0.1710433496020407063, 14.98650505531991506, 4.637963194678765610 ) ) ;
#17097=CARTESIAN_POINT ( 'NONE',  ( 15.72281364106769352, 146.8976350983841144, 0.3655119725415951204 ) ) ;
#17098=DIRECTION ( 'NONE',  ( 0.8620390596215063983, 0.5065490486308654727, 0.01722559195018080053 ) ) ;
#17101=CARTESIAN_POINT ( 'NONE',  ( -8.788814435013840409, 117.7123315311960710, -0.3507367455258986189 ) ) ;
#17102=CARTESIAN_POINT ( 'NONE',  ( 5.586884702347363785, 117.3144662015457271, 0.1116392523995368424 ) ) ;
#17104=CARTESIAN_POINT ( 'NONE',  ( -4.855072294470597072, 115.7029491485453718, 1.279409886141102071 ) ) ;
#17107=CARTESIAN_POINT ( 'NONE',  ( -0.9514613986627886710, 10.21077804425927305, -8.405459466743828045 ) ) ;
#17108=EDGE_CURVE ( 'NONE', #40141, #38260, #13605, .T. ) ;
#17113=CARTESIAN_POINT ( 'NONE',  ( -3.265120802789957200, 159.4600617640778353, 0.2122772200314293756 ) ) ;
#17116=CARTESIAN_POINT ( 'NONE',  ( 7.795928871158808171, 122.5882798252810062, 0.001158467290666534508 ) ) ;
#17119=CARTESIAN_POINT ( 'NONE',  ( -14.67383990354524492, 148.8475317811793559, -0.3438330757172305407 ) ) ;
#17120=CARTESIAN_POINT ( 'NONE',  ( 6.086938242954471612, -13.85866328171454853, 1.967354546201298682 ) ) ;
#17122=CARTESIAN_POINT ( 'NONE',  ( -21.15257933310689253, 148.4376209648218321, 1.514591261405503930 ) ) ;
#17123=CARTESIAN_POINT ( 'NONE',  ( 3.979181138743986601, 26.09377549647152961, 2.406711837290479661 ) ) ;
#17124=CARTESIAN_POINT ( 'NONE',  ( 3.764301891765636121, 116.7207137014398626, 0.2841661138181406088 ) ) ;
#17125=CARTESIAN_POINT ( 'NONE',  ( -6.453647670433203483E-14, 66.13346620154574396, 1.207165459738467839E-19 ) ) ;
#17127=CARTESIAN_POINT ( 'NONE',  ( 0.2014313232957813393, -8.551994341567581870, -0.9548264729560895780 ) ) ;
#17128=CARTESIAN_POINT ( 'NONE',  ( -1.837930215757131558, 116.5452236745340429, -0.1764961812833932275 ) ) ;
#17130=CARTESIAN_POINT ( 'NONE',  ( 4.937033159817793226, 117.4086831280190637, 1.082238659715207607 ) ) ;
#17131=CARTESIAN_POINT ( 'NONE',  ( 8.759280421985048193, 117.8332167676661868, 0.5881991161353357089 ) ) ;
#17132=CARTESIAN_POINT ( 'NONE',  ( -2.123774309200991972, 157.0334531201187644, 1.456117127909798414 ) ) ;
#17134=CARTESIAN_POINT ( 'NONE',  ( 21.11954758237290619, 149.1058327099893290, 2.305704729659640240 ) ) ;
#17135=CARTESIAN_POINT ( 'NONE',  ( 19.58040708638629468, 147.7952244890416296, -1.737278836974155416 ) ) ;
#17136=CARTESIAN_POINT ( 'NONE',  ( -0.02964290590182637811, -9.142985105544495283, 0.9735349185509928338 ) ) ;
#17137=CARTESIAN_POINT ( 'NONE',  ( -21.44537552191025753, 145.9698620541949765, -2.253500464710097795 ) ) ;
#17141=CARTESIAN_POINT ( 'NONE',  ( 4.755892522628037966, 104.6144662015434932, 2.421412838250809774 ) ) ;
#17142=CARTESIAN_POINT ( 'NONE',  ( 7.181592176188103416, 121.6016026263613838, -0.5649366106928355169 ) ) ;
#17143=CARTESIAN_POINT ( 'NONE',  ( 7.819172660177973633, 122.4257783361165366, 0.5980713627250896502 ) ) ;
#17144=VERTEX_POINT ( 'NONE', #12126 ) ;
#17145=CARTESIAN_POINT ( 'NONE',  ( -8.285153246922989823, 121.0263440914440736, -1.363535410649704627 ) ) ;
#17146=CARTESIAN_POINT ( 'NONE',  ( 2.197863461560763287, -15.74995721546218519, 5.600911867769769792 ) ) ;
#17148=CARTESIAN_POINT ( 'NONE',  ( -4.590648100572289003, 117.9758294621954064, -0.9228213078436219297 ) ) ;
#17152=CARTESIAN_POINT ( 'NONE',  ( 11.58692091624685183, 123.4149316504530702, 1.682406715187617419 ) ) ;
#17153=CARTESIAN_POINT ( 'NONE',  ( 0.03519895179118932155, 115.7029491485452866, -1.761499482103553449 ) ) ;
#17155=CARTESIAN_POINT ( 'NONE',  ( 17.29948542670041078, 122.7677429521249053, 0.3279718759250788152 ) ) ;
#17156=CARTESIAN_POINT ( 'NONE',  ( -8.041749784432907333, 11.96416136180153345, -2.598976288244244870 ) ) ;
#17157=CARTESIAN_POINT ( 'NONE',  ( 7.635798533888219275, 122.3449549946481056, 0.5106263504299668465 ) ) ;
#17158=CARTESIAN_POINT ( 'NONE',  ( 14.96085986107146226, 121.2513550155162960, -0.6271060280491597139 ) ) ;
#17163=CARTESIAN_POINT ( 'NONE',  ( -18.81756541077873734, 125.3161215262879580, -0.3201835051929644016 ) ) ;
#17164=ORIENTED_EDGE ( 'NONE', *, *, #12808, .T. ) ;
#17165=CARTESIAN_POINT ( 'NONE',  ( -5.198628926520693305, 120.3590328494841231, -0.8315808706636761416 ) ) ;
#17167=ORIENTED_EDGE ( 'NONE', *, *, #26607, .F. ) ;
#17169=CARTESIAN_POINT ( 'NONE',  ( -15.70678031088822202, 147.2451778420852406, -0.7656494529899995349 ) ) ;
#17170=CARTESIAN_POINT ( 'NONE',  ( 4.589616127059429118, -13.46842606041413681, 3.597705605327369494 ) ) ;
#17171=CARTESIAN_POINT ( 'NONE',  ( -1.068372181839257751, 117.3444111807523882, 0.4585463030235088500 ) ) ;
#17173=CARTESIAN_POINT ( 'NONE',  ( 3.725034515352382503, 116.6403000632267464, 0.1520601685204153175 ) ) ;
#17174=VERTEX_POINT ( 'NONE', #25326 ) ;
#17175=CARTESIAN_POINT ( 'NONE',  ( -4.288638401707804526, -7.253218809911426312, -1.756103832032595680 ) ) ;
#17176=CARTESIAN_POINT ( 'NONE',  ( -20.69846590548381826, 152.5542719854981044, -0.4384689201006752857 ) ) ;
#17180=CARTESIAN_POINT ( 'NONE',  ( -4.860571518730761653, 119.0032906492853328, 0.8981773809672630726 ) ) ;
#17181=CARTESIAN_POINT ( 'NONE',  ( 2.776928087254650013, 2.301956178644051221, 3.707541451904531105 ) ) ;
#17182=CARTESIAN_POINT ( 'NONE',  ( 22.23208127788751298, 149.2301036976659816, 1.887777678714757990 ) ) ;
#17184=DIRECTION ( 'NONE',  ( 0.01997839162482749689, 1.040247600000945640E-18, -0.9998004120163610509 ) ) ;
#17185=CARTESIAN_POINT ( 'NONE',  ( 20.75411281516084117, 147.9587796579421308, -1.616985229673752578 ) ) ;
#17186=CARTESIAN_POINT ( 'NONE',  ( 4.587442282481145384, -5.694351208059624803, -0.5507456681084095251 ) ) ;
#17187=CARTESIAN_POINT ( 'NONE',  ( 0.006942562093231309170, 117.0978366787122127, -0.3474341964894883117 ) ) ;
#17190=CARTESIAN_POINT ( 'NONE',  ( -15.68661553393327779, 147.2319784351455780, 0.01612984191841678600 ) ) ;
#17191=CARTESIAN_POINT ( 'NONE',  ( 5.819126084642364916, -14.14507005385615201, 2.709888076677010371 ) ) ;
#17193=CARTESIAN_POINT ( 'NONE',  ( -0.07396841670801596047, 117.3993836134566067, -1.494938445543764427 ) ) ;
#17195=CARTESIAN_POINT ( 'NONE',  ( 12.32670121879455927, 122.4057692182592092, 1.805994760647165576 ) ) ;
#17197=ADVANCED_FACE ( 'NONE', ( #6367 ), #39544, .T. ) ;
#17200=CARTESIAN_POINT ( 'NONE',  ( -22.48855060683877838, 149.3130771379323392, 0.8549704587061034422 ) ) ;
#17201=CARTESIAN_POINT ( 'NONE',  ( -7.252988161461171757, 9.422892264050933164, 4.294140714350721311 ) ) ;
#17202=CARTESIAN_POINT ( 'NONE',  ( 5.176742542608628206, 120.9449653624321144, 0.6121131393098595552 ) ) ;
#17203=DIRECTION ( 'NONE',  ( 0.01997839162482749689, 1.040247600000945640E-18, -0.9998004120163610509 ) ) ;
#17205=CARTESIAN_POINT ( 'NONE',  ( 8.172070396905905199, 117.7057695168643932, -0.3161122371724935376 ) ) ;
#17209=CARTESIAN_POINT ( 'NONE',  ( 5.274109024393328404, 115.7029491485453150, -0.8140283081321303404 ) ) ;
#17212=ADVANCED_FACE ( 'NONE', ( #15775 ), #22470, .T. ) ;
#17213=CARTESIAN_POINT ( 'NONE',  ( -4.486895273669365025, 118.1299698726477914, 0.5326488260592314727 ) ) ;
#17214=CARTESIAN_POINT ( 'NONE',  ( 2.918624193109982112, 107.9147049449184976, -4.333181634890918232 ) ) ;
#17217=CARTESIAN_POINT ( 'NONE',  ( -3.967643248668881295, 119.1178733970733958, -0.9224967296737327516 ) ) ;
#17218=CARTESIAN_POINT ( 'NONE',  ( -5.345964095105384395, 116.9256180743815179, -0.9586058045032990194 ) ) ;
#17220=CARTESIAN_POINT ( 'NONE',  ( 4.585886860456856340, 118.0663496363380318, 0.7419266980658387745 ) ) ;
#17221=CARTESIAN_POINT ( 'NONE',  ( -9.787166303541962264, 124.1138826855306831, -0.8907577946409741543 ) ) ;
#17222=CARTESIAN_POINT ( 'NONE',  ( -0.1695618695486382776, 115.7029491485452866, -1.764636181574767537 ) ) ;
#17223=CARTESIAN_POINT ( 'NONE',  ( 0.4467141430003514491, 117.3993820575490901, -1.478549762435686699 ) ) ;
#17224=CARTESIAN_POINT ( 'NONE',  ( 5.302326897023531771, 116.4520502601644409, -0.8833424955642699139 ) ) ;
#17225=CARTESIAN_POINT ( 'NONE',  ( -16.68619938060346541, 146.1290494286844819, -1.780952809221992172 ) ) ;
#17228=CARTESIAN_POINT ( 'NONE',  ( 8.131384943450600034, 121.0503350093198662, -0.9968526362123016904 ) ) ;
#17229=CARTESIAN_POINT ( 'NONE',  ( -7.784012320790520967, 122.6313477007502115, -0.1555430920740401568 ) ) ;
#17231=CARTESIAN_POINT ( 'NONE',  ( 0.9708930699731092018, 116.8374933757159795, 0.3283832199399772112 ) ) ;
#17232=DIRECTION ( 'NONE',  ( 0.9998004120163609398, 0.000000000000000000, 0.01997839162482749689 ) ) ;
#17233=CARTESIAN_POINT ( 'NONE',  ( 2.233744238265779281, -15.22787141332636374, 5.055619554762198931 ) ) ;
#17234=CARTESIAN_POINT ( 'NONE',  ( -7.478391884465417583, 120.4750020944285609, 1.007254920367567808 ) ) ;
#17235=CARTESIAN_POINT ( 'NONE',  ( -0.9396370176409497565, -11.09013235204027659, 0.2555656002325920051 ) ) ;
#17236=CARTESIAN_POINT ( 'NONE',  ( 0.006534887713546001439, 159.5822087645323393, -0.3270325034788579277 ) ) ;
#17238=CARTESIAN_POINT ( 'NONE',  ( -0.5432096421966324806, 25.39095905668347797, -0.8082079942862561150 ) ) ;
#17241=CARTESIAN_POINT ( 'NONE',  ( 2.249496549248389154, 107.4436264546101967, 4.650814322000806911 ) ) ;
#17243=CARTESIAN_POINT ( 'NONE',  ( -9.732488649496342958, 124.0009531390599591, 0.4956537337270182642 ) ) ;
#17245=CARTESIAN_POINT ( 'NONE',  ( 4.513689648792266418, -13.57929909251434708, 3.776549439516510898 ) ) ;
#17246=CARTESIAN_POINT ( 'NONE',  ( 15.51360955034711253, 150.7699688800196611, -1.541415763164774466 ) ) ;
#17248=CARTESIAN_POINT ( 'NONE',  ( -9.741115574333473859, 120.9522862504114897, -1.586783935194494788 ) ) ;
#17249=CARTESIAN_POINT ( 'NONE',  ( -3.571940676860559272, 104.6144662015457953, 3.260099875215366705 ) ) ;
#17250=CARTESIAN_POINT ( 'NONE',  ( 3.149239739297259533, -13.85570235734440203, 1.885463239856044027 ) ) ;
#17251=CARTESIAN_POINT ( 'NONE',  ( -4.773986132821358197, 117.6391641637075338, -1.128576530690340585 ) ) ;
#17253=CARTESIAN_POINT ( 'NONE',  ( 3.725873884401345926, 121.0563512343167645, -0.03194638937107874971 ) ) ;
#17255=CARTESIAN_POINT ( 'NONE',  ( -2.730960582676723369, 107.1167599116663780, 4.574583874852882204 ) ) ;
#17256=CARTESIAN_POINT ( 'NONE',  ( 2.864732365555376692, 107.5209036112635630, 4.491122542952314944 ) ) ;
#17258=CARTESIAN_POINT ( 'NONE',  ( -3.148524768479886937, 30.89467502894792972, -0.4672404312464801812 ) ) ;
#17259=ADVANCED_FACE ( 'NONE', ( #33878 ), #12962, .T. ) ;
#17261=CARTESIAN_POINT ( 'NONE',  ( 14.80501208800821011, 120.3086691715681695, 0.1403833142216709406 ) ) ;
#17264=CARTESIAN_POINT ( 'NONE',  ( 1.758948546174424976, -15.24573455742719830, 5.911464237579555636 ) ) ;
#17266=CARTESIAN_POINT ( 'NONE',  ( -3.409520279599585368, 31.22297404472999816, -0.3972485071703515946 ) ) ;
#17267=CARTESIAN_POINT ( 'NONE',  ( 9.074718672963324906, 157.1510513929294177, 1.991881423077543012 ) ) ;
#17268=VERTEX_POINT ( 'NONE', #41849 ) ;
#17269=CARTESIAN_POINT ( 'NONE',  ( -4.930748812479134990, 13.88268055242722987, 6.853499169485068876 ) ) ;
#17270=CARTESIAN_POINT ( 'NONE',  ( 2.394128288074550248, 117.2927635608798056, -0.5979285131003549969 ) ) ;
#17271=CARTESIAN_POINT ( 'NONE',  ( -5.854120942168551167, 124.7508695889173111, -0.1197652058513695994 ) ) ;
#17277=CARTESIAN_POINT ( 'NONE',  ( -1.576536484031922480, 10.66345178295009788, -4.350723848753511369 ) ) ;
#17279=CARTESIAN_POINT ( 'NONE',  ( -1.906939736952270925, 106.4592480297309436, -4.997920180712069893 ) ) ;
#17280=CARTESIAN_POINT ( 'NONE',  ( 3.134184212546501591, -13.48855807073397273, 1.578073873303884156 ) ) ;
#17281=CARTESIAN_POINT ( 'NONE',  ( 5.705706447001112736, 123.8402959710505087, 0.07212015369193675030 ) ) ;
#17282=CARTESIAN_POINT ( 'NONE',  ( -15.41192216945103866, 121.3506620944898060, 0.4643526128083735327 ) ) ;
#17283=CARTESIAN_POINT ( 'NONE',  ( 1.733480476724572616, 35.69352191795299234, 2.306000102516378547 ) ) ;
#17286=CARTESIAN_POINT ( 'NONE',  ( -4.980122306282216194, 105.1217006149118163, -1.944304085884134503 ) ) ;
#17288=CARTESIAN_POINT ( 'NONE',  ( 4.642828252855901283, -15.60299999947604910, 2.403246459791627210 ) ) ;
#17289=CARTESIAN_POINT ( 'NONE',  ( -14.15994444794836227, 154.3735777161816429, 1.715400944796409366 ) ) ;
#17290=CARTESIAN_POINT ( 'NONE',  ( -0.5842699607273857954, -4.454521554441356557, 4.585487691134133570 ) ) ;
#17291=ADVANCED_FACE ( 'NONE', ( #12646 ), #12286, .F. ) ;
#17293=DIRECTION ( 'NONE',  ( 0.9998004120163608288, -1.039227405372660929E-20, 0.01997839162482763914 ) ) ;
#17294=CARTESIAN_POINT ( 'NONE',  ( 0.8775954529456102549, 122.2453746293775652, 0.2818696459738750382 ) ) ;
#17295=CARTESIAN_POINT ( 'NONE',  ( -14.77909737591013695, 150.5114039713088516, 1.257293140667801179 ) ) ;
#17297=CARTESIAN_POINT ( 'NONE',  ( 16.46509630982077255, 135.1966315799913900, -1.639354953089778633 ) ) ;
#17298=CARTESIAN_POINT ( 'NONE',  ( -13.54337464129344504, 122.2126086331852974, -1.756000464972328867 ) ) ;
#17300=CARTESIAN_POINT ( 'NONE',  ( 4.168088869111308270, 118.2394494485767780, -0.2219757712405359684 ) ) ;
#17301=CARTESIAN_POINT ( 'NONE',  ( 9.597885446028643130, 124.1734284925964573, -0.3307417288639280528 ) ) ;
#17304=CARTESIAN_POINT ( 'NONE',  ( 1.853042888461218007, -15.33088210119805339, 5.380378780177352382 ) ) ;
#17305=EDGE_CURVE ( 'NONE', #37319, #18840, #32692, .T. ) ;
#17309=CARTESIAN_POINT ( 'NONE',  ( 4.627658001546194555, 13.29687521248714610, 0.05192310334374634212 ) ) ;
#17310=CARTESIAN_POINT ( 'NONE',  ( 5.844382469224909116, 120.7327493588883840, 0.8888191899821259456 ) ) ;
#17311=CARTESIAN_POINT ( 'NONE',  ( -2.672954704825328598, 29.71133030240788386, 0.5376189070171468742 ) ) ;
#17312=CARTESIAN_POINT ( 'NONE',  ( 4.523211737919912601, 7.414965188139293950, 0.9565071382433593117 ) ) ;
#17313=CARTESIAN_POINT ( 'NONE',  ( 7.044165191775438650, 122.0728772437221323, 0.1705051815768212631 ) ) ;
#17314=CARTESIAN_POINT ( 'NONE',  ( -5.212194349666299686, 114.7155706869413052, 1.248445758411629969 ) ) ;
#17316=CARTESIAN_POINT ( 'NONE',  ( -2.168002701389783571, 116.2668357660312068, -0.2200461739608741141 ) ) ;
#17319=CARTESIAN_POINT ( 'NONE',  ( 1.868457900240731773, -15.55086107261450223, 5.421086310357070559 ) ) ;
#17321=CARTESIAN_POINT ( 'NONE',  ( 3.617035938018385632, 9.361278981710560387, -7.607506385697127449 ) ) ;
#17325=CARTESIAN_POINT ( 'NONE',  ( 0.01331772328568395919, 119.9741034315943864, -0.6664733318052135091 ) ) ;
#17326=CARTESIAN_POINT ( 'NONE',  ( -23.08840689075984898, 149.5685596498530288, 0.1330139495868551958 ) ) ;
#17329=CARTESIAN_POINT ( 'NONE',  ( -6.986578011841114488, 121.9508038282781968, -0.1709446046045101919 ) ) ;
#17332=CARTESIAN_POINT ( 'NONE',  ( -5.964965236245769908, 155.3820107761045790, -0.1591880423168908210 ) ) ;
#17333=CARTESIAN_POINT ( 'NONE',  ( 2.110383923269381512, -15.54165552008020335, 5.912460941884730481 ) ) ;
#17334=CARTESIAN_POINT ( 'NONE',  ( -14.20167894085462734, 122.0820592118662091, 1.087754808798858441 ) ) ;
#17335=CARTESIAN_POINT ( 'NONE',  ( 20.19069946793830894, 128.9119615565081176, 0.7900021088785407208 ) ) ;
#17336=CARTESIAN_POINT ( 'NONE',  ( 2.864695407350143164, 156.1076416471755977, 0.1877241569260537923 ) ) ;
#17338=CARTESIAN_POINT ( 'NONE',  ( 0.9751244372034794106, -10.72340290332181567, 0.05698045496536860433 ) ) ;
#17339=CARTESIAN_POINT ( 'NONE',  ( -23.37685013984168236, 146.7932648766621639, -0.8013420975766073484 ) ) ;
#17341=CARTESIAN_POINT ( 'NONE',  ( 4.756814333351318425, 117.4032681585794791, 1.206529664789174339 ) ) ;
#17343=CARTESIAN_POINT ( 'NONE',  ( -5.553480690675685949, 116.8696988207415899, 0.2846251051479010696 ) ) ;
#17344=CARTESIAN_POINT ( 'NONE',  ( -11.41761608106104475, 123.3954635094115702, 1.178011644471332442 ) ) ;
#17346=CARTESIAN_POINT ( 'NONE',  ( 20.70190595857150129, 149.9184980045912425, 2.291194810033231111 ) ) ;
#17347=CARTESIAN_POINT ( 'NONE',  ( 12.27894764211867695, 122.3148578561100948, -1.306772475271723799 ) ) ;
#17348=CARTESIAN_POINT ( 'NONE',  ( -0.9608913863540493594, -11.74124177384809542, -0.1559992898937096195 ) ) ;
#17349=CARTESIAN_POINT ( 'NONE',  ( -16.48954130525400075, 125.2933801378020888, -1.785035858276808884 ) ) ;
#17351=CARTESIAN_POINT ( 'NONE',  ( -3.223859242259529356, 50.63946620154572997, 1.416295642791933984 ) ) ;
#17352=CARTESIAN_POINT ( 'NONE',  ( 9.244484035386456355, 123.0263237342149978, -0.6646791600263457500 ) ) ;
#17353=CARTESIAN_POINT ( 'NONE',  ( -4.911102353720303348, 117.7098496952192477, 0.7294018754363704726 ) ) ;
#17356=CARTESIAN_POINT ( 'NONE',  ( -6.586386431196567415, 120.2999964176511014, -1.183541128842728662 ) ) ;
#17357=CARTESIAN_POINT ( 'NONE',  ( 4.827739681024636909, -15.50696398224166117, 1.464145260785405522 ) ) ;
#17359=CARTESIAN_POINT ( 'NONE',  ( -4.509696226152874132, 118.1210427847854163, -0.6597157338689267903 ) ) ;
#17360=EDGE_CURVE ( 'NONE', #23764, #5065, #38800, .T. ) ;
#17362=CARTESIAN_POINT ( 'NONE',  ( 4.113055949110636433, 118.2429491485453354, 0.3449990421833045162 ) ) ;
#17363=CARTESIAN_POINT ( 'NONE',  ( 16.91058881216872223, 149.6223975874448229, 2.301385465272872910 ) ) ;
#17364=CARTESIAN_POINT ( 'NONE',  ( -5.212520885064538589, 31.45212241211192605, -0.4657032193360505778 ) ) ;
#17365=CARTESIAN_POINT ( 'NONE',  ( 8.078287538471617069, 158.6595088495342338, 0.1614234102745199240 ) ) ;
#17366=CARTESIAN_POINT ( 'NONE',  ( -7.328769482851726025, 13.23335216599729947, 4.212906450523355772 ) ) ;
#17367=CARTESIAN_POINT ( 'NONE',  ( 15.38106487260171562, 148.0444422243178337, 0.8962548396073237722 ) ) ;
#17368=CARTESIAN_POINT ( 'NONE',  ( 16.34457059127843692, 122.7783120765077030, -0.5554794724330635036 ) ) ;
#17372=CARTESIAN_POINT ( 'NONE',  ( -5.789608264049685538, 116.9447284183608389, -0.03249775470882597384 ) ) ;
#17376=CARTESIAN_POINT ( 'NONE',  ( 6.649258020143044234, 120.6764540553069196, -0.8254125331649241337 ) ) ;
#17379=CARTESIAN_POINT ( 'NONE',  ( -5.332935397695337087, 104.6144662015457243, -0.1065647409268298818 ) ) ;
#17380=CARTESIAN_POINT ( 'NONE',  ( -9.821648630411685232, 124.8790005272986861, -0.5336917924355369935 ) ) ;
#17381=CARTESIAN_POINT ( 'NONE',  ( 5.004296470405577679, -11.88282826624689825, 0.9770688040177184508 ) ) ;
#17382=CARTESIAN_POINT ( 'NONE',  ( -3.000642688540978487, 117.3922842568077698, 0.5420849065376541764 ) ) ;
#17384=CARTESIAN_POINT ( 'NONE',  ( 22.83278390340148789, 150.4073064562084880, 0.5330863269314419783 ) ) ;
#17386=CARTESIAN_POINT ( 'NONE',  ( 3.895047602890354010, -2.730319773039217690, 2.488009491782988469 ) ) ;
#17387=CARTESIAN_POINT ( 'NONE',  ( 0.0002511744760183973928, 116.4254662015457171, -0.01256979787922174636 ) ) ;
#17390=ORIENTED_EDGE ( 'NONE', *, *, #14746, .F. ) ;
#17391=CARTESIAN_POINT ( 'NONE',  ( -8.137098263763151706, 121.0228228821670911, 1.007425014759447013 ) ) ;
#17392=CARTESIAN_POINT ( 'NONE',  ( 1.861163356255745915, -7.643417679262992870, 4.233688895527200735 ) ) ;
#17393=CARTESIAN_POINT ( 'NONE',  ( 1.049200951577147878, 117.3444111807523882, 0.5008604537731423667 ) ) ;
#17395=CARTESIAN_POINT ( 'NONE',  ( 3.150705211532580652, 118.1710492231644736, -0.7255832847742738068 ) ) ;
#17396=CARTESIAN_POINT ( 'NONE',  ( 4.406646451516359697, -6.344046434980911364, 1.391598188203984288 ) ) ;
#17397=CARTESIAN_POINT ( 'NONE',  ( -17.90421410101181721, 154.0540368679750998, -1.594113676345344732 ) ) ;
#17399=CARTESIAN_POINT ( 'NONE',  ( -9.115521395012626371, 123.9337093609977529, 0.04715588286475777546 ) ) ;
#17400=CARTESIAN_POINT ( 'NONE',  ( 3.037190435423921642, -15.45437603076259236, 5.639675387367293347 ) ) ;
#17402=CARTESIAN_POINT ( 'NONE',  ( -0.3314327031344502239, 118.1651004622152783, -0.8947675711121312325 ) ) ;
#17404=VERTEX_POINT ( 'NONE', #23046 ) ;
#17405=CARTESIAN_POINT ( 'NONE',  ( 12.24350972434449147, 123.0735437985678971, 1.806721486477698591 ) ) ;
#17406=DIRECTION ( 'NONE',  ( 0.9998004120163609398, 0.000000000000000000, 0.01997839162482749689 ) ) ;
#17407=CARTESIAN_POINT ( 'NONE',  ( -6.515206564940426254E-14, 69.43546620154573645, -8.744632320494937509E-18 ) ) ;
#17408=CARTESIAN_POINT ( 'NONE',  ( -8.102197167285096313, 117.9965348323767671, 0.5618759090088268904 ) ) ;
#17409=CARTESIAN_POINT ( 'NONE',  ( -6.209159877377784298, 7.473591768893033560, -5.687189600455027971 ) ) ;
#17410=CARTESIAN_POINT ( 'NONE',  ( 15.67318563778015061, 143.6801599334541208, 1.294273616026768492 ) ) ;
#17412=CARTESIAN_POINT ( 'NONE',  ( 22.94521658075144188, 142.4877946823990271, -0.4044642804735132380 ) ) ;
#17415=FILL_AREA_STYLE ('',( #34459 ) ) ;
#17418=CARTESIAN_POINT ( 'NONE',  ( -4.514281675679005623, 118.1172348940403367, 0.5455092187523593594 ) ) ;
#17419=CARTESIAN_POINT ( 'NONE',  ( 2.730790556997842788, 107.1172351171862118, -4.574511410390974753 ) ) ;
#17422=CARTESIAN_POINT ( 'NONE',  ( 6.160900166467479622, 119.5651146182915738, -1.008937348957311242 ) ) ;
#17423=CARTESIAN_POINT ( 'NONE',  ( -5.229314312453288593, 116.0897965414613964, -1.239798673375258842 ) ) ;
#17424=CARTESIAN_POINT ( 'NONE',  ( 4.638744064954714474, 118.0266105220047024, 0.7608683655302644899 ) ) ;
#17425=CARTESIAN_POINT ( 'NONE',  ( -10.86813797462349740, 153.1125297277760069, -1.236783938685797279 ) ) ;
#17426=CARTESIAN_POINT ( 'NONE',  ( -0.6181410509038570700, 115.7031374082930455, -1.759523019197690274 ) ) ;
#17427=CARTESIAN_POINT ( 'NONE',  ( 0.5464446624898103844, 117.9496048909628456, -1.385902395265538267 ) ) ;
#17429=CARTESIAN_POINT ( 'NONE',  ( -3.685501180670149424, 30.72893705507438611, -2.802369389919810772 ) ) ;
#17430=CARTESIAN_POINT ( 'NONE',  ( -5.849275934571582347, 120.8872308857076519, -0.8185814695607154245 ) ) ;
#17431=CARTESIAN_POINT ( 'NONE',  ( 4.678875543802746506, 116.0444662015457737, -3.608683038041131663 ) ) ;
#17433=CARTESIAN_POINT ( 'NONE',  ( 8.764399874728660222, 117.8902759020840563, -0.3181776094565843538 ) ) ;
#17434=CARTESIAN_POINT ( 'NONE',  ( -4.633229131069707130, 121.2001890545385976, 0.01432855803707623957 ) ) ;
#17437=CARTESIAN_POINT ( 'NONE',  ( 19.64956762203114593, 128.7577553591919752, 1.229466013835583738 ) ) ;
#17439=CARTESIAN_POINT ( 'NONE',  ( 3.263309282894114371, -14.66069363451780205, 2.445366243406764006 ) ) ;
#17440=CARTESIAN_POINT ( 'NONE',  ( -16.81178602683906220, 135.2943057719725459, 1.678525023343173661 ) ) ;
#17441=CARTESIAN_POINT ( 'NONE',  ( -0.3089908097382615959, -9.589635095254870123, 0.9269408180416041088 ) ) ;
#17442=CARTESIAN_POINT ( 'NONE',  ( 0.009748065369120871224, 159.5507987164374981, -0.4878330526048096361 ) ) ;
#17443=CARTESIAN_POINT ( 'NONE',  ( -0.8611515851325071136, 16.54815110656625166, -0.4551624184793268135 ) ) ;
#17446=CARTESIAN_POINT ( 'NONE',  ( 5.733418603097385713, 118.4539739381501988, 0.6622650514401648980 ) ) ;
#17447=CARTESIAN_POINT ( 'NONE',  ( -14.68012063964734004, 139.2174805014774392, 0.5696158742132094721 ) ) ;
#17448=CARTESIAN_POINT ( 'NONE',  ( 2.226119369219526689, -15.10343733042141068, 5.886803469647748699 ) ) ;
#17449=CARTESIAN_POINT ( 'NONE',  ( 17.30559516374531626, 146.8699245690979751, -1.364999074652126110 ) ) ;
#17451=CARTESIAN_POINT ( 'NONE',  ( -10.57181108402536829, 155.7851685111067184, -2.170362527570921962 ) ) ;
#17452=CARTESIAN_POINT ( 'NONE',  ( 2.500242650891530971, 104.6144662015457527, 4.137678032133335293 ) ) ;
#17453=ADVANCED_FACE ( 'NONE', ( #29675 ), #6843, .F. ) ;
#17454=CARTESIAN_POINT ( 'NONE',  ( 3.134184212546501591, -13.48855807073397273, 1.578073873303884156 ) ) ;
#17455=CARTESIAN_POINT ( 'NONE',  ( -4.942124793971827579, 117.4083539704047183, -1.067544502694063979 ) ) ;
#17457=CARTESIAN_POINT ( 'NONE',  ( 9.007539097974285980, 123.9742709865185191, 0.1460878630902627262 ) ) ;
#17458=ORIENTED_EDGE ( 'NONE', *, *, #10202, .F. ) ;
#17459=CARTESIAN_POINT ( 'NONE',  ( 13.40750253236522127, 122.4565580348552913, 1.800089891214285531 ) ) ;
#17460=CARTESIAN_POINT ( 'NONE',  ( 2.321315766260381608, 107.3040393085556445, 4.704548974857680754 ) ) ;
#17461=( BOUNDED_CURVE ( )  B_SPLINE_CURVE ( 1, ( #18474, #5733 ),
 .UNSPECIFIED., .F., .T. ) 
 B_SPLINE_CURVE_WITH_KNOTS ( ( 2, 2 ),
 ( 0.04437134223310085224, 0.9700710138315444819 ),
 .UNSPECIFIED. ) 
 CURVE ( )  GEOMETRIC_REPRESENTATION_ITEM ( )  RATIONAL_B_SPLINE_CURVE ( ( 0.9983552002448072837, 0.9999484871150284837 ) ) 
 REPRESENTATION_ITEM ( '' )  );
#17465=CARTESIAN_POINT ( 'NONE',  ( 8.048392397359023676, 158.6767594643193604, -0.003330354478298842586 ) ) ;
#17467=CARTESIAN_POINT ( 'NONE',  ( 1.667695940653114883, -15.52399890817349259, 5.699764172519937055 ) ) ;
#17469=CARTESIAN_POINT ( 'NONE',  ( 2.912792906754999134, 38.59631781016217644, -1.173005823891349220 ) ) ;
#17470=CARTESIAN_POINT ( 'NONE',  ( 1.154696340448265524, 118.0995038195805904, 0.6495305470935905934 ) ) ;
#17472=CARTESIAN_POINT ( 'NONE',  ( 8.403146708066456583, 17.13307930518084632, 0.5673920214783956251 ) ) ;
#17473=CARTESIAN_POINT ( 'NONE',  ( -2.367130307693360081, 117.2935156952702016, -0.6933524696228330342 ) ) ;
#17474=CARTESIAN_POINT ( 'NONE',  ( -3.776803835208340843, 121.1194860566822626, -0.3725146398702259276 ) ) ;
#17476=CARTESIAN_POINT ( 'NONE',  ( -4.703828842912097130, 114.7515309228077030, -1.852197097316329311 ) ) ;
#17477=CARTESIAN_POINT ( 'NONE',  ( -0.005880675322317568607, 122.2435587914035295, 0.2942930402745070340 ) ) ;
#17479=CARTESIAN_POINT ( 'NONE',  ( 2.801506786573456420, 9.139157206818806500, -3.684590140147142368 ) ) ;
#17482=CARTESIAN_POINT ( 'NONE',  ( 3.334874478900925254, -13.11215654211414439, 1.739483084651320066 ) ) ;
#17483=EDGE_CURVE ( 'NONE', #35734, #14389, #22264, .T. ) ;
#17484=CARTESIAN_POINT ( 'NONE',  ( 4.141015252736647057, 122.5143120247930142, -0.07252455213604046269 ) ) ;
#17485=CARTESIAN_POINT ( 'NONE',  ( 0.6408964823745235684, 37.72669835237458358, 1.782185992127281793 ) ) ;
#17488=VERTEX_POINT ( 'NONE', #6682 ) ;
#17489=CARTESIAN_POINT ( 'NONE',  ( -4.831300404072987220, 104.6144662015457811, -0.2179056330698100619 ) ) ;
#17490=CARTESIAN_POINT ( 'NONE',  ( 1.930844028328122519, -15.65960119559217745, 5.531553210582124791 ) ) ;
#17491=CARTESIAN_POINT ( 'NONE',  ( -19.68629672748976489, 145.2539617268756729, 1.742627101631720077 ) ) ;
#17492=CARTESIAN_POINT ( 'NONE',  ( 0.6989348986720191892, -4.029744825116962303, 4.573446973323917142 ) ) ;
#17493=VERTEX_POINT ( 'NONE', #3710 ) ;
#17496=CARTESIAN_POINT ( 'NONE',  ( 0.3557171951617904004, 107.2171362991012842, 4.792661424475801901 ) ) ;
#17497=CARTESIAN_POINT ( 'NONE',  ( -9.956456675072866247, 154.0333045108203009, 1.106646445589350325 ) ) ;
#17499=CARTESIAN_POINT ( 'NONE',  ( 15.87040186760622262, 150.9007765090757971, -1.629155861667390681 ) ) ;
#17500=CARTESIAN_POINT ( 'NONE',  ( -20.64857576366725667, 148.2641884961211076, -2.442776014760721370 ) ) ;
#17502=ADVANCED_FACE ( 'NONE', ( #19648 ), #26259, .T. ) ;
#17503=CARTESIAN_POINT ( 'NONE',  ( 4.280713456108180992, 118.2124846597233869, -0.3641107394327984803 ) ) ;
#17504=CARTESIAN_POINT ( 'NONE',  ( 0.6165924928997299492, 120.7136710450757988, -0.2143668442300579458 ) ) ;
#17506=CARTESIAN_POINT ( 'NONE',  ( 3.392805262616394035, -14.86080682751021698, 1.607197643132475040 ) ) ;
#17511=CARTESIAN_POINT ( 'NONE',  ( 4.099978103716023448, 4.450953565018914482, -2.131961072590273343 ) ) ;
#17512=CARTESIAN_POINT ( 'NONE',  ( 10.56433624517442738, 123.7931190674884050, 1.348085882050163553 ) ) ;
#17513=CARTESIAN_POINT ( 'NONE',  ( -1.879194370357706756, 31.42354579518680424, 3.981814511614890417 ) ) ;
#17514=CARTESIAN_POINT ( 'NONE',  ( -6.279970060868473425, 120.0898888515776264, 0.2014705954985339942 ) ) ;
#17515=CARTESIAN_POINT ( 'NONE',  ( 2.801506786573456420, 9.139157206818806500, -3.684590140147142368 ) ) ;
#17516=CARTESIAN_POINT ( 'NONE',  ( 11.84172335778361251, 151.9972573545839225, 0.3576891575424543945 ) ) ;
#17519=CARTESIAN_POINT ( 'NONE',  ( 2.168201787175106698, 116.3152343823800265, -0.1794994579355096709 ) ) ;
#17520=CARTESIAN_POINT ( 'NONE',  ( 0.002462548249238089102, 123.7646714092002611, -0.1232359841710924941 ) ) ;
#17522=CARTESIAN_POINT ( 'NONE',  ( -2.005270804404902574, 106.7492432543866130, 4.871661368785221491 ) ) ;
#17524=CARTESIAN_POINT ( 'NONE',  ( -6.252972126910993467, 3.963778981710710969, 5.644239715445565686 ) ) ;
#17528=CARTESIAN_POINT ( 'NONE',  ( 0.0002200197269684159480, 124.8375573595198063, -0.01101068683960094302 ) ) ;
#17529=CARTESIAN_POINT ( 'NONE',  ( -0.3220477894875805047, 116.6413645472259617, 0.1880332438949533225 ) ) ;
#17532=CARTESIAN_POINT ( 'NONE',  ( -7.784332312133520837, 122.6279626997426533, -0.1742668636873402899 ) ) ;
#17534=ORIENTED_EDGE ( 'NONE', *, *, #32590, .F. ) ;
#17536=CARTESIAN_POINT ( 'NONE',  ( -9.501049366036612653, 124.7903798759050460, -0.1436111869418686404 ) ) ;
#17537=CARTESIAN_POINT ( 'NONE',  ( 5.253367374056280070, -14.88852847978991356, 3.689182801501961428 ) ) ;
#17538=CARTESIAN_POINT ( 'NONE',  ( -20.86711222142712074, 145.7124547906547889, 1.576573076165909360 ) ) ;
#17539=CARTESIAN_POINT ( 'NONE',  ( -0.004355829920669731722, 116.7171338949676738, 0.2179835409713598571 ) ) ;
#17541=CARTESIAN_POINT ( 'NONE',  ( 20.00278215841951379, 152.4248492066682559, -0.8711105393690438126 ) ) ;
#17543=CARTESIAN_POINT ( 'NONE',  ( -23.30140632484793528, 142.7201128741078833, -0.7978754358820899784 ) ) ;
#17547=CARTESIAN_POINT ( 'NONE',  ( -5.556907610490653404, 116.8023684160186519, 0.1994680161719879219 ) ) ;
#17548=CARTESIAN_POINT ( 'NONE',  ( -11.30191013352091467, 123.2561760277034324, 1.170227508207775324 ) ) ;
#17550=CARTESIAN_POINT ( 'NONE',  ( 11.12579521122935944, 121.4866960210745503, -1.254162869557706061 ) ) ;
#17551=CARTESIAN_POINT ( 'NONE',  ( 0.7724745873405186591, -15.29971413243098688, -0.5873327843062005060 ) ) ;
#17552=CARTESIAN_POINT ( 'NONE',  ( -6.794677088231817486, 118.4250403807481575, -1.128628347181275693 ) ) ;
#17554=CARTESIAN_POINT ( 'NONE',  ( 14.29925251870365699, 150.3563008155378213, -0.9573768768026650333 ) ) ;
#17556=CARTESIAN_POINT ( 'NONE',  ( -11.83539255247756117, 152.0195595274622349, -0.2364993098673504601 ) ) ;
#17558=CARTESIAN_POINT ( 'NONE',  ( -13.11083847086530874, 125.9194590699508893, -1.866409529942264944 ) ) ;
#17559=CARTESIAN_POINT ( 'NONE',  ( 2.110750219194173827, -15.67940412490098723, 5.433654451060461632 ) ) ;
#17560=DIRECTION ( 'NONE',  ( 4.017660918040594346E-17, -1.000000000000000000, -2.376309959284834438E-19 ) ) ;
#17561=CARTESIAN_POINT ( 'NONE',  ( -4.299846727470445273, 118.2124326582062963, -0.4976427630063417484 ) ) ;
#17564=CARTESIAN_POINT ( 'NONE',  ( 10.84669103489406972, 122.6724665872831679, 1.607685377936340032 ) ) ;
#17565=DIRECTION ( 'NONE',  ( -0.9998004120163609398, 0.000000000000000000, -0.01997839162482749689 ) ) ;
#17566=CARTESIAN_POINT ( 'NONE',  ( 4.713631738767327661, 116.7564862437112794, 0.09418957996065577265 ) ) ;
#17567=CARTESIAN_POINT ( 'NONE',  ( -2.166771814436331045, 10.43868160547798674, -8.139002505017437272 ) ) ;
#17568=CARTESIAN_POINT ( 'NONE',  ( 5.248704524870055010, 121.2670714900434206, 0.3264022214948026912 ) ) ;
#17569=EDGE_CURVE ( 'NONE', #1073, #16433, #18719, .T. ) ;
#17570=CARTESIAN_POINT ( 'NONE',  ( 19.39512251848550761, 128.7092500879292345, -0.6293422422100684033 ) ) ;
#17572=CARTESIAN_POINT ( 'NONE',  ( 2.791705395246603327, 115.6909491485452577, 1.685629878066634113 ) ) ;
#17574=CARTESIAN_POINT ( 'NONE',  ( -22.83585328881722276, 150.4073064562084880, -0.3794817294851793865 ) ) ;
#17577=CARTESIAN_POINT ( 'NONE',  ( -5.923576811503439288, 121.3842984696033653, -0.3127082814038080194 ) ) ;
#17578=FACE_OUTER_BOUND ( 'NONE', #27858, .T. ) ;
#17580=CARTESIAN_POINT ( 'NONE',  ( 0.2889217817199783434, 115.7029882075844540, -1.754376360704741122 ) ) ;
#17581=CARTESIAN_POINT ( 'NONE',  ( -8.575029486087489161, 123.3373102669514765, -0.3234659723512184337 ) ) ;
#17582=CARTESIAN_POINT ( 'NONE',  ( 4.994336218630399671, -12.17445384341683834, 1.469335147697719890 ) ) ;
#17583=CARTESIAN_POINT ( 'NONE',  ( -21.43028413922730024, 149.8571540977637255, 1.275288106631634832 ) ) ;
#17585=CARTESIAN_POINT ( 'NONE',  ( 23.34655412193302837, 148.8653451956335516, 0.6207958181910346873 ) ) ;
#17587=ORIENTED_EDGE ( 'NONE', *, *, #35079, .T. ) ;
#17588=CARTESIAN_POINT ( 'NONE',  ( 4.349802767100347189, -10.92635770930747796, -1.576909098649299512 ) ) ;
#17589=CARTESIAN_POINT ( 'NONE',  ( -3.302029177305334073, 159.4671159221996959, -0.06598240135525369754 ) ) ;
#17590=CARTESIAN_POINT ( 'NONE',  ( -6.707568152035292797E-14, 117.3144662015457271, 2.632902133564923224E-18 ) ) ;
#17593=ORIENTED_EDGE ( 'NONE', *, *, #2212, .F. ) ;
#17594=CARTESIAN_POINT ( 'NONE',  ( 8.208067840267224469, 120.4389322928407324, 1.432930303473133993 ) ) ;
#17595=CARTESIAN_POINT ( 'NONE',  ( -4.434453077421578904, -10.21728329253013179, 1.368390957472948921 ) ) ;
#17596=CARTESIAN_POINT ( 'NONE',  ( 21.87689675406251411, 150.0588410196355937, 1.874897916013938737 ) ) ;
#17598=CARTESIAN_POINT ( 'NONE',  ( 20.72967856921734864, 148.2641884961211076, -1.615940018417327373 ) ) ;
#17599=CARTESIAN_POINT ( 'NONE',  ( -4.598078022480850180, -10.86695742004451404, -0.5832510952623800593 ) ) ;
#17600=CARTESIAN_POINT ( 'NONE',  ( -14.71083544318262071, 121.0688405154646858, -1.213083844406487977 ) ) ;
#17603=CARTESIAN_POINT ( 'NONE',  ( -11.97065782033005554, 130.4318746828361100, -0.03484989721007628743 ) ) ;
#17605=CARTESIAN_POINT ( 'NONE',  ( 4.211475536325941071, -15.04083557003654903, 4.983330352733777779 ) ) ;
#17608=CARTESIAN_POINT ( 'NONE',  ( -0.4814620969468332845, 118.1651003975972998, -0.8929907497847521247 ) ) ;
#17610=CARTESIAN_POINT ( 'NONE',  ( 9.741115574333344185, 120.9522862504114897, 1.586783935194494788 ) ) ;
#17612=DIRECTION ( 'NONE',  ( 0.9998004120163608288, 0.000000000000000000, 0.01997839162482749342 ) ) ;
#17613=CARTESIAN_POINT ( 'NONE',  ( -14.55782549726419894, 156.0472725025049954, 0.8788902920476678871 ) ) ;
#17614=CARTESIAN_POINT ( 'NONE',  ( -4.386519595447357922, 0.5779702600499575516, 7.231359419481246498 ) ) ;
#17615=CARTESIAN_POINT ( 'NONE',  ( 12.64766777886143068, 130.7634385742845780, 1.140803344710751510 ) ) ;
#17617=CARTESIAN_POINT ( 'NONE',  ( 13.30049347609353561, 119.7426348059052685, -0.3046699512218788430 ) ) ;
#17620=CARTESIAN_POINT ( 'NONE',  ( -6.484670282503085616E-14, 71.97546620154574271, 3.533028205012241021E-29 ) ) ;
#17624=CARTESIAN_POINT ( 'NONE',  ( -4.158059140961544387, 118.2391353841180432, 0.2335865895784110802 ) ) ;
#17625=LINE ( 'NONE', #40649, #3660 ) ;
#17629=CARTESIAN_POINT ( 'NONE',  ( -8.253346482873464396, 120.2166765077018340, -1.447820397028310779 ) ) ;
#17630=AXIS2_PLACEMENT_3D ( 'NONE', #5561, #31738, #41552 ) ;
#17631=CARTESIAN_POINT ( 'NONE',  ( -4.762298162519812195, 112.7561542417671916, -2.571201254457596175 ) ) ;
#17632=CARTESIAN_POINT ( 'NONE',  ( 4.233096343644137782, 118.2249610142085032, 0.4811101450830501669 ) ) ;
#17633=CARTESIAN_POINT ( 'NONE',  ( -15.67318563778028206, 143.6801599334541208, -1.294273616026768270 ) ) ;
#17634=CARTESIAN_POINT ( 'NONE',  ( 0.6048459695572244721, 117.3993834314627236, -1.469644289381657254 ) ) ;
#17636=CARTESIAN_POINT ( 'NONE',  ( 0.1065646865914872399, 105.8844662015456777, -5.332932678536313809 ) ) ;
#17637=CARTESIAN_POINT ( 'NONE',  ( -3.381852828898228136, 156.3978305292817481, -1.289121224278521938 ) ) ;
#17638=CARTESIAN_POINT ( 'NONE',  ( -0.1561264326628848120, 116.0444662015457027, 6.158975241439932802 ) ) ;
#17641=CARTESIAN_POINT ( 'NONE',  ( -15.76305951754530099, 145.8995318477080332, -0.1132554252373959985 ) ) ;
#17643=CARTESIAN_POINT ( 'NONE',  ( 11.33669861507955190, 118.9804978796424706, 0.9069902030348427902 ) ) ;
#17645=CARTESIAN_POINT ( 'NONE',  ( 2.667920334613889555, -13.82128762729334426, -0.01087480101406306660 ) ) ;
#17646=CARTESIAN_POINT ( 'NONE',  ( 21.43028413922716879, 149.8571540977637255, -1.275288106631634610 ) ) ;
#17647=CARTESIAN_POINT ( 'NONE',  ( -0.9814465556261140478, 157.4778559999684830, 1.561959177316862180 ) ) ;
#17648=CARTESIAN_POINT ( 'NONE',  ( -0.9543378889979354796, -1.596235181177088291, 0.1924800533990675688 ) ) ;
#17649=CARTESIAN_POINT ( 'NONE',  ( 0.005431400947611031600, 116.8580640273661118, -0.2718095133625907933 ) ) ;
#17650=CARTESIAN_POINT ( 'NONE',  ( 0.9751022921854990422, 22.16746322748675624, -0.05045228706074462999 ) ) ;
#17654=CARTESIAN_POINT ( 'NONE',  ( -11.75634259954081529, 128.3321206738457647, 0.5010001888332091813 ) ) ;
#17655=CARTESIAN_POINT ( 'NONE',  ( 2.069070256058832324, -15.20480250118845511, 5.930115229603830862 ) ) ;
#17656=CARTESIAN_POINT ( 'NONE',  ( 0.5698427240850039155, 120.0661220204379305, -0.4260729765348976184 ) ) ;
#17658=DIRECTION ( 'NONE',  ( -4.017660918040594346E-17, 1.000000000000000000, 2.376309959284834438E-19 ) ) ;
#17659=CARTESIAN_POINT ( 'NONE',  ( 3.394644278243977187, -13.41358914320520057, 2.304069835958892032 ) ) ;
#17660=CARTESIAN_POINT ( 'NONE',  ( -5.176850267262477878, 31.60528704468920580, -0.07969122161898611889 ) ) ;
#17661=CARTESIAN_POINT ( 'NONE',  ( 0.6477285649443610405, 156.3042436901572216, -0.05974520555407228373 ) ) ;
#17662=CIRCLE ( 'NONE', #31965, 5.588000000000006295 ) ;
#17664=CARTESIAN_POINT ( 'NONE',  ( 19.98568676637946950, 149.3093937917295762, 2.465107550769984890 ) ) ;
#17665=CARTESIAN_POINT ( 'NONE',  ( 4.943369476187105427, 113.9634657096399053, 2.116106984914523093 ) ) ;
#17668=CARTESIAN_POINT ( 'NONE',  ( 0.02768730785345232051, 158.9256195073445213, -1.385586103196075447 ) ) ;
#17669=CARTESIAN_POINT ( 'NONE',  ( 15.79392588796402208, 121.0087326939336378, 0.08323308591264581835 ) ) ;
#17671=CARTESIAN_POINT ( 'NONE',  ( 1.848236747766272892, -15.62973196022113243, 5.883794544018126516 ) ) ;
#17672=DIRECTION ( 'NONE',  ( 4.017660918040594346E-17, -1.000000000000000000, -2.376309959284834438E-19 ) ) ;
#17673=CARTESIAN_POINT ( 'NONE',  ( 1.122158211225881885, 34.81801111161350804, -0.09678150280622686841 ) ) ;
#17674=CARTESIAN_POINT ( 'NONE',  ( 0.4162271216348931713, 118.1045761740670201, 0.5784513839558712567 ) ) ;
#17675=ORIENTED_EDGE ( 'NONE', *, *, #40687, .T. ) ;
#17676=CARTESIAN_POINT ( 'NONE',  ( -8.291425676780491472, 12.16085651096402032, -1.523321141447528948 ) ) ;
#17677=CARTESIAN_POINT ( 'NONE',  ( -8.672386296370172332, 118.2230072205180420, -0.9366548366208437004 ) ) ;
#17678=CARTESIAN_POINT ( 'NONE',  ( -3.448667622495882323, 119.7720183225874138, -0.5479595714127596384 ) ) ;
#17679=CARTESIAN_POINT ( 'NONE',  ( 4.825270798805025407, 117.7346728073316626, 1.017784339641811808 ) ) ;
#17681=CARTESIAN_POINT ( 'NONE',  ( -4.423373769213096551, 104.6144662015457243, 1.938597605103610011 ) ) ;
#17682=CARTESIAN_POINT ( 'NONE',  ( -1.544744425833544099, 4.816215111148435923, 4.377641278133862279 ) ) ;
#17684=CARTESIAN_POINT ( 'NONE',  ( -2.780279277094420021, 107.4064198780910431, -4.544082669632513394 ) ) ;
#17685=CARTESIAN_POINT ( 'NONE',  ( 3.815374714676033729, -13.42234902974577615, 3.291045305163978085 ) ) ;
#17686=CARTESIAN_POINT ( 'NONE',  ( 0.2613516939665402328, 106.0087397856094356, -5.279363957283110587 ) ) ;
#17687=AXIS2_PLACEMENT_3D ( 'NONE', #33253, #20436, #10862 ) ;
#17688=CARTESIAN_POINT ( 'NONE',  ( 2.461214384022098134, 39.20946620154573026, 1.319434448097693169 ) ) ;
#17689=CARTESIAN_POINT ( 'NONE',  ( -2.055040306894160729, 115.7029326251217185, 1.635618938382796816 ) ) ;
#17691=CARTESIAN_POINT ( 'NONE',  ( -5.255091509764169722, 104.6144662015501012, -0.9306984194723886272 ) ) ;
#17692=CARTESIAN_POINT ( 'NONE',  ( 5.310739065812000170, -15.29705283487872691, 0.1354967992945097788 ) ) ;
#17693=CARTESIAN_POINT ( 'NONE',  ( -13.71253074539983530, 123.6869008171703541, 1.368039988124472695 ) ) ;
#17694=CARTESIAN_POINT ( 'NONE',  ( -0.5268263777171366957, 24.48095756788062261, 0.8226642508852344271 ) ) ;
#17698=CARTESIAN_POINT ( 'NONE',  ( 2.486440349385794502, 120.2382744777187611, 0.5044468955786926001 ) ) ;
#17700=CARTESIAN_POINT ( 'NONE',  ( -5.181828529333126099, 120.8264575521020987, 0.4749581527667977032 ) ) ;
#17702=( BOUNDED_CURVE ( )  B_SPLINE_CURVE ( 3, ( #12867, #6910, #33107, #7330 ),
 .UNSPECIFIED., .F., .T. ) 
 B_SPLINE_CURVE_WITH_KNOTS ( ( 4, 4 ),
 ( 1.570796326794896558, 3.141592653589793116 ),
 .UNSPECIFIED. ) 
 CURVE ( )  GEOMETRIC_REPRESENTATION_ITEM ( )  RATIONAL_B_SPLINE_CURVE ( ( 1.000000000000000000, 0.8047378541243649375, 0.8047378541243649375, 1.000000000000000000 ) ) 
 REPRESENTATION_ITEM ( '' )  );
#17703=CARTESIAN_POINT ( 'NONE',  ( 4.550223619785835005, 118.0718490517250814, -0.6268591698733608775 ) ) ;
#17704=CARTESIAN_POINT ( 'NONE',  ( 17.87798177106712672, 144.5560955566678558, -1.636306359874433847 ) ) ;
#17705=CARTESIAN_POINT ( 'NONE',  ( -17.00694855514576886, 128.5677977248401476, -2.111551361116177361 ) ) ;
#17707=CIRCLE ( 'NONE', #5480, 5.588000000000006295 ) ;
#17708=CARTESIAN_POINT ( 'NONE',  ( 4.242333036053028472, 118.2242299894752335, -0.3186625456669344159 ) ) ;
#17709=CARTESIAN_POINT ( 'NONE',  ( 15.66930740726043148, 147.5723176251010784, -0.2779681209298466293 ) ) ;
#17711=CARTESIAN_POINT ( 'NONE',  ( 1.850858793973401584, -15.28950465061244834, 5.390636727418374186 ) ) ;
#17712=AXIS2_PLACEMENT_3D ( 'NONE', #9448, #32247, #3077 ) ;
#17715=CARTESIAN_POINT ( 'NONE',  ( 4.628409624684510781, -5.919234854628785847, 0.1277143096542201761 ) ) ;
#17716=CARTESIAN_POINT ( 'NONE',  ( 0.5523667267584208007, 120.0661220204379305, 0.4484973920728143049 ) ) ;
#17717=CARTESIAN_POINT ( 'NONE',  ( -2.190789743540378698, 30.46265602596804811, 2.500874623987990208 ) ) ;
#17718=CARTESIAN_POINT ( 'NONE',  ( -4.093446853122649109, 111.5999093057820772, 2.867423493935855827 ) ) ;
#17719=CARTESIAN_POINT ( 'NONE',  ( -1.861891798414337940, 1.167894131763866250, -4.247245584637167504 ) ) ;
#17720=CARTESIAN_POINT ( 'NONE',  ( 1.611903344789260117, 120.9971453638330985, 0.05790686387416384834 ) ) ;
#17723=CARTESIAN_POINT ( 'NONE',  ( -2.156330945748770045, 116.3329555247961480, -0.2805685296613497637 ) ) ;
#17724=DIRECTION ( 'NONE',  ( 0.9998004120163608288, 0.000000000000000000, 0.01997839162482736852 ) ) ;
#17726=CARTESIAN_POINT ( 'NONE',  ( 1.842426711869075362, -15.45708672024492003, 5.391926158250407219 ) ) ;
#17727=CARTESIAN_POINT ( 'NONE',  ( -0.01632536679074437017, 38.84944212800221663, 1.323018725044087018 ) ) ;
#17729=CARTESIAN_POINT ( 'NONE',  ( 6.435022864794023079, 6.566661361801033436, 5.478585407919045025 ) ) ;
#17731=CARTESIAN_POINT ( 'NONE',  ( -0.09641566778521773462, 105.7853610664052866, 4.825034276358891816 ) ) ;
#17733=ADVANCED_FACE ( 'NONE', ( #20909 ), #7401, .T. ) ;
#17735=CARTESIAN_POINT ( 'NONE',  ( -23.14523085694538196, 149.5941399179437781, -0.009123583346247826631 ) ) ;
#17738=ORIENTED_EDGE ( 'NONE', *, *, #21226, .T. ) ;
#17741=CARTESIAN_POINT ( 'NONE',  ( -5.959810334499720419, 155.3892724211786742, -0.1190911940436165245 ) ) ;
#17742=CARTESIAN_POINT ( 'NONE',  ( 4.034131674322845029, -15.09852482505488780, 5.122685350376444902 ) ) ;
#17743=CARTESIAN_POINT ( 'NONE',  ( -20.98992760039535099, 147.8517002469272370, 1.565498118541299277 ) ) ;
#17744=CARTESIAN_POINT ( 'NONE',  ( 22.35542929045582383, 148.9358926463403918, -0.9984386947210761587 ) ) ;
#17745=CARTESIAN_POINT ( 'NONE',  ( -2.923568588381722844, 13.88697512809157786, 3.594856661414283394 ) ) ;
#17746=CARTESIAN_POINT ( 'NONE',  ( -6.905720769004730641, 117.2044255678715814, -0.3198409844323960027 ) ) ;
#17749=CARTESIAN_POINT ( 'NONE',  ( 8.796266902338841120, 117.6874721126187779, 0.2328958698391284388 ) ) ;
#17750=CARTESIAN_POINT ( 'NONE',  ( -10.06933303711913474, 122.3915136462027817, 1.070338282017660791 ) ) ;
#17752=CARTESIAN_POINT ( 'NONE',  ( 10.95471005835502609, 121.6366708983051836, -1.250572042008267326 ) ) ;
#17753=CARTESIAN_POINT ( 'NONE',  ( -7.089439975188652099, 158.1912585135832785, -1.657816039754273163 ) ) ;
#17756=CARTESIAN_POINT ( 'NONE',  ( 9.647033449255031812, 123.8920215319950842, -0.4922632944252960385 ) ) ;
#17758=ORIENTED_EDGE ( 'NONE', *, *, #19283, .F. ) ;
#17759=CARTESIAN_POINT ( 'NONE',  ( -16.10024230344514962, 135.1141785778430346, -2.240991319914668711 ) ) ;
#17760=CARTESIAN_POINT ( 'NONE',  ( 4.504576368470070591, -15.30243295294880745, -0.5136648547128764841 ) ) ;
#17761=CARTESIAN_POINT ( 'NONE',  ( -4.531929919898019854, 118.1072688352402338, -0.6771984859318007643 ) ) ;
#17765=CARTESIAN_POINT ( 'NONE',  ( -4.866602953137410204, 117.4089747018453238, 0.9905608030323003188 ) ) ;
#17766=CARTESIAN_POINT ( 'NONE',  ( 7.368974454111232752, 120.7277362223577768, 1.240556355415273870 ) ) ;
#17767=CARTESIAN_POINT ( 'NONE',  ( -5.332935381406168851, 115.7029491485442634, -0.1065653510733624160 ) ) ;
#17770=CARTESIAN_POINT ( 'NONE',  ( 23.21412382727100976, 149.6303025714371131, 0.4381719528662393337 ) ) ;
#17772=CARTESIAN_POINT ( 'NONE',  ( 0.7039615705130309875, 19.50765702457006157, -8.391957350905826729 ) ) ;
#17773=CARTESIAN_POINT ( 'NONE',  ( 15.70678031088808879, 147.2451778420852406, 0.7656494529899997570 ) ) ;
#17777=CARTESIAN_POINT ( 'NONE',  ( 2.186287969701115497, 115.6909491485452577, 1.711441318780086540 ) ) ;
#17779=CARTESIAN_POINT ( 'NONE',  ( -3.297133786507796760, 159.4684106755469202, -0.01890815954691990250 ) ) ;
#17780=VERTEX_POINT ( 'NONE', #15779 ) ;
#17782=CARTESIAN_POINT ( 'NONE',  ( -7.874818391576265064, 122.1194222050971518, -0.8646837367724872214 ) ) ;
#17785=CARTESIAN_POINT ( 'NONE',  ( -4.757314290308038984, 117.4006805855117364, -1.206872172350066164 ) ) ;
#17786=CARTESIAN_POINT ( 'NONE',  ( -2.787004648571314025, 120.9517662584847102, -0.1965090384792944900 ) ) ;
#17787=CARTESIAN_POINT ( 'NONE',  ( 4.523112235310252416, -13.07411707498565256, 2.966381825927230764 ) ) ;
#17788=TOROIDAL_SURFACE ( 'NONE', #5575, 5.080000000000005400, 0.5080000000000000071 ) ;
#17789=CARTESIAN_POINT ( 'NONE',  ( -1.091392056213116746, 117.4935207075373569, 0.4954137919519209232 ) ) ;
#17790=DIRECTION ( 'NONE',  ( 0.9998004120163609398, 0.000000000000000000, 0.01997839162482749689 ) ) ;
#17792=CARTESIAN_POINT ( 'NONE',  ( 6.903663268456370794, 117.1865127098105575, 0.2656477445430290296 ) ) ;
#17793=CARTESIAN_POINT ( 'NONE',  ( 10.99029326479648461, 127.9870517001798760, 0.2725059437867732859 ) ) ;
#17795=CARTESIAN_POINT ( 'NONE',  ( 0.4606059098249736805, 26.09511874640634943, 0.8667040019166204479 ) ) ;
#17796=CARTESIAN_POINT ( 'NONE',  ( -22.98488057257204886, 150.1591296352320910, -0.4592926148156235011 ) ) ;
#17802=CARTESIAN_POINT ( 'NONE',  ( -8.499151694004579483, 119.2578417338014702, 1.013587109124426178 ) ) ;
#17803=CARTESIAN_POINT ( 'NONE',  ( -3.254339884055971854, 0.1279812147911008058, 3.287934741457726684 ) ) ;
#17804=CARTESIAN_POINT ( 'NONE',  ( 14.46681479972615136, 121.7426775721902175, 1.517288920005034791 ) ) ;
#17806=CARTESIAN_POINT ( 'NONE',  ( 0.03153870137008670665, 158.4432089348667319, -1.578325583784928154 ) ) ;
#17807=CARTESIAN_POINT ( 'NONE',  ( -1.011143250135940530, 20.41458852336931074, 8.389224627043086358 ) ) ;
#17808=CARTESIAN_POINT ( 'NONE',  ( -14.51109376910522286, 156.0472725025049954, -1.459756479172738874 ) ) ;
#17809=CARTESIAN_POINT ( 'NONE',  ( 4.772939762337750302, 117.6315509942823923, -0.9548895502630124765 ) ) ;
#17810=ORIENTED_EDGE ( 'NONE', *, *, #34479, .F. ) ;
#17811=EDGE_CURVE ( 'NONE', #31901, #32861, #25900, .T. ) ;
#17812=CARTESIAN_POINT ( 'NONE',  ( -15.81858318527965324, 146.5893318786020814, 0.01456738144011954575 ) ) ;
#17813=CARTESIAN_POINT ( 'NONE',  ( 4.034131674322845029, -15.09852482505488780, 5.122685350376444902 ) ) ;
#17814=EDGE_CURVE ( 'NONE', #7084, #18074, #10061, .T. ) ;
#17816=CARTESIAN_POINT ( 'NONE',  ( -3.099633551182617186, 108.5668320698263898, -4.179674138198564926 ) ) ;
#17818=CARTESIAN_POINT ( 'NONE',  ( 4.182621382391884524, 157.4559852174668322, 1.843664507743932424 ) ) ;
#17823=CARTESIAN_POINT ( 'NONE',  ( -0.5256976547266306588, 110.0486234891351245, 3.677594289785357518 ) ) ;
#17825=CARTESIAN_POINT ( 'NONE',  ( -2.748994976520039213, 10.49642266832308124, 7.958378898918418543 ) ) ;
#17826=CARTESIAN_POINT ( 'NONE',  ( 14.94238115049589588, 139.3652335140928074, 1.424457715676853642 ) ) ;
#17828=CARTESIAN_POINT ( 'NONE',  ( 2.863213894092299316, 116.8186761214209213, -0.2817159656421848180 ) ) ;
#17834=CARTESIAN_POINT ( 'NONE',  ( -4.257826819935623064, 118.2250077456210846, 0.3017621733391205874 ) ) ;
#17838=CARTESIAN_POINT ( 'NONE',  ( 8.312601280572751605, 120.1777224443565615, -1.117780186305196821 ) ) ;
#17839=CARTESIAN_POINT ( 'NONE',  ( -7.326027964658058167, 123.0350022594044219, -0.2150643116641766939 ) ) ;
#17840=CARTESIAN_POINT ( 'NONE',  ( 4.296427252414747322, 118.2130177109110321, 0.5011668729022451529 ) ) ;
#17841=CARTESIAN_POINT ( 'NONE',  ( -0.6009856513686788748, 120.6441756478195089, -0.2688776736664573175 ) ) ;
#17845=CARTESIAN_POINT ( 'NONE',  ( -0.9950013725589796909, 29.65466048987409309, -4.513790593961638287 ) ) ;
#17846=CARTESIAN_POINT ( 'NONE',  ( -13.40915985073344352, 130.9706359334022920, -1.586196205478585197 ) ) ;
#17850=CARTESIAN_POINT ( 'NONE',  ( -15.64684598352423350, 147.2230049032471868, -0.1119480208309122649 ) ) ;
#17851=CARTESIAN_POINT ( 'NONE',  ( 4.636249899789679496, -11.37698174978397958, -0.2454043791197063895 ) ) ;
#17852=CARTESIAN_POINT ( 'NONE',  ( 22.71262516694549660, 146.4845460041848355, 1.645735859231715725 ) ) ;
#17854=CARTESIAN_POINT ( 'NONE',  ( 3.221735024265227398, -14.36526069886394730, 2.718910799868354378 ) ) ;
#17855=CARTESIAN_POINT ( 'NONE',  ( 0.009513433763446757160, 117.6614778598761291, -0.4760911276077179899 ) ) ;
#17856=CARTESIAN_POINT ( 'NONE',  ( -11.27019207447484384, 122.4230570912197038, 1.244363564371071540 ) ) ;
#17857=CARTESIAN_POINT ( 'NONE',  ( -0.8659212883131867100, -1.167510040683709560, 0.4517697218592801600 ) ) ;
#17858=CARTESIAN_POINT ( 'NONE',  ( -15.17352684164009524, 120.8830733721255370, -0.9063557954379339865 ) ) ;
#17860=CARTESIAN_POINT ( 'NONE',  ( 0.4978855121113271442, 23.66801414613304289, -0.8366695591092367934 ) ) ;
#17861=ORIENTED_EDGE ( 'NONE', *, *, #1224, .T. ) ;
#17863=CARTESIAN_POINT ( 'NONE',  ( -9.542276680740393147, 123.9284174147966269, 0.4124357159827420349 ) ) ;
#17864=CARTESIAN_POINT ( 'NONE',  ( 4.564001774108119136, -12.95384785397724059, 2.770574723176509657 ) ) ;
#17865=CARTESIAN_POINT ( 'NONE',  ( 5.875224328284113895, 120.7327493588883840, -0.6546335550538250336 ) ) ;
#17867=CARTESIAN_POINT ( 'NONE',  ( 0.5746707734919784816, 115.7029522474750820, 1.760669174839533557 ) ) ;
#17869=CARTESIAN_POINT ( 'NONE',  ( 3.398501971686946010, -13.69110397484313246, 2.823423868610629217 ) ) ;
#17870=CARTESIAN_POINT ( 'NONE',  ( -4.707310151561321376, 117.7551317797143469, -1.085303849379790186 ) ) ;
#17871=CARTESIAN_POINT ( 'NONE',  ( 9.119960873764027198, 153.9201329141909866, 0.06997149051007753306 ) ) ;
#17873=CARTESIAN_POINT ( 'NONE',  ( 13.15656197906093894, 122.1656469061080514, 1.777190774585285071 ) ) ;
#17874=FACE_OUTER_BOUND ( 'NONE', #25745, .T. ) ;
#17877=CARTESIAN_POINT ( 'NONE',  ( 0.02615319344467511437, 156.8698190429800832, -1.308812744920978322 ) ) ;
#17878=CARTESIAN_POINT ( 'NONE',  ( 9.784355093145334692, 118.0142902678875885, -0.004515160920743642621 ) ) ;
#17881=AXIS2_PLACEMENT_3D ( 'NONE', #39837, #33442, #17232 ) ;
#17882=CARTESIAN_POINT ( 'NONE',  ( 1.931858869400174150, -15.61904180168537160, 5.924774731895777080 ) ) ;
#17884=CARTESIAN_POINT ( 'NONE',  ( -1.912856793975784786, 32.45769749710033381, 0.9767251062931671113 ) ) ;
#17885=CARTESIAN_POINT ( 'NONE',  ( -4.753021167359183785, 117.9428942815730466, 0.6272315166840956024 ) ) ;
#17889=CARTESIAN_POINT ( 'NONE',  ( -8.482050796837413031, 119.1145137661371933, -1.313062426393583060 ) ) ;
#17890=CARTESIAN_POINT ( 'NONE',  ( -5.854942301702540597, 124.9344662015456890, -0.1169956811762812854 ) ) ;
#17891=CARTESIAN_POINT ( 'NONE',  ( 4.883721824859848404, 117.6381041156431024, 1.023514187599162906 ) ) ;
#17893=CARTESIAN_POINT ( 'NONE',  ( -0.9884870862450249041, 123.5966405200008325, 0.1018174175105951568 ) ) ;
#17895=CARTESIAN_POINT ( 'NONE',  ( 1.961646697876492373, -0.1315482170498871728, -4.191205975169975950 ) ) ;
#17896=CARTESIAN_POINT ( 'NONE',  ( 5.002599301907898699, 117.4023545182666055, -0.8031422281648238348 ) ) ;
#17897=CARTESIAN_POINT ( 'NONE',  ( -3.332395206781303187, 108.2587724951642087, -4.156421558053723153 ) ) ;
#17898=CARTESIAN_POINT ( 'NONE',  ( 3.350179296191433398, -14.02378440268806159, 3.677192885962260682 ) ) ;
#17899=CARTESIAN_POINT ( 'NONE',  ( 0.1065646865914872121, 105.8844662015457061, -5.332932678536314697 ) ) ;
#17900=CARTESIAN_POINT ( 'NONE',  ( -4.338858593134309771, 28.47720539748115698, 2.044640056223529179 ) ) ;
#17901=CARTESIAN_POINT ( 'NONE',  ( -2.051726258433167693, 115.7029491863252133, 1.635864041877385100 ) ) ;
#17902=CARTESIAN_POINT ( 'NONE',  ( 0.9564925537785137211, 29.00497265395555857, -4.523030980006896407 ) ) ;
#17903=VERTEX_POINT ( 'NONE', #33042 ) ;
#17904=CARTESIAN_POINT ( 'NONE',  ( -5.344509134975541365, 104.6144662015523750, 0.1077285959981589963 ) ) ;
#17905=CARTESIAN_POINT ( 'NONE',  ( 4.028426573186930426, -15.65323953938244017, 3.316845843096514201 ) ) ;
#17906=CARTESIAN_POINT ( 'NONE',  ( -7.699499347746557198, 119.6133147451300971, 1.075113282820071570 ) ) ;
#17907=CARTESIAN_POINT ( 'NONE',  ( 0.2459283266301676152, 20.16186220226971315, -0.9436028068393225166 ) ) ;
#17908=ORIENTED_EDGE ( 'NONE', *, *, #23999, .T. ) ;
#17910=DIRECTION ( 'NONE',  ( -0.9998004120163608288, 0.000000000000000000, -0.01997839162482749342 ) ) ;
#17911=CARTESIAN_POINT ( 'NONE',  ( 1.040151681621031221, 108.5039085404744981, 4.268591994808179635 ) ) ;
#17912=CARTESIAN_POINT ( 'NONE',  ( -12.75300196040212874, 152.1353413313561305, 1.119124812251137691 ) ) ;
#17914=CARTESIAN_POINT ( 'NONE',  ( 4.531563741779123689, 118.0870819156608320, -0.6068543356175654102 ) ) ;
#17915=CARTESIAN_POINT ( 'NONE',  ( 5.873949295438634977, 120.1673030736515955, -0.8402073876045390577 ) ) ;
#17917=CARTESIAN_POINT ( 'NONE',  ( 0.01133701039331720326, 118.4098733054621277, -0.5673503590873751889 ) ) ;
#17918=CARTESIAN_POINT ( 'NONE',  ( -6.639407854763120941E-14, 101.6934662015457320, 3.307182826377456566E-30 ) ) ;
#17919=CARTESIAN_POINT ( 'NONE',  ( 4.270423886376517153, 118.2236112661795175, -0.2874234743081488519 ) ) ;
#17921=CARTESIAN_POINT ( 'NONE',  ( 7.650102001921197825, 122.3449549946481056, -0.2051776793030276602 ) ) ;
#17923=CARTESIAN_POINT ( 'NONE',  ( 2.233078627056604759, -15.14192004606506536, 5.083345892419886880 ) ) ;
#17926=CARTESIAN_POINT ( 'NONE',  ( 0.6256056815405413030, -8.068247431453825058, 4.577905309659676014 ) ) ;
#17927=CARTESIAN_POINT ( 'NONE',  ( 16.96873827569982041, 146.4457527449227143, 1.929048950080526126 ) ) ;
#17928=CARTESIAN_POINT ( 'NONE',  ( -2.804869963407872202, 28.95498092762696984, 0.1876698244966022444 ) ) ;
#17929=CARTESIAN_POINT ( 'NONE',  ( -7.256067632580425197, 123.0461458356614628, -0.07605313119184028969 ) ) ;
#17932=CARTESIAN_POINT ( 'NONE',  ( -3.416230376366909294, -5.529048218071860532, 3.121479803864907865 ) ) ;
#17933=CARTESIAN_POINT ( 'NONE',  ( 15.77055413937410222, 146.5697412905949477, 0.3665361178749760307 ) ) ;
#17934=CARTESIAN_POINT ( 'NONE',  ( 8.237246883283409815, -6.118032110028554627, 1.824569540066587114 ) ) ;
#17936=CARTESIAN_POINT ( 'NONE',  ( -8.777543396403881815, 117.7565081666817832, -0.4614390791137490955 ) ) ;
#17937=CARTESIAN_POINT ( 'NONE',  ( 0.009645608633017716330, 120.9711055683165597, -0.4827056984855355171 ) ) ;
#17940=CARTESIAN_POINT ( 'NONE',  ( 2.058067359092983661, -15.63668844659656187, 5.842422791592847275 ) ) ;
#17942=CARTESIAN_POINT ( 'NONE',  ( 4.223004820120735303, -0.3563183945215069870, -7.287282906663286930 ) ) ;
#17943=CYLINDRICAL_SURFACE ( 'NONE', #13010, 3.175000000000001155 ) ;
#17945=CARTESIAN_POINT ( 'NONE',  ( 2.350639260211558668, -15.10312717587823705, 4.966175652281853203 ) ) ;
#17947=CARTESIAN_POINT ( 'NONE',  ( -15.06072413439841817, 156.1474796653986630, 0.2161187639505617319 ) ) ;
#17950=( BOUNDED_SURFACE ( )  B_SPLINE_SURFACE ( 3, 2, ( 
 ( #25380, #9197, #38385 ),
 ( #13587, #29571, #16562 ),
 ( #407, #21953, #15359 ),
 ( #3811, #16775, #28366 ),
 ( #10389, #12176, #36179 ),
 ( #16346, #29351, #35186 ),
 ( #13165, #23361, #25172 ),
 ( #5805, #26576, #18760 ),
 ( #22154, #31771, #13375 ),
 ( #18973, #22934, #26155 ),
 ( #39156, #9962, #35963 ),
 ( #26362, #39371, #10173 ),
 ( #39584, #36395, #17816 ),
 ( #24415, #4861, #1451 ),
 ( #39803, #1033, #26793 ),
 ( #30609, #23575, #30192 ),
 ( #20171, #36598, #4232 ),
 ( #13997, #33614, #30816 ),
 ( #4651, #33822, #7834 ),
 ( #37420, #33197, #37218 ) ),
 .UNSPECIFIED., .F., .F., .F. ) 
 B_SPLINE_SURFACE_WITH_KNOTS ( ( 4, 2, 2, 2, 2, 2, 2, 2, 2, 4 ),
 ( 3, 3 ),
 ( -3.009270892369297901E-16, 0.0008043714308976721581, 0.001608742861795645291, 0.002413114292693618532, 0.003217485723591591556, 0.004021857154489564580, 0.004826228585387538038, 0.006434971447183484086, 0.009652457170775376183, 0.01286994289436726828 ),
 ( 0.000000000000000000, 1.000000000000000000 ),
 .UNSPECIFIED. ) 
 GEOMETRIC_REPRESENTATION_ITEM ( )  RATIONAL_B_SPLINE_SURFACE ( (
 ( 1.000000000000000000, 0.9815197824473285149, 1.000000000000000000),
 ( 1.000000000000000000, 0.9811723635258926546, 1.000000000000000000),
 ( 1.000000000000000000, 0.9803956462538041539, 1.000000000000000000),
 ( 1.000000000000000000, 0.9775604298907969447, 1.000000000000000000),
 ( 1.000000000000000000, 0.9755054586208901091, 1.000000000000000000),
 ( 1.000000000000000000, 0.9704993482238920555, 1.000000000000000000),
 ( 1.000000000000000000, 0.9675447666335766916, 1.000000000000000000),
 ( 1.000000000000000000, 0.9610561756468071204, 1.000000000000000000),
 ( 1.000000000000000000, 0.9575813355064265453, 1.000000000000000000),
 ( 1.000000000000000000, 0.9503236772837940771, 1.000000000000000000),
 ( 1.000000000000000000, 0.9465499958478611475, 1.000000000000000000),
 ( 1.000000000000000000, 0.9387344193221167643, 1.000000000000000000),
 ( 1.000000000000000000, 0.9346745718259914515, 1.000000000000000000),
 ( 1.000000000000000000, 0.9222609948196353047, 1.000000000000000000),
 ( 1.000000000000000000, 0.9134583146165992096, 1.000000000000000000),
 ( 1.000000000000000000, 0.8860507374761776855, 1.000000000000000000),
 ( 1.000000000000000000, 0.8669451626876586436, 1.000000000000000000),
 ( 1.000000000000000000, 0.8330907799448757922, 1.000000000000000000),
 ( 1.000000000000000000, 0.8189901318540898645, 1.000000000000000000),
 ( 1.000000000000000000, 0.8121911378916643054, 1.000000000000000000) ) ) 
 REPRESENTATION_ITEM ( '' )  SURFACE ( )  );
#17953=CARTESIAN_POINT ( 'NONE',  ( -9.118174893680297544, 124.1671967267183589, -0.1822028344259498389 ) ) ;
#17954=CARTESIAN_POINT ( 'NONE',  ( 4.666472529085985421, -15.22678077218547799, 4.383143511210439769 ) ) ;
#17955=CARTESIAN_POINT ( 'NONE',  ( -3.126689565637764456, 118.0390668470448929, 0.7034308075613268096 ) ) ;
#17957=CARTESIAN_POINT ( 'NONE',  ( 22.59368173950831604, 146.4122051224262577, -0.8656317577275308706 ) ) ;
#17958=CARTESIAN_POINT ( 'NONE',  ( -2.755274729907521980, 20.69627551736597226, -3.746277899328600558 ) ) ;
#17959=CARTESIAN_POINT ( 'NONE',  ( -15.20946960781377832, 120.7148350616293300, -0.7222319099908601769 ) ) ;
#17962=CARTESIAN_POINT ( 'NONE',  ( 5.561693798059717864, 116.7001734479162138, 0.1683348082849521199 ) ) ;
#17964=CARTESIAN_POINT ( 'NONE',  ( -1.391675519083843460, 119.6596719632383383, 0.5469696729655013634 ) ) ;
#17966=ADVANCED_FACE ( 'NONE', ( #35605 ), #37481, .T. ) ;
#17967=CARTESIAN_POINT ( 'NONE',  ( 1.284628845569729894, 118.8689652838214244, -0.6394392525890019163 ) ) ;
#17969=CARTESIAN_POINT ( 'NONE',  ( -15.17292428814161553, 123.1171956318823533, -1.668999667383225471 ) ) ;
#17971=CARTESIAN_POINT ( 'NONE',  ( 7.796255004792614685, 122.1031240515655298, -0.5053261734565677177 ) ) ;
#17973=CARTESIAN_POINT ( 'NONE',  ( -17.13831219182137033, 149.7102054596878702, -2.353104315458284468 ) ) ;
#17974=CARTESIAN_POINT ( 'NONE',  ( 4.184971198371238543, -15.30562903706386635, -0.2021278847381603183 ) ) ;
#17976=CARTESIAN_POINT ( 'NONE',  ( -4.468857898947769414, 118.1303058819741381, -0.7050480387964153106 ) ) ;
#17979=CARTESIAN_POINT ( 'NONE',  ( -4.888083438996877916, 117.4785984266663803, 0.9708402414164146732 ) ) ;
#17980=CARTESIAN_POINT ( 'NONE',  ( 6.574985064279017521, 120.4115791468657903, 1.154926965394999394 ) ) ;
#17981=CARTESIAN_POINT ( 'NONE',  ( -6.566230858599542383E-14, 82.13546620154573930, -5.726718672203201028E-18 ) ) ;
#17982=CARTESIAN_POINT ( 'NONE',  ( -8.022552064266685434, 3.315157024569945765, 2.561087356634513590 ) ) ;
#17983=CARTESIAN_POINT ( 'NONE',  ( 15.76219760562750771, 147.2673792861271522, 0.9072345144146886087 ) ) ;
#17986=CARTESIAN_POINT ( 'NONE',  ( -2.558524215040917316, 118.1588900017448509, 0.7376291965803625228 ) ) ;
#17987=CARTESIAN_POINT ( 'NONE',  ( 2.765784402779746465, 118.7629491485453883, 1.199736011334208818 ) ) ;
#17991=CARTESIAN_POINT ( 'NONE',  ( -0.9075203043614510356, 116.4850453793277865, 0.07935580435194651561 ) ) ;
#17994=CARTESIAN_POINT ( 'NONE',  ( 5.869729252252017915, 121.2845232542697573, -0.2003997253776844401 ) ) ;
#17995=CARTESIAN_POINT ( 'NONE',  ( -8.020178813430042908, 121.5755450013093224, 0.8283951592328122615 ) ) ;
#17996=CARTESIAN_POINT ( 'NONE',  ( 1.144851334150850164, 115.6909491485452719, -1.703252225057385161 ) ) ;
#17997=CARTESIAN_POINT ( 'NONE',  ( -15.76594527475419483, 145.7191243368997675, -0.6468106390071731715 ) ) ;
#17998=CARTESIAN_POINT ( 'NONE',  ( 4.475827780916731946, -13.19141740729908108, 3.156716699630707890 ) ) ;
#17999=CARTESIAN_POINT ( 'NONE',  ( -3.032027503100559240, 117.5448765310053005, 0.5892388327060571473 ) ) ;
#18000=CARTESIAN_POINT ( 'NONE',  ( 3.682264917456193221, 75.78546620154573077, 0.07358041635423968885 ) ) ;
#18001=CARTESIAN_POINT ( 'NONE',  ( 8.213135470206557542, 117.5064756823292385, 0.2531991783344220703 ) ) ;
#18002=CARTESIAN_POINT ( 'NONE',  ( 0.6405796906021217207, 156.3034662015458593, 0.04853048433328251837 ) ) ;
#18004=CARTESIAN_POINT ( 'NONE',  ( 0.1338929724787690234, 25.55936205620983515, 0.9658879472844225100 ) ) ;
#18006=CARTESIAN_POINT ( 'NONE',  ( -5.774842806153472452, 116.9337168780244696, -0.1296094601971083948 ) ) ;
#18008=ORIENTED_EDGE ( 'NONE', *, *, #11000, .F. ) ;
#18009=DIRECTION ( 'NONE',  ( -0.01997839162482737546, -1.040247600000940825E-18, 0.9998004120163610509 ) ) ;
#18011=CARTESIAN_POINT ( 'NONE',  ( 3.713122095021297753, 118.0206735692917022, 0.9242336517888254388 ) ) ;
#18013=CARTESIAN_POINT ( 'NONE',  ( 20.44519586420840440, 150.9797539340098069, 2.100688152434085243 ) ) ;
#18015=CARTESIAN_POINT ( 'NONE',  ( 18.27466214341546191, 151.8090458617612057, -1.628071726616033388 ) ) ;
#18016=CARTESIAN_POINT ( 'NONE',  ( 4.581850893073086795, -15.30275035579069254, -0.5110622633019785699 ) ) ;
#18017=CARTESIAN_POINT ( 'NONE',  ( -22.07768208608597504, 150.1365687424457178, -1.739787554465966668 ) ) ;
#18018=CARTESIAN_POINT ( 'NONE',  ( 4.900207408254827257, 117.6430132448414270, -0.8582711705238391664 ) ) ;
#18020=CARTESIAN_POINT ( 'NONE',  ( -5.925782188533705863, 121.5237468798633955, 0.003878672073842466105 ) ) ;
#18021=CARTESIAN_POINT ( 'NONE',  ( 3.194259428633707376, -15.59200274161393018, 5.439406988142795107 ) ) ;
#18025=CARTESIAN_POINT ( 'NONE',  ( 5.835242038117685048, 119.5807162246413498, 1.179424802705185238 ) ) ;
#18027=CARTESIAN_POINT ( 'NONE',  ( -0.7550517280344761772, 118.1535578050699087, -0.9127457894755339751 ) ) ;
#18028=CARTESIAN_POINT ( 'NONE',  ( -2.352838477949809270, 119.2037781873646622, 0.5921520780602628209 ) ) ;
#18029=CARTESIAN_POINT ( 'NONE',  ( -7.647780498939813931, -9.906183224868927439, 3.644365410659974991 ) ) ;
#18030=CARTESIAN_POINT ( 'NONE',  ( 16.01418025823780766, 147.7157881801689427, 1.429122529412921061 ) ) ;
#18031=DIRECTION ( 'NONE',  ( -0.9998004120163609398, 0.000000000000000000, -0.01997839162482749689 ) ) ;
#18032=ADVANCED_FACE ( 'NONE', ( #29628 ), #26601, .T. ) ;
#18034=CARTESIAN_POINT ( 'NONE',  ( 16.59152294496558966, 155.2525159475892167, -0.4418349252515506587 ) ) ;
#18040=CARTESIAN_POINT ( 'NONE',  ( -4.157387891345566189, 118.2390912615641838, 0.2342884288663792947 ) ) ;
#18041=CARTESIAN_POINT ( 'NONE',  ( 3.563983649201253989, 108.3861600575944379, -3.960794436007483821 ) ) ;
#18042=ORIENTED_EDGE ( 'NONE', *, *, #16476, .T. ) ;
#18045=CARTESIAN_POINT ( 'NONE',  ( 6.279405009837805807, 119.8162689779731949, -0.9809252895020896812 ) ) ;
#18047=CARTESIAN_POINT ( 'NONE',  ( 4.279885407778224682, 118.2143666532004715, 0.5181637047333805812 ) ) ;
#18048=CARTESIAN_POINT ( 'NONE',  ( -9.600854460372945098, 124.0356975489027036, -0.7994020406953789015 ) ) ;
#18049=CARTESIAN_POINT ( 'NONE',  ( 16.31694223957253698, 121.4173703750124531, 0.3260513381110077824 ) ) ;
#18051=CARTESIAN_POINT ( 'NONE',  ( 2.332027132427558769, 25.33165720878049498, 3.998286310156994983 ) ) ;
#18052=CARTESIAN_POINT ( 'NONE',  ( -5.158718007120306481, 120.8264575521020987, -0.6815868816981844880 ) ) ;
#18056=CARTESIAN_POINT ( 'NONE',  ( -6.062687220451711489, 121.4407148395792007, -0.04901857013319344675 ) ) ;
#18058=CARTESIAN_POINT ( 'NONE',  ( -4.621355134897683570, 27.56591289442953041, -0.4301045952606497025 ) ) ;
#18059=CARTESIAN_POINT ( 'NONE',  ( 22.82453445504499356, 148.6346580502994073, 1.538154475459325043 ) ) ;
#18061=CARTESIAN_POINT ( 'NONE',  ( 2.993548201347409510, -14.88003303992029025, 3.932447912750371977 ) ) ;
#18062=CARTESIAN_POINT ( 'NONE',  ( 21.16640241758159036, 149.7512365312068709, -1.384406599442889130 ) ) ;
#18063=CARTESIAN_POINT ( 'NONE',  ( -2.279834263381315562, 157.4004113605966211, 1.585270110160261758 ) ) ;
#18064=CARTESIAN_POINT ( 'NONE',  ( -3.632229383214316876, 17.08265688572556584, -2.901706292871565562 ) ) ;
#18065=CARTESIAN_POINT ( 'NONE',  ( -9.660431270553321070, 118.1749183431956425, -0.7024802509354080016 ) ) ;
#18067=CARTESIAN_POINT ( 'NONE',  ( 0.9269407327955943021, 12.00036500698010578, 0.3089908296573128932 ) ) ;
#18071=CARTESIAN_POINT ( 'NONE',  ( -8.072651008563880737, 154.6119571123129788, 0.5584669891872423575 ) ) ;
#18072=CARTESIAN_POINT ( 'NONE',  ( 5.898638393742167807, -12.20234047945549527, 0.6047796074133310329 ) ) ;
#18073=CARTESIAN_POINT ( 'NONE',  ( 8.983288137945146801, 154.9128698100208794, -1.355969927742461723 ) ) ;
#18074=VERTEX_POINT ( 'NONE', #32194 ) ;
#18075=CARTESIAN_POINT ( 'NONE',  ( 1.357034515785712880, 115.7027987071164574, 1.737102370113531746 ) ) ;
#18076=CARTESIAN_POINT ( 'NONE',  ( 1.848046085800040483, -15.12359198595263088, 5.521975501593071378 ) ) ;
#18077=CARTESIAN_POINT ( 'NONE',  ( -4.742396055309614056, 117.8491596531413563, -0.9896183798233539886 ) ) ;
#18078=CARTESIAN_POINT ( 'NONE',  ( 15.77879114986260589, 146.5725700477668170, 0.1868612039608988085 ) ) ;
#18080=EDGE_LOOP ( 'NONE', ( #29438, #37809, #29408, #3559 ) ) ;
#18081=CARTESIAN_POINT ( 'NONE',  ( 7.694773992301578325, 119.4405053107883958, 1.366649582720010025 ) ) ;
#18085=CARTESIAN_POINT ( 'NONE',  ( 13.57554913733958557, 119.6371495169912436, 0.05144635950012921982 ) ) ;
#18087=CARTESIAN_POINT ( 'NONE',  ( 1.683587623118159682, -15.20357760260822388, 5.672209996086073680 ) ) ;
#18089=CARTESIAN_POINT ( 'NONE',  ( -5.274544067074300457, 115.7029491485454002, 0.8135768287290441325 ) ) ;
#18092=CARTESIAN_POINT ( 'NONE',  ( -4.640960256449444543, 117.9807172536480238, 0.7263108157050279790 ) ) ;
#18094=VERTEX_POINT ( 'NONE', #465 ) ;
#18096=CARTESIAN_POINT ( 'NONE',  ( -4.974399692199978240, 117.4065978902591354, 0.8873519537265817103 ) ) ;
#18097=CARTESIAN_POINT ( 'NONE',  ( -5.764161295553385855, 118.7617298297994637, -1.235935067645903329 ) ) ;
#18098=CARTESIAN_POINT ( 'NONE',  ( 0.1065646865915093611, 105.8844662015456777, -5.332932678536313809 ) ) ;
#18099=CARTESIAN_POINT ( 'NONE',  ( 4.752655214354502888, 117.6359145343736117, 1.138150416757013339 ) ) ;
#18101=CARTESIAN_POINT ( 'NONE',  ( -0.4103500344927140664, 124.0591982226670211, 0.08506156519360540125 ) ) ;
#18102=CARTESIAN_POINT ( 'NONE',  ( 0.09481320634720795393, -4.229605868409334057, 4.636458411128852930 ) ) ;
#18103=CARTESIAN_POINT ( 'NONE',  ( 4.889703507614793665, 117.4101837603834468, -0.9754936775373431734 ) ) ;
#18105=CARTESIAN_POINT ( 'NONE',  ( 3.377503200524144322, -12.59127376242380514, 1.184662976626496000 ) ) ;
#18106=CARTESIAN_POINT ( 'NONE',  ( 5.249845242698079062, 116.4925209815607730, -0.8804580864248582328 ) ) ;
#18107=CARTESIAN_POINT ( 'NONE',  ( -4.445868218450056197, 29.55296359113615523, 3.403299529360248599 ) ) ;
#18108=CARTESIAN_POINT ( 'NONE',  ( -0.7131320481206968598, 115.7031549148529734, 1.731730113216342071 ) ) ;
#18109=CARTESIAN_POINT ( 'NONE',  ( 1.790774717077139089, 25.13178105314743860, 4.274281468382033822 ) ) ;
#18110=ORIENTED_EDGE ( 'NONE', *, *, #41205, .T. ) ;
#18111=CARTESIAN_POINT ( 'NONE',  ( -4.808149584360944750, 104.6144662015457527, 0.4147572885131461939 ) ) ;
#18112=CARTESIAN_POINT ( 'NONE',  ( 3.591698533489739553, -15.62560650602327961, 3.738647084555763112 ) ) ;
#18113=CARTESIAN_POINT ( 'NONE',  ( -5.881924083617415810, 119.0696708348911699, 0.9594134845634217923 ) ) ;
#18114=CARTESIAN_POINT ( 'NONE',  ( -0.7486558104752240039, 25.82057725623272759, -0.6268360674696834556 ) ) ;
#18116=CARTESIAN_POINT ( 'NONE',  ( -0.4721710868402241301, 14.98625149489145159, 0.8573358612705738180 ) ) ;
#18119=PLANE ( 'NONE',  #9113 ) ;
#18120=CARTESIAN_POINT ( 'NONE',  ( 1.600579373209928269, 119.3928400758114918, 0.6828601607076615343 ) ) ;
#18121=CARTESIAN_POINT ( 'NONE',  ( -8.566376370482908342, 122.4751019636825049, 0.6322842599711311351 ) ) ;
#18123=CARTESIAN_POINT ( 'NONE',  ( 3.247910276010201880, -14.18928037215049009, 3.960261243354706640 ) ) ;
#18124=CARTESIAN_POINT ( 'NONE',  ( 18.19397457907784599, 146.9188445454784357, -1.620492285849223224 ) ) ;
#18125=CARTESIAN_POINT ( 'NONE',  ( 0.03153870137009017610, 158.4432089348667319, -1.578325583784927932 ) ) ;
#18127=CARTESIAN_POINT ( 'NONE',  ( 4.119003220443754110, 118.2429491485453354, -0.1854851255534567256 ) ) ;
#18128=CARTESIAN_POINT ( 'NONE',  ( 0.003052472355804966304, 120.8426702770480148, -0.1527581987772200500 ) ) ;
#18131=CARTESIAN_POINT ( 'NONE',  ( 2.930607426163104545, -14.92094031927118714, 4.083576684136651203 ) ) ;
#18134=CARTESIAN_POINT ( 'NONE',  ( -0.05192310401019068627, -8.293124787585329116, 4.627658001227512585 ) ) ;
#18135=CARTESIAN_POINT ( 'NONE',  ( 0.7424407951589586663, 156.5584078035761593, 0.9879031837870264621 ) ) ;
#18136=CARTESIAN_POINT ( 'NONE',  ( 0.06674422508556764055, 33.39646256408616409, 3.182828529663568773 ) ) ;
#18137=CARTESIAN_POINT ( 'NONE',  ( -2.817215192601065787, 108.0685014782224442, 4.280041469292686251 ) ) ;
#18139=CARTESIAN_POINT ( 'NONE',  ( -4.627450822138572839, 2.892058097378844117, -0.1328416527703782657 ) ) ;
#18140=CARTESIAN_POINT ( 'NONE',  ( 14.16569067496505774, 138.8670163227233161, 0.2830642121559648339 ) ) ;
#18141=CARTESIAN_POINT ( 'NONE',  ( -2.830841276205400270, 0.8888151952923978305, 7.984752373722160179 ) ) ;
#18143=CARTESIAN_POINT ( 'NONE',  ( 5.522311800473831411, 117.0453351255057726, -0.4840448646347706441 ) ) ;
#18147=CARTESIAN_POINT ( 'NONE',  ( -5.495523183683927115, 31.57050297546189199, 3.325088329614593885 ) ) ;
#18148=CARTESIAN_POINT ( 'NONE',  ( 4.037907715354051241, 27.70556447992504445, -2.267523456217593214 ) ) ;
#18150=CARTESIAN_POINT ( 'NONE',  ( -5.078986093043186045, 98.39146620154573952, -0.1014902294541237954 ) ) ;
#18152=CARTESIAN_POINT ( 'NONE',  ( 0.2204105866771658151, 106.6745790697264056, -5.009819746185714351 ) ) ;
#18153=CARTESIAN_POINT ( 'NONE',  ( -15.73021646601979384, 121.2535323456646523, 0.2080526303901672758 ) ) ;
#18159=CARTESIAN_POINT ( 'NONE',  ( -10.18105065676974519, 125.9743313966586129, -0.2034416216762104657 ) ) ;
#18160=CARTESIAN_POINT ( 'NONE',  ( 6.376069600431401696, -13.97715805579494130, 0.6469259796868158663 ) ) ;
#18161=CARTESIAN_POINT ( 'NONE',  ( -17.34031924846188133, 128.5728276651957742, 1.378292450406111147 ) ) ;
#18162=CARTESIAN_POINT ( 'NONE',  ( 21.01108318401065134, 151.1643092826112138, -1.006483555388256068 ) ) ;
#18163=CARTESIAN_POINT ( 'NONE',  ( 4.636458409304901274, 17.36039413176390411, -0.09481320587925551324 ) ) ;
#18164=CARTESIAN_POINT ( 'NONE',  ( -17.01700507317055511, 122.6950552906510694, -0.6769824155666206433 ) ) ;
#18167=CARTESIAN_POINT ( 'NONE',  ( 5.562220668319040939, 116.6985801738751292, 0.1494643777500437865 ) ) ;
#18169=CARTESIAN_POINT ( 'NONE',  ( -15.51360955034724043, 150.7699688800196611, 1.541415763164774466 ) ) ;
#18171=CARTESIAN_POINT ( 'NONE',  ( 14.27152401005723448, 125.7140216354555804, -1.459898031787023376 ) ) ;
#18172=CARTESIAN_POINT ( 'NONE',  ( -12.00897459848981796, 120.6765805525287334, -1.550193712165490956 ) ) ;
#18175=CARTESIAN_POINT ( 'NONE',  ( 10.46017523140576344, 124.8149993102252182, -0.6249645713522342660 ) ) ;
#18177=CARTESIAN_POINT ( 'NONE',  ( -11.01279815837321863, 154.4909003399924643, -2.068435761307119147 ) ) ;
#18178=CARTESIAN_POINT ( 'NONE',  ( 3.827285340041869155, -15.59443631323044421, 3.224486442507772388 ) ) ;
#18179=CARTESIAN_POINT ( 'NONE',  ( -4.455953229021707429, 118.1125578900950757, -0.7543243153411564039 ) ) ;
#18181=TOROIDAL_SURFACE ( 'NONE', #36488, 3.683000000000000718, 0.5080000000000000071 ) ;
#18183=CARTESIAN_POINT ( 'NONE',  ( 15.43964774321182354, 150.7699688800196611, 2.159935508548367356 ) ) ;
#18184=CARTESIAN_POINT ( 'NONE',  ( 0.02537255736346701387, 39.20946620154573736, -1.269746523260778970 ) ) ;
#18185=CARTESIAN_POINT ( 'NONE',  ( -5.045332104996713696, -5.333490553104357268, 6.775881858851239947 ) ) ;
#18186=CARTESIAN_POINT ( 'NONE',  ( 14.74011517316798248, 148.8440819608433969, 0.7404754567584960201 ) ) ;
#18187=CARTESIAN_POINT ( 'NONE',  ( 4.801216665947148243, 117.4032681888235459, -1.015537427445656782 ) ) ;
#18190=CARTESIAN_POINT ( 'NONE',  ( -3.931412874456751361, 118.1588900401562938, 0.5787760988833658971 ) ) ;
#18195=CARTESIAN_POINT ( 'NONE',  ( -23.09707919911562612, 149.8924475812327159, -0.2317116236470734003 ) ) ;
#18196=ORIENTED_EDGE ( 'NONE', *, *, #15927, .T. ) ;
#18198=CARTESIAN_POINT ( 'NONE',  ( 7.924075518182773337, 122.0230495997628140, -0.6113557723677206512 ) ) ;
#18199=CARTESIAN_POINT ( 'NONE',  ( -8.072253591115543969, 121.3304565451442727, 0.9161511751190034580 ) ) ;
#18201=CARTESIAN_POINT ( 'NONE',  ( 1.648710697724705687, 115.6909491485466646, -1.667653344520376724 ) ) ;
#18202=CARTESIAN_POINT ( 'NONE',  ( -15.27538331669057570, 143.4753230507764670, -0.6393389556987904010 ) ) ;
#18203=CARTESIAN_POINT ( 'NONE',  ( 5.309946395046844181, -12.59883844183437596, 1.960244440597288529 ) ) ;
#18204=CARTESIAN_POINT ( 'NONE',  ( -21.68724320794237670, 149.9601031839316079, 1.147785971009648298 ) ) ;
#18206=CARTESIAN_POINT ( 'NONE',  ( 20.41771265994151463, 129.0384130229076334, 0.5332683426449600361 ) ) ;
#18207=CARTESIAN_POINT ( 'NONE',  ( 3.768629899957671281, 121.0935559710094509, 0.1102337842458726014 ) ) ;
#18208=FACE_OUTER_BOUND ( 'NONE', #27155, .T. ) ;
#18209=CARTESIAN_POINT ( 'NONE',  ( 0.03997419820544263758, 30.08235846857972007, -0.9743396344490610206 ) ) ;
#18210=CARTESIAN_POINT ( 'NONE',  ( 0.0002734175338603746100, 159.6054662015457382, -0.01368293144939978188 ) ) ;
#18214=CARTESIAN_POINT ( 'NONE',  ( 6.037009026191382688, 118.8442016224334594, 1.226040081825612527 ) ) ;
#18216=CARTESIAN_POINT ( 'NONE',  ( 21.32959265000921434, 150.3702682424204511, 2.003547396033109607 ) ) ;
#18218=CARTESIAN_POINT ( 'NONE',  ( 20.44439181834784236, 148.1475078817917961, -1.665223645801947594 ) ) ;
#18219=CARTESIAN_POINT ( 'NONE',  ( 7.630415381941168640, 23.66608445915806058, -3.560124470299026900 ) ) ;
#18220=CARTESIAN_POINT ( 'NONE',  ( -2.036215858770317855, 117.3535355059730705, -0.5825239229278258435 ) ) ;
#18221=CARTESIAN_POINT ( 'NONE',  ( 4.833494790946907038, 117.7366326795467586, -0.8572946300570807310 ) ) ;
#18222=CARTESIAN_POINT ( 'NONE',  ( 7.089375086749911681, 122.4291926079955317, 0.2513136963589434059 ) ) ;
#18224=CARTESIAN_POINT ( 'NONE',  ( -15.79579396213704001, 146.5797798787131399, -0.08547097745249035428 ) ) ;
#18225=CARTESIAN_POINT ( 'NONE',  ( -15.41952259888553911, 128.5596447653542498, -2.179146846741407906 ) ) ;
#18226=CARTESIAN_POINT ( 'NONE',  ( 2.659284927817582744, -15.52939239755456136, 5.761088356787748666 ) ) ;
#18229=CARTESIAN_POINT ( 'NONE',  ( -4.367291737180500455, 117.9496054766628674, -1.181649046108978585 ) ) ;
#18231=CARTESIAN_POINT ( 'NONE',  ( -0.01133701094408546065, 119.0130636887059410, 0.5673503866435171128 ) ) ;
#18232=CARTESIAN_POINT ( 'NONE',  ( -5.332935397695336199, 105.1224662015457199, -0.1065647409268299373 ) ) ;
#18233=CARTESIAN_POINT ( 'NONE',  ( -5.328528283132492938, 115.6909491485453003, -0.4166226019199130159 ) ) ;
#18234=CARTESIAN_POINT ( 'NONE',  ( -1.600813358578796031, 118.7759820277219944, 0.7642889039740425883 ) ) ;
#18235=CARTESIAN_POINT ( 'NONE',  ( -7.266063235143556120, -1.810023253287891487, -4.326994388187479501 ) ) ;
#18236=CARTESIAN_POINT ( 'NONE',  ( 5.869717882709199586, 121.2452591720019370, 0.5958057796325609834 ) ) ;
#18237=CARTESIAN_POINT ( 'NONE',  ( -4.787624606785451320, 118.5930653697794384, -0.9408880203060064895 ) ) ;
#18238=CARTESIAN_POINT ( 'NONE',  ( 6.914686169612705768, 117.4533518774869947, -0.3713220847589204787 ) ) ;
#18242=CARTESIAN_POINT ( 'NONE',  ( 2.081461833008364515, -15.42522581128936210, 5.972092850182500356 ) ) ;
#18243=CARTESIAN_POINT ( 'NONE',  ( -4.171376165246405421, 118.2392936340378498, 0.2183368768271861937 ) ) ;
#18244=CARTESIAN_POINT ( 'NONE',  ( -18.86374853661781970, 125.3403196291361610, -0.3769425889880997360 ) ) ;
#18247=CARTESIAN_POINT ( 'NONE',  ( 4.336810308868679797, 119.4260466530178348, -0.7558801875816598681 ) ) ;
#18248=CARTESIAN_POINT ( 'NONE',  ( -6.589702033682734540E-14, 87.97746620154572383, -4.338478393988997516E-18 ) ) ;
#18249=CARTESIAN_POINT ( 'NONE',  ( 4.426091836488892817, 118.1635172220246517, 0.6237344508278885868 ) ) ;
#18250=CARTESIAN_POINT ( 'NONE',  ( -4.418888662852294757, 155.8637389808261275, -0.7167756870077639508 ) ) ;
#18251=PRODUCT_DEFINITION_FORMATION_WITH_SPECIFIED_SOURCE ( 'ANY', '', #20129, .NOT_KNOWN. ) ;
#18253=CARTESIAN_POINT ( 'NONE',  ( 6.894732321505262718, 117.1676844715483270, 0.1377731603346603051 ) ) ;
#18256=CARTESIAN_POINT ( 'NONE',  ( -2.755274729907521980, 20.69627551736597226, -3.746277899328600558 ) ) ;
#18260=CARTESIAN_POINT ( 'NONE',  ( 7.788361015690092870, 122.6175610730192176, 0.07939682999910972760 ) ) ;
#18261=CARTESIAN_POINT ( 'NONE',  ( 6.070467230626295674, 121.4441374072678883, 0.2166268477916202806 ) ) ;
#18263=CARTESIAN_POINT ( 'NONE',  ( -2.133573495637306916, 19.78131850274109382, 4.120466288703205748 ) ) ;
#18264=CARTESIAN_POINT ( 'NONE',  ( 22.70157303802166737, 149.4207734315791072, 1.531927632650241788 ) ) ;
#18265=CARTESIAN_POINT ( 'NONE',  ( -4.502681726546150287, 104.6144662015457811, -1.767325709528040134 ) ) ;
#18266=CARTESIAN_POINT ( 'NONE',  ( 3.178324225997528618, -14.33742748831649827, 1.935164598152447679 ) ) ;
#18267=CARTESIAN_POINT ( 'NONE',  ( 20.87437586479479634, 150.1670661137953289, -1.386469220648549383 ) ) ;
#18268=CARTESIAN_POINT ( 'NONE',  ( -10.29797255167336978, 122.2012759285571946, 1.140151759267314269 ) ) ;
#18270=CARTESIAN_POINT ( 'NONE',  ( 2.838909340336904563, 21.51804255560577772, 3.663749385350952181 ) ) ;
#18271=CARTESIAN_POINT ( 'NONE',  ( -22.90231444567494989, 149.5023856264156450, -1.310353656364537045 ) ) ;
#18272=CARTESIAN_POINT ( 'NONE',  ( -0.9107729336552147226, 17.84451472381387305, 0.3451692354151053577 ) ) ;
#18276=CARTESIAN_POINT ( 'NONE',  ( -9.401300499464442240, 153.8930958044198576, 0.5598851911991608032 ) ) ;
#18277=CARTESIAN_POINT ( 'NONE',  ( 3.566861488287894844, -14.88765406650577283, 5.398167181214303945 ) ) ;
#18278=CARTESIAN_POINT ( 'NONE',  ( 7.304865317682085468, 121.1388872696715282, -0.8066302172824779682 ) ) ;
#18280=CARTESIAN_POINT ( 'NONE',  ( 1.556864280699287395, 115.7027529739286535, 1.730863229191432318 ) ) ;
#18282=CARTESIAN_POINT ( 'NONE',  ( -4.649178111515271716, 117.8875442298166831, -1.000802408407167166 ) ) ;
#18283=CARTESIAN_POINT ( 'NONE',  ( 15.77201034003348745, 145.9134097338176730, 0.1865891569459579291 ) ) ;
#18285=CARTESIAN_POINT ( 'NONE',  ( 8.897726962874816792, 119.7003323559047061, 1.444919796022273273 ) ) ;
#18286=DIRECTION ( 'NONE',  ( -4.017660918040594346E-17, 1.000000000000000000, 2.376309959284834438E-19 ) ) ;
#18289=CARTESIAN_POINT ( 'NONE',  ( 0.02969003158472036108, 157.1787724364823760, -1.485810588193620552 ) ) ;
#18290=CARTESIAN_POINT ( 'NONE',  ( 22.50450395291942129, 150.7830971219523519, 0.1219060866366472456 ) ) ;
#18292=CIRCLE ( 'NONE', #17630, 0.5080000000000002292 ) ;
#18293=CARTESIAN_POINT ( 'NONE',  ( 0.09909826073474366226, 106.8097931225389488, -4.959282197179095242 ) ) ;
#18295=CARTESIAN_POINT ( 'NONE',  ( 1.881137653242185959, -15.44088361928680442, 5.378024698638343537 ) ) ;
#18298=CARTESIAN_POINT ( 'NONE',  ( -4.757343136932370875, 117.8474671740875550, 0.8187060929519298647 ) ) ;
#18301=CARTESIAN_POINT ( 'NONE',  ( -3.208471139890875179, 118.3820369523956941, -0.9069343936787985783 ) ) ;
#18302=CARTESIAN_POINT ( 'NONE',  ( -4.850755190081010859, 117.2937442104795593, -0.9187341308512858573 ) ) ;
#18303=CARTESIAN_POINT ( 'NONE',  ( 4.744653392920721302, 117.6672350140714229, 1.125260125251866583 ) ) ;
#18305=CARTESIAN_POINT ( 'NONE',  ( -0.7705677718992680614, 119.3684187487962305, 0.7342037314787066560 ) ) ;
#18308=DIRECTION ( 'NONE',  ( -4.017660918040594346E-17, 1.000000000000000000, 2.376309959284834438E-19 ) ) ;
#18309=CARTESIAN_POINT ( 'NONE',  ( 2.845270837621566518, -14.55731563485390723, 4.954299782322259205 ) ) ;
#18310=CARTESIAN_POINT ( 'NONE',  ( 0.3027292972882736910, 105.9597790263619146, -5.298406829468305546 ) ) ;
#18311=CARTESIAN_POINT ( 'NONE',  ( -5.087176912069907075, 120.2090573957402455, -0.9271508619376559457 ) ) ;
#18312=B_SPLINE_CURVE_WITH_KNOTS ( 'NONE', 3,
 ( #33405, #30195, #14206, #822, #7421, #24002, #1036, #36812 ),
 .UNSPECIFIED., .F., .F.,
 ( 4, 2, 2, 4 ),
 ( 0.000000000000000000, 0.1320084156803643383, 0.1980126235205464935, 0.2567263020195166834 ),
 .UNSPECIFIED. ) ;
#18314=LINE ( 'NONE', #31954, #32608 ) ;
#18315=CARTESIAN_POINT ( 'NONE',  ( -0.5072216500879573875, 115.7034658939820417, 1.744308663346807897 ) ) ;
#18316=CARTESIAN_POINT ( 'NONE',  ( 4.585487687326599726, 17.13547844546973309, 0.5842699607688729424 ) ) ;
#18317=CARTESIAN_POINT ( 'NONE',  ( 23.20005416489656724, 148.7951734159264561, 1.060305963766563053 ) ) ;
#18319=CARTESIAN_POINT ( 'NONE',  ( 2.418018609469429148, 104.6144662015533555, -4.757618545730919024 ) ) ;
#18320=CARTESIAN_POINT ( 'NONE',  ( 2.046246934637348858, -15.60107924929197942, 5.318501171315276999 ) ) ;
#18321=CARTESIAN_POINT ( 'NONE',  ( -4.191956958763880969, 119.0775769483117870, 0.8365378509937178020 ) ) ;
#18322=CARTESIAN_POINT ( 'NONE',  ( 0.8739363859948088287, 22.79536383596403226, -0.4369566804381688208 ) ) ;
#18323=CARTESIAN_POINT ( 'NONE',  ( -0.1409938471676187022, 25.13008524939761656, 0.9676832235670267401 ) ) ;
#18326=VERTEX_POINT ( 'NONE', #20857 ) ;
#18327=LINE ( 'NONE', #8765, #22829 ) ;
#18328=CARTESIAN_POINT ( 'NONE',  ( 2.259516459295608737, 118.2243428780609662, 0.9293431707136512454 ) ) ;
#18329=CARTESIAN_POINT ( 'NONE',  ( -10.43918028506331730, 123.9810924921358151, 0.8290978625009026715 ) ) ;
#18331=CARTESIAN_POINT ( 'NONE',  ( 3.201139452527619333, -14.28037012539873274, 4.574913560108570643 ) ) ;
#18332=CARTESIAN_POINT ( 'NONE',  ( 0.5282936316506747776, 119.4440140289964774, -0.5434071943388011361 ) ) ;
#18333=CARTESIAN_POINT ( 'NONE',  ( -2.584978638890317537, 158.3255140430775043, -1.682483135129622998 ) ) ;
#18335=CARTESIAN_POINT ( 'NONE',  ( -10.39928917620371784, 153.1223395828141918, -0.2078025466733117443 ) ) ;
#18336=CARTESIAN_POINT ( 'NONE',  ( 4.123474937902314785, 118.2429491485453354, -0.1804386993445105669 ) ) ;
#18337=CARTESIAN_POINT ( 'NONE',  ( 9.835128631861913107, 124.8790005272986861, -0.1409026022053573302 ) ) ;
#18340=CARTESIAN_POINT ( 'NONE',  ( 2.831922340016455042, -13.93067033233365315, 0.4309514144534042912 ) ) ;
#18342=CARTESIAN_POINT ( 'NONE',  ( 0.9281906404964570534, 34.59732502943162302, 2.863135987906453739 ) ) ;
#18344=CARTESIAN_POINT ( 'NONE',  ( -1.959332070151295291, -8.942847522256865744, 4.198131957625402144 ) ) ;
#18345=CARTESIAN_POINT ( 'NONE',  ( 10.87485472805859210, 124.6990478933366404, 1.296628760762302823 ) ) ;
#18346=CARTESIAN_POINT ( 'NONE',  ( -2.746491374733735835, 29.57032072151200097, 1.693051300424941230 ) ) ;
#18347=CARTESIAN_POINT ( 'NONE',  ( -0.8777885371163713923, 105.9485402691003060, 5.279836415571006469 ) ) ;
#18348=EDGE_CURVE ( 'NONE', #31017, #32583, #15627, .T. ) ;
#18349=CARTESIAN_POINT ( 'NONE',  ( 3.728136974946417492, 6.765255174955887796, 2.739693761753763113 ) ) ;
#18350=CARTESIAN_POINT ( 'NONE',  ( 15.78437780952694069, 146.2378312303354448, 0.3154094333657936899 ) ) ;
#18351=CARTESIAN_POINT ( 'NONE',  ( -5.378050908718009282, 0.3500678860072145016, 6.480130142454380682 ) ) ;
#18353=CARTESIAN_POINT ( 'NONE',  ( -8.764338194681526417, 117.8116005833410043, -0.5569156411200119061 ) ) ;
#18354=CARTESIAN_POINT ( 'NONE',  ( -1.009032787326002323, 123.9312678891798640, -0.1103529103309998094 ) ) ;
#18357=CARTESIAN_POINT ( 'NONE',  ( -0.5673920217975719771, -4.456920702667952483, 8.403146712094516246 ) ) ;
#18358=CARTESIAN_POINT ( 'NONE',  ( 2.549837469103328313, 117.9394487944890955, 1.339571799219352100 ) ) ;
#18361=CARTESIAN_POINT ( 'NONE',  ( 0.3886773557327865558, 118.1497763966932695, -1.061209395727771509 ) ) ;
#18362=CARTESIAN_POINT ( 'NONE',  ( -8.185302851676581781, 117.6493956690293317, 0.2478838862282038424 ) ) ;
#18363=ORIENTED_EDGE ( 'NONE', *, *, #22449, .T. ) ;
#18367=CARTESIAN_POINT ( 'NONE',  ( -4.599243292695419427, 121.2024757821991159, -0.09190382657876439154 ) ) ;
#18368=CARTESIAN_POINT ( 'NONE',  ( 4.192023472006414231, -15.34368243816432198, 4.862536176465709126 ) ) ;
#18369=CARTESIAN_POINT ( 'NONE',  ( -6.947343058555404127, 158.0090104422344268, 1.506406725519188194 ) ) ;
#18370=CARTESIAN_POINT ( 'NONE',  ( 2.024878990865616846, 117.2046888992736200, -0.4535333368958820444 ) ) ;
#18371=CARTESIAN_POINT ( 'NONE',  ( -1.932895124392534303, 20.38400505531995321, -4.219463811995566083 ) ) ;
#18372=CARTESIAN_POINT ( 'NONE',  ( -23.26560126724731958, 148.8247458934765461, -0.9199859812867272613 ) ) ;
#18375=CARTESIAN_POINT ( 'NONE',  ( 2.183058710814191450, 116.1883852919004596, 0.05356175840457068349 ) ) ;
#18377=CARTESIAN_POINT ( 'NONE',  ( -0.009513407573735708014, 119.7614543879625586, 0.4760898169610159325 ) ) ;
#18379=CARTESIAN_POINT ( 'NONE',  ( 16.91343413265443729, 151.2926467857828072, -1.744909534579184074 ) ) ;
#18381=CARTESIAN_POINT ( 'NONE',  ( -11.86420439699956120, 156.4809912657682673, -1.954521554489340618 ) ) ;
#18383=CARTESIAN_POINT ( 'NONE',  ( 4.473055752542707708, 120.8671296916768227, -0.3242568198034685989 ) ) ;
#18384=ORIENTED_EDGE ( 'NONE', *, *, #7838, .T. ) ;
#18385=CARTESIAN_POINT ( 'NONE',  ( -12.00230265366671389, 124.3217332413628640, -1.707838685025481196 ) ) ;
#18386=CARTESIAN_POINT ( 'NONE',  ( 2.493951430369484523, -15.64112390455543711, 5.038688225235472551 ) ) ;
#18390=CARTESIAN_POINT ( 'NONE',  ( -4.848785805035457308, 117.5456108509605002, 0.9615705178007863951 ) ) ;
#18391=CARTESIAN_POINT ( 'NONE',  ( 17.72773402338096460, 148.0643276405518804, 2.286219595833943963 ) ) ;
#18394=AXIS2_PLACEMENT_3D ( 'NONE', #1279, #37053, #7245 ) ;
#18395=EDGE_CURVE ( 'NONE', #37991, #26452, #38174, .T. ) ;
#18396=CARTESIAN_POINT ( 'NONE',  ( -7.580879709009198386, 3.543476842659112780, 3.722543307504006194 ) ) ;
#18397=CARTESIAN_POINT ( 'NONE',  ( -0.001786757842290606548, 120.9379535345006076, 0.08941666878750630099 ) ) ;
#18400=EDGE_LOOP ( 'NONE', ( #20343, #40839, #15344, #35212 ) ) ;
#18401=CARTESIAN_POINT ( 'NONE',  ( -1.102837227558988831, 118.1588900165301652, 0.8471146098009928460 ) ) ;
#18402=AXIS2_PLACEMENT_3D ( 'NONE', #3027, #13644, #39643 ) ;
#18407=CARTESIAN_POINT ( 'NONE',  ( -15.44479738614508868, 120.7004057517279989, -0.1507993925391200030 ) ) ;
#18410=CARTESIAN_POINT ( 'NONE',  ( -7.836266847366137434, 122.3234956677103185, -0.6997315686990351891 ) ) ;
#18411=CARTESIAN_POINT ( 'NONE',  ( -8.343164213270990004, 120.0286413096533664, 1.117317573728694002 ) ) ;
#18413=CARTESIAN_POINT ( 'NONE',  ( 1.447157367358747004, 115.6909491485452719, -1.681836580404131087 ) ) ;
#18414=CARTESIAN_POINT ( 'NONE',  ( -7.049298115861525105, 122.0434499869739540, -0.3314598731120508290 ) ) ;
#18415=CARTESIAN_POINT ( 'NONE',  ( 5.179289707447474633, -13.00434337860746581, 2.646125397160491222 ) ) ;
#18416=CARTESIAN_POINT ( 'NONE',  ( -22.03832501185546633, 149.1257232373000647, 1.146528549967842370 ) ) ;
#18418=CARTESIAN_POINT ( 'NONE',  ( 18.71175911766644617, 125.2636347375217838, 0.5504587009833171729 ) ) ;
#18419=CARTESIAN_POINT ( 'NONE',  ( 15.76967257419122781, 146.5682726256061130, 0.3822029702838447007 ) ) ;
#18421=CARTESIAN_POINT ( 'NONE',  ( 0.3093957028193324299, 29.65535775802675289, -0.9258560203679269129 ) ) ;
#18422=CARTESIAN_POINT ( 'NONE',  ( -21.90252518039365981, 151.4352167165723415, -0.5139180553509251625 ) ) ;
#18424=CARTESIAN_POINT ( 'NONE',  ( -7.383526124176625238, 117.2783386306103921, -0.1475404267317128315 ) ) ;
#18426=CARTESIAN_POINT ( 'NONE',  ( 2.893028018094861320, 117.2553914413831535, 0.7100786824799962815 ) ) ;
#18428=CARTESIAN_POINT ( 'NONE',  ( 9.289280848106727717, 118.8811571165754941, 1.201727579052786599 ) ) ;
#18429=CARTESIAN_POINT ( 'NONE',  ( 2.710741864450562755, 158.4754809254847601, -1.535472453293832418 ) ) ;
#18430=CARTESIAN_POINT ( 'NONE',  ( 7.231359443275770182, 22.16797014818540745, 4.386519482779798196 ) ) ;
#18431=CARTESIAN_POINT ( 'NONE',  ( -14.73734951358261824, 121.3346631531286164, -1.319546682830233797 ) ) ;
#18432=CARTESIAN_POINT ( 'NONE',  ( 4.746482201166442927, 117.7550804213460651, -0.8965027487333476763 ) ) ;
#18434=CARTESIAN_POINT ( 'NONE',  ( 5.469471049222477177, 117.5088849381099436, 0.8278104034524698118 ) ) ;
#18436=CARTESIAN_POINT ( 'NONE',  ( -15.23158847265895410, 143.4365109762209158, -0.1756275167766374046 ) ) ;
#18437=CARTESIAN_POINT ( 'NONE',  ( -6.637665810843349057, 119.8184877057495754, -1.268479684707346289 ) ) ;
#18438=CARTESIAN_POINT ( 'NONE',  ( 3.006733222167471631, -15.59844357659602387, 5.538909454127313836 ) ) ;
#18440=CARTESIAN_POINT ( 'NONE',  ( 4.787476607852438448, 115.6909491485453145, 1.476299238943078906 ) ) ;
#18441=CARTESIAN_POINT ( 'NONE',  ( -0.9880787409092588458, 117.9496054967312375, -1.392611192464434211 ) ) ;
#18443=CARTESIAN_POINT ( 'NONE',  ( 1.300143943178173833, 119.1766673560425858, 0.6697961403939317604 ) ) ;
#18444=CARTESIAN_POINT ( 'NONE',  ( -6.591743005429100447E-14, 88.48546620154573361, -4.217761848057333172E-18 ) ) ;
#18447=CARTESIAN_POINT ( 'NONE',  ( -2.162440637018797407, 123.3349985135950959, 0.07568789353404307974 ) ) ;
#18448=CARTESIAN_POINT ( 'NONE',  ( -8.215080244096204964, -10.21703095211954704, 2.011605797521776928 ) ) ;
#18449=CARTESIAN_POINT ( 'NONE',  ( 3.075464349291132216, 156.1450793681712241, 0.7387695966741768538 ) ) ;
#18451=ADVANCED_FACE ( 'NONE', ( #7688, #24473 ), #10655, .F. ) ;
#18452=CARTESIAN_POINT ( 'NONE',  ( 7.877688851764411915, 158.6543443936584481, -0.4710593659051897641 ) ) ;
#18455=CARTESIAN_POINT ( 'NONE',  ( -5.562421465964138001, 116.6996505075888422, -0.1685898161880411972 ) ) ;
#18458=CARTESIAN_POINT ( 'NONE',  ( -4.168157594931272136, 118.2394498548492265, 0.2219570363417781578 ) ) ;
#18459=CARTESIAN_POINT ( 'NONE',  ( 3.174366308151880922, 104.6144662015457243, 0.06343139340882769650 ) ) ;
#18462=CARTESIAN_POINT ( 'NONE',  ( 4.359163536690966900, 119.4473459596788842, -0.7549756355859075230 ) ) ;
#18464=CARTESIAN_POINT ( 'NONE',  ( -16.04872481256650829, 146.6973543426590254, -1.173426683271128868 ) ) ;
#18465=CARTESIAN_POINT ( 'NONE',  ( 4.959033476919109340, 117.6447102886128988, -0.6722175906395938538 ) ) ;
#18466=CARTESIAN_POINT ( 'NONE',  ( 0.1336191844408766705, 117.3993836134489044, -1.490790351259109414 ) ) ;
#18468=CARTESIAN_POINT ( 'NONE',  ( -4.598301960400187127, 22.30806413504685537, 0.5496829067130363233 ) ) ;
#18471=DIRECTION ( 'NONE',  ( -5.206863593109713661E-17, 1.000000000000000000, -1.077750396879097183E-30 ) ) ;
#18473=CARTESIAN_POINT ( 'NONE',  ( 6.071400464523738272, 121.4469273266857670, 0.1932373124915481855 ) ) ;
#18474=CARTESIAN_POINT ( 'NONE',  ( 5.332935397695205637, 105.1224662015457199, 0.1065647409268305201 ) ) ;
#18475=CARTESIAN_POINT ( 'NONE',  ( 2.899385524442493534, 117.0242007548465608, 0.5112881796358940134 ) ) ;
#18476=CARTESIAN_POINT ( 'NONE',  ( 4.808131379915037584, 104.6144662015457527, -0.4149153341867691802 ) ) ;
#18477=CARTESIAN_POINT ( 'NONE',  ( 1.850858793973401584, -15.28950465061244834, 5.390636727418374186 ) ) ;
#18478=CARTESIAN_POINT ( 'NONE',  ( 21.26977539036077403, 145.8710773725474610, -1.472442194194814702 ) ) ;
#18479=CARTESIAN_POINT ( 'NONE',  ( -4.278356142284035712, 119.7015364213435333, 0.7555980432150397608 ) ) ;
#18480=CARTESIAN_POINT ( 'NONE',  ( 1.072590735131739414, 20.86836736082219801, 4.503669761903479341 ) ) ;
#18481=CARTESIAN_POINT ( 'NONE',  ( -10.49915001570439266, 157.9057380314836223, -0.9855651801815565882 ) ) ;
#18482=CARTESIAN_POINT ( 'NONE',  ( -0.7773729966126706747, -2.891840825076433585, -0.5888577047253038543 ) ) ;
#18485=CARTESIAN_POINT ( 'NONE',  ( -9.542306315654425219, 124.2661852542617709, 0.2373755145837090630 ) ) ;
#18486=CARTESIAN_POINT ( 'NONE',  ( 2.287996554222524903, -15.35138490607948469, 5.941601703801219436 ) ) ;
#18487=CARTESIAN_POINT ( 'NONE',  ( 16.63213601294257415, 144.0643239018434940, -1.266953209168786953 ) ) ;
#18489=CARTESIAN_POINT ( 'NONE',  ( 3.014676604589255238, 115.7029491485453292, 1.668003145632996231 ) ) ;
#18491=CARTESIAN_POINT ( 'NONE',  ( -4.858315324244927069, 117.7455535390209604, -0.9239789875634819571 ) ) ;
#18492=EDGE_CURVE ( 'NONE', #22451, #13790, #8770, .T. ) ;
#18493=CARTESIAN_POINT ( 'NONE',  ( 8.935197197525127422, 123.9063447689825779, 0.1785465045940571871 ) ) ;
#18495=CARTESIAN_POINT ( 'NONE',  ( 7.650403556475533939, 119.6133147451300971, 1.381840873585064688 ) ) ;
#18496=CARTESIAN_POINT ( 'NONE',  ( -6.503981220335420706E-14, 66.64146620154573952, -9.408573323119121831E-18 ) ) ;
#18497=CARTESIAN_POINT ( 'NONE',  ( 3.682264917456193665, 69.43546620154573645, 0.07358041635423968885 ) ) ;
#18499=CARTESIAN_POINT ( 'NONE',  ( 0.002459401150240396027, 159.6023738651833810, -0.1230784904792617679 ) ) ;
#18500=CARTESIAN_POINT ( 'NONE',  ( 20.66439279448287181, 152.5811724025633112, 0.09276230403812320280 ) ) ;
#18502=CARTESIAN_POINT ( 'NONE',  ( 4.854022926505809465, 118.7629491485453030, -0.1809382747281913784 ) ) ;
#18503=CARTESIAN_POINT ( 'NONE',  ( 1.803749805595953326, -15.30621593874753650, 5.393099756912645759 ) ) ;
#18504=DIRECTION ( 'NONE',  ( -5.206863593109713661E-17, 1.000000000000000000, -1.077750396879097183E-30 ) ) ;
#18507=CARTESIAN_POINT ( 'NONE',  ( -4.767607816231247853, 117.8956932628570513, 0.7411698513071134364 ) ) ;
#18511=CARTESIAN_POINT ( 'NONE',  ( -8.406060086832516376, 119.4770703846445059, -1.395343900433620110 ) ) ;
#18512=CARTESIAN_POINT ( 'NONE',  ( -4.819599041176440224, 120.7138498849978987, -0.4051376471031730153 ) ) ;
#18513=CARTESIAN_POINT ( 'NONE',  ( 4.911660101568102732, 117.6260080863869320, 0.9594402546315066171 ) ) ;
#18515=CARTESIAN_POINT ( 'NONE',  ( -1.058122102717379942, 124.9344662015457459, -0.02114379780294212835 ) ) ;
#18520=CARTESIAN_POINT ( 'NONE',  ( 3.391857759029038633, -13.93828481737184610, 3.530066096054821134 ) ) ;
#18521=CARTESIAN_POINT ( 'NONE',  ( 3.253275476659236443, 108.9521120498200730, -3.903703133364782030 ) ) ;
#18522=CARTESIAN_POINT ( 'NONE',  ( -7.266810130343835716, 121.1388872696715282, -1.097806971394259312 ) ) ;
#18523=CARTESIAN_POINT ( 'NONE',  ( -7.785295067471754926, 122.6196652447830502, -0.2112362379013654756 ) ) ;
#18525=EDGE_CURVE ( 'NONE', #11900, #23570, #33383, .T. ) ;
#18526=CARTESIAN_POINT ( 'NONE',  ( -0.2141370455737806877, 115.7030700810080930, 1.756908310108165505 ) ) ;
#18527=CARTESIAN_POINT ( 'NONE',  ( 4.419457123578296454, 17.78516144714274105, -1.360477052881604143 ) ) ;
#18528=CARTESIAN_POINT ( 'NONE',  ( 18.48423909989026725, 154.1703991122031994, 0.9245180971295520189 ) ) ;
#18530=CARTESIAN_POINT ( 'NONE',  ( 2.860261174899399350, 104.6144662015456959, -3.897939397042970544 ) ) ;
#18531=CARTESIAN_POINT ( 'NONE',  ( 4.104683988343100332, -15.63859574289259946, 3.129333468668611840 ) ) ;
#18532=CARTESIAN_POINT ( 'NONE',  ( -12.06323264149831154, 122.4500365997666336, 1.303827596403756672 ) ) ;
#18533=CARTESIAN_POINT ( 'NONE',  ( 0.9751022921854990422, 22.16746322748675624, -0.05045228706074462999 ) ) ;
#18534=CARTESIAN_POINT ( 'NONE',  ( 0.9280917288853990366, 18.63875360461660335, -0.3060232888646727822 ) ) ;
#18535=EDGE_CURVE ( 'NONE', #1100, #18074, #35136, .T. ) ;
#18540=CARTESIAN_POINT ( 'NONE',  ( 3.998531074477424507, 117.0582680968029905, 1.101271957883943164 ) ) ;
#18541=CARTESIAN_POINT ( 'NONE',  ( -16.05848832435436435, 147.7157881801689427, 0.7882342824236393541 ) ) ;
#18543=CARTESIAN_POINT ( 'NONE',  ( 3.377503200524144322, -12.59127376242380514, 1.184662976626496000 ) ) ;
#18544=CARTESIAN_POINT ( 'NONE',  ( 0.5414988153859304765, 119.6443647996702566, -0.5124704023889977700 ) ) ;
#18545=CARTESIAN_POINT ( 'NONE',  ( -19.94553544501724573, 148.6304843473828043, -2.499072228797274864 ) ) ;
#18548=CARTESIAN_POINT ( 'NONE',  ( -3.682264917456324227, 88.48546620154573361, -0.07358041635423923088 ) ) ;
#18549=CARTESIAN_POINT ( 'NONE',  ( -3.991072007095600949, 33.40439263831326855, 3.842775004540742501 ) ) ;
#18550=CARTESIAN_POINT ( 'NONE',  ( 15.40459090795122776, 148.0444422243178337, -0.2810841713230231020 ) ) ;
#18551=ORIENTED_EDGE ( 'NONE', *, *, #7890, .F. ) ;
#18552=CARTESIAN_POINT ( 'NONE',  ( 2.567065079198288746, -15.08448375773686934, 4.691402903081304920 ) ) ;
#18557=CARTESIAN_POINT ( 'NONE',  ( -4.626086514281606554, -10.66701884381306087, 0.02375484599842511355 ) ) ;
#18558=CARTESIAN_POINT ( 'NONE',  ( 16.27782172975856412, 148.1602266505728380, 1.760797687140677414 ) ) ;
#18559=FACE_OUTER_BOUND ( 'NONE', #41194, .T. ) ;
#18560=CARTESIAN_POINT ( 'NONE',  ( 3.715898061424960375, 116.6275173757784813, 0.03328880940299697860 ) ) ;
#18561=CARTESIAN_POINT ( 'NONE',  ( -7.669269000495163802, 124.9344662015457317, -0.1532502464757266036 ) ) ;
#18563=CARTESIAN_POINT ( 'NONE',  ( -3.158589313471108273, 4.191505055319898254, 3.400481138232230194 ) ) ;
#18564=CARTESIAN_POINT ( 'NONE',  ( 4.223292309264916611, 155.8535809751167562, 0.1210084730045380141 ) ) ;
#18566=CARTESIAN_POINT ( 'NONE',  ( -1.603550922812138735, -3.093932695209369754, -8.287855504117967342 ) ) ;
#18568=CARTESIAN_POINT ( 'NONE',  ( 2.165612022977871920, 116.6455396352414624, -0.3652780253405325528 ) ) ;
#18569=CARTESIAN_POINT ( 'NONE',  ( -0.3459730346048953131, 118.1497763966932695, -1.075889458897477668 ) ) ;
#18571=CARTESIAN_POINT ( 'NONE',  ( -3.991072007095600949, 33.40439263831326855, 3.842775004540742501 ) ) ;
#18572=CARTESIAN_POINT ( 'NONE',  ( -4.559029627765868398, 31.49133049583988253, -0.6947656260628575220 ) ) ;
#18573=CARTESIAN_POINT ( 'NONE',  ( 0.7773589538612868388, 118.1588881499372832, 0.8997936918793348893 ) ) ;
#18576=CARTESIAN_POINT ( 'NONE',  ( 0.2562694446381907354, 108.5751225745497806, -4.260274975122999130 ) ) ;
#18577=CARTESIAN_POINT ( 'NONE',  ( -23.01821387067777991, 149.5377445326608665, 0.2676165590851173892 ) ) ;
#18578=EDGE_CURVE ( 'NONE', #17268, #38830, #36142, .T. ) ;
#18584=CARTESIAN_POINT ( 'NONE',  ( -15.53033519385735417, 147.5364864818501189, -0.1767648362992366440 ) ) ;
#18585=CARTESIAN_POINT ( 'NONE',  ( 3.223661160190148145, -15.48894043311785396, 5.519697737696615647 ) ) ;
#18586=CARTESIAN_POINT ( 'NONE',  ( -18.13891979603535631, 131.7244750738095149, 1.506900917850658050 ) ) ;
#18587=CARTESIAN_POINT ( 'NONE',  ( 3.950580610160879580, 117.4679918459733585, -0.5815556119072163854 ) ) ;
#18588=CARTESIAN_POINT ( 'NONE',  ( -3.234384296441582762, 11.31316835407710819, -3.315160845070126427 ) ) ;
#18589=CARTESIAN_POINT ( 'NONE',  ( -15.81407516854451245, 121.2341309109925334, -0.7422539548746109883 ) ) ;
#18591=CIRCLE ( 'NONE', #32901, 5.080000000000006288 ) ;
#18592=ORIENTED_EDGE ( 'NONE', *, *, #37489, .F. ) ;
#18593=CARTESIAN_POINT ( 'NONE',  ( 2.182332163943836001, 116.1897970688731760, 0.04360819029793291252 ) ) ;
#18594=CARTESIAN_POINT ( 'NONE',  ( -0.02615319344480911481, 156.8698190429800832, 1.308812744920978322 ) ) ;
#18597=CARTESIAN_POINT ( 'NONE',  ( 10.65007529713506962, 155.7851685111067184, -1.746298732392691289 ) ) ;
#18598=CARTESIAN_POINT ( 'NONE',  ( -13.40516742707921516, 121.5866728338796463, -1.646856811522066089 ) ) ;
#18600=AXIS2_PLACEMENT_3D ( 'NONE', #11391, #24377, #21798 ) ;
#18602=CARTESIAN_POINT ( 'NONE',  ( 12.88338908221804324, 130.8243885708800747, -0.7627239795610333273 ) ) ;
#18603=ORIENTED_EDGE ( 'NONE', *, *, #10800, .T. ) ;
#18604=CARTESIAN_POINT ( 'NONE',  ( -9.190671247346116957, 121.6705353891887995, -1.423780222299954046 ) ) ;
#18605=CARTESIAN_POINT ( 'NONE',  ( 4.210067206397440032, -15.44688347603401191, 1.362376457177303157 ) ) ;
#18606=CARTESIAN_POINT ( 'NONE',  ( -4.108446860257354061, 118.2429491485453070, -0.3498540877621626466 ) ) ;
#18608=CARTESIAN_POINT ( 'NONE',  ( -4.799585727462988949, 117.4716807894286461, 1.004530280717990331 ) ) ;
#18609=CARTESIAN_POINT ( 'NONE',  ( 11.20916139128192235, 123.4744472594011739, 1.589032359792267757 ) ) ;
#18610=FACE_OUTER_BOUND ( 'NONE', #41492, .T. ) ;
#18611=AXIS2_PLACEMENT_3D ( 'NONE', #40046, #20621, #24244 ) ;
#18612=CARTESIAN_POINT ( 'NONE',  ( -1.796629210684171918, -4.683219827815034542, 8.244768259809569955 ) ) ;
#18613=CARTESIAN_POINT ( 'NONE',  ( 7.049298115861396319, 122.0434499869739540, 0.3314598731120510511 ) ) ;
#18617=ORIENTED_EDGE ( 'NONE', *, *, #42077, .F. ) ;
#18618=CARTESIAN_POINT ( 'NONE',  ( -0.5515347699655459568, 117.3993826269703362, 1.472900392318948093 ) ) ;
#18620=CARTESIAN_POINT ( 'NONE',  ( -7.974902364581113900, 121.6049040996757782, -1.136138042282031968 ) ) ;
#18624=CARTESIAN_POINT ( 'NONE',  ( -22.82234304556254401, 150.4043717142618277, -0.2269822898261399657 ) ) ;
#18625=EDGE_LOOP ( 'NONE', ( #12891, #3525, #462, #10328 ) ) ;
#18627=CARTESIAN_POINT ( 'NONE',  ( 7.852298358788947219, 122.3486847557867208, -0.3610446264703879860 ) ) ;
#18628=CARTESIAN_POINT ( 'NONE',  ( -8.348968351562039203, 120.0002459142761211, 1.116349756213214972 ) ) ;
#18630=CARTESIAN_POINT ( 'NONE',  ( 2.051617846517921340, 115.7029490350661405, -1.635872274556314121 ) ) ;
#18631=CARTESIAN_POINT ( 'NONE',  ( -15.22644562805688295, 143.4365109762209158, -0.4329964906482475229 ) ) ;
#18633=CARTESIAN_POINT ( 'NONE',  ( 2.999908722124702720, -15.10219813539979938, 5.696538855611934515 ) ) ;
#18634=CARTESIAN_POINT ( 'NONE',  ( -21.56827676951031236, 148.6087350971780836, 1.383610176320235308 ) ) ;
#18635=CARTESIAN_POINT ( 'NONE',  ( 1.028482355383298241, 117.3993836102110464, -1.440227903949694577 ) ) ;
#18636=CARTESIAN_POINT ( 'NONE',  ( 20.28976221201013175, 128.9598305440861452, 0.6839793015867966508 ) ) ;
#18637=CARTESIAN_POINT ( 'NONE',  ( 7.775851458259090521, 154.6677978696501725, 0.2111400444086546369 ) ) ;
#18639=CARTESIAN_POINT ( 'NONE',  ( 0.2459283266301676152, 20.16186220226971315, -0.9436028068393225166 ) ) ;
#18640=CARTESIAN_POINT ( 'NONE',  ( -22.66113959641441511, 150.6410255081855212, -0.5295512721432396042 ) ) ;
#18641=CARTESIAN_POINT ( 'NONE',  ( -6.651972016613293606E-14, 104.1064662015457287, 7.011588703784780528E-31 ) ) ;
#18644=CARTESIAN_POINT ( 'NONE',  ( 8.329591456240351022, 119.8454013155109834, 1.442285711102194723 ) ) ;
#18645=CARTESIAN_POINT ( 'NONE',  ( 7.956670401304478446, 118.4344479264803169, 1.111586840565143675 ) ) ;
#18646=CARTESIAN_POINT ( 'NONE',  ( 7.786520497867073232, 119.2688035297948659, -1.033142384104571043 ) ) ;
#18648=CARTESIAN_POINT ( 'NONE',  ( -5.424866478234207534, 26.46299946464603181, -6.465121161284864471 ) ) ;
#18649=CARTESIAN_POINT ( 'NONE',  ( -14.30926610799427934, 121.2650221238243944, -1.406141635412307300 ) ) ;
#18650=CARTESIAN_POINT ( 'NONE',  ( 4.905962780720105165, 117.7163134916238363, -0.7387128614738237564 ) ) ;
#18652=CARTESIAN_POINT ( 'NONE',  ( 5.227922695814323006, 116.4790307410953289, 1.091139864702252549 ) ) ;
#18653=B_SPLINE_CURVE_WITH_KNOTS ( 'NONE', 3,
 ( #34928, #5756, #23146, #7003, #36183, #29575, #19129, #6162, #29355, #3816, #411, #2967, #35967, #10177, #39161, #6365, #19973, #22310 ),
 .UNSPECIFIED., .F., .F.,
 ( 4, 1, 1, 1, 1, 1, 2, 1, 1, 1, 2, 1, 1, 4 ),
 ( 0.000000000000000000, 0.1631003137318064733, 0.3262006274636129466, 0.4077507843295161694, 0.4893009411954193921, 0.5708510980613227259, 0.6524012549272260042, 0.6576100072399926333, 0.6628187595527593734, 0.6680275118655260025, 0.6732362641782927426, 0.7053937736304701778, 0.7375512830826475019, 0.7543499533669120183 ),
 .UNSPECIFIED. ) ;
#18654=CARTESIAN_POINT ( 'NONE',  ( -5.292481242636031702, 121.3432423864224177, -0.03610140192510977175 ) ) ;
#18655=CARTESIAN_POINT ( 'NONE',  ( -2.358209769532914724, 119.0637060312156024, -0.7902384042126600061 ) ) ;
#18656=CARTESIAN_POINT ( 'NONE',  ( 2.643346398695107347, -15.60183157139904964, 5.704389875863137505 ) ) ;
#18658=CARTESIAN_POINT ( 'NONE',  ( -2.723305694757628626, 118.1651002906158539, -0.8146868860962922509 ) ) ;
#18660=CARTESIAN_POINT ( 'NONE',  ( 18.80567741551205785, 148.1672603684278329, 2.476295349149460812 ) ) ;
#18663=CARTESIAN_POINT ( 'NONE',  ( -2.994815693583476879, 122.7580772961051707, 0.09506955764664398734 ) ) ;
#18664=CARTESIAN_POINT ( 'NONE',  ( 4.267473507877284078, -4.198009126799147062, -7.300781474974544771 ) ) ;
#18665=CARTESIAN_POINT ( 'NONE',  ( 8.311356586561950976, 122.7091975629380585, 0.7066836605292580176 ) ) ;
#18667=CARTESIAN_POINT ( 'NONE',  ( 22.01496335533477833, 136.8935083344700558, -0.5016514318445886023 ) ) ;
#18672=CARTESIAN_POINT ( 'NONE',  ( -0.2924095564369283418, 116.4254662015451913, -0.005843038833676939166 ) ) ;
#18675=CARTESIAN_POINT ( 'NONE',  ( -4.830459837891577735, 119.9522586551379817, -0.8951123600124439861 ) ) ;
#18676=CARTESIAN_POINT ( 'NONE',  ( -5.260208640450895423, 116.0444662015457595, -1.274361246762516942 ) ) ;
#18677=CARTESIAN_POINT ( 'NONE',  ( -0.6802018490772304693, 156.3636429644085695, -0.5246204485115751881 ) ) ;
#18678=CARTESIAN_POINT ( 'NONE',  ( 5.035933200060415338, 117.3993844219003648, -0.5513780243448201945 ) ) ;
#18679=CARTESIAN_POINT ( 'NONE',  ( 0.2924095564367995559, 116.4254662015451913, 0.005843038833676869777 ) ) ;
#18681=CARTESIAN_POINT ( 'NONE',  ( 4.377640660406503237, 26.40621510375495973, 1.544744264128281364 ) ) ;
#18685=CARTESIAN_POINT ( 'NONE',  ( 6.994627636368861978, 121.9501463612105425, 0.2166421691076159950 ) ) ;
#18686=CARTESIAN_POINT ( 'NONE',  ( -3.990024091077861268, 18.91925256873344807, 2.329872802929966902 ) ) ;
#18687=CARTESIAN_POINT ( 'NONE',  ( 22.64839633469820868, 142.3612397021088611, 1.542087416992684146 ) ) ;
#18690=CARTESIAN_POINT ( 'NONE',  ( 21.33845497820654202, 148.5140355411650717, -1.460612514688959029 ) ) ;
#18691=CARTESIAN_POINT ( 'NONE',  ( -9.322612814602798892, 121.5662863950884400, 1.087844926965479964 ) ) ;
#18692=CARTESIAN_POINT ( 'NONE',  ( -0.9239673467531356321, 25.61616486456964736, -4.531977062890359065 ) ) ;
#18693=CARTESIAN_POINT ( 'NONE',  ( -22.26995438616712519, 150.5193240506149550, -1.407572089812798799 ) ) ;
#18694=CARTESIAN_POINT ( 'NONE',  ( -0.8879284396340286767, 8.347861319067646946, 0.4041202799994399464 ) ) ;
#18697=CARTESIAN_POINT ( 'NONE',  ( -3.676778326629141169, 120.9289264519876070, 0.1742216996082329994 ) ) ;
#18698=CARTESIAN_POINT ( 'NONE',  ( 4.549387865739121573, -13.93190642666217194, 4.188617477609191120 ) ) ;
#18699=CARTESIAN_POINT ( 'NONE',  ( 10.40651172546656333, 123.5464890276372785, -0.9122707376378307309 ) ) ;
#18701=CARTESIAN_POINT ( 'NONE',  ( 1.900651210107762834, 115.7024232297718100, 1.719628578966114096 ) ) ;
#18702=CARTESIAN_POINT ( 'NONE',  ( -4.716505708007757036, 117.7575842814051299, -1.081295402246875037 ) ) ;
#18703=CARTESIAN_POINT ( 'NONE',  ( -7.220421660630267272E-14, 120.9974662015457341, -1.809054757420055726E-18 ) ) ;
#18706=CARTESIAN_POINT ( 'NONE',  ( 1.216597929035199588, 118.5604221528582372, 0.6894197161374838734 ) ) ;
#18708=DIRECTION ( 'NONE',  ( -0.9998004120163609398, 0.000000000000000000, -0.01997839162482749689 ) ) ;
#18709=CARTESIAN_POINT ( 'NONE',  ( 4.995400918032669502, 117.4677412550548610, -0.7873132084926519614 ) ) ;
#18710=CARTESIAN_POINT ( 'NONE',  ( 23.04498962259524930, 149.8694456586574972, 0.007884547560928708426 ) ) ;
#18715=CARTESIAN_POINT ( 'NONE',  ( 1.740647812522833959, -15.18628559522394639, 5.503367792502267264 ) ) ;
#18718=CARTESIAN_POINT ( 'NONE',  ( -4.555200029879727275, 118.0893311008628501, 0.5840147855654914677 ) ) ;
#18719=B_SPLINE_CURVE_WITH_KNOTS ( 'NONE', 3,
 ( #10701, #14105, #37326, #27104, #14519, #11538, #40536, #39908, #27729, #24318, #7940, #23681, #7523, #20700, #33724, #8141 ),
 .UNSPECIFIED., .F., .F.,
 ( 4, 2, 1, 1, 2, 2, 2, 2, 4 ),
 ( 0.000000000000000000, 0.06250000000000000000, 0.1250000000000000000, 0.2500000000000000000, 0.5000000000000000000, 0.6250000000000000000, 0.7500000000000000000, 0.8750000000000000000, 1.000000000000000000 ),
 .UNSPECIFIED. ) ;
#18721=CARTESIAN_POINT ( 'NONE',  ( -0.7080441033280816532, 118.7629491485454025, 1.246623510331355211 ) ) ;
#18722=CARTESIAN_POINT ( 'NONE',  ( -3.504900662208191520, 118.6790270643119527, -0.9350548551792551288 ) ) ;
#18723=CARTESIAN_POINT ( 'NONE',  ( -2.643983731439692786, 108.0685014782224442, -4.389169220726125253 ) ) ;
#18724=CARTESIAN_POINT ( 'NONE',  ( 4.642288039849367998, 117.9634434738006092, 0.9175853795829764792 ) ) ;
#18725=CARTESIAN_POINT ( 'NONE',  ( 1.979187190576821465, -15.21425526833739639, 5.301287498526151332 ) ) ;
#18726=CARTESIAN_POINT ( 'NONE',  ( -0.3781434503562681737, 120.9711055683163323, 0.4753422346318208480 ) ) ;
#18727=CARTESIAN_POINT ( 'NONE',  ( 1.968029828064305153, -3.592386099649644837, 4.203610184747879508 ) ) ;
#18728=CARTESIAN_POINT ( 'NONE',  ( 4.814838716269237651, 117.4047667081807305, -1.012532368900667556 ) ) ;
#18730=CARTESIAN_POINT ( 'NONE',  ( 1.441108623025248781, 106.3840144300045409, -5.062828720429449980 ) ) ;
#18731=CARTESIAN_POINT ( 'NONE',  ( -5.146579651471840045, 156.3268443366877989, -1.619031734741227968 ) ) ;
#18732=CARTESIAN_POINT ( 'NONE',  ( 6.078424119085688027, 121.4421096791099188, 0.1217658744218859945 ) ) ;
#18733=CARTESIAN_POINT ( 'NONE',  ( 0.4675636154070875738, 39.04908508565743830, 1.310637636393764627 ) ) ;
#18735=CARTESIAN_POINT ( 'NONE',  ( -4.855072294470597072, 115.7029491485453718, 1.279409886141102071 ) ) ;
#18736=CARTESIAN_POINT ( 'NONE',  ( 4.087030650986479330, 6.990161447142720696, 2.163025551504125232 ) ) ;
#18737=CARTESIAN_POINT ( 'NONE',  ( 9.693497654998099122, 118.1218853900603136, 0.6301662642801912906 ) ) ;
#18739=CARTESIAN_POINT ( 'NONE',  ( -0.1152527507162018766, 104.6144662015368851, -5.344087831667617472 ) ) ;
#18740=CARTESIAN_POINT ( 'NONE',  ( 4.222520559145931607, -15.42613134656034646, 1.120547993087879446 ) ) ;
#18741=CARTESIAN_POINT ( 'NONE',  ( -15.49426794143308683, 128.5596447653542498, 1.561415741013214120 ) ) ;
#18742=CARTESIAN_POINT ( 'NONE',  ( -0.2169513509689728059, 19.34598098455444770, 0.9497947498389193166 ) ) ;
#18743=CARTESIAN_POINT ( 'NONE',  ( 0.6244633603679663469, 9.902617207799803367, -0.7572168304597820532 ) ) ;
#18748=CARTESIAN_POINT ( 'NONE',  ( -4.908369780149227424, 117.6445054487819704, -0.9443798348817722399 ) ) ;
#18749=CARTESIAN_POINT ( 'NONE',  ( 0.7907262360440370230, 106.8474934270474392, 4.937153267606968932 ) ) ;
#18751=CARTESIAN_POINT ( 'NONE',  ( -11.19133892028646926, 126.1638007343821641, 0.6664143115430061215 ) ) ;
#18752=CARTESIAN_POINT ( 'NONE',  ( 3.427377709871179512, -13.85078959623727002, 3.379007147668904754 ) ) ;
#18753=CARTESIAN_POINT ( 'NONE',  ( 14.94938132205795789, 131.2528086460777388, -1.477614431843955467 ) ) ;
#18754=CARTESIAN_POINT ( 'NONE',  ( -11.40914533023179800, 121.1873859956591843, -1.678693868224012009 ) ) ;
#18756=CARTESIAN_POINT ( 'NONE',  ( 7.869695484959776444, 122.1458944043033057, 0.8493936842156786238 ) ) ;
#18757=CARTESIAN_POINT ( 'NONE',  ( -3.202519050486192231, 34.47767571226007277, 3.235088606727665184 ) ) ;
#18758=CARTESIAN_POINT ( 'NONE',  ( 13.04043193504457498, 133.9378623523624299, -0.05483593244790751359 ) ) ;
#18760=CARTESIAN_POINT ( 'NONE',  ( -2.163474658736635359, 107.1110135075344942, -4.788244450165834998 ) ) ;
#18763=CARTESIAN_POINT ( 'NONE',  ( 4.906163051172606870, 117.7581308566543186, -0.5365533941472381274 ) ) ;
#18766=CARTESIAN_POINT ( 'NONE',  ( 7.630415381941168640, 23.66608445915806058, -3.560124470299026900 ) ) ;
#18767=CARTESIAN_POINT ( 'NONE',  ( -0.007600002268445282295, 120.2037396364829505, 0.3803351912374557386 ) ) ;
#18769=CARTESIAN_POINT ( 'NONE',  ( 11.72569139212691169, 118.7251779360019270, 0.1869994294823658365 ) ) ;
#18770=CARTESIAN_POINT ( 'NONE',  ( -7.475619626241609694, 123.6620266863018855, -0.1149006695610368389 ) ) ;
#18771=DIRECTION ( 'NONE',  ( 0.9998004120163609398, 0.000000000000000000, 0.01997839162482749689 ) ) ;
#18772=CARTESIAN_POINT ( 'NONE',  ( 0.6412933796112577634, 156.3034662015457741, 0.01281456791805622546 ) ) ;
#18774=CARTESIAN_POINT ( 'NONE',  ( 7.865828698536367902, -6.344330755464622662, 3.006797519310529854 ) ) ;
#18775=CARTESIAN_POINT ( 'NONE',  ( -2.140231652025115672, 116.5286393870344028, -0.3979261928235908741 ) ) ;
#18776=CARTESIAN_POINT ( 'NONE',  ( -0.3991458833605321943, 123.7646714092001190, -0.1312610764096185101 ) ) ;
#18779=CARTESIAN_POINT ( 'NONE',  ( 8.411406395146093118, -11.38171290258811119, -0.9481482025471229536 ) ) ;
#18780=CARTESIAN_POINT ( 'NONE',  ( 0.4906649483725750716, 117.9394484190330843, 1.408234383443731641 ) ) ;
#18781=CARTESIAN_POINT ( 'NONE',  ( 3.682264917456193221, 78.83346620154574680, 0.07358041635424013294 ) ) ;
#18783=CARTESIAN_POINT ( 'NONE',  ( 0.4023205627559981457, 108.3383513567250986, -4.340400160729728007 ) ) ;
#18784=CARTESIAN_POINT ( 'NONE',  ( -1.391432384042666337, 159.5643428290674990, 0.4004207282219807706 ) ) ;
#18787=ORIENTED_EDGE ( 'NONE', *, *, #33646, .F. ) ;
#18789=CARTESIAN_POINT ( 'NONE',  ( -15.64525404011971332, 147.2221590072177548, -0.1788206097943383921 ) ) ;
#18790=CARTESIAN_POINT ( 'NONE',  ( 4.016706779461339138, -15.37834506377831723, 5.009826762111060816 ) ) ;
#18791=CARTESIAN_POINT ( 'NONE',  ( -6.779039758441160579, 118.9580315507705706, 0.9776869392460788566 ) ) ;
#18792=CARTESIAN_POINT ( 'NONE',  ( 4.901524533163292396, 117.5843641943970681, -0.6192240155325964279 ) ) ;
#18793=CARTESIAN_POINT ( 'NONE',  ( 3.728136974946417492, 6.765255174955887796, 2.739693761753763113 ) ) ;
#18798=AXIS2_PLACEMENT_3D ( 'NONE', #30361, #24170, #39771 ) ;
#18799=CARTESIAN_POINT ( 'NONE',  ( -4.801770124281918406, 117.3993836135855133, 1.016061139389656587 ) ) ;
#18801=CARTESIAN_POINT ( 'NONE',  ( -6.570524231284120553, 120.8223817900871495, 0.7604033795411313523 ) ) ;
#18802=CARTESIAN_POINT ( 'NONE',  ( 5.149812983838432778, 116.8469558424508534, 0.1790270373415662197 ) ) ;
#18803=CARTESIAN_POINT ( 'NONE',  ( 7.566762702257193496, 120.1328256275108828, -1.061688055624673721 ) ) ;
#18804=CARTESIAN_POINT ( 'NONE',  ( -16.78381336521981382, 153.6818489539412553, -2.151947388239846770 ) ) ;
#18806=ADVANCED_FACE ( 'NONE', ( #15521, #5539 ), #24902, .F. ) ;
#18807=CARTESIAN_POINT ( 'NONE',  ( 11.89914747278627161, 128.3619849303985632, -0.5991027734528262538 ) ) ;
#18810=CARTESIAN_POINT ( 'NONE',  ( -16.72996320514150881, 149.5530097695598215, -2.252745029998447723 ) ) ;
#18811=CARTESIAN_POINT ( 'NONE',  ( 2.686089547800571964, -15.51909802064466248, 4.724564614977055044 ) ) ;
#18812=CARTESIAN_POINT ( 'NONE',  ( -4.110765650185568276, 118.2429491485452928, -0.3474004633102953932 ) ) ;
#18816=CARTESIAN_POINT ( 'NONE',  ( -4.815039658666428579, 117.6402044532089377, 0.9372080113549726699 ) ) ;
#18817=CARTESIAN_POINT ( 'NONE',  ( 8.183297913988958783, 121.2453320564195280, 1.294587653635732138 ) ) ;
#18819=( BOUNDED_CURVE ( )  B_SPLINE_CURVE ( 3, ( #35314, #3151, #31693, #12725 ),
 .UNSPECIFIED., .F., .T. ) 
 B_SPLINE_CURVE_WITH_KNOTS ( ( 4, 4 ),
 ( 0.4854033284062813647, 0.4997054356531658859 ),
 .UNSPECIFIED. ) 
 CURVE ( )  GEOMETRIC_REPRESENTATION_ITEM ( )  RATIONAL_B_SPLINE_CURVE ( ( 0.9433178161976487619, 0.9612738889930489972, 0.9797754291796525461, 0.9988224367574596307 ) ) 
 REPRESENTATION_ITEM ( '' )  );
#18821=CARTESIAN_POINT ( 'NONE',  ( 7.890306666665830804, -2.504341373917490898, 2.985612812370990632 ) ) ;
#18822=CARTESIAN_POINT ( 'NONE',  ( 15.75631923737907947, 146.9135488020124001, 0.6449975968329650922 ) ) ;
#18826=EDGE_CURVE ( 'NONE', #27965, #10570, #10276, .T. ) ;
#18832=EDGE_CURVE ( 'NONE', #26111, #30442, #27275, .T. ) ;
#18835=CARTESIAN_POINT ( 'NONE',  ( -22.97142009758403702, 150.1545470440437953, -0.2295619762022473587 ) ) ;
#18838=CARTESIAN_POINT ( 'NONE',  ( 5.997220096930487188, 121.4340474584781333, 0.01630150470699537335 ) ) ;
#18840=VERTEX_POINT ( 'NONE', #18497 ) ;
#18841=CARTESIAN_POINT ( 'NONE',  ( 0.6554072075965952093, 115.7029491485453718, -1.735615680197917010 ) ) ;
#18842=CARTESIAN_POINT ( 'NONE',  ( -4.578033532675611639, 121.1907927009877000, -0.1597499619731679310 ) ) ;
#18843=CARTESIAN_POINT ( 'NONE',  ( 5.214050246812039546, -13.77884693253300696, 3.484500232556287269 ) ) ;
#18844=CARTESIAN_POINT ( 'NONE',  ( -4.024684254631618607, 117.9114980025989752, 0.7134393008021915339 ) ) ;
#18846=CARTESIAN_POINT ( 'NONE',  ( -0.002459401150369191873, 159.6023738651833810, 0.1230784904792619899 ) ) ;
#18848=CARTESIAN_POINT ( 'NONE',  ( 10.39028434690761671, 153.1476064233308989, 0.3279402672483373582 ) ) ;
#18849=CARTESIAN_POINT ( 'NONE',  ( -0.9676832378731173856, 3.540085264489355676, -0.1409938603398425416 ) ) ;
#18850=CARTESIAN_POINT ( 'NONE',  ( -11.72380150228551976, 118.7251779360019270, -0.2815772452395033931 ) ) ;
#18851=CARTESIAN_POINT ( 'NONE',  ( -6.376221727585796537E-14, 51.14746620154573264, 5.777789833161707559E-29 ) ) ;
#18852=CARTESIAN_POINT ( 'NONE',  ( -5.913343974123855595, 116.9636705795739573, -0.1181626924810776913 ) ) ;
#18854=CARTESIAN_POINT ( 'NONE',  ( 8.718793965502175780, 118.0120498888943246, 0.7790975575022228705 ) ) ;
#18856=CARTESIAN_POINT ( 'NONE',  ( 20.18025034597661715, 150.8812763393641490, 2.199297964380012349 ) ) ;
#18858=CARTESIAN_POINT ( 'NONE',  ( 12.60853345059990538, 122.2722385251898771, -1.300450782769299707 ) ) ;
#18859=CARTESIAN_POINT ( 'NONE',  ( 2.488832714281139946, 5.747567886007050042, -8.044950587805361764 ) ) ;
#18860=CARTESIAN_POINT ( 'NONE',  ( -21.58117366275210003, 150.4657531037631486, -1.865176240683389608 ) ) ;
#18861=CARTESIAN_POINT ( 'NONE',  ( 4.763862057462126209, 117.8479813596402295, -0.8127542836191120612 ) ) ;
#18862=CARTESIAN_POINT ( 'NONE',  ( 6.308735553862782730, 120.0717973201777511, 0.4535485300176086976 ) ) ;
#18864=CARTESIAN_POINT ( 'NONE',  ( -11.86471938700715256, 151.9842433124228762, -0.02191723269355095108 ) ) ;
#18865=CARTESIAN_POINT ( 'NONE',  ( -18.57470247777332872, 148.7425187291823363, -2.467219961595396693 ) ) ;
#18866=CARTESIAN_POINT ( 'NONE',  ( 4.647714231081432779, -15.48178215826023774, 3.998406189266252131 ) ) ;
#18867=DIRECTION ( 'NONE',  ( -0.9998004120163609398, -4.016384292689130894E-17, -0.01997839162482749689 ) ) ;
#18868=CARTESIAN_POINT ( 'NONE',  ( -1.940560682967259032, 118.1651005317671945, -0.8495063313247263048 ) ) ;
#18871=CARTESIAN_POINT ( 'NONE',  ( 10.55536611456372320, 121.9340018749941663, 1.633389464556823878 ) ) ;
#18875=CARTESIAN_POINT ( 'NONE',  ( -5.854232237047567011, 124.7508695889173111, -0.1141955550013106363 ) ) ;
#18876=CARTESIAN_POINT ( 'NONE',  ( -3.806420843250353681, -2.673146571556306750, -7.510622214715559686 ) ) ;
#18877=CARTESIAN_POINT ( 'NONE',  ( 10.75107117262875533, 153.0872561326487187, 1.097343645257591760 ) ) ;
#18878=CARTESIAN_POINT ( 'NONE',  ( 0.009748065369121088064, 159.5507987164374981, -0.4878330526048096361 ) ) ;
#18881=CARTESIAN_POINT ( 'NONE',  ( 5.565051029437463548, 116.7025977693256351, 0.02599261142907015321 ) ) ;
#18883=CARTESIAN_POINT ( 'NONE',  ( -4.468667403750213651, 27.88063884994054220, 0.5133561255362272258 ) ) ;
#18884=CARTESIAN_POINT ( 'NONE',  ( -3.703049682113393359, 116.6240124373522065, -0.07399574541707870656 ) ) ;
#18885=EDGE_CURVE ( 'NONE', #34968, #32786, #18653, .T. ) ;
#18886=EDGE_LOOP ( 'NONE', ( #39556, #2730, #30086, #35546 ) ) ;
#18887=CARTESIAN_POINT ( 'NONE',  ( 4.513834119875788531, 119.5960505434745613, -0.7443551714737827174 ) ) ;
#18888=CARTESIAN_POINT ( 'NONE',  ( 5.304438957985845526, 116.0444662015456885, -1.082911341041116637 ) ) ;
#18889=CARTESIAN_POINT ( 'NONE',  ( -5.891535241408227819, 121.4229528491920576, -0.4202535615248633172 ) ) ;
#18890=CARTESIAN_POINT ( 'NONE',  ( 7.784012320830338005, 122.6313477005580665, 0.1555430910899518460 ) ) ;
#18891=CARTESIAN_POINT ( 'NONE',  ( 15.72148175706224826, 120.8394623874526275, 0.3311059221235125305 ) ) ;
#18893=CARTESIAN_POINT ( 'NONE',  ( -4.151662239014343392, 13.23730288530712862, 2.070234887608822572 ) ) ;
#18895=CARTESIAN_POINT ( 'NONE',  ( -4.999848113220977552, 117.4046874637221833, 0.8305944942939621489 ) ) ;
#18898=CARTESIAN_POINT ( 'NONE',  ( 7.802483560484270164, 122.5107354630703185, 0.4689056730029690367 ) ) ;
#18899=CARTESIAN_POINT ( 'NONE',  ( 4.103230867730633058, 22.16771668783608007, 2.168033597859526651 ) ) ;
#18900=CARTESIAN_POINT ( 'NONE',  ( 12.90531570856114207, 156.9034992427187376, 1.273604633583561796 ) ) ;
#18901=CARTESIAN_POINT ( 'NONE',  ( -4.378631914228641620, 104.6144662015457243, -2.055837668634139970 ) ) ;
#18902=CARTESIAN_POINT ( 'NONE',  ( 1.761579046708144691, 106.7079731062244718, 4.966399410128932601 ) ) ;
#18903=CARTESIAN_POINT ( 'NONE',  ( 15.35657197080316294, 154.8698957928756954, -1.403577372161787906 ) ) ;
#18904=CARTESIAN_POINT ( 'NONE',  ( -11.57150582532061378, 123.3156264706956478, 1.212837404772455274 ) ) ;
#18905=CARTESIAN_POINT ( 'NONE',  ( 1.677595020332960152, 24.74158224480939339, -4.309653081027373211 ) ) ;
#18906=CARTESIAN_POINT ( 'NONE',  ( -22.44014329066014568, 150.2745577238280816, -1.412889903812419412 ) ) ;
#18910=CARTESIAN_POINT ( 'NONE',  ( -15.47786622725302941, 148.0679034673509875, 0.4116497765502036832 ) ) ;
#18911=CARTESIAN_POINT ( 'NONE',  ( 5.472227756958008449, -13.43587746834383445, 2.852490916751204697 ) ) ;
#18912=CARTESIAN_POINT ( 'NONE',  ( 16.58715205660926983, 148.2569838091642964, -1.247478730927799484 ) ) ;
#18914=CARTESIAN_POINT ( 'NONE',  ( -4.663648155852026633, 118.0052748788920383, -0.7714184625502767956 ) ) ;
#18915=CARTESIAN_POINT ( 'NONE',  ( 9.108749339472423046, 153.9337724597031070, 0.1375672075132169658 ) ) ;
#18917=CARTESIAN_POINT ( 'NONE',  ( 6.391991208684993708, 157.5392376370035095, 1.942695856706931679 ) ) ;
#18920=CARTESIAN_POINT ( 'NONE',  ( 5.005702202344075147, 117.4009237673399610, -0.7895530272732956822 ) ) ;
#18921=CARTESIAN_POINT ( 'NONE',  ( 23.22010346901273792, 149.3105122542552863, 0.009921264925044916486 ) ) ;
#18927=CARTESIAN_POINT ( 'NONE',  ( 2.003160442218029136, -15.10791216010797022, 5.854173571448314739 ) ) ;
#18931=CARTESIAN_POINT ( 'NONE',  ( -4.595531677754072675, 118.0173238459723990, 0.6950376821852393139 ) ) ;
#18932=EDGE_LOOP ( 'NONE', ( #4203, #3212, #24913, #35256 ) ) ;
#18934=CARTESIAN_POINT ( 'NONE',  ( -0.3690176902731273079, 115.6909491485452435, -1.766244235947253216 ) ) ;
#18936=CARTESIAN_POINT ( 'NONE',  ( 3.677254471647890099, 118.8081103207223350, -0.7906174721324027432 ) ) ;
#18937=CARTESIAN_POINT ( 'NONE',  ( -5.429077642219940714, 122.7706071131974994, -0.2216225483982831312 ) ) ;
#18938=CARTESIAN_POINT ( 'NONE',  ( 4.721342683323704215, 117.8485734799888291, 1.008627725644892559 ) ) ;
#18940=CARTESIAN_POINT ( 'NONE',  ( 3.220330141560203696, -14.30903721375789317, 2.546581355196453345 ) ) ;
#18941=CARTESIAN_POINT ( 'NONE',  ( 0.01596947694123658501, 156.4635559983122448, -0.7991779281049287142 ) ) ;
#18943=CARTESIAN_POINT ( 'NONE',  ( -0.2371737209061060558, 105.9787871742262979, 5.291462458420934212 ) ) ;
#18944=DIRECTION ( 'NONE',  ( 0.01997839162482749689, 1.040247600000945640E-18, -0.9998004120163610509 ) ) ;
#18945=CARTESIAN_POINT ( 'NONE',  ( 0.8068095026010809745, 106.0274289318137306, -5.250488437364327687 ) ) ;
#18946=CARTESIAN_POINT ( 'NONE',  ( -12.21508602987361058, 126.0625018263836807, -1.612267168929819361 ) ) ;
#18949=CARTESIAN_POINT ( 'NONE',  ( -3.613484950294342024, 115.7029504968768521, 1.483737492548300674 ) ) ;
#18950=CARTESIAN_POINT ( 'NONE',  ( 3.728136974946417492, 6.765255174955887796, 2.739693761753763113 ) ) ;
#18951=CARTESIAN_POINT ( 'NONE',  ( 19.93082032328723940, 128.8226523212408949, 1.025501306202716956 ) ) ;
#18953=CARTESIAN_POINT ( 'NONE',  ( 3.161028851456020750, 105.1241932395464147, -4.308685071247855269 ) ) ;
#18954=CARTESIAN_POINT ( 'NONE',  ( 1.842426711869078471, -15.45708672024491470, 5.391926158250404555 ) ) ;
#18955=CARTESIAN_POINT ( 'NONE',  ( -7.655434399952044444, 119.7866739149480253, 1.082013720931114920 ) ) ;
#18956=CARTESIAN_POINT ( 'NONE',  ( -0.3594991891230457370, 15.46976683256975704, -0.9053751552070300468 ) ) ;
#18957=CARTESIAN_POINT ( 'NONE',  ( 0.6269268744496204748, 0.2942410971610713855, -0.7472855871245592807 ) ) ;
#18958=ORIENTED_EDGE ( 'NONE', *, *, #16719, .T. ) ;
#18960=CARTESIAN_POINT ( 'NONE',  ( -4.882471689226330902, 117.7035670401112952, -0.9281964497351922194 ) ) ;
#18961=CARTESIAN_POINT ( 'NONE',  ( 5.124638537096516622, 121.7269124416356192, 0.3048162158978749425 ) ) ;
#18963=CARTESIAN_POINT ( 'NONE',  ( -8.403980202277468337, 154.6912814427390970, 0.9387012965349954552 ) ) ;
#18964=CARTESIAN_POINT ( 'NONE',  ( -9.118174893680297544, 124.1671967267183589, -0.1822028344259498389 ) ) ;
#18965=CARTESIAN_POINT ( 'NONE',  ( 3.041920762657289057, -14.42862556718194078, 4.364129476586208867 ) ) ;
#18966=CARTESIAN_POINT ( 'NONE',  ( 10.93624696698907961, 154.4230204216147513, -1.584134132468239198 ) ) ;
#18967=CARTESIAN_POINT ( 'NONE',  ( -12.33952200554344536, 155.1253022143813496, -2.231822996700852269 ) ) ;
#18969=CARTESIAN_POINT ( 'NONE',  ( 8.798071512540863282, 117.6842349196870572, 0.1758064070670784795 ) ) ;
#18970=CARTESIAN_POINT ( 'NONE',  ( 4.120272809047287765, 118.2429491485453354, -0.1840329633741082382 ) ) ;
#18971=CARTESIAN_POINT ( 'NONE',  ( 11.92666644034612489, 151.9662372315928280, -0.1848526535252735803 ) ) ;
#18972=ORIENTED_EDGE ( 'NONE', *, *, #29947, .T. ) ;
#18973=CARTESIAN_POINT ( 'NONE',  ( -2.864724612585762387, 107.5205933461715517, -4.491126036370093111 ) ) ;
#18978=B_SPLINE_CURVE_WITH_KNOTS ( 'NONE', 3,
 ( #32778, #9767, #628, #35555 ),
 .UNSPECIFIED., .F., .F.,
 ( 4, 4 ),
 ( 0.000000000000000000, 0.0004289155515219138953 ),
 .UNSPECIFIED. ) ;
#18979=CARTESIAN_POINT ( 'NONE',  ( 4.997973268168866667, 117.5914567208410091, -0.6225120149425793503 ) ) ;
#18980=CARTESIAN_POINT ( 'NONE',  ( 1.217031898716552707, 25.17763362506526192, -8.368877290174015826 ) ) ;
#18981=CARTESIAN_POINT ( 'NONE',  ( 14.47722597845726433, 150.4300676932417389, 1.698653275673423835 ) ) ;
#18982=DIRECTION ( 'NONE',  ( -4.017660918040594346E-17, 1.000000000000000000, 2.376309959284834438E-19 ) ) ;
#18983=CARTESIAN_POINT ( 'NONE',  ( 15.93439728059123794, 121.0320206851898206, 0.2674320648195326333 ) ) ;
#18984=CARTESIAN_POINT ( 'NONE',  ( -5.239677827970801616, 116.1170857923940787, 1.027392938984838633 ) ) ;
#18985=CARTESIAN_POINT ( 'NONE',  ( 0.4343283552818534288, -9.202337043772711667, -4.603842121470758997 ) ) ;
#18987=CARTESIAN_POINT ( 'NONE',  ( 4.023942337083048493, 118.1249481555716301, 0.9214969356372304521 ) ) ;
#18988=CARTESIAN_POINT ( 'NONE',  ( -7.610815090270081740, 30.95102479468643963, -3.615626113024899002 ) ) ;
#18989=CARTESIAN_POINT ( 'NONE',  ( -5.481196946644558921, 117.2620904849268868, -0.8344542377508360476 ) ) ;
#18990=CARTESIAN_POINT ( 'NONE',  ( -0.03413713131426455299, 107.6766875080336376, -4.617405654744151988 ) ) ;
#18991=CARTESIAN_POINT ( 'NONE',  ( 5.586884702347363785, 110.9644662015457328, 0.1116392523995368424 ) ) ;
#18992=CARTESIAN_POINT ( 'NONE',  ( 0.1058213901577000071, 105.9761915687834772, -5.295735085524063024 ) ) ;
#18993=CARTESIAN_POINT ( 'NONE',  ( -0.9950013725589796909, 29.65466048987409309, -4.513790593961638287 ) ) ;
#18994=CARTESIAN_POINT ( 'NONE',  ( 3.354524074468420380, 117.9394488116011814, 1.288362988575229240 ) ) ;
#18995=DIRECTION ( 'NONE',  ( -5.206863593109713661E-17, 1.000000000000000000, -1.077750396879097183E-30 ) ) ;
#18996=CARTESIAN_POINT ( 'NONE',  ( 2.666490510518176649, -13.49855353256042889, 0.05227394649444832425 ) ) ;
#18997=CARTESIAN_POINT ( 'NONE',  ( 0.3848090724907686777, 122.5569158606515003, -0.2475921850528963741 ) ) ;
#18998=CARTESIAN_POINT ( 'NONE',  ( -20.43054131464321443, 152.5480347002736607, 0.4178791510274247334 ) ) ;
#18999=VERTEX_POINT ( 'NONE', #32135 ) ;
#19001=AXIS2_PLACEMENT_3D ( 'NONE', #34018, #4431, #1646 ) ;
#19003=DIRECTION ( 'NONE',  ( 0.9998004120163608288, 0.000000000000000000, 0.01997839162482736852 ) ) ;
#19004=CARTESIAN_POINT ( 'NONE',  ( 4.596189786833723367, -15.64549520875656263, 3.377287787771500849 ) ) ;
#19005=CARTESIAN_POINT ( 'NONE',  ( -4.992797058275008304, 118.5534682650580862, 0.8674252695128578106 ) ) ;
#19006=CARTESIAN_POINT ( 'NONE',  ( 1.320630737124448117, 159.3505072347868747, -0.9467419726141094172 ) ) ;
#19007=CARTESIAN_POINT ( 'NONE',  ( -3.426874451426485724, 1.805113900313119357, -3.130497002818263930 ) ) ;
#19009=ORIENTED_EDGE ( 'NONE', *, *, #14409, .F. ) ;
#19011=CARTESIAN_POINT ( 'NONE',  ( -0.01635612298167265014, 119.2343925067225427, 0.8185272769043292485 ) ) ;
#19012=DIRECTION ( 'NONE',  ( -0.9998004120163609398, 0.000000000000000000, -0.01997839162482749689 ) ) ;
#19013=CARTESIAN_POINT ( 'NONE',  ( -15.09269357795387911, 134.7883251604851580, 1.349233830697068148 ) ) ;
#19014=CARTESIAN_POINT ( 'NONE',  ( 5.143063430802804703, 116.8705556046722620, 0.2506579733502571350 ) ) ;
#19015=CARTESIAN_POINT ( 'NONE',  ( 9.673022701212177665, 121.1143850344477215, -1.180881524473704758 ) ) ;
#19016=CARTESIAN_POINT ( 'NONE',  ( -2.782193507150807932, 158.7847427699215928, -1.504205172470084673 ) ) ;
#19018=CARTESIAN_POINT ( 'NONE',  ( 0.004916276843073956807, 120.6356583033945782, -0.2460305967400716332 ) ) ;
#19020=CARTESIAN_POINT ( 'NONE',  ( 0.02969003158472036108, 157.1787724364823760, -1.485810588193620552 ) ) ;
#19021=CARTESIAN_POINT ( 'NONE',  ( 3.745939827176673731, -15.15858284179406823, -0.4807645327530354340 ) ) ;
#19022=CARTESIAN_POINT ( 'NONE',  ( -4.147540096004632915, 118.2392522295950670, -0.3974202085649201077 ) ) ;
#19026=CARTESIAN_POINT ( 'NONE',  ( -4.765692302950382597, 117.6625622553268471, 0.9423543906840938789 ) ) ;
#19027=CARTESIAN_POINT ( 'NONE',  ( 17.92612601409326345, 146.8415343102147972, 2.296925525151568781 ) ) ;
#19030=CARTESIAN_POINT ( 'NONE',  ( -0.1328416520900886078, 24.48205809745167372, 4.627450821846854190 ) ) ;
#19031=CARTESIAN_POINT ( 'NONE',  ( 11.90976107009709395, 151.9662372315928280, 0.6611612027286484228 ) ) ;
#19035=CARTESIAN_POINT ( 'NONE',  ( -0.02983097934279877947, 117.3993836135855418, 1.492864285909964561 ) ) ;
#19038=CARTESIAN_POINT ( 'NONE',  ( -8.504453550875423318, 119.0083879741271602, -1.280283385220987835 ) ) ;
#19041=EDGE_CURVE ( 'NONE', #38830, #17268, #40938, .T. ) ;
#19042=CARTESIAN_POINT ( 'NONE',  ( -23.07880092997899979, 149.8841935741895384, -0.1310273949726223075 ) ) ;
#19045=CARTESIAN_POINT ( 'NONE',  ( -7.831385197639477269, 122.3498825523410716, -0.6732435565748877693 ) ) ;
#19046=CARTESIAN_POINT ( 'NONE',  ( 4.828460766595028097, 117.4062652275384693, -1.009527310354734642 ) ) ;
#19047=ORIENTED_EDGE ( 'NONE', *, *, #21855, .F. ) ;
#19048=CARTESIAN_POINT ( 'NONE',  ( 0.7744055587462789214, 115.7029695782703982, -1.727565141520491121 ) ) ;
#19049=CARTESIAN_POINT ( 'NONE',  ( -3.737471135337945949, 121.0798372856833538, -0.1416028149587413298 ) ) ;
#19050=CARTESIAN_POINT ( 'NONE',  ( 5.906500239725072987, -12.19293670846725774, 0.5532178544325924152 ) ) ;
#19051=CARTESIAN_POINT ( 'NONE',  ( -9.669117252159470155, 157.4977751962898083, 1.392273965589622575 ) ) ;
#19053=CARTESIAN_POINT ( 'NONE',  ( 13.39999158873808405, 156.9487217736090940, 0.4592210153261411798 ) ) ;
#19054=CARTESIAN_POINT ( 'NONE',  ( 8.677412068956916968, 123.6667082555040480, 0.3039716813630899406 ) ) ;
#19055=CARTESIAN_POINT ( 'NONE',  ( 4.825602063014114762, 118.5266822147775940, -0.7769288410131838241 ) ) ;
#19056=CARTESIAN_POINT ( 'NONE',  ( 0.3789452347801735566, 6.767153838948093636, 0.8990310622920915096 ) ) ;
#19057=CARTESIAN_POINT ( 'NONE',  ( -16.84361796505737630, 155.2300590059875844, -0.4756075834919731293 ) ) ;
#19060=VERTEX_POINT ( 'NONE', #6781 ) ;
#19061=CARTESIAN_POINT ( 'NONE',  ( -5.622202078731264763, 117.6368178314116477, 0.7310929967662477269 ) ) ;
#19063=EDGE_CURVE ( 'NONE', #24401, #21265, #34130, .T. ) ;
#19065=CARTESIAN_POINT ( 'NONE',  ( 5.008743879648425157, 158.5910778905036977, 1.550406713891092414 ) ) ;
#19066=CARTESIAN_POINT ( 'NONE',  ( 19.92238394974707205, 148.9191654756151024, -1.700261758071553775 ) ) ;
#19067=CARTESIAN_POINT ( 'NONE',  ( -2.798479926918381544, 16.31753791307728818, -7.953355231451358698 ) ) ;
#19068=CARTESIAN_POINT ( 'NONE',  ( -6.844670616442416922, 117.9658002137636856, -0.9618333202595320541 ) ) ;
#19069=CARTESIAN_POINT ( 'NONE',  ( 4.745547297112636898, 117.9479177059493082, -0.6406879345116325286 ) ) ;
#19070=CARTESIAN_POINT ( 'NONE',  ( 11.74288454345096788, 118.7273140689154616, 0.2346507796901761422 ) ) ;
#19072=CARTESIAN_POINT ( 'NONE',  ( -7.047330174099129430, 122.0696255612902519, -0.06645725506650262959 ) ) ;
#19073=CARTESIAN_POINT ( 'NONE',  ( -19.20800265940886931, 147.1635184732690220, -2.509201515169785957 ) ) ;
#19075=CARTESIAN_POINT ( 'NONE',  ( 2.394017677299879576, -15.71294128685811486, 5.613897423981592638 ) ) ;
#19076=SHAPE_REPRESENTATION ( 'Center Spindle', ( #3275 ), #21588 ) ;
#19077=DIRECTION ( 'NONE',  ( -5.206863593109713661E-17, 1.000000000000000000, -1.077750396879097183E-30 ) ) ;
#19079=ADVANCED_FACE ( 'NONE', ( #26159 ), #15727, .F. ) ;
#19082=B_SPLINE_SURFACE_WITH_KNOTS ( 'NONE', 3, 3, ( 
 ( #31810, #41409, #25422, #28404, #22610, #13044, #3268, #19222, #12216, #38423, #2438, #25620, #22818, #15606, #32233, #5844, #3064, #41837, #38630, #9643, #22195, #19011, #16227, #9433, #35426, #28611, #6253, #39043, #41620, #6457, #38210, #42040, #22402, #35224 ),
 ( #6049, #12632, #9850, #76, #26034, #32015, #21992, #16021, #35856, #6669, #31601, #15401, #35023, #2854, #15815, #29022, #12836, #25824, #38832, #29449, #503, #16443, #10689, #1123, #20472, #7302, #288, #13475, #32647, #13682, #10897, #6877, #20261, #36063 ),
 ( #23669, #23242, #23032, #13891, #33288, #36276, #19849, #26463, #16655, #17294, #7511, #20058, #4329, #30283, #39255, #36688, #29872, #33499, #14094, #32863, #29662, #39467, #3909, #27093, #3694, #40101, #10062, #3483, #10270, #23886, #7097, #19632, #4118, #33077 ),
 ( #36904, #36481, #39892, #16871, #13261, #26245, #711, #26674, #26883, #39682, #10484, #17078, #23454, #30079, #917, #40932, #18120, #14293, #11316, #11740, #24942, #24727, #11951, #30698, #37730, #21513, #41145, #7722, #21307, #30915, #17496, #37514, #14502, #31125 ),
 ( #5373, #8554, #24304, #34337, #15133, #20687, #27303, #1548, #40318, #27517, #1961, #11111, #17698, #14922, #33712, #24100, #33917, #40525, #37310, #21101, #18328, #5165, #27926, #34548, #8339, #31330, #30493, #2175, #17911, #28137, #4533, #1335, #37108, #7927 ),
 ( #20895, #4746, #8126, #34125, #4952, #1754, #14713, #27717, #40726, #11523, #24507, #41361, #34970, #25774, #38371, #9386, #9186, #41987, #15971, #22142, #22562, #35173, #3013, #28969, #41572, #12164, #32180, #22350, #12381, #25158, #18749, #5792, #35592, #38782 ),
 ( #5582, #6203, #28771, #38159, #19174, #16177, #31758, #18961, #29180, #6409, #9592, #8974, #31543, #31968, #19379, #32384, #3215, #27, #12785, #2389, #18540, #41782, #12991, #37941, #12581, #8766, #2600, #21726, #34750, #15347, #5999, #28352, #21941, #15560 ),
 ( #35374, #28563, #2806, #25367, #25570, #15767, #38575, #39202, #13423, #10642, #33028, #10011, #7044, #7255, #16608, #17029, #22983, #26621, #35803, #36010, #20215, #6824, #39630, #23622, #30028, #29616, #10435, #33450, #17241, #3428, #19793, #32594, #32813, #36436 ),
 ( #13631, #30236, #20011, #36642, #452, #26411, #38994, #16822, #39846, #39416, #10218, #1075, #9803, #4279, #20423, #3644, #13841, #23188, #36223, #13215, #16393, #662, #29399, #26197, #4070, #33241, #3857, #23406, #868, #6616, #25986, #29824, #7464, #22770 ),
 ( #19584, #26839, #238, #41041, #11851, #18222, #20633, #28032, #35080, #36856, #21620, #40056, #17446, #11634, #2497, #15032, #28248, #24837, #18652, #34861, #37832, #41467, #8659, #21833, #5693, #31223, #30445, #8870, #41252, #2067, #1289, #37627, #24619, #12275 ),
 ( #31658, #23835, #25047, #5474, #14247, #38051, #5901, #8451, #34646, #18862, #25265, #15460, #27254, #7674, #18434, #28461, #38268, #9085, #22051, #31866, #33661, #4486, #31441, #14044, #27048, #2284, #10849, #21409, #40270, #34436, #5271, #15247, #12058, #25482 ),
 ( #29516, #38477, #9296, #35920, #13109, #22257, #6311, #6730, #19914, #19697, #6946, #25683, #32716, #16509, #36129, #2706, #16296, #25887, #12487, #32500, #9495, #26101, #42105, #39107, #41894, #19491, #19284, #41679, #35706, #6516, #32291, #3120, #28669, #9911 ) ),
 .UNSPECIFIED., .F., .F., .F.,
 ( 4, 1, 1, 1, 1, 1, 3, 4 ),
 ( 4, 1, 1, 1, 1, 1, 1, 1, 1, 1, 1, 1, 1, 1, 1, 1, 1, 1, 1, 2, 1, 1, 1, 1, 1, 1, 1, 1, 1, 1, 4 ),
 ( 0.000000000000000000, 0.1666666666666666574, 0.2500000000000000000, 0.5000000000000000000, 0.5555555555555555802, 0.7500000000000000000, 1.000000000000000000, 1.010000000000000009 ),
 ( 0.000000000000000000, 0.02126250000000000015, 0.04252500000000000030, 0.06378749999999999698, 0.08505000000000000060, 0.1063125000000000042, 0.1275749999999999940, 0.1488374999999999837, 0.1701000000000000012, 0.1913624999999999909, 0.2126250000000000084, 0.2338874999999999704, 0.2551500000000000434, 0.2764124999999999499, 0.2870437499999999864, 0.2976749999999999674, 0.3083062500000000039, 0.3189375000000000404, 0.3295687499999999659, 0.3402000000000000024, 0.4226750000000000229, 0.5051499999999999879, 0.5876249999999998419, 0.6700999999999999179, 0.7525749999999999940, 0.7938125000000000320, 0.8350499999999999590, 0.8762874999999994419, 0.9175249999999994799, 0.9587624999999999620, 1.000000000000000000 ),
 .UNSPECIFIED. ) ;
#19083=CARTESIAN_POINT ( 'NONE',  ( 10.15136974315531049, 155.5514087735115822, 2.139549497352468244 ) ) ;
#19087=CARTESIAN_POINT ( 'NONE',  ( -2.121281617407082987, 114.8832439220486350, 1.889083087725355048 ) ) ;
#19088=CARTESIAN_POINT ( 'NONE',  ( -7.610815090270081740, 30.95102479468643963, -3.615626113024899002 ) ) ;
#19089=CARTESIAN_POINT ( 'NONE',  ( 15.52857178871868093, 148.0963874134046705, 1.155438959258077380 ) ) ;
#19090=CARTESIAN_POINT ( 'NONE',  ( 17.93297959639523143, 125.1504969321615164, -0.5028613125471299572 ) ) ;
#19093=CARTESIAN_POINT ( 'NONE',  ( -22.98549031890228989, 150.1594536303649932, -0.4336790679505425072 ) ) ;
#19095=CARTESIAN_POINT ( 'NONE',  ( -6.324598044711755129, 120.0162699490936120, -1.207732045962844669 ) ) ;
#19097=CARTESIAN_POINT ( 'NONE',  ( -6.479751845157381673, 121.6679077367135591, -0.4493306481243477535 ) ) ;
#19099=CIRCLE ( 'NONE', #3475, 0.5080000000000002292 ) ;
#19100=CARTESIAN_POINT ( 'NONE',  ( 15.19604463793433169, 156.0859089222169587, 0.3036531364422415669 ) ) ;
#19102=CARTESIAN_POINT ( 'NONE',  ( -3.234384296441582762, 11.31316835407710819, -3.315160845070126427 ) ) ;
#19104=CARTESIAN_POINT ( 'NONE',  ( -4.976922239355512367, 117.4076159968771833, 0.8840036975013897402 ) ) ;
#19105=CARTESIAN_POINT ( 'NONE',  ( 0.9670297670242945509, 105.9617104547169788, 5.250135314356312755 ) ) ;
#19106=ADVANCED_FACE ( 'NONE', ( #16350 ), #22727, .T. ) ;
#19108=CARTESIAN_POINT ( 'NONE',  ( -7.959258266637833756, 121.8607301277289565, 0.7063002939533309377 ) ) ;
#19109=CARTESIAN_POINT ( 'NONE',  ( 4.309711357183296343, 3.151582320728117725, 1.677628897243969464 ) ) ;
#19111=CARTESIAN_POINT ( 'NONE',  ( 22.50377699857059000, 149.0203452686010337, 1.755643737887156997 ) ) ;
#19112=DIRECTION ( 'NONE',  ( -0.9998004120163609398, -4.016384292689130894E-17, -0.01997839162482749689 ) ) ;
#19114=CARTESIAN_POINT ( 'NONE',  ( 2.188165212810265103, 117.9909145081919917, -0.6446704472730118152 ) ) ;
#19116=CARTESIAN_POINT ( 'NONE',  ( 4.428293322310913993, 12.87204911218450576, 1.319288874004734158 ) ) ;
#19117=CARTESIAN_POINT ( 'NONE',  ( -15.29070941918909199, 121.1074504348956964, -0.9956366180447245862 ) ) ;
#19119=CARTESIAN_POINT ( 'NONE',  ( -15.52187087609533478, 147.8629129908177049, 0.2796426011346636042 ) ) ;
#19121=CARTESIAN_POINT ( 'NONE',  ( 4.196136289373067818, -14.93657984310306475, 5.004071965215434403 ) ) ;
#19124=CARTESIAN_POINT ( 'NONE',  ( -4.604761013128439551, 118.0233142930135557, -0.8446000906974990841 ) ) ;
#19125=CARTESIAN_POINT ( 'NONE',  ( 1.617373050801646839, 120.9968702744464366, 0.03231896268895514263 ) ) ;
#19127=CARTESIAN_POINT ( 'NONE',  ( 19.78444808418223033, 147.9128418260961837, 2.517891032746079283 ) ) ;
#19129=CARTESIAN_POINT ( 'NONE',  ( 10.18105065676961729, 125.9743313966586129, 0.2034416216762106322 ) ) ;
#19130=EDGE_CURVE ( 'NONE', #26452, #19060, #32758, .T. ) ;
#19132=CARTESIAN_POINT ( 'NONE',  ( -15.10519797802286845, 121.1899582252741112, 0.5359826722732081716 ) ) ;
#19133=B_SPLINE_CURVE_WITH_KNOTS ( 'NONE', 3,
 ( #31003, #28020, #11838, #8021 ),
 .UNSPECIFIED., .F., .F.,
 ( 4, 4 ),
 ( 0.000000000000000000, 1.000000000000000000 ),
 .UNSPECIFIED. ) ;
#19134=CARTESIAN_POINT ( 'NONE',  ( 4.853781638280933564, 117.4081357529187528, -0.9972794204146671060 ) ) ;
#19135=CARTESIAN_POINT ( 'NONE',  ( 22.92015980622311844, 150.1344166263168347, 0.006220127847215254323 ) ) ;
#19143=CARTESIAN_POINT ( 'NONE',  ( -4.606047465314773603, 118.0409777277905334, 0.6500082233937537479 ) ) ;
#19147=CARTESIAN_POINT ( 'NONE',  ( 5.979754242620736626, 119.1689217970666732, -1.027035715780954428 ) ) ;
#19148=CARTESIAN_POINT ( 'NONE',  ( -1.370820134808223623, 106.2483430537416638, -5.168860673143087503 ) ) ;
#19149=CARTESIAN_POINT ( 'NONE',  ( 4.710630312300388312, 117.8980792669073310, 0.9560384519295030969 ) ) ;
#19151=CARTESIAN_POINT ( 'NONE',  ( 2.671714809844681238, -14.97371442308345380, 4.574436322856921144 ) ) ;
#19152=CARTESIAN_POINT ( 'NONE',  ( -9.472608709197698929, 123.5188755717998816, -0.9573233835003830405 ) ) ;
#19153=CARTESIAN_POINT ( 'NONE',  ( -3.782657323308230790, 115.7032134869121052, -1.604837383391216177 ) ) ;
#19154=CARTESIAN_POINT ( 'NONE',  ( -2.307087371449152435, 107.0582400219110468, 4.722921399226381212 ) ) ;
#19156=CARTESIAN_POINT ( 'NONE',  ( 6.697645968159008589, 121.2318545172250737, -0.07433936815196268144 ) ) ;
#19157=CARTESIAN_POINT ( 'NONE',  ( 0.008945177887895646232, 119.9096241394016715, -0.4476532798976758376 ) ) ;
#19159=CARTESIAN_POINT ( 'NONE',  ( 0.4584169952490399491, 38.71425902074634706, 1.375259010134687765 ) ) ;
#19160=CARTESIAN_POINT ( 'NONE',  ( -3.014526234809750793, 115.7029722856716631, 1.552890539658475566 ) ) ;
#19161=CARTESIAN_POINT ( 'NONE',  ( 2.862861873098513144, -10.07698056833738143, -3.640125809621839625 ) ) ;
#19162=CARTESIAN_POINT ( 'NONE',  ( 1.362313394648025699, 159.5452856091935132, 0.5382632954014164861 ) ) ;
#19164=CARTESIAN_POINT ( 'NONE',  ( -0.7308287095922618715, 104.6144662015455964, -4.780214960664815216 ) ) ;
#19165=CARTESIAN_POINT ( 'NONE',  ( 3.526206095277399033, -15.04645431008844270, 1.792912095860496269 ) ) ;
#19166=CARTESIAN_POINT ( 'NONE',  ( -11.12579521122948734, 121.4866960210745503, 1.254162869557706284 ) ) ;
#19167=AXIS2_PLACEMENT_3D ( 'NONE', #11920, #8943, #5764 ) ;
#19168=CARTESIAN_POINT ( 'NONE',  ( -0.9635192623308774795, 7.475506455475952272, -0.1398073520734665620 ) ) ;
#19170=CARTESIAN_POINT ( 'NONE',  ( 0.9727671068909850005, -1.206248505109467795, 0.1081409728948927729 ) ) ;
#19174=CARTESIAN_POINT ( 'NONE',  ( 5.572611807913179227, 123.3023672762779910, 0.1864456790743030112 ) ) ;
#19176=CARTESIAN_POINT ( 'NONE',  ( -14.98735845036259917, 139.3652335140928074, 0.8263902896301494883 ) ) ;
#19178=CARTESIAN_POINT ( 'NONE',  ( 3.826441825042426359, -13.78667705120290066, 4.058770776067232688 ) ) ;
#19179=CARTESIAN_POINT ( 'NONE',  ( 11.33340168069282861, 123.5700555580090594, -1.145074488444943306 ) ) ;
#19180=CARTESIAN_POINT ( 'NONE',  ( 0.01147819631900381596, 118.5605975114896609, -0.5744158801423951966 ) ) ;
#19182=EDGE_CURVE ( 'NONE', #27127, #25568, #38858, .T. ) ;
#19183=CARTESIAN_POINT ( 'NONE',  ( 8.133233755128500775, 120.8101225051349701, 1.375441441843951340 ) ) ;
#19184=CARTESIAN_POINT ( 'NONE',  ( -5.848753628616515599, 31.48281334387809238, 0.7289013152532436424 ) ) ;
#19185=CARTESIAN_POINT ( 'NONE',  ( 0.6667004703451558933, 156.3175253132196190, -0.2457982560305634334 ) ) ;
#19190=CARTESIAN_POINT ( 'NONE',  ( 9.696059495791431004, 123.7664141286412871, 0.9760873372638446677 ) ) ;
#19192=CARTESIAN_POINT ( 'NONE',  ( 23.35954322469556033, 148.8716009884483071, 0.3896314068422420118 ) ) ;
#19193=CARTESIAN_POINT ( 'NONE',  ( -6.697645968159137375, 121.2318545172250737, 0.07433936815196282022 ) ) ;
#19195=FACE_OUTER_BOUND ( 'NONE', #35715, .T. ) ;
#19197=CARTESIAN_POINT ( 'NONE',  ( -3.999880774356848523, 33.21692059697370070, 1.336717509662867398 ) ) ;
#19198=CARTESIAN_POINT ( 'NONE',  ( 5.843718602766560188, 118.4234969239897453, 1.100938688348692240 ) ) ;
#19199=CARTESIAN_POINT ( 'NONE',  ( -6.116428202004375869, -11.74185255526443505, -5.788024375304219760 ) ) ;
#19200=CARTESIAN_POINT ( 'NONE',  ( 2.183490310512786525, 116.7443332818461670, -0.4098265381987980516 ) ) ;
#19201=CARTESIAN_POINT ( 'NONE',  ( 0.03040743767353545901, 116.4813942609868178, -1.521712522323299677 ) ) ;
#19203=CARTESIAN_POINT ( 'NONE',  ( 4.337287324166744895, 111.8944019378196515, -2.742125067219324919 ) ) ;
#19204=CARTESIAN_POINT ( 'NONE',  ( 0.1093955723348968428, 105.1224543976622243, 5.344227820326648448 ) ) ;
#19205=CARTESIAN_POINT ( 'NONE',  ( -4.544942180623752215, 12.81246518813932589, 0.8472608254572608910 ) ) ;
#19208=CARTESIAN_POINT ( 'NONE',  ( 3.187349844189338199, -14.38168857376666310, 3.261415970826748278 ) ) ;
#19209=CARTESIAN_POINT ( 'NONE',  ( 2.271240278323836126, 124.1308405194309188, -0.008591128553798579870 ) ) ;
#19210=CARTESIAN_POINT ( 'NONE',  ( -13.22272649419669932, 119.7880570645780978, 0.3832108753485274355 ) ) ;
#19213=ORIENTED_EDGE ( 'NONE', *, *, #16135, .F. ) ;
#19215=CARTESIAN_POINT ( 'NONE',  ( 3.555926573287145231, -15.62149673449747489, 5.135790484437000814 ) ) ;
#19216=CARTESIAN_POINT ( 'NONE',  ( -20.34707623724171199, 149.4216517587604756, 1.615871423115795347 ) ) ;
#19217=CARTESIAN_POINT ( 'NONE',  ( 0.01887972822138636597, 159.3676309965788960, -0.9448188026860500077 ) ) ;
#19218=CARTESIAN_POINT ( 'NONE',  ( 4.634220987317881679, -1.855718946426311078, -0.01876340930339078644 ) ) ;
#19220=ORIENTED_EDGE ( 'NONE', *, *, #21380, .T. ) ;
#19222=CARTESIAN_POINT ( 'NONE',  ( -0.003708075274190775900, 123.1683257372384901, 0.1855672496570263952 ) ) ;
#19223=DIRECTION ( 'NONE',  ( 0.000000000000000000, 0.000000000000000000, 1.000000000000000000 ) ) ;
#19224=CARTESIAN_POINT ( 'NONE',  ( -17.12300761254207870, 147.7912591418244403, 1.363423146152764165 ) ) ;
#19225=DIRECTION ( 'NONE',  ( 0.9998004120163608288, 0.000000000000000000, 0.01997839162482749342 ) ) ;
#19226=CARTESIAN_POINT ( 'NONE',  ( 2.416701088390823760, 119.2205458019918751, -0.6800916218662635959 ) ) ;
#19227=CARTESIAN_POINT ( 'NONE',  ( -13.26090510203115969, 121.6721647909590303, -1.681263517196597723 ) ) ;
#19229=AXIS2_PLACEMENT_3D ( 'NONE', #40915, #8536, #21496 ) ;
#19230=ORIENTED_EDGE ( 'NONE', *, *, #14365, .F. ) ;
#19231=CARTESIAN_POINT ( 'NONE',  ( 4.473451502231345245, 118.1283369050730130, -0.5456401070386401875 ) ) ;
#19232=CARTESIAN_POINT ( 'NONE',  ( 14.68012063964721214, 139.2174805014774392, -0.5696158742132092501 ) ) ;
#19234=CARTESIAN_POINT ( 'NONE',  ( -0.8355136867052901373, 157.0053619834820324, -1.416332280276762834 ) ) ;
#19235=CARTESIAN_POINT ( 'NONE',  ( 3.526206095277399033, -15.04645431008844270, 1.792912095860496269 ) ) ;
#19236=CARTESIAN_POINT ( 'NONE',  ( -4.065972646788793554, 118.2429491485452928, -0.3080848862740693250 ) ) ;
#19240=CARTESIAN_POINT ( 'NONE',  ( -4.888505472423630316, 117.6743111526193388, 0.8475594030621235175 ) ) ;
#19241=CARTESIAN_POINT ( 'NONE',  ( 12.49704818634931414, 126.0212559692275249, 1.705261654849119068 ) ) ;
#19243=CARTESIAN_POINT ( 'NONE',  ( -4.563195415240126174, 21.88328375387019165, -0.7336086519975816289 ) ) ;
#19244=CARTESIAN_POINT ( 'NONE',  ( 3.706155879761894756, 121.0264708767875561, 0.2234555574396433764 ) ) ;
#19247=CARTESIAN_POINT ( 'NONE',  ( -6.573280687130626123E-14, 88.99346620154574339, 1.699031322814114629E-29 ) ) ;
#19255=CARTESIAN_POINT ( 'NONE',  ( -1.860994725976048425, 116.5907236856068181, 0.1449800026146565723 ) ) ;
#19256=B_SPLINE_CURVE_WITH_KNOTS ( 'NONE', 3,
 ( #29102, #36148, #6533, #35509 ),
 .UNSPECIFIED., .F., .F.,
 ( 4, 4 ),
 ( 0.5009815572441199683, 1.000000000000000000 ),
 .UNSPECIFIED. ) ;
#19259=CARTESIAN_POINT ( 'NONE',  ( 7.840780172454366870, 122.3995516869274383, -0.3066307168558741747 ) ) ;
#19261=CARTESIAN_POINT ( 'NONE',  ( 1.330693927565623991, 115.7029491485453576, -1.688181875448171665 ) ) ;
#19262=CARTESIAN_POINT ( 'NONE',  ( -14.19780223135882835, 138.9094276006951247, -0.4095818057664819545 ) ) ;
#19263=CARTESIAN_POINT ( 'NONE',  ( 6.287662417442902552, -13.15673151805442309, 0.9153646538742283845 ) ) ;
#19264=CARTESIAN_POINT ( 'NONE',  ( -3.087569247026613617, 117.8293475852256904, 0.6612947004247919924 ) ) ;
#19267=CARTESIAN_POINT ( 'NONE',  ( 5.799544261406283319, 116.9771394561422539, 0.2896453145609861890 ) ) ;
#19268=CARTESIAN_POINT ( 'NONE',  ( 11.75192402136879366, 130.2587789749062210, 0.3484658256491862116 ) ) ;
#19269=CARTESIAN_POINT ( 'NONE',  ( 4.855010706775262364, 115.6909491485453145, -1.281361498472391336 ) ) ;
#19270=CARTESIAN_POINT ( 'NONE',  ( 0.4504873307288463358, 16.48674109716143477, 0.8651787211232140340 ) ) ;
#19271=CARTESIAN_POINT ( 'NONE',  ( -20.36427691206304402, 129.0035756037533758, -0.5974333909176803292 ) ) ;
#19274=EDGE_LOOP ( 'NONE', ( #32381, #1019 ) ) ;
#19275=CARTESIAN_POINT ( 'NONE',  ( -5.594955721643887436, 117.4948600716806908, 0.6777700223702270987 ) ) ;
#19278=CARTESIAN_POINT ( 'NONE',  ( 19.06843068773014238, 131.8899703912256314, 2.039348754248471174 ) ) ;
#19279=CARTESIAN_POINT ( 'NONE',  ( 11.46709954559036859, 121.1873859956591843, -1.221572053168039185 ) ) ;
#19280=CARTESIAN_POINT ( 'NONE',  ( 3.006797519324799772, 15.24566924451032435, -7.865828698519952589 ) ) ;
#19281=CARTESIAN_POINT ( 'NONE',  ( -1.253347288035753460, 159.2526592949493534, -1.130111582746273768 ) ) ;
#19282=CARTESIAN_POINT ( 'NONE',  ( 4.739872878304939974, 117.9513957112883276, -0.6506048652930741527 ) ) ;
#19283=EDGE_CURVE ( 'NONE', #11900, #2737, #34438, .T. ) ;
#19284=CARTESIAN_POINT ( 'NONE',  ( 3.430439322123106649, 108.6576027043044377, 4.130303871225995849 ) ) ;
#19285=EDGE_CURVE ( 'NONE', #39868, #15268, #10393, .T. ) ;
#19286=CARTESIAN_POINT ( 'NONE',  ( -15.72781737677524738, 145.6903699455376113, -0.2627434299976844634 ) ) ;
#19287=CARTESIAN_POINT ( 'NONE',  ( -19.09005709338569545, 148.2829752965438956, -2.500029303593213292 ) ) ;
#19288=CARTESIAN_POINT ( 'NONE',  ( 5.933841582263978509, -14.80544765534526341, -0.2634432552157287555 ) ) ;
#19293=CARTESIAN_POINT ( 'NONE',  ( 18.29412156995171301, 148.6295804641074483, 2.431306780064794726 ) ) ;
#19294=CARTESIAN_POINT ( 'NONE',  ( -15.38000172824470368, 147.8312228276848543, -0.3073290369001835387 ) ) ;
#19295=CARTESIAN_POINT ( 'NONE',  ( -5.433597316833275848, 122.7706071131974994, 0.004560450986766876290 ) ) ;
#19296=CARTESIAN_POINT ( 'NONE',  ( -5.416678580886389760, 20.69493382693234196, -6.515560366292809213 ) ) ;
#19297=CARTESIAN_POINT ( 'NONE',  ( 14.64564643111550879, 139.2174805014774392, 1.155614491733866211 ) ) ;
#19298=CARTESIAN_POINT ( 'NONE',  ( 19.54046365593621815, 128.7319734376252143, -0.5398260955622251611 ) ) ;
#19303=CARTESIAN_POINT ( 'NONE',  ( -13.43845804798116106, 156.9141898299356512, -0.2685323735513600041 ) ) ;
#19305=CARTESIAN_POINT ( 'NONE',  ( 6.326077193401762777, 119.9160889050335186, -0.9682899027979984252 ) ) ;
#19306=CARTESIAN_POINT ( 'NONE',  ( 6.088215427201158825, -14.09263546912463028, 1.889225179162022927 ) ) ;
#19307=VECTOR ( 'NONE', #132, 999.9999999999998863 ) ;
#19308=CARTESIAN_POINT ( 'NONE',  ( -15.71402047398562019, 147.5983985311728759, -1.037567014598419490 ) ) ;
#19309=CARTESIAN_POINT ( 'NONE',  ( 1.960603841440088146, -15.05276691075377293, 5.730201639535507319 ) ) ;
#19311=CARTESIAN_POINT ( 'NONE',  ( 15.54780490071025056, 120.7212560704218589, 0.3275748350740995130 ) ) ;
#19313=CARTESIAN_POINT ( 'NONE',  ( 2.267534764145236803, 6.115564135048844108, 4.037922524061999141 ) ) ;
#19314=CARTESIAN_POINT ( 'NONE',  ( -14.91134437181082717, 120.3281135998953459, -0.2979641475761142244 ) ) ;
#19315=CARTESIAN_POINT ( 'NONE',  ( -4.854889821517595294, 117.4070850134769728, 0.9981808394738391765 ) ) ;
#19318=CARTESIAN_POINT ( 'NONE',  ( -7.851952014490078291, 122.3505504179107390, 0.3628578151170098742 ) ) ;
#19320=CARTESIAN_POINT ( 'NONE',  ( -4.623654898565560778, 8.549082320728111029, 0.09932813335659773646 ) ) ;
#19321=CARTESIAN_POINT ( 'NONE',  ( 3.104962560943341554, 159.3365417412370562, 0.8543937160244111650 ) ) ;
#19322=CARTESIAN_POINT ( 'NONE',  ( 15.64207015331054862, 147.2204672151589193, 0.3125657877211908686 ) ) ;
#19324=CARTESIAN_POINT ( 'NONE',  ( 5.883034912960730445, 118.4234969239897453, -0.8666102449821462272 ) ) ;
#19325=CARTESIAN_POINT ( 'NONE',  ( 3.900846188197024667, 12.44727460162280863, 2.488979119290085862 ) ) ;
#19326=CARTESIAN_POINT ( 'NONE',  ( -15.06876432237292995, 120.9194639129320734, -0.9861043747356995626 ) ) ;
#19328=CARTESIAN_POINT ( 'NONE',  ( -4.537977675602711258, 121.1059516323014549, 0.1178196913276178259 ) ) ;
#19329=CARTESIAN_POINT ( 'NONE',  ( 2.850627862023833892, -15.32561772411503220, 5.765353718581858189 ) ) ;
#19332=ORIENTED_EDGE ( 'NONE', *, *, #25820, .F. ) ;
#19333=CARTESIAN_POINT ( 'NONE',  ( 10.99314024304344883, 156.0189320485970086, 2.156370349642059203 ) ) ;
#19336=CARTESIAN_POINT ( 'NONE',  ( -1.363555988950395870, 159.4956652290339605, 0.6451735917158238909 ) ) ;
#19337=CARTESIAN_POINT ( 'NONE',  ( 4.931598085382976393, 117.4109156735239452, -0.9380226465277491377 ) ) ;
#19338=CARTESIAN_POINT ( 'NONE',  ( 9.739177221546302832, 118.0756159837034716, -0.1634508798788866235 ) ) ;
#19343=FACE_OUTER_BOUND ( 'NONE', #25628, .T. ) ;
#19347=CARTESIAN_POINT ( 'NONE',  ( -4.587462187188385165, 118.0383919587454642, 0.6669115617459517864 ) ) ;
#19353=CARTESIAN_POINT ( 'NONE',  ( 8.406963674677495391, 119.7153034306578974, -1.094654629815129177 ) ) ;
#19354=CARTESIAN_POINT ( 'NONE',  ( -5.433204070470928571, 117.5340897209903517, -0.8253704096831885328 ) ) ;
#19355=CARTESIAN_POINT ( 'NONE',  ( 4.767144615469286251, 117.8468057660086430, 0.9623966903202456624 ) ) ;
#19357=CARTESIAN_POINT ( 'NONE',  ( -9.932629385191992455, 123.7598584631124794, -1.097969866555963403 ) ) ;
#19358=CARTESIAN_POINT ( 'NONE',  ( -3.014963585057483630, 115.7029491485453576, -1.667984629301600075 ) ) ;
#19359=EDGE_CURVE ( 'NONE', #20685, #38830, #4192, .T. ) ;
#19362=CARTESIAN_POINT ( 'NONE',  ( 7.669306984062364663, 124.7206709383052043, 0.1533317827557520718 ) ) ;
#19363=CARTESIAN_POINT ( 'NONE',  ( -16.94372847238233248, 146.2370505443881257, -1.929411111270964652 ) ) ;
#19364=CARTESIAN_POINT ( 'NONE',  ( -0.0002734175339917587714, 159.6054662015457382, 0.01368293144939993107 ) ) ;
#19365=CARTESIAN_POINT ( 'NONE',  ( -3.646844371775973315, 115.7029492783617854, 1.479374498987925168 ) ) ;
#19366=CARTESIAN_POINT ( 'NONE',  ( 1.961646697876492373, -0.1315482170498871728, -4.191205975169975950 ) ) ;
#19367=CARTESIAN_POINT ( 'NONE',  ( 16.63860074592936300, 155.2617138006751532, 0.9902706816744292206 ) ) ;
#19370=CARTESIAN_POINT ( 'NONE',  ( 3.057239904206551895, -15.51127639645041789, 4.278020201805971645 ) ) ;
#19371=CARTESIAN_POINT ( 'NONE',  ( -19.17469122182637875, 148.2829752965438956, 1.735408567215429576 ) ) ;
#19372=CARTESIAN_POINT ( 'NONE',  ( -0.01718310852247704676, 5.323846764136113130, -0.9747645957998940514 ) ) ;
#19373=CARTESIAN_POINT ( 'NONE',  ( -21.37844900359480960, 132.5159896776619917, -0.8378797052005129142 ) ) ;
#19374=CARTESIAN_POINT ( 'NONE',  ( -0.5978751570792395498, 11.96162690172616294, -0.7744233872902203109 ) ) ;
#19378=EDGE_CURVE ( 'NONE', #3203, #21896, #5544, .T. ) ;
#19379=CARTESIAN_POINT ( 'NONE',  ( 4.183818394377241567, 118.4033805524614849, 0.7412457532797814830 ) ) ;
#19382=CARTESIAN_POINT ( 'NONE',  ( -6.515494676152068010, 155.4519854478747902, 0.9200225795255462247 ) ) ;
#19383=CARTESIAN_POINT ( 'NONE',  ( 3.354142537596241702, -14.24820561377959649, 4.738596845331590757 ) ) ;
#19384=CARTESIAN_POINT ( 'NONE',  ( 17.98452544307424006, 146.6345634702618952, -1.580200905155534574 ) ) ;
#19385=CARTESIAN_POINT ( 'NONE',  ( -2.522816026436837333, 158.1729697732556588, -1.709197703933636125 ) ) ;
#19387=CARTESIAN_POINT ( 'NONE',  ( 8.682895647160147945, 118.1675475142423437, 0.9202857585879714586 ) ) ;
#19388=CARTESIAN_POINT ( 'NONE',  ( -0.08015702708839873847, 38.63184331614436218, 0.5155861021556068513 ) ) ;
#19389=CARTESIAN_POINT ( 'NONE',  ( 15.81463230642810025, 145.9351319680867221, -0.01551611691150889434 ) ) ;
#19396=CARTESIAN_POINT ( 'NONE',  ( -0.01596947694136538129, 156.4635559983122448, 0.7991779281049289363 ) ) ;
#19397=DIRECTION ( 'NONE',  ( -0.9998004120163609398, 0.000000000000000000, -0.01997839162482749689 ) ) ;
#19398=CARTESIAN_POINT ( 'NONE',  ( 4.735783051744282268, 116.7698466342620378, 0.01422048256815234418 ) ) ;
#19399=CARTESIAN_POINT ( 'NONE',  ( -2.686051902181577855, 107.2142675576569530, 4.629644704627760454 ) ) ;
#19400=FACE_OUTER_BOUND ( 'NONE', #36599, .T. ) ;
#19401=CARTESIAN_POINT ( 'NONE',  ( 4.611808778022512989, -11.57686662695173929, 0.3579861242195471194 ) ) ;
#19402=CARTESIAN_POINT ( 'NONE',  ( -3.469629447173708137, 31.73985764285065869, 0.6454790148241180692 ) ) ;
#19403=CARTESIAN_POINT ( 'NONE',  ( 20.60480707444001069, 141.5323519391372997, 2.354057365763566168 ) ) ;
#19404=VECTOR ( 'NONE', #25554, 1000.000000000000114 ) ;
#19405=CARTESIAN_POINT ( 'NONE',  ( -3.182929088426432074, 26.46582164074821009, -3.363547984189534379 ) ) ;
#19406=CARTESIAN_POINT ( 'NONE',  ( 3.771486885279011325, -13.69470344665998773, -7.544622693077620568 ) ) ;
#19407=CARTESIAN_POINT ( 'NONE',  ( 8.741995348237278307, 118.0171073936068069, -0.4338951289030384406 ) ) ;
#19408=CARTESIAN_POINT ( 'NONE',  ( 0.06390210066009133216, 106.1446358501009826, -5.228158908302722452 ) ) ;
#19409=CARTESIAN_POINT ( 'NONE',  ( -5.152689475313444234, 116.8412042432202185, -0.1029630068797482562 ) ) ;
#19410=CARTESIAN_POINT ( 'NONE',  ( 0.4328132676559295899, 105.9956125065441199, -5.278019706336061212 ) ) ;
#19411=CARTESIAN_POINT ( 'NONE',  ( -2.419178179742970336, 105.1243363418205234, 4.754978004784589096 ) ) ;
#19412=CARTESIAN_POINT ( 'NONE',  ( 4.377640660406503237, 26.40621510375495973, 1.544744264128281364 ) ) ;
#19413=EDGE_CURVE ( 'NONE', #2737, #6467, #28314, .T. ) ;
#19416=CARTESIAN_POINT ( 'NONE',  ( 2.769760999665409340, -14.92388480464812872, 4.423285184949336646 ) ) ;
#19417=CARTESIAN_POINT ( 'NONE',  ( 2.656358736808067000, 121.0686911241271702, -0.2846299364715210722 ) ) ;
#19418=CARTESIAN_POINT ( 'NONE',  ( -0.3417028577848571502, 116.8490449975401617, 0.2775575361029122279 ) ) ;
#19419=VERTEX_POINT ( 'NONE', #5077 ) ;
#19421=ORIENTED_EDGE ( 'NONE', *, *, #22219, .F. ) ;
#19422=CARTESIAN_POINT ( 'NONE',  ( -6.642949970123351200, 30.31777535218072117, -0.3443277341910152556 ) ) ;
#19423=CARTESIAN_POINT ( 'NONE',  ( 5.933841582263978509, -14.80544765534526341, -0.2634432552157287555 ) ) ;
#19424=CARTESIAN_POINT ( 'NONE',  ( -13.46871114105396039, 122.4565580348552913, 1.263039180185647314 ) ) ;
#19425=CARTESIAN_POINT ( 'NONE',  ( 5.259787267153561707, 158.8115599018184412, -1.116423854902495849 ) ) ;
#19426=CARTESIAN_POINT ( 'NONE',  ( 4.364008504204949013, 7.202613900313124873, 1.580794030135405537 ) ) ;
#19431=CARTESIAN_POINT ( 'NONE',  ( 4.973583767373020770, 117.3966162183443203, 0.9753880922370259388 ) ) ;
#19433=CARTESIAN_POINT ( 'NONE',  ( -3.633016119382598941, 156.6183338678525558, 1.377765736259032758 ) ) ;
#19434=CARTESIAN_POINT ( 'NONE',  ( 5.041094711636397996, 117.2685085068581827, 0.6814997454729904147 ) ) ;
#19435=CARTESIAN_POINT ( 'NONE',  ( 7.522503210159232623, 120.3045338523282197, -1.038419263833407324 ) ) ;
#19436=CARTESIAN_POINT ( 'NONE',  ( -19.59170213216434320, 150.6586468064772646, -2.354958926090490845 ) ) ;
#19438=EDGE_LOOP ( 'NONE', ( #5833, #32444, #32657, #4911, #38520, #33190, #28553, #13902, #14595 ) ) ;
#19439=CARTESIAN_POINT ( 'NONE',  ( 4.485924072207432722, 118.1136089101166533, -0.5726866988169239114 ) ) ;
#19440=CARTESIAN_POINT ( 'NONE',  ( 13.98505335951042916, 150.2679186505038160, -0.6609695396245743870 ) ) ;
#19441=AXIS2_PLACEMENT_3D ( 'NONE', #17590, #1846, #2055 ) ;
#19443=CARTESIAN_POINT ( 'NONE',  ( -17.39571694528383361, 144.3974720067888313, -2.245075470287479114 ) ) ;
#19444=CARTESIAN_POINT ( 'NONE',  ( 2.617865251411226613, -15.35234423845867369, 4.678879665404411803 ) ) ;
#19447=CARTESIAN_POINT ( 'NONE',  ( -4.847551152455588763, 117.7642220418352679, 0.8118171574421505499 ) ) ;
#19448=CARTESIAN_POINT ( 'NONE',  ( 1.387234972287218593, 119.7856413326322667, 0.5781392410077789146 ) ) ;
#19450=CARTESIAN_POINT ( 'NONE',  ( 3.979181138743986601, 26.09377549647152961, 2.406711837290479661 ) ) ;
#19451=CARTESIAN_POINT ( 'NONE',  ( 10.32597032162030892, 126.0505730134521230, 0.3842079712423250859 ) ) ;
#19454=CARTESIAN_POINT ( 'NONE',  ( -6.426369768295692736E-14, 159.6054662015457382, 1.032716915552223178E-16 ) ) ;
#19456=LINE ( 'NONE', #6695, #39744 ) ;
#19459=DIRECTION ( 'NONE',  ( -0.9998004120163609398, 0.000000000000000000, -0.01997839162482749689 ) ) ;
#19463=CARTESIAN_POINT ( 'NONE',  ( -1.843513859164668034, 116.5452236745340429, 0.1029321673164913797 ) ) ;
#19468=CARTESIAN_POINT ( 'NONE',  ( 6.986329010373957260, 121.9533422367003510, 0.08619055661058230844 ) ) ;
#19470=CARTESIAN_POINT ( 'NONE',  ( 1.423520143629432910, 115.7027630957402238, -1.681658721634869513 ) ) ;
#19471=CARTESIAN_POINT ( 'NONE',  ( -2.816370844846016297, 121.0122979933374978, -0.1218616300372572514 ) ) ;
#19472=CARTESIAN_POINT ( 'NONE',  ( 6.101987814473650573, -12.39306998090061640, 0.4902605208062851827 ) ) ;
#19473=CARTESIAN_POINT ( 'NONE',  ( -20.25200034474484667, 150.8812763393641490, 1.391365372170581649 ) ) ;
#19475=CARTESIAN_POINT ( 'NONE',  ( 23.06561215160514422, 149.8841935741895384, 0.7910477959972080919 ) ) ;
#19476=CARTESIAN_POINT ( 'NONE',  ( 8.911975660322296378, 123.9583942952993993, 0.2665811367707756063 ) ) ;
#19478=CARTESIAN_POINT ( 'NONE',  ( 0.6244633603679663469, 9.902617207799803367, -0.7572168304597820532 ) ) ;
#19479=CARTESIAN_POINT ( 'NONE',  ( -23.40831777029536198, 146.8136392739129974, -0.6999192077533367140 ) ) ;
#19482=CARTESIAN_POINT ( 'NONE',  ( 5.707320923441908889, 118.0767569068514717, 1.090126761366801533 ) ) ;
#19485=CARTESIAN_POINT ( 'NONE',  ( 21.49578583461345005, 148.6087350971780836, 2.244132633923697551 ) ) ;
#19486=CARTESIAN_POINT ( 'NONE',  ( 12.07139305262844076, 121.8643784861682065, -1.276542069712922389 ) ) ;
#19487=CARTESIAN_POINT ( 'NONE',  ( -0.4136891606132181431, 9.424461778640809584, 0.8817368238460310259 ) ) ;
#19488=CARTESIAN_POINT ( 'NONE',  ( 1.824569540066833584, 15.47196788996624583, -8.237246883284143451 ) ) ;
#19489=CARTESIAN_POINT ( 'NONE',  ( -13.41577631804585202, 120.9245410081625209, -1.450210030139598594 ) ) ;
#19490=CARTESIAN_POINT ( 'NONE',  ( 4.685061364228054082, 117.8874929293646119, -0.8143947462202356657 ) ) ;
#19491=CARTESIAN_POINT ( 'NONE',  ( 3.930440796539790060, 109.7948460773305897, 3.685213129881072636 ) ) ;
#19492=CARTESIAN_POINT ( 'NONE',  ( -15.21929369751766714, 143.4245298570049840, -0.2523546585945006249 ) ) ;
#19493=VERTEX_POINT ( 'NONE', #21217 ) ;
#19494=CARTESIAN_POINT ( 'NONE',  ( -18.63140056563947411, 147.4429432625130119, -2.446051816127021716 ) ) ;
#19495=CARTESIAN_POINT ( 'NONE',  ( 5.949011718796170634, -14.81501284647598915, 0.9937821824230966827 ) ) ;
#19500=CARTESIAN_POINT ( 'NONE',  ( 2.214684683099545470, 157.4004113605966211, 1.675081295071568332 ) ) ;
#19501=CARTESIAN_POINT ( 'NONE',  ( 4.560443946511397506, -11.68866997254031936, 0.6947937310338139216 ) ) ;
#19503=CARTESIAN_POINT ( 'NONE',  ( -4.298926901474686701, 118.7880935209305591, 0.4986311761637902684 ) ) ;
#19504=CARTESIAN_POINT ( 'NONE',  ( 8.358864306157585133, 27.05150166619590379, -1.223686670289468870 ) ) ;
#19505=CARTESIAN_POINT ( 'NONE',  ( 9.165636745951982078, 123.6526633469202920, 0.6866826908162830811 ) ) ;
#19506=CARTESIAN_POINT ( 'NONE',  ( 22.64859486804662581, 149.7032342875954498, -0.6240689893612099137 ) ) ;
#19509=AXIS2_PLACEMENT_3D ( 'NONE', #924, #36695, #26889 ) ;
#19510=AXIS2_PLACEMENT_3D ( 'NONE', #18851, #131, #13096 ) ;
#19511=CARTESIAN_POINT ( 'NONE',  ( -0.0002511744761480867835, 116.4254662015457171, 0.01256979787922183657 ) ) ;
#19513=CARTESIAN_POINT ( 'NONE',  ( 6.591391745114316691, 120.5237581640276687, -0.8625721502728334045 ) ) ;
#19514=CARTESIAN_POINT ( 'NONE',  ( 22.83540780336915432, 150.4058779721138421, 0.4563057931615321361 ) ) ;
#19516=CARTESIAN_POINT ( 'NONE',  ( -15.98475566209953058, 146.3393691146323761, -1.048177900600803403 ) ) ;
#19517=CARTESIAN_POINT ( 'NONE',  ( 3.745401017337624872, -13.88268793655436717, 4.204469449000409753 ) ) ;
#19518=CARTESIAN_POINT ( 'NONE',  ( -5.135293214769152570, 116.9399052598554221, 0.1794300269087395205 ) ) ;
#19519=CARTESIAN_POINT ( 'NONE',  ( 8.216553068272158811, 117.5004391570743394, 0.1790601237764438691 ) ) ;
#19520=ORIENTED_EDGE ( 'NONE', *, *, #40789, .F. ) ;
#19521=CARTESIAN_POINT ( 'NONE',  ( -1.544744425833544099, 4.816215111148435923, 4.377641278133862279 ) ) ;
#19522=CARTESIAN_POINT ( 'NONE',  ( 3.559183564918581677, 105.1232307390661731, 3.986110174556340979 ) ) ;
#19523=CARTESIAN_POINT ( 'NONE',  ( -4.923390193968213424, 117.4088236311152542, 0.9490106074932443958 ) ) ;
#19526=CARTESIAN_POINT ( 'NONE',  ( 7.831006910361074880, 122.3515375996227590, 0.6751902815995498575 ) ) ;
#19527=CARTESIAN_POINT ( 'NONE',  ( -4.137704358559117779, 17.39492794009094823, -2.099109474953318788 ) ) ;
#19528=CARTESIAN_POINT ( 'NONE',  ( 22.07768208608584359, 150.1365687424457178, 1.739787554465966890 ) ) ;
#19530=CARTESIAN_POINT ( 'NONE',  ( -3.009276887026423264, 44.28946620154572855, 1.210121013456480377 ) ) ;
#19531=CARTESIAN_POINT ( 'NONE',  ( 14.84976704640051182, 123.2524255416106342, -1.171266444394655881 ) ) ;
#19532=CARTESIAN_POINT ( 'NONE',  ( 0.1277143096572389558, 15.67076514537015974, -4.628409624684062251 ) ) ;
#19533=CARTESIAN_POINT ( 'NONE',  ( -22.71262516694562805, 146.4845460041848355, -1.645735859231715503 ) ) ;
#19535=CARTESIAN_POINT ( 'NONE',  ( -0.006534791579925431325, 156.3267223255430167, 0.3270276925529296275 ) ) ;
#19536=CARTESIAN_POINT ( 'NONE',  ( 3.428369065731536658, -15.18705194980916851, 5.515041984116586526 ) ) ;
#19540=CARTESIAN_POINT ( 'NONE',  ( -0.01147819631913260877, 118.8623374019222894, 0.5744158801423951966 ) ) ;
#19542=CARTESIAN_POINT ( 'NONE',  ( -22.74864191258943080, 148.7873826295267747, 0.7277888646341180712 ) ) ;
#19543=CARTESIAN_POINT ( 'NONE',  ( 22.40468623258662362, 137.0915487549672491, -0.1281257692620773048 ) ) ;
#19547=CARTESIAN_POINT ( 'NONE',  ( 2.049043543842966386, -15.30400295934178345, 5.355738895901667185 ) ) ;
#19549=FACE_BOUND ( 'NONE', #9590, .T. ) ;
#19550=EDGE_CURVE ( 'NONE', #18840, #39307, #28673, .T. ) ;
#19551=CARTESIAN_POINT ( 'NONE',  ( -4.585060147380330520, 118.0136138934147993, 0.7023266209943478389 ) ) ;
#19555=CARTESIAN_POINT ( 'NONE',  ( 0.03523692298770234738, 115.6909491485452435, -1.763399716047880039 ) ) ;
#19556=( BOUNDED_CURVE ( )  B_SPLINE_CURVE ( 3, ( #7784, #36344, #17351, #563 ),
 .UNSPECIFIED., .F., .T. ) 
 B_SPLINE_CURVE_WITH_KNOTS ( ( 4, 4 ),
 ( 3.141592653589793116, 4.712388980384689674 ),
 .UNSPECIFIED. ) 
 CURVE ( )  GEOMETRIC_REPRESENTATION_ITEM ( )  RATIONAL_B_SPLINE_CURVE ( ( 1.000000000000000000, 0.8047378541243649375, 0.8047378541243649375, 1.000000000000000000 ) ) 
 REPRESENTATION_ITEM ( '' )  );
#19557=CARTESIAN_POINT ( 'NONE',  ( 3.544058460572470093, 118.6794394583634329, -0.7947981566704515055 ) ) ;
#19558=CARTESIAN_POINT ( 'NONE',  ( -4.730021378956903000, 112.7831754354443348, -2.563638443952895418 ) ) ;
#19559=CARTESIAN_POINT ( 'NONE',  ( 4.696638897187899175, 117.9693123291577024, 0.8144611834090730307 ) ) ;
#19560=DIRECTION ( 'NONE',  ( -0.9998004120163609398, 0.000000000000000000, -0.01997839162482749342 ) ) ;
#19561=CARTESIAN_POINT ( 'NONE',  ( -14.05504870572974419, 134.4521314832425389, -1.517394082013088674 ) ) ;
#19563=CARTESIAN_POINT ( 'NONE',  ( -3.999779825473023465, 115.7036092819612350, -1.581685738513307626 ) ) ;
#19566=CARTESIAN_POINT ( 'NONE',  ( 3.568456891169458078, 108.6786390861269922, -3.983803253449686110 ) ) ;
#19567=CARTESIAN_POINT ( 'NONE',  ( -5.014048726638253406, 156.2174774745075183, -1.508183953414442335 ) ) ;
#19570=CARTESIAN_POINT ( 'NONE',  ( -0.02399864187742892577, 159.1630378086529731, 1.200990174154242585 ) ) ;
#19572=CARTESIAN_POINT ( 'NONE',  ( -8.439845240644384461, 123.3184153607739404, -0.08348901510681934479 ) ) ;
#19573=CARTESIAN_POINT ( 'NONE',  ( 1.968029828064305153, -3.592386099649644837, 4.203610184747879508 ) ) ;
#19574=CARTESIAN_POINT ( 'NONE',  ( 14.40286820143207969, 120.3907653763288579, 0.8772178161575925337 ) ) ;
#19576=CARTESIAN_POINT ( 'NONE',  ( -5.078986093043186045, 85.18346620154574111, -0.1014902294541237954 ) ) ;
#19577=CARTESIAN_POINT ( 'NONE',  ( 3.879201355988149746, -15.32975156973215292, 1.565980057466964670 ) ) ;
#19578=CARTESIAN_POINT ( 'NONE',  ( -12.22472920326803525, 122.9664497093790629, 1.310580005724927499 ) ) ;
#19579=CARTESIAN_POINT ( 'NONE',  ( 0.7251766580790658390, 11.37246313919491314, 0.6538263676454795226 ) ) ;
#19580=CARTESIAN_POINT ( 'NONE',  ( -22.32005725002931484, 150.7328461917231550, -1.166919501784766666 ) ) ;
#19581=CARTESIAN_POINT ( 'NONE',  ( 0.9253733321238560849, 8.064964547470342637, 0.3089666344597190029 ) ) ;
#19582=ORIENTED_EDGE ( 'NONE', *, *, #31623, .F. ) ;
#19584=CARTESIAN_POINT ( 'NONE',  ( 7.643874070029819556, 124.9344662015457317, 0.1527427953284561934 ) ) ;
#19586=CARTESIAN_POINT ( 'NONE',  ( -0.7132078119428603147, 156.3865044363621450, 0.5782112914057383479 ) ) ;
#19587=CARTESIAN_POINT ( 'NONE',  ( 3.951736590037845609, -12.73914099834651203, 2.215835717905272784 ) ) ;
#19588=CARTESIAN_POINT ( 'NONE',  ( 9.926448497735728793, 122.5082557396031291, -1.019319756893169115 ) ) ;
#19589=CARTESIAN_POINT ( 'NONE',  ( -19.26131898708122137, 149.3473233412102275, -2.496341295301664154 ) ) ;
#19591=FACE_OUTER_BOUND ( 'NONE', #13528, .T. ) ;
#19592=CARTESIAN_POINT ( 'NONE',  ( -5.477793340596218918, 31.72728063616241201, 0.5271671279843670455 ) ) ;
#19594=CARTESIAN_POINT ( 'NONE',  ( 8.132787923797314633, 122.8458379852381910, -0.04721391815988586205 ) ) ;
#19596=CARTESIAN_POINT ( 'NONE',  ( 0.4875792343844080889, 105.8266127453845229, 5.318343663435395996 ) ) ;
#19598=FACE_OUTER_BOUND ( 'NONE', #38991, .T. ) ;
#19599=EDGE_CURVE ( 'NONE', #2172, #1729, #31867, .T. ) ;
#19602=CARTESIAN_POINT ( 'NONE',  ( 16.84917212821870436, 155.2300590059875844, 0.1976545469556810486 ) ) ;
#19603=CARTESIAN_POINT ( 'NONE',  ( -5.362262919127019245, 116.9387654363850260, 0.7435593652664854725 ) ) ;
#19604=CARTESIAN_POINT ( 'NONE',  ( -4.855449335888874174, 115.6909491485452719, 1.281272725539412294 ) ) ;
#19605=CARTESIAN_POINT ( 'NONE',  ( 4.114294302962228755, -10.72644468530807416, -2.136776772127288559 ) ) ;
#19606=CARTESIAN_POINT ( 'NONE',  ( -4.370579818869743782, 31.84755045023585751, 0.2525336677614991032 ) ) ;
#19607=CARTESIAN_POINT ( 'NONE',  ( 1.153229101628888476, 158.8088198215516229, 1.472604719115123029 ) ) ;
#19608=CARTESIAN_POINT ( 'NONE',  ( 3.547999066118234346, 14.38381850277834317, -2.990331240093012877 ) ) ;
#19609=CARTESIAN_POINT ( 'NONE',  ( -3.468545696377880461, 29.88095345675903403, -7.690089085670218871 ) ) ;
#19610=CARTESIAN_POINT ( 'NONE',  ( 8.739301385803836197, 118.0314441295146679, -0.4462037359528160940 ) ) ;
#19611=CARTESIAN_POINT ( 'NONE',  ( -0.5453179846285600707, 107.9696733310005214, -4.488644025489748834 ) ) ;
#19614=CARTESIAN_POINT ( 'NONE',  ( -2.188542869591966866, 104.6144662015456959, 4.302051086437162830 ) ) ;
#19615=CARTESIAN_POINT ( 'NONE',  ( -1.287880193524239658, 20.15907059199006923, -4.440276399826991849 ) ) ;
#19618=CARTESIAN_POINT ( 'NONE',  ( 2.858040400949144022, -14.78363303536489681, 4.300485631455113200 ) ) ;
#19619=CARTESIAN_POINT ( 'NONE',  ( 2.994815693583348537, 122.7580772961051707, -0.09506955764664386244 ) ) ;
#19620=CARTESIAN_POINT ( 'NONE',  ( -9.680782865131792647, 118.1749183431956425, 0.3159967629729718008 ) ) ;
#19623=ORIENTED_EDGE ( 'NONE', *, *, #22899, .F. ) ;
#19625=CARTESIAN_POINT ( 'NONE',  ( 5.114706464973534317, -15.35711304900182128, 3.188446684335360271 ) ) ;
#19626=CARTESIAN_POINT ( 'NONE',  ( -2.272333812996736757, 118.4336326928681729, 0.6977090181727383378 ) ) ;
#19627=CARTESIAN_POINT ( 'NONE',  ( 21.87215423617511334, 148.4185114426368841, -1.275166548224078822 ) ) ;
#19628=CARTESIAN_POINT ( 'NONE',  ( 4.574821423538755205, -2.080616851812391310, 0.6590154617212384824 ) ) ;
#19630=EDGE_CURVE ( 'NONE', #40413, #20535, #3512, .T. ) ;
#19632=CARTESIAN_POINT ( 'NONE',  ( 0.02009831008142323738, 106.6745790697264056, 5.014625686322316866 ) ) ;
#19633=( LENGTH_UNIT ( ) NAMED_UNIT ( * ) SI_UNIT ( .MILLI., .METRE. ) );
#19634=CARTESIAN_POINT ( 'NONE',  ( -11.98504388954668087, 126.0992317015783328, 1.027991910846090207 ) ) ;
#19635=CARTESIAN_POINT ( 'NONE',  ( -6.573280687130626123E-14, 88.99346620154574339, 1.699031322814114629E-29 ) ) ;
#19636=AXIS2_PLACEMENT_3D ( 'NONE', #19247, #9462, #38235 ) ;
#19637=ADVANCED_FACE ( 'NONE', ( #22063 ), #20473, .F. ) ;
#19638=CARTESIAN_POINT ( 'NONE',  ( 8.477251816686347752, 120.7201681212196291, -1.097727670418841450 ) ) ;
#19640=CARTESIAN_POINT ( 'NONE',  ( -6.881618033700713788, 158.0090104422344268, -1.782742279240755456 ) ) ;
#19643=CARTESIAN_POINT ( 'NONE',  ( 4.505706913051673368, 118.1291065022491154, -0.5122133236055396166 ) ) ;
#19644=CARTESIAN_POINT ( 'NONE',  ( 1.542034982439605795, 120.6610732671444595, -0.2472410911860530025 ) ) ;
#19646=CARTESIAN_POINT ( 'NONE',  ( -4.277613954752526482, 119.9149831030956932, -0.8793409099722718780 ) ) ;
#19647=CARTESIAN_POINT ( 'NONE',  ( 3.848634119772940565, -15.36481979860233871, 1.996958912074897396 ) ) ;
#19648=FACE_OUTER_BOUND ( 'NONE', #1217, .T. ) ;
#19651=CARTESIAN_POINT ( 'NONE',  ( -4.820374670814820739, 117.7660393779071057, 0.8433105318405139661 ) ) ;
#19652=CARTESIAN_POINT ( 'NONE',  ( 10.79589323670136736, 123.3109526380878833, 1.504350731661494134 ) ) ;
#19653=CARTESIAN_POINT ( 'NONE',  ( -2.742835824903626207, 31.05151501484152732, 0.8589415642670262807 ) ) ;
#19655=CARTESIAN_POINT ( 'NONE',  ( 4.300553167417687561, 27.50566818391071422, -1.719522505244270860 ) ) ;
#19656=CARTESIAN_POINT ( 'NONE',  ( 8.534567384671277068, 123.3353292868209365, 0.2519373819028137285 ) ) ;
#19661=CARTESIAN_POINT ( 'NONE',  ( 5.564123858037556936, 116.7166602743764514, -0.04122317672195889571 ) ) ;
#19666=FACE_OUTER_BOUND ( 'NONE', #39504, .T. ) ;
#19667=DIRECTION ( 'NONE',  ( 0.01997839162482749689, 1.040247600000945640E-18, -0.9998004120163610509 ) ) ;
#19671=CARTESIAN_POINT ( 'NONE',  ( -5.719359222665208797, 159.1232349745254453, 0.1048325176007954412 ) ) ;
#19674=CARTESIAN_POINT ( 'NONE',  ( -6.052889781086392418, 121.4336901549234113, -0.1296568525282296436 ) ) ;
#19676=CARTESIAN_POINT ( 'NONE',  ( 3.566795953268722563, 115.7029539211179667, -1.489760979346105518 ) ) ;
#19677=CARTESIAN_POINT ( 'NONE',  ( -9.190025975546058490, 124.2403664864748549, -0.2180328680397457530 ) ) ;
#19678=CARTESIAN_POINT ( 'NONE',  ( 2.294645149923727701, -15.44887909491890454, 5.922367448919703570 ) ) ;
#19679=CARTESIAN_POINT ( 'NONE',  ( -16.31190729917925708, 125.3309463260932830, 1.192360770973151851 ) ) ;
#19681=CARTESIAN_POINT ( 'NONE',  ( 13.50792085693134048, 119.6474162840860771, 0.5731308571144442254 ) ) ;
#19682=DIRECTION ( 'NONE',  ( -4.017660918040594346E-17, 1.000000000000000000, 2.376309959284834438E-19 ) ) ;
#19683=CARTESIAN_POINT ( 'NONE',  ( 5.267996062361754994, 115.6909491485453145, -0.8700017381306309749 ) ) ;
#19684=CARTESIAN_POINT ( 'NONE',  ( -0.9401033786448180773, 4.191251494893229790, 0.2723526238743522732 ) ) ;
#19685=CARTESIAN_POINT ( 'NONE',  ( -16.23049043870597075, 121.3954344197762083, -0.4305223454732413080 ) ) ;
#19688=CARTESIAN_POINT ( 'NONE',  ( 2.553816101320873333, 116.8400682929857481, 0.5498680602850822829 ) ) ;
#19689=ORIENTED_EDGE ( 'NONE', *, *, #26485, .F. ) ;
#19690=CARTESIAN_POINT ( 'NONE',  ( -17.20821608673157144, 140.2562023718666353, 1.644530994948828928 ) ) ;
#19692=CARTESIAN_POINT ( 'NONE',  ( 21.44537552191012608, 145.9698620541949765, 2.253500464710097795 ) ) ;
#19693=CARTESIAN_POINT ( 'NONE',  ( 0.4598942929538996638, 118.4074432378348689, -0.5883637925338033314 ) ) ;
#19694=CARTESIAN_POINT ( 'NONE',  ( 0.4369565669422456611, 1.205365006982008547, 0.8739355888918843851 ) ) ;
#19695=CARTESIAN_POINT ( 'NONE',  ( -16.77501307560222799, 125.2521365416322254, -1.703383479906432685 ) ) ;
#19696=CARTESIAN_POINT ( 'NONE',  ( 4.742695500909063000, 117.8453989086928004, -0.8301742325441545667 ) ) ;
#19697=CARTESIAN_POINT ( 'NONE',  ( 6.329649118423095189, 120.0627515544778134, 0.4542292512502630886 ) ) ;
#19699=CARTESIAN_POINT ( 'NONE',  ( 10.18692116311725648, 123.6566696788710686, -0.8138387218406052392 ) ) ;
#19700=CARTESIAN_POINT ( 'NONE',  ( -9.108749339472550943, 153.9337724597031070, -0.1375672075132167438 ) ) ;
#19701=VERTEX_POINT ( 'NONE', #5704 ) ;
#19702=CARTESIAN_POINT ( 'NONE',  ( -14.41820472940927900, 152.7616507467334372, -2.289036833064873822 ) ) ;
#19704=CIRCLE ( 'NONE', #13575, 0.5080000000000002292 ) ;
#19705=CARTESIAN_POINT ( 'NONE',  ( 5.825557336981400880, -14.92341722037543406, 1.564612827344095569 ) ) ;
#19706=CARTESIAN_POINT ( 'NONE',  ( -4.769585057922912874, 31.49133049583777932, -0.6989730246579993755 ) ) ;
#19710=CARTESIAN_POINT ( 'NONE',  ( 14.47078677760122467, 128.5519869857110393, 2.060874889273090815 ) ) ;
#19711=CARTESIAN_POINT ( 'NONE',  ( 0.2924095564367995559, 116.4254662015451913, 0.005843038833677049321 ) ) ;
#19712=CARTESIAN_POINT ( 'NONE',  ( -3.568793996894023657, 120.2162445758188056, 0.3416935720284705602 ) ) ;
#19713=CARTESIAN_POINT ( 'NONE',  ( 8.348643983786249834, 26.63118458923209175, 1.112826146890550483 ) ) ;
#19714=CARTESIAN_POINT ( 'NONE',  ( 1.635131992100914200, 156.2910218135955631, 0.4893959945316868065 ) ) ;
#19715=CARTESIAN_POINT ( 'NONE',  ( 21.45272375726293035, 151.3201912522522719, -0.6338752469853822236 ) ) ;
#19717=CARTESIAN_POINT ( 'NONE',  ( -6.583861033951825950E-14, 91.02546620154572565, 1.480257718193877056E-29 ) ) ;
#19718=TOROIDAL_SURFACE ( 'NONE', #7501, 5.080000000000005400, 0.5080000000000000071 ) ;
#19719=CARTESIAN_POINT ( 'NONE',  ( -22.83607019214389666, 150.4065277667444036, -0.4307393832409497914 ) ) ;
#19721=CARTESIAN_POINT ( 'NONE',  ( 8.032207078087980179, 121.5191168587267185, -0.8512761726684724417 ) ) ;
#19722=CARTESIAN_POINT ( 'NONE',  ( 2.081416901521091933, -15.50639809317535089, 5.943648939154567934 ) ) ;
#19723=CARTESIAN_POINT ( 'NONE',  ( -1.635131992101042986, 156.2910218135955631, -0.4893959945316865845 ) ) ;
#19724=CARTESIAN_POINT ( 'NONE',  ( 4.304563788583176454, -12.55325912034982494, 2.095985231258857162 ) ) ;
#19725=CARTESIAN_POINT ( 'NONE',  ( 23.29144772315967771, 149.3526176766912101, 0.4654185560736371352 ) ) ;
#19727=CARTESIAN_POINT ( 'NONE',  ( 2.801506786573456420, 9.139157206818806500, -3.684590140147142368 ) ) ;
#19728=CARTESIAN_POINT ( 'NONE',  ( 4.623799210569877083, 105.1214572271058785, 2.682504979537780443 ) ) ;
#19729=CARTESIAN_POINT ( 'NONE',  ( -4.801687489738192482, 117.4019780203432646, 1.015655943361054581 ) ) ;
#19731=CARTESIAN_POINT ( 'NONE',  ( 5.918055438912293909, 120.3534538399959786, 1.025969926474026517 ) ) ;
#19732=CARTESIAN_POINT ( 'NONE',  ( 0.1277143096572389558, 15.67076514537015974, -4.628409624684062251 ) ) ;
#19733=CARTESIAN_POINT ( 'NONE',  ( 4.843103592331835294, 117.3073154462328063, 0.6875571908837337931 ) ) ;
#19736=CARTESIAN_POINT ( 'NONE',  ( 18.63828149932687595, 131.8045874826418071, -1.403896228398082036 ) ) ;
#19737=CARTESIAN_POINT ( 'NONE',  ( 3.490194016315742331, 12.22236127277748174, 3.029891289224248219 ) ) ;
#19738=CARTESIAN_POINT ( 'NONE',  ( -14.11323155926173456, 120.5239346615589540, -1.094216903015625020 ) ) ;
#19742=CARTESIAN_POINT ( 'NONE',  ( -15.80820582674417274, 146.9282941555416073, 0.1367419433413215590 ) ) ;
#19743=CARTESIAN_POINT ( 'NONE',  ( 6.341500637990160172, -13.03620802017263536, 0.6512942508830525945 ) ) ;
#19748=CARTESIAN_POINT ( 'NONE',  ( 16.71878049915325448, 131.5287050380659082, 2.312093064668929721 ) ) ;
#19750=DIRECTION ( 'NONE',  ( -0.9998004120163608288, 0.000000000000000000, -0.01997839162482750383 ) ) ;
#19751=CARTESIAN_POINT ( 'NONE',  ( -22.27630879610708803, 150.1947564971097222, 0.7286472789443333431 ) ) ;
#19752=CARTESIAN_POINT ( 'NONE',  ( 1.824569540066833584, 15.47196788996624583, -8.237246883284143451 ) ) ;
#19753=CARTESIAN_POINT ( 'NONE',  ( 23.08840689075971753, 149.5685596498530288, -0.1330139495868549737 ) ) ;
#19758=CARTESIAN_POINT ( 'NONE',  ( 2.209012367505132080, -15.11364764369361957, 5.670533105609369073 ) ) ;
#19760=CARTESIAN_POINT ( 'NONE',  ( -5.078986093043185157, 75.78546620154573077, -0.1014902294541231847 ) ) ;
#19761=CARTESIAN_POINT ( 'NONE',  ( -4.473658520889312484, 118.1283618854176893, 0.5455511291602485047 ) ) ;
#19764=ORIENTED_EDGE ( 'NONE', *, *, #30849, .F. ) ;
#19765=ORIENTED_EDGE ( 'NONE', *, *, #15940, .T. ) ;
#19766=CARTESIAN_POINT ( 'NONE',  ( -1.565525540593865950, 118.7629491485440099, -1.245867024842673532 ) ) ;
#19767=CARTESIAN_POINT ( 'NONE',  ( 6.175143553146828168, 119.5953855062382871, -1.005919626096980490 ) ) ;
#19768=CARTESIAN_POINT ( 'NONE',  ( -6.465481721428130157, 120.6581566633936404, -0.3941859656685692270 ) ) ;
#19770=CARTESIAN_POINT ( 'NONE',  ( 4.512464582872506291, 118.1196997639598862, 0.6561311196536673274 ) ) ;
#19772=CARTESIAN_POINT ( 'NONE',  ( -10.02582114772209287, 123.8737202207250618, -1.106617482833785804 ) ) ;
#19775=CARTESIAN_POINT ( 'NONE',  ( 7.304536785993802184, 123.0387167848234355, 0.07720001398428681660 ) ) ;
#19776=CARTESIAN_POINT ( 'NONE',  ( -15.81386139960078197, 149.2064892436030163, -1.885719434888957657 ) ) ;
#19778=CARTESIAN_POINT ( 'NONE',  ( -0.0005468344959711694646, 156.3034662015456604, 0.02736583427618486872 ) ) ;
#19779=CARTESIAN_POINT ( 'NONE',  ( 7.966529119766866174, 121.8269078720123701, -0.7202784793015850617 ) ) ;
#19780=CARTESIAN_POINT ( 'NONE',  ( -7.045758995674062497, 122.0730845715159063, -0.06312930854005696646 ) ) ;
#19781=EDGE_CURVE ( 'NONE', #20726, #10933, #7180, .T. ) ;
#19782=CARTESIAN_POINT ( 'NONE',  ( 4.219463811995017188, -1.205994944679912306, -1.932895124392335573 ) ) ;
#19783=CARTESIAN_POINT ( 'NONE',  ( 15.01050271945730863, 120.7699597703182945, 0.9001124940000719832 ) ) ;
#19784=CARTESIAN_POINT ( 'NONE',  ( 5.586884702347362897, 130.0144662015457300, 0.1116392523995368424 ) ) ;
#19785=CARTESIAN_POINT ( 'NONE',  ( 1.871808270187516943, -15.45276866356297418, 5.379583495939216142 ) ) ;
#19786=CARTESIAN_POINT ( 'NONE',  ( -0.5002616235673846834, 119.0154928070276412, 0.5875571981567379032 ) ) ;
#19787=CARTESIAN_POINT ( 'NONE',  ( -0.8879284396340286767, 8.347861319067646946, 0.4041202799994399464 ) ) ;
#19788=CARTESIAN_POINT ( 'NONE',  ( -1.889792677999466486, 116.7132768022172797, -0.3078404110637329993 ) ) ;
#19789=CARTESIAN_POINT ( 'NONE',  ( 0.8148283262528154269, -11.57344599616632763, 0.5628321559398594687 ) ) ;
#19791=EDGE_CURVE ( 'NONE', #37473, #10724, #8937, .T. ) ;
#19793=CARTESIAN_POINT ( 'NONE',  ( 1.237704251691374546, 106.3840144300045409, 5.116357776886615305 ) ) ;
#19795=CARTESIAN_POINT ( 'NONE',  ( -14.11809548624358435, 150.3034377993741657, 0.8008162161465686157 ) ) ;
#19796=CARTESIAN_POINT ( 'NONE',  ( 4.273959209556542405, -12.80518358089995168, 2.504334382443756724 ) ) ;
#19797=CARTESIAN_POINT ( 'NONE',  ( 2.082154424532988379, 156.9412006218898057, -1.407003841209468531 ) ) ;
#19798=CARTESIAN_POINT ( 'NONE',  ( -9.988019213705189969, 120.6268241347409855, -1.591717657363032723 ) ) ;
#19800=AXIS2_PLACEMENT_3D ( 'NONE', #31760, #2603, #6206 ) ;
#19802=CARTESIAN_POINT ( 'NONE',  ( 1.854781166956293248, -15.20994639552496253, 5.427130820981656001 ) ) ;
#19803=CARTESIAN_POINT ( 'NONE',  ( -0.02863553844924360964, 38.94824868342700341, -0.3880333552236577277 ) ) ;
#19804=CARTESIAN_POINT ( 'NONE',  ( 15.79043079689192552, 145.9231181611787918, 0.08479106802855336522 ) ) ;
#19807=DIRECTION ( 'NONE',  ( -4.017660918040594346E-17, 1.000000000000000000, 2.376309959284834438E-19 ) ) ;
#19810=CARTESIAN_POINT ( 'NONE',  ( -5.028575548160166164, 117.3993840946898075, 0.6249845981789815541 ) ) ;
#19812=CARTESIAN_POINT ( 'NONE',  ( 17.22554230343049397, 122.7389118244895769, 0.2345756144184562297 ) ) ;
#19813=CARTESIAN_POINT ( 'NONE',  ( -0.3655860903869697087, 105.8811906981200934, 5.329044222542315801 ) ) ;
#19815=CARTESIAN_POINT ( 'NONE',  ( -4.758926732810884630, 118.7629491485454309, 0.8043858395770803194 ) ) ;
#19817=CARTESIAN_POINT ( 'NONE',  ( -3.688991022714105839, 31.45506795701765412, -0.1149108006718590896 ) ) ;
#19818=CARTESIAN_POINT ( 'NONE',  ( 21.10215338253914297, 147.9292434580435724, 2.361242315759021437 ) ) ;
#19819=CARTESIAN_POINT ( 'NONE',  ( -1.792273654952471595, 16.32048121479114045, -4.264856162967389785 ) ) ;
#19820=CARTESIAN_POINT ( 'NONE',  ( -6.340062920055459017, 30.52953040661039807, -5.581008500864042432 ) ) ;
#19821=CARTESIAN_POINT ( 'NONE',  ( -8.714206658535026406, 118.0327614349573366, -0.7961205384438058141 ) ) ;
#19822=CARTESIAN_POINT ( 'NONE',  ( -0.7330347863451183166, 118.7604188656930120, -0.9075975635256806617 ) ) ;
#19826=CARTESIAN_POINT ( 'NONE',  ( -1.280342683972266693, 105.1232991681604858, 5.188841635131638874 ) ) ;
#19828=CARTESIAN_POINT ( 'NONE',  ( -1.178223178616622402, 14.53665720681882689, 4.476207649055042204 ) ) ;
#19829=CARTESIAN_POINT ( 'NONE',  ( 4.784930192204152277, 117.3993836135881708, 1.202631631483913832 ) ) ;
#19831=CARTESIAN_POINT ( 'NONE',  ( 1.826496821415126037, -15.21410320048187437, 5.439012564009855666 ) ) ;
#19833=CARTESIAN_POINT ( 'NONE',  ( 1.604275531929067578, 118.9836165220538504, -0.7112099450351575536 ) ) ;
#19835=CARTESIAN_POINT ( 'NONE',  ( -13.14342457437329159, 119.8381915656929380, 0.4562891928474253067 ) ) ;
#19841=CARTESIAN_POINT ( 'NONE',  ( 3.255875469058810978, -15.74984210207193414, 5.086368125509904026 ) ) ;
#19842=CARTESIAN_POINT ( 'NONE',  ( -20.17730036299085938, 147.7236477000422497, 1.702857440531004407 ) ) ;
#19843=CARTESIAN_POINT ( 'NONE',  ( 4.934953413367771269, 117.8999350694477926, -0.7268823312289467431 ) ) ;
#19845=CARTESIAN_POINT ( 'NONE',  ( 0.9647673288271847447, 27.50405299253531410, 0.1566625405351598777 ) ) ;
#19848=CARTESIAN_POINT ( 'NONE',  ( -4.848458278871826010, 117.4106395692391516, -1.171953005487281096 ) ) ;
#19849=CARTESIAN_POINT ( 'NONE',  ( 0.9570916872344990001, 123.2612876230388395, 0.1732974146428332418 ) ) ;
#19850=CARTESIAN_POINT ( 'NONE',  ( 4.961775220622199889, 117.4031003928707548, 1.033713290510416716 ) ) ;
#19851=CARTESIAN_POINT ( 'NONE',  ( -12.98740932513253554, 152.2092440956282076, 1.257387005612584874 ) ) ;
#19852=CARTESIAN_POINT ( 'NONE',  ( -4.962228733194765873, 117.4031047975369404, -1.033509257472498444 ) ) ;
#19853=CARTESIAN_POINT ( 'NONE',  ( 11.64084037886360257, 123.0696236843973281, -1.242201319703144069 ) ) ;
#19854=CARTESIAN_POINT ( 'NONE',  ( -4.023942337083176390, 118.1249481555716301, -0.9214969356372303411 ) ) ;
#19857=CARTESIAN_POINT ( 'NONE',  ( 4.464715371412748546, 118.1580834965288318, -0.4253963240309212024 ) ) ;
#19858=CARTESIAN_POINT ( 'NONE',  ( 8.002172173406759015, 154.6030710842251494, -0.4507127070663226043 ) ) ;
#19860=CARTESIAN_POINT ( 'NONE',  ( -12.10021064141429292, 153.5325627063460843, -2.025425248842403825 ) ) ;
#19861=CARTESIAN_POINT ( 'NONE',  ( 3.411744169395244164, -14.91921274028452871, 2.011823270444000666 ) ) ;
#19862=CARTESIAN_POINT ( 'NONE',  ( -5.145869062083050061, 105.1220833959279730, -1.445893102178412715 ) ) ;
#19863=AXIS2_PLACEMENT_3D ( 'NONE', #18150, #33531, #4782 ) ;
#19866=CARTESIAN_POINT ( 'NONE',  ( -3.254339884055971854, 0.1279812147911008058, 3.287934741457726684 ) ) ;
#19867=CARTESIAN_POINT ( 'NONE',  ( 10.41670863957350512, 122.9580799906392343, 1.467069541016857048 ) ) ;
#19868=CARTESIAN_POINT ( 'NONE',  ( -2.394634909045491700, 30.36160847033138310, 1.723844942078720521 ) ) ;
#19869=CARTESIAN_POINT ( 'NONE',  ( 4.622858883031034871, 26.85595184169372374, 0.2084198311932836112 ) ) ;
#19870=CARTESIAN_POINT ( 'NONE',  ( 9.185235947232817111, 124.1858035287836231, 0.2689572614166577114 ) ) ;
#19871=CARTESIAN_POINT ( 'NONE',  ( -4.026309595109284878, 109.3894556192956173, 3.506482798589841465 ) ) ;
#19872=CIRCLE ( 'NONE', #12418, 3.683000000000001162 ) ;
#19879=DIRECTION ( 'NONE',  ( -0.01997839162482737546, -1.040247600000940825E-18, 0.9998004120163610509 ) ) ;
#19881=CARTESIAN_POINT ( 'NONE',  ( -4.074955089416341991, 118.2429491485453354, 0.1454234154749719787 ) ) ;
#19885=CARTESIAN_POINT ( 'NONE',  ( -2.784667331447816974, 116.5968896900294709, 0.09290643507641029031 ) ) ;
#19886=ORIENTED_EDGE ( 'NONE', *, *, #1448, .T. ) ;
#19888=CARTESIAN_POINT ( 'NONE',  ( -7.789722586531418358, 122.5884748538522047, -0.3097450211583079316 ) ) ;
#19892=CARTESIAN_POINT ( 'NONE',  ( -5.974701571114539256, 155.3719879121972838, -0.2191910023528569340 ) ) ;
#19893=CARTESIAN_POINT ( 'NONE',  ( 6.387155697962850986, -12.89254730397265725, 0.3290856906432634288 ) ) ;
#19894=CARTESIAN_POINT ( 'NONE',  ( -2.167900391131186044, 117.8876587302075194, 0.6265904732959522994 ) ) ;
#19895=CARTESIAN_POINT ( 'NONE',  ( -4.598301960400187127, 22.30806413504685537, 0.5496829067130363233 ) ) ;
#19896=CARTESIAN_POINT ( 'NONE',  ( 8.021187395864771474, 158.6806155330135084, 0.3964977924059487346 ) ) ;
#19898=CARTESIAN_POINT ( 'NONE',  ( 9.420913146467203347, 124.7671794033526851, 0.3269489669365729934 ) ) ;
#19899=CARTESIAN_POINT ( 'NONE',  ( 4.847733185841858194, 115.6909491485453145, -1.282834277461510908 ) ) ;
#19900=CARTESIAN_POINT ( 'NONE',  ( 0.5139362334885246852, 0.5165572279304807557, -0.8313783143454911428 ) ) ;
#19901=CARTESIAN_POINT ( 'NONE',  ( -23.34743456777632531, 142.7586093370927074, -0.6964168797349270523 ) ) ;
#19905=CARTESIAN_POINT ( 'NONE',  ( -2.274883502654467815, 116.3490410268270665, 0.1699064989630479361 ) ) ;
#19907=CARTESIAN_POINT ( 'NONE',  ( -15.87040186760635407, 150.9007765090757971, 1.629155861667390903 ) ) ;
#19909=CARTESIAN_POINT ( 'NONE',  ( 9.146501239663530569, 119.1751624949753534, 1.313831160619747473 ) ) ;
#19910=CARTESIAN_POINT ( 'NONE',  ( 19.88689915616616233, 147.6055923437354238, -1.726923636697636377 ) ) ;
#19911=CARTESIAN_POINT ( 'NONE',  ( -0.2316695588195925026, 0.1309245165040176240, 0.9467938775014126396 ) ) ;
#19912=CARTESIAN_POINT ( 'NONE',  ( -21.80375291804149285, 148.4185114426368841, -2.147915116047498962 ) ) ;
#19913=CARTESIAN_POINT ( 'NONE',  ( 4.667063153570271794, 118.0255431904385404, -0.5722037917038420574 ) ) ;
#19914=CARTESIAN_POINT ( 'NONE',  ( 6.530233653228945556, 120.6338824379019172, 0.3959831657380196712 ) ) ;
#19916=CARTESIAN_POINT ( 'NONE',  ( 17.03225580939797013, 146.4457527449227143, -1.249628170391535509 ) ) ;
#19917=CARTESIAN_POINT ( 'NONE',  ( -8.041889123127157646, 122.8518031662551948, -0.1606960833125205546 ) ) ;
#19919=CARTESIAN_POINT ( 'NONE',  ( -11.93340282868953750, 123.0912118827050108, -1.763528850166467210 ) ) ;
#19920=CARTESIAN_POINT ( 'NONE',  ( 5.059117473032719303, -15.50674158137822722, 2.046454293345789655 ) ) ;
#19922=CARTESIAN_POINT ( 'NONE',  ( -4.596595486785018281, 117.9777161510301227, -0.9190962615854699758 ) ) ;
#19924=CARTESIAN_POINT ( 'NONE',  ( 4.145420271487251895, 118.2391365653420650, 0.3994957887817748299 ) ) ;
#19925=CARTESIAN_POINT ( 'NONE',  ( 0.9182646862278995847, 157.4778559999684830, 1.599919928990593210 ) ) ;
#19926=CARTESIAN_POINT ( 'NONE',  ( -0.01249116623180958861, 38.87185441664305330, -1.227828225846576693 ) ) ;
#19928=CARTESIAN_POINT ( 'NONE',  ( 15.19604463793433169, 156.0859089222169587, 0.3036531364422415669 ) ) ;
#19930=CARTESIAN_POINT ( 'NONE',  ( -0.3027292972884025324, 105.9597790263619146, 5.298406829468305546 ) ) ;
#19931=CARTESIAN_POINT ( 'NONE',  ( -8.379105243356219646, 21.88232641057985361, -0.8402904295462267914 ) ) ;
#19932=CARTESIAN_POINT ( 'NONE',  ( 13.78138926674702525, 150.2278160098252329, 0.9796190600867308307 ) ) ;
#19934=CARTESIAN_POINT ( 'NONE',  ( 1.373401713467732543, 159.5224216140176168, -0.5650407700211931283 ) ) ;
#19938=CARTESIAN_POINT ( 'NONE',  ( -16.30362368704351539, 121.4145675751456253, -0.3085868453551564583 ) ) ;
#19940=CARTESIAN_POINT ( 'NONE',  ( -7.964318472288553608, 121.6586585215090679, -1.114152107595608676 ) ) ;
#19941=CARTESIAN_POINT ( 'NONE',  ( 6.373744154335938994, -13.69897431215970052, 0.7397752478428293310 ) ) ;
#19942=CARTESIAN_POINT ( 'NONE',  ( -7.868938471672525026, 154.6027768716304820, -0.5345728592648680833 ) ) ;
#19943=CARTESIAN_POINT ( 'NONE',  ( 2.810721824165392846, -14.60963343767143741, 5.218503737131710452 ) ) ;
#19944=CARTESIAN_POINT ( 'NONE',  ( -14.20701772348855130, 121.1589565784038456, 0.8306491748466006131 ) ) ;
#19946=CARTESIAN_POINT ( 'NONE',  ( 13.67522198567651515, 119.6429072192227494, 0.3220992662749119217 ) ) ;
#19948=ORIENTED_EDGE ( 'NONE', *, *, #10800, .F. ) ;
#19949=CARTESIAN_POINT ( 'NONE',  ( 4.114294302962228755, -10.72644468530807416, -2.136776772127288559 ) ) ;
#19950=CARTESIAN_POINT ( 'NONE',  ( 4.033169965737029017, 105.1222026749920246, 3.507333144493335109 ) ) ;
#19953=CARTESIAN_POINT ( 'NONE',  ( 8.178139910812117108, 120.5865972341469359, 1.415288944234376345 ) ) ;
#19954=CARTESIAN_POINT ( 'NONE',  ( 4.382351430540762927, 4.226039240006542741, -1.512498627010908647 ) ) ;
#19955=CARTESIAN_POINT ( 'NONE',  ( 17.71751426720048173, 153.9999837190418930, 1.728000864493653976 ) ) ;
#19956=CARTESIAN_POINT ( 'NONE',  ( -6.631541954483209765E-14, 98.39146620154573952, -1.863789202389766375E-18 ) ) ;
#19957=CARTESIAN_POINT ( 'NONE',  ( 19.75353020121325187, 136.1149058410947532, -1.478659091479562759 ) ) ;
#19959=CARTESIAN_POINT ( 'NONE',  ( -2.651420880294951488, 7.049774601622781134, -3.792306073587544901 ) ) ;
#19960=CARTESIAN_POINT ( 'NONE',  ( -0.9938236163261908729, 116.9791385580615781, -0.3849800449318573348 ) ) ;
#19963=AXIS2_PLACEMENT_3D ( 'NONE', #9919, #34866, #18867 ) ;
#19964=CARTESIAN_POINT ( 'NONE',  ( -9.835128631862042781, 124.8790005272986861, 0.1409026022053574689 ) ) ;
#19965=CARTESIAN_POINT ( 'NONE',  ( 3.036109343602874322, -15.28514977651167150, 5.695352409590039855 ) ) ;
#19968=CARTESIAN_POINT ( 'NONE',  ( 3.198224922426783579, -14.19254063666773291, 2.189163805996276579 ) ) ;
#19970=CARTESIAN_POINT ( 'NONE',  ( 17.77132669990250236, 135.5811125208551857, 2.431814553008901481 ) ) ;
#19973=CARTESIAN_POINT ( 'NONE',  ( 7.869802931801260115, 122.7053923345152953, 0.1572573916674578076 ) ) ;
#19974=CARTESIAN_POINT ( 'NONE',  ( -9.582280438405419432, 118.3624989119526418, 0.5072503739029416980 ) ) ;
#19975=CARTESIAN_POINT ( 'NONE',  ( 6.480130183504051011, 21.94006803110874415, 5.378050974841823262 ) ) ;
#19976=CARTESIAN_POINT ( 'NONE',  ( 3.247806582136902431, 159.4494809562368971, -0.3030341850868439324 ) ) ;
#19981=CARTESIAN_POINT ( 'NONE',  ( -4.937777651546055857, 117.4065511353899041, -1.082295458227385154 ) ) ;
#19984=CARTESIAN_POINT ( 'NONE',  ( -4.402139039590816871, 118.1614230090776800, 0.4936525752913482057 ) ) ;
#19988=CARTESIAN_POINT ( 'NONE',  ( 3.904474273848753008, 119.0221123855851033, -0.7730353223355832526 ) ) ;
#19989=CARTESIAN_POINT ( 'NONE',  ( -6.266908424742289263, 120.0898888515776264, -0.4521870875522996380 ) ) ;
#19990=CARTESIAN_POINT ( 'NONE',  ( 4.516265718371130333, 118.0894310158977021, 0.7770291299768713467 ) ) ;
#19991=CARTESIAN_POINT ( 'NONE',  ( -15.03094698176529853, 148.9283877096812034, -1.255086756411655902 ) ) ;
#19994=CARTESIAN_POINT ( 'NONE',  ( 1.586608521452973486, 106.2379067940291293, -5.113598281387616851 ) ) ;
#19995=CARTESIAN_POINT ( 'NONE',  ( -17.21112184089944463, 146.3482411845097886, -2.056990446313781362 ) ) ;
#19996=DIRECTION ( 'NONE',  ( -0.9998004120163610509, -4.016384292689131511E-17, -0.01997839162482749689 ) ) ;
#19998=CARTESIAN_POINT ( 'NONE',  ( 8.614520148390900189, 118.6763556054874158, -0.8198081090887602285 ) ) ;
#19999=CARTESIAN_POINT ( 'NONE',  ( -14.67652612023663039, 148.8571924874472074, -0.2271985726276186113 ) ) ;
#20000=CARTESIAN_POINT ( 'NONE',  ( -4.399545650080316506, 2.442302885307133131, -1.471791394725966873 ) ) ;
#20001=CARTESIAN_POINT ( 'NONE',  ( 13.14908049612667185, 156.9583929045107595, 0.9825115876436357754 ) ) ;
#20002=CARTESIAN_POINT ( 'NONE',  ( -6.451606698686837575E-14, 65.62546620154573418, 4.217636114931141265E-29 ) ) ;
#20003=CARTESIAN_POINT ( 'NONE',  ( 3.118150858982619233, -14.63350761981947734, -0.02509704758125085033 ) ) ;
#20005=CARTESIAN_POINT ( 'NONE',  ( -18.96108613168469503, 147.8663216482595146, 1.723626476717959433 ) ) ;
#20006=CARTESIAN_POINT ( 'NONE',  ( -0.08600706866453224075, 15.02498995931601122, -0.9728917428382349852 ) ) ;
#20007=CARTESIAN_POINT ( 'NONE',  ( -18.42221188220390360, 125.1790410860780298, -0.8413473246917883008 ) ) ;
#20008=CARTESIAN_POINT ( 'NONE',  ( -0.4650136207426652235, -7.476398416381191403, -0.8572754866018892361 ) ) ;
#20009=ORIENTED_EDGE ( 'NONE', *, *, #32940, .F. ) ;
#20011=CARTESIAN_POINT ( 'NONE',  ( 7.563243396832008081, 124.2956292408697863, 0.1602470646927417752 ) ) ;
#20012=CARTESIAN_POINT ( 'NONE',  ( -9.482824821900010193, 153.9068681542131856, 0.6648444853843686886 ) ) ;
#20013=CARTESIAN_POINT ( 'NONE',  ( 4.284293204009990141, -11.98693494109343050, 1.176118521537933725 ) ) ;
#20014=CARTESIAN_POINT ( 'NONE',  ( 17.71558884668061751, 147.6919162452172145, -1.529690151225475470 ) ) ;
#20016=CARTESIAN_POINT ( 'NONE',  ( -2.398927117899045225, 157.8629595415303584, -1.727538386417435179 ) ) ;
#20017=CARTESIAN_POINT ( 'NONE',  ( 3.385259569132474944, 115.7029692307686162, 1.641278830299353508 ) ) ;
#20018=CARTESIAN_POINT ( 'NONE',  ( 1.979733141779612016, -15.19599036556555660, 5.309005240801834447 ) ) ;
#20019=CARTESIAN_POINT ( 'NONE',  ( -4.223161182163281957, 33.49016550088244060, 2.148155765408566342 ) ) ;
#20020=CARTESIAN_POINT ( 'NONE',  ( 9.248842176949983340, 124.1957968681474824, 0.02334546025992364007 ) ) ;
#20022=CARTESIAN_POINT ( 'NONE',  ( -3.182864231321134163, 107.7307366742556667, 4.270808201732677389 ) ) ;
#20023=CARTESIAN_POINT ( 'NONE',  ( 0.1816879500932431502, 105.8845321911205133, 5.338643427584144341 ) ) ;
#20026=CARTESIAN_POINT ( 'NONE',  ( 5.789608264049557640, 116.9447284183608389, 0.03249775470882608486 ) ) ;
#20027=CARTESIAN_POINT ( 'NONE',  ( -5.317809737553872651, 116.7000894413872629, 0.8094161617621953297 ) ) ;
#20028=CARTESIAN_POINT ( 'NONE',  ( -3.205472953781653533, 118.7629491485510442, 1.047959515690910060 ) ) ;
#20030=CARTESIAN_POINT ( 'NONE',  ( -5.208405493689606480, 31.38331509014777154, -0.6716542322870746595 ) ) ;
#20031=CARTESIAN_POINT ( 'NONE',  ( 2.699166815671171005, 158.5977336698458089, 1.597229775447004618 ) ) ;
#20032=CARTESIAN_POINT ( 'NONE',  ( -0.9239673467531356321, 25.61616486456964736, -4.531977062890359065 ) ) ;
#20033=CARTESIAN_POINT ( 'NONE',  ( -6.244303144875123834, 11.31477948022340208, -5.679040650537692692 ) ) ;
#20034=CARTESIAN_POINT ( 'NONE',  ( -8.636847134335058129, 118.3872487031030403, -1.029711822167878710 ) ) ;
#20035=CARTESIAN_POINT ( 'NONE',  ( -2.157690779482436927, 123.3349985135950959, -0.1620144005770981221 ) ) ;
#20036=CARTESIAN_POINT ( 'NONE',  ( 4.847990641624395636, 117.4106256157386809, 1.172052288416076005 ) ) ;
#20038=CARTESIAN_POINT ( 'NONE',  ( -1.157812389548250165, 104.6144662015456959, 4.694735647476201201 ) ) ;
#20039=CARTESIAN_POINT ( 'NONE',  ( -4.374560056058969693, 13.03735028915297534, 1.504755201125916875 ) ) ;
#20041=CARTESIAN_POINT ( 'NONE',  ( -3.168818291390510300, 117.3993833748032216, -1.398835752645559927 ) ) ;
#20042=CARTESIAN_POINT ( 'NONE',  ( 3.066387819753066069, -14.51305101688413224, 3.912045622741378903 ) ) ;
#20044=CARTESIAN_POINT ( 'NONE',  ( 2.578112510117919864, 120.6526784328644339, -0.3421008684282440537 ) ) ;
#20045=CARTESIAN_POINT ( 'NONE',  ( -1.373401713467861329, 159.5224216140176168, 0.5650407700211933504 ) ) ;
#20046=CARTESIAN_POINT ( 'NONE',  ( 4.828582363101557640, 117.4037123032867385, -1.009936161916218378 ) ) ;
#20050=CARTESIAN_POINT ( 'NONE',  ( -2.667392527469405916, 31.33771804890096746, 0.9893360403373154810 ) ) ;
#20051=CARTESIAN_POINT ( 'NONE',  ( 3.166528004143551289, -15.72052770450255110, 4.635360722337766859 ) ) ;
#20052=CARTESIAN_POINT ( 'NONE',  ( -20.46161261025647349, 147.6366098820875266, 1.667455336067830807 ) ) ;
#20053=CARTESIAN_POINT ( 'NONE',  ( 9.254844111042901389, 119.0402042963619351, -0.8977872906997165225 ) ) ;
#20054=CARTESIAN_POINT ( 'NONE',  ( 0.3093957028193324299, 29.65535775802675289, -0.9258560203679269129 ) ) ;
#20058=CARTESIAN_POINT ( 'NONE',  ( 0.8285762425323237590, 121.5536190086353372, 0.3701497059917960297 ) ) ;
#20059=CARTESIAN_POINT ( 'NONE',  ( -3.514252322483388813, 120.2313485970928326, 0.5318214084310807221 ) ) ;
#20061=CARTESIAN_POINT ( 'NONE',  ( 18.22365405440197250, 148.2327041560005512, -1.660465927639720229 ) ) ;
#20062=CARTESIAN_POINT ( 'NONE',  ( -20.20973109032216541, 149.9354415288716780, -2.375026552130124369 ) ) ;
#20065=CARTESIAN_POINT ( 'NONE',  ( 4.463504259782801853, 118.1585507804028907, -0.4269113537636273770 ) ) ;
#20066=CARTESIAN_POINT ( 'NONE',  ( 2.740744172220221042, 120.7841308545065431, -0.2151145298216794455 ) ) ;
#20068=CARTESIAN_POINT ( 'NONE',  ( 3.261251233531137217, -14.70027692227136917, 2.623613175195522285 ) ) ;
#20070=ADVANCED_FACE ( 'NONE', ( #16310 ), #3485, .T. ) ;
#20072=CARTESIAN_POINT ( 'NONE',  ( 1.583070580811935191, 1.852152477310867074, 4.353984577079609508 ) ) ;
#20073=CARTESIAN_POINT ( 'NONE',  ( 5.838061318222974805, 120.4133487461328826, 1.005638731867922964 ) ) ;
#20074=CARTESIAN_POINT ( 'NONE',  ( -2.525735733961075979, 30.63084530247838444, 1.130430605335521310 ) ) ;
#20075=CARTESIAN_POINT ( 'NONE',  ( 4.087030650986479330, 6.990161447142720696, 2.163025551504125232 ) ) ;
#20076=CARTESIAN_POINT ( 'NONE',  ( 9.099523502024073451, 123.9936668703698075, 0.3412791990392153307 ) ) ;
#20079=CARTESIAN_POINT ( 'NONE',  ( 8.797372769768484702, 117.7003220351452910, 0.04568619392659034606 ) ) ;
#20080=CARTESIAN_POINT ( 'NONE',  ( -0.8290918312103936483, 117.3993839334940077, 1.455271914084780738 ) ) ;
#20086=DIRECTION ( 'NONE',  ( 0.9998004120163608288, 0.000000000000000000, 0.01997839162482736852 ) ) ;
#20090=CARTESIAN_POINT ( 'NONE',  ( -21.84047376210821767, 151.4369626909183637, 0.009531295849831233555 ) ) ;
#20093=CARTESIAN_POINT ( 'NONE',  ( 6.982279026085625340, 121.9522648198741024, 0.07242179238622248327 ) ) ;
#20096=CARTESIAN_POINT ( 'NONE',  ( -7.557080711912884219, 122.4263405438208991, -0.1815966937148653093 ) ) ;
#20097=CARTESIAN_POINT ( 'NONE',  ( 5.816378023188423896, -13.23522671163289388, 2.128111738716565338 ) ) ;
#20098=CARTESIAN_POINT ( 'NONE',  ( -14.09802512849282863, 121.9525460547650226, 1.083329899170117683 ) ) ;
#20099=CARTESIAN_POINT ( 'NONE',  ( -0.3239230800893593276, 29.42979164457532804, -4.628216972995994993 ) ) ;
#20100=CARTESIAN_POINT ( 'NONE',  ( 17.01700507317042366, 122.6950552906510694, 0.6769824155666206433 ) ) ;
#20101=CARTESIAN_POINT ( 'NONE',  ( 10.90720410752496150, 127.9361718968202126, 0.3766330825069126864 ) ) ;
#20102=CARTESIAN_POINT ( 'NONE',  ( 3.655561289726139140, 27.93047918286777076, -2.829280713513928180 ) ) ;
#20103=CARTESIAN_POINT ( 'NONE',  ( -0.4866770014159069180, -4.230873095947595530, 0.8487236227246106601 ) ) ;
#20104=CARTESIAN_POINT ( 'NONE',  ( -1.404208078696352002, 159.5982469381528972, -0.2156159867753335013 ) ) ;
#20106=EDGE_CURVE ( 'NONE', #23143, #17488, #11458, .T. ) ;
#20107=CARTESIAN_POINT ( 'NONE',  ( -6.654617103318593247E-14, 104.6144662015457243, 1.534725424433578570E-31 ) ) ;
#20110=CARTESIAN_POINT ( 'NONE',  ( 2.266257171229604683, 116.3486079626738530, 0.2607109679900413424 ) ) ;
#20111=CARTESIAN_POINT ( 'NONE',  ( -17.98452544307437506, 146.6345634702618952, 1.580200905155535018 ) ) ;
#20113=CARTESIAN_POINT ( 'NONE',  ( 11.86420439699943330, 156.4809912657682673, 1.954521554489341062 ) ) ;
#20114=CARTESIAN_POINT ( 'NONE',  ( 15.53591925045075861, 153.1703808545849483, -1.736877461573578030 ) ) ;
#20115=CARTESIAN_POINT ( 'NONE',  ( 0.9728917428133897483, -6.565010040704528649, -0.08600706860408523224 ) ) ;
#20116=CARTESIAN_POINT ( 'NONE',  ( -14.28642979620163267, 121.5541609676003389, -1.504719748795722012 ) ) ;
#20117=CARTESIAN_POINT ( 'NONE',  ( 4.672671725886756278, 117.9840379399288395, -0.6970879283291996353 ) ) ;
#20118=CARTESIAN_POINT ( 'NONE',  ( 4.761265772527523588, 104.6144662015456959, 0.8484901397391942934 ) ) ;
#20119=CARTESIAN_POINT ( 'NONE',  ( 6.676265340062377263, 155.5185402614932570, -1.076558685701346940 ) ) ;
#20120=CARTESIAN_POINT ( 'NONE',  ( -6.500720044509902706, 121.7799842514348541, -0.1008652220075045153 ) ) ;
#20121=EDGE_LOOP ( 'NONE', ( #29170, #23282 ) ) ;
#20122=CARTESIAN_POINT ( 'NONE',  ( -2.275810046414789678, 157.5529522918930638, -1.704261365023472141 ) ) ;
#20123=CARTESIAN_POINT ( 'NONE',  ( 3.858334187661429215, -15.75373651934012997, 4.144460154494749915 ) ) ;
#20125=CARTESIAN_POINT ( 'NONE',  ( -4.716528458602361695, 117.9480174125288414, -0.8296297511114593126 ) ) ;
#20126=ADVANCED_FACE ( 'NONE', ( #29706 ), #41901, .T. ) ;
#20128=CARTESIAN_POINT ( 'NONE',  ( 4.065926199369043204, 118.2429491485453354, 0.3080910687088499467 ) ) ;
#20129=PRODUCT ( 'Center Spindle', 'Center Spindle', '', ( #20424 ) ) ;
#20130=CARTESIAN_POINT ( 'NONE',  ( 9.734001924785392390, 155.3230018269108825, 2.058186707467866583 ) ) ;
#20131=CARTESIAN_POINT ( 'NONE',  ( -4.834802360910630981, 32.27718159487177729, 0.9856153350916389000 ) ) ;
#20133=CARTESIAN_POINT ( 'NONE',  ( 1.798461198689400797, 116.4670535197835051, 0.02282230188723655823 ) ) ;
#20135=CARTESIAN_POINT ( 'NONE',  ( 8.331117840153179799, 7.414970825009634225, 1.249357972265521255 ) ) ;
#20136=CARTESIAN_POINT ( 'NONE',  ( 14.86280047924396008, 148.8756053271976327, 1.012714816113364780 ) ) ;
#20138=CARTESIAN_POINT ( 'NONE',  ( 1.353295744334168216, 159.4649289425152858, -0.7236632733165270226 ) ) ;
#20141=CARTESIAN_POINT ( 'NONE',  ( 0.7582820727000408878, 118.7629491485454025, 1.270951156714173580 ) ) ;
#20143=CARTESIAN_POINT ( 'NONE',  ( -15.48485754026178540, 120.7065362441885981, -0.2052890747276163996 ) ) ;
#20145=CARTESIAN_POINT ( 'NONE',  ( -7.924630949180505368, 121.8615034964088295, -1.018655858764297761 ) ) ;
#20147=CARTESIAN_POINT ( 'NONE',  ( -9.187421481788835109, 153.8854248570426080, -0.5770480568347666761 ) ) ;
#20148=CARTESIAN_POINT ( 'NONE',  ( 3.901187470525758094, -13.68826627043556776, 3.907672046116945186 ) ) ;
#20149=CARTESIAN_POINT ( 'NONE',  ( -19.78757913416918868, 132.0165317526581816, 1.053352019815566587 ) ) ;
#20150=CARTESIAN_POINT ( 'NONE',  ( -2.884051542275779756, 156.0957788938021054, -0.05763021347587621995 ) ) ;
#20151=CARTESIAN_POINT ( 'NONE',  ( 5.755000932441415529, 159.1151184437813981, 0.1316611545253207338 ) ) ;
#20153=CARTESIAN_POINT ( 'NONE',  ( -4.187759052228169132, -5.978784877027076838, 2.003160513425938483 ) ) ;
#20154=CARTESIAN_POINT ( 'NONE',  ( -3.284316801889665349, 105.1240599693624631, 4.214405307443403359 ) ) ;
#20155=CARTESIAN_POINT ( 'NONE',  ( -4.825036788391023457, 51.14746620154573264, -0.09641571798141751470 ) ) ;
#20157=CARTESIAN_POINT ( 'NONE',  ( -6.395303539164157947, 119.4668496938549396, 1.005475218501896251 ) ) ;
#20158=CARTESIAN_POINT ( 'NONE',  ( -4.603752034695621553, -0.9465464349810851497, 0.4006815057252178236 ) ) ;
#20159=CARTESIAN_POINT ( 'NONE',  ( 22.34269864632755898, 148.4347612714453248, 1.893969414928640793 ) ) ;
#20162=CARTESIAN_POINT ( 'NONE',  ( 20.57754816582968260, 149.5144255282053223, -1.563875036196712420 ) ) ;
#20163=CARTESIAN_POINT ( 'NONE',  ( -2.587970193024280441, -12.16632112844677494, -3.833404006186521773 ) ) ;
#20164=CARTESIAN_POINT ( 'NONE',  ( -1.336693583852524458, 159.4956652290339605, -0.6991310044172545091 ) ) ;
#20167=CIRCLE ( 'NONE', #20830, 5.588000000000006295 ) ;
#20168=CARTESIAN_POINT ( 'NONE',  ( -2.776805996813621391, 120.9068798055765370, 0.1259499506852534423 ) ) ;
#20169=CARTESIAN_POINT ( 'NONE',  ( 3.435007001638270996, -15.26001923902611779, 5.499761658607620340 ) ) ;
#20171=CARTESIAN_POINT ( 'NONE',  ( -4.679371059064479255, 111.8765634536042626, -2.628838740615948577 ) ) ;
#20173=CARTESIAN_POINT ( 'NONE',  ( 18.24829758291878434, 150.1405190176936344, 2.471583571221721343 ) ) ;
#20175=DIRECTION ( 'NONE',  ( -5.206863593109713661E-17, 1.000000000000000000, -1.077750396879097183E-30 ) ) ;
#20177=CARTESIAN_POINT ( 'NONE',  ( -22.59368173950844749, 146.4122051224262577, 0.8656317577275310926 ) ) ;
#20178=ADVANCED_FACE ( 'NONE', ( #19343 ), #16730, .T. ) ;
#20179=CARTESIAN_POINT ( 'NONE',  ( 7.154006291674216200, 2.952895779142483246, 4.500751621275830061 ) ) ;
#20180=CARTESIAN_POINT ( 'NONE',  ( 0.5759676376929014907, 120.3589971203204669, 0.3694376532493068854 ) ) ;
#20182=CARTESIAN_POINT ( 'NONE',  ( 22.98897055778763132, 149.8455236008688303, -0.1339715990509169341 ) ) ;
#20187=CARTESIAN_POINT ( 'NONE',  ( -4.493393903509352860, 118.1153619691203573, 0.5661490535317686978 ) ) ;
#20192=CARTESIAN_POINT ( 'NONE',  ( -3.944803911500280869, 119.0966328791857762, -0.9223804097932700730 ) ) ;
#20193=CARTESIAN_POINT ( 'NONE',  ( -5.244916502329433960, 116.2229785614576798, -1.177106425564501402 ) ) ;
#20194=CARTESIAN_POINT ( 'NONE',  ( 4.491034488983506101, 118.0837758977322238, 0.7972306053495301637 ) ) ;
#20195=CARTESIAN_POINT ( 'NONE',  ( -15.74774640517369662, 148.1776054874778197, -1.420244701258233988 ) ) ;
#20196=CARTESIAN_POINT ( 'NONE',  ( -0.5744809549289578987, 115.7029491485453292, -1.760674903347913212 ) ) ;
#20197=CARTESIAN_POINT ( 'NONE',  ( 1.620813648195540191, 117.9496053335228822, -1.310909995308043197 ) ) ;
#20198=CARTESIAN_POINT ( 'NONE',  ( 0.8805184999822103231, 105.9455060897651748, -5.280965183963572507 ) ) ;
#20199=CARTESIAN_POINT ( 'NONE',  ( -4.351716102370955852, 120.3584862571861436, -0.7474562918332058326 ) ) ;
#20200=CARTESIAN_POINT ( 'NONE',  ( 5.299048467822902175, 104.6144662015457527, -1.294354682138050050 ) ) ;
#20202=CARTESIAN_POINT ( 'NONE',  ( 8.334503520420716072, 120.0709494557483339, -1.118110265123128055 ) ) ;
#20203=CARTESIAN_POINT ( 'NONE',  ( -15.78614082382951977, 146.2329385241212378, -0.1139063483988971143 ) ) ;
#20204=FACE_OUTER_BOUND ( 'NONE', #2225, .T. ) ;
#20205=CARTESIAN_POINT ( 'NONE',  ( 21.97734904378678422, 136.8935083344700558, 1.380722529463845660 ) ) ;
#20206=DIRECTION ( 'NONE',  ( -4.017660918040594346E-17, 1.000000000000000000, 2.376309959284834438E-19 ) ) ;
#20207=CARTESIAN_POINT ( 'NONE',  ( 3.392805262616394035, -14.86080682751021698, 1.607197643132475040 ) ) ;
#20208=CARTESIAN_POINT ( 'NONE',  ( -17.15907173562178301, 135.3907879583883869, 1.705144375702607462 ) ) ;
#20209=CARTESIAN_POINT ( 'NONE',  ( -0.06925455797148694081, -4.192134993018743927, -0.9746272421430232091 ) ) ;
#20210=CARTESIAN_POINT ( 'NONE',  ( -22.38168272118577207, 137.0915487549672491, -1.023064006592828035 ) ) ;
#20212=CARTESIAN_POINT ( 'NONE',  ( 0.5759086045921885111, -9.199343823100290862, -0.7873135961421041662 ) ) ;
#20215=CARTESIAN_POINT ( 'NONE',  ( 4.758673294993224445, 116.4582014290525507, 1.187054331573000665 ) ) ;
#20216=CARTESIAN_POINT ( 'NONE',  ( -16.12610658153788634, 147.0533492130506943, 0.6457432798159423726 ) ) ;
#20217=CARTESIAN_POINT ( 'NONE',  ( 4.523112235310252416, -13.07411707498565256, 2.966381825927230764 ) ) ;
#20218=CARTESIAN_POINT ( 'NONE',  ( 10.60072409500453894, 154.2769816202975051, -1.465916755537046257 ) ) ;
#20219=CARTESIAN_POINT ( 'NONE',  ( -0.9995654073149882191, 157.9544661020348997, -1.649992931013676056 ) ) ;
#20220=CARTESIAN_POINT ( 'NONE',  ( -2.605357903967354893, 104.6144662015456959, 4.072382052623323645 ) ) ;
#20221=CARTESIAN_POINT ( 'NONE',  ( 1.826496821415126037, -15.21410320048187437, 5.439012564009855666 ) ) ;
#20222=CARTESIAN_POINT ( 'NONE',  ( -4.796574687651021129, 117.5429962573173981, -1.162632163661158735 ) ) ;
#20223=CARTESIAN_POINT ( 'NONE',  ( 14.69813734295220442, 148.8396455022467535, 0.06702550439777867075 ) ) ;
#20226=CARTESIAN_POINT ( 'NONE',  ( -4.687559322878096957, 113.9922470800761687, 1.949581705681876276 ) ) ;
#20227=CARTESIAN_POINT ( 'NONE',  ( 4.824354732525579337, 115.9539249584174740, 1.371586674499254421 ) ) ;
#20229=CARTESIAN_POINT ( 'NONE',  ( 3.967518560505680636, 117.3993838585351881, 1.334307535890729035 ) ) ;
#20230=EDGE_CURVE ( 'NONE', #17780, #35799, #35610, .T. ) ;
#20231=CARTESIAN_POINT ( 'NONE',  ( -5.008948584507882273, 27.92152162925472325, 0.4889012661100834434 ) ) ;
#20232=CARTESIAN_POINT ( 'NONE',  ( 22.83127913370401529, 150.4067493646842593, 0.3029848903584390074 ) ) ;
#20233=CARTESIAN_POINT ( 'NONE',  ( -1.581412096509254628, 106.2431249238853894, 5.111785082781967304 ) ) ;
#20234=CARTESIAN_POINT ( 'NONE',  ( 2.067624514165773419, -15.48293130374715787, 5.973957261547347741 ) ) ;
#20236=CARTESIAN_POINT ( 'NONE',  ( -4.870677750350147051, 117.7576918812740558, -0.8062859734791398836 ) ) ;
#20237=CARTESIAN_POINT ( 'NONE',  ( 13.20682171306282449, 121.8780043825237982, 1.728041046422398086 ) ) ;
#20239=CARTESIAN_POINT ( 'NONE',  ( 0.7039615705130309875, 19.50765702457006157, -8.391957350905826729 ) ) ;
#20240=CARTESIAN_POINT ( 'NONE',  ( 2.231875883732710619, 116.9306593240908683, -0.4829567074209755173 ) ) ;
#20241=CARTESIAN_POINT ( 'NONE',  ( -0.1328480158796658539, 107.4969721965504021, -4.685401909699153045 ) ) ;
#20244=CARTESIAN_POINT ( 'NONE',  ( -0.05238710761692585982, 113.0327356262574341, 2.621665085262908867 ) ) ;
#20245=CARTESIAN_POINT ( 'NONE',  ( -3.609430071560130848, 3.966570591990036032, 2.889066364458971137 ) ) ;
#20248=CARTESIAN_POINT ( 'NONE',  ( 3.370512099616890467, -13.86485436517860492, 3.147780574041331825 ) ) ;
#20249=CARTESIAN_POINT ( 'NONE',  ( 5.811537524186114467, 124.3836500214474654, 0.1011232793223460352 ) ) ;
#20250=CARTESIAN_POINT ( 'NONE',  ( -18.06489503062833535, 125.1493905788104684, 0.4137567899827963025 ) ) ;
#20255=CARTESIAN_POINT ( 'NONE',  ( 3.150932678494966055, -15.78083729861913476, 4.935700751529307873 ) ) ;
#20256=CARTESIAN_POINT ( 'NONE',  ( -4.124323422702007136, 118.5849532427036905, 0.8258982430451994317 ) ) ;
#20257=CARTESIAN_POINT ( 'NONE',  ( 4.114294302962228755, -10.72644468530807416, -2.136776772127288559 ) ) ;
#20261=CARTESIAN_POINT ( 'NONE',  ( -0.07931638298556013822, 106.1822392402443143, 5.212590348647615279 ) ) ;
#20263=CARTESIAN_POINT ( 'NONE',  ( -6.553475369667642880, 120.9817801663137971, 0.6941111757064589716 ) ) ;
#20265=CARTESIAN_POINT ( 'NONE',  ( 14.85905242749865707, 128.5561590274816126, -1.519445497462470263 ) ) ;
#20266=CARTESIAN_POINT ( 'NONE',  ( -11.58042324368383014, 121.0393782313542346, -1.653871040030608475 ) ) ;
#20267=PLANE ( 'NONE',  #19509 ) ;
#20269=CARTESIAN_POINT ( 'NONE',  ( 4.117084068517360862, 118.2429491485453354, -0.1876423749214011782 ) ) ;
#20270=CARTESIAN_POINT ( 'NONE',  ( 13.37097581265829938, 134.1388935151753401, -0.4393653360420517462 ) ) ;
#20272=CARTESIAN_POINT ( 'NONE',  ( 3.348477204222540138, -14.79883842983281639, 1.177367440313774605 ) ) ;
#20273=CARTESIAN_POINT ( 'NONE',  ( 1.490983790026257028, 105.1236484711430847, -5.131369187154176004 ) ) ;
#20276=CARTESIAN_POINT ( 'NONE',  ( -3.663749374568059380, -0.07195744677916669774, 2.838909333946205482 ) ) ;
#20277=CARTESIAN_POINT ( 'NONE',  ( 5.014048726638124620, 156.2174774745075183, 1.508183953414442557 ) ) ;
#20278=CARTESIAN_POINT ( 'NONE',  ( -2.647397774264983017, 29.53842282114184670, -0.004108860927264268610 ) ) ;
#20279=CARTESIAN_POINT ( 'NONE',  ( 4.076717266748975277, 8.489475128091552136, -2.202413229635628689 ) ) ;
#20280=CARTESIAN_POINT ( 'NONE',  ( 11.17680165766851808, 128.1157469881088105, 0.4152311708251575362 ) ) ;
#20281=CARTESIAN_POINT ( 'NONE',  ( -5.101912418190827303, 113.7221701807922329, 1.664754118330573851 ) ) ;
#20283=CARTESIAN_POINT ( 'NONE',  ( -5.544930032391052421, 116.7707190791428928, -0.4007225579332259202 ) ) ;
#20284=CARTESIAN_POINT ( 'NONE',  ( 8.078287538471617069, 158.6595088495342338, 0.1614234102745199240 ) ) ;
#20288=CARTESIAN_POINT ( 'NONE',  ( -6.529493367164978770E-14, 72.99146620154573384, -7.899616498973244731E-18 ) ) ;
#20292=CARTESIAN_POINT ( 'NONE',  ( 0.4220321208936545498, 124.6436471961814050, -0.02396868521112067649 ) ) ;
#20293=CARTESIAN_POINT ( 'NONE',  ( -20.63094779205708562, 152.5829384802601396, 0.02634999427677331418 ) ) ;
#20296=CARTESIAN_POINT ( 'NONE',  ( 6.967896315201691948, 121.9471128632948620, 0.02251729312944412628 ) ) ;
#20300=CARTESIAN_POINT ( 'NONE',  ( -12.88021573494099314, 133.7932622986943159, -0.3045934876098301269 ) ) ;
#20301=CARTESIAN_POINT ( 'NONE',  ( 6.169188725349925129, -14.24425063093240418, 1.535968726618487379 ) ) ;
#20303=CARTESIAN_POINT ( 'NONE',  ( -21.06902287100059823, 145.7918284779248665, 1.526944944257475845 ) ) ;
#20304=CARTESIAN_POINT ( 'NONE',  ( -4.563195415240126174, 21.88328375387019165, -0.7336086519975816289 ) ) ;
#20305=CARTESIAN_POINT ( 'NONE',  ( 11.56079167746327130, 118.7825156662901378, 0.6096482884850571438 ) ) ;
#20307=CARTESIAN_POINT ( 'NONE',  ( 3.211436584971100849, 28.15539441671475274, -3.345526564039049688 ) ) ;
#20308=CARTESIAN_POINT ( 'NONE',  ( 0.7576854961709549308, -2.078890728193560467, 0.6140693529290401909 ) ) ;
#20309=CARTESIAN_POINT ( 'NONE',  ( -0.9122582399081905491, 116.5216256635990391, -0.1489946802529017456 ) ) ;
#20312=CARTESIAN_POINT ( 'NONE',  ( 5.539609713687273285, 116.8468292325185587, 0.4796846802364603812 ) ) ;
#20313=CARTESIAN_POINT ( 'NONE',  ( -17.40456409200978527, 148.7932787949812905, 1.578286399122462935 ) ) ;
#20315=CARTESIAN_POINT ( 'NONE',  ( 2.141138273642768208, 117.8876587302075194, 0.7126953207602170215 ) ) ;
#20316=CARTESIAN_POINT ( 'NONE',  ( 13.00445675891829467, 122.7019651155717384, -1.321991537619922497 ) ) ;
#20317=CARTESIAN_POINT ( 'NONE',  ( -0.1719059670432218079, -9.367746741450257986, 0.9581547781327369728 ) ) ;
#20318=CARTESIAN_POINT ( 'NONE',  ( -13.54946078406819332, 121.5020190402118203, -1.609302047640724931 ) ) ;
#20320=CARTESIAN_POINT ( 'NONE',  ( 4.971145480241967007, 105.1217302803469664, 1.943640820323331742 ) ) ;
#20321=ADVANCED_FACE ( 'NONE', ( #40593 ), #27783, .T. ) ;
#20322=CARTESIAN_POINT ( 'NONE',  ( 3.332096981532907343, 156.3062290909284116, -1.017430637527963588 ) ) ;
#20323=CARTESIAN_POINT ( 'NONE',  ( 7.785313405276816034, 122.6175842484440324, 0.2316741178401685586 ) ) ;
#20325=CARTESIAN_POINT ( 'NONE',  ( -12.01154561878613336, 123.1955650103826798, -1.772196977085516156 ) ) ;
#20326=CARTESIAN_POINT ( 'NONE',  ( 5.270497567351643653, -15.36183412081716604, 0.7307456425073816098 ) ) ;
#20328=CARTESIAN_POINT ( 'NONE',  ( -4.565208948191195937, 118.0820071162333988, -0.7244444172681095973 ) ) ;
#20331=CARTESIAN_POINT ( 'NONE',  ( 4.065926199369043204, 118.2429491485453354, 0.3080910687088499467 ) ) ;
#20332=CARTESIAN_POINT ( 'NONE',  ( 8.349261126152542900, 120.8878392079396065, 1.399984990019641717 ) ) ;
#20333=CARTESIAN_POINT ( 'NONE',  ( -4.679832524073478162, 32.47693947602098063, 1.143146696348500635 ) ) ;
#20335=CARTESIAN_POINT ( 'NONE',  ( 0.0002511744760192916428, 116.4254662015457171, -0.01256979787922172728 ) ) ;
#20336=CARTESIAN_POINT ( 'NONE',  ( -7.546363725996330984, 11.73557930518083303, -3.739946900464478752 ) ) ;
#20337=CARTESIAN_POINT ( 'NONE',  ( 6.479597433594296518, 121.6155390319085683, 0.5171962410403526667 ) ) ;
#20339=CARTESIAN_POINT ( 'NONE',  ( 14.74755344529021173, 121.0688405154646858, -0.6244351273456010265 ) ) ;
#20342=CARTESIAN_POINT ( 'NONE',  ( -16.27668397883912377, 121.4070763266325628, -0.2738251655545989038 ) ) ;
#20343=ORIENTED_EDGE ( 'NONE', *, *, #35530, .F. ) ;
#20345=CARTESIAN_POINT ( 'NONE',  ( -6.800033062875029621, 121.3213576459294529, -0.8666892964309956815 ) ) ;
#20348=DIRECTION ( 'NONE',  ( -5.206863593109713661E-17, 1.000000000000000000, -1.077750396879097183E-30 ) ) ;
#20349=CARTESIAN_POINT ( 'NONE',  ( -10.48728279712184452, 126.1106773019354819, -0.5683957799248650078 ) ) ;
#20350=CARTESIAN_POINT ( 'NONE',  ( 3.920414950246539298, -14.18668476855415506, 4.724392046630619291 ) ) ;
#20351=CARTESIAN_POINT ( 'NONE',  ( -14.77829941377254563, 121.3346631531286164, 0.7297537739211615859 ) ) ;
#20352=CARTESIAN_POINT ( 'NONE',  ( -5.959810334499720419, 155.3892724211786742, -0.1190911940436165245 ) ) ;
#20353=CARTESIAN_POINT ( 'NONE',  ( 10.82992898448777730, 157.9016520041087688, 0.2364045824791625727 ) ) ;
#20355=CARTESIAN_POINT ( 'NONE',  ( -2.646443841375008432, -8.127818987380491578, -3.789199236247322133 ) ) ;
#20357=CARTESIAN_POINT ( 'NONE',  ( -23.36005780523123576, 148.8745345081378559, -0.4925575130201674812 ) ) ;
#20362=CARTESIAN_POINT ( 'NONE',  ( -4.680895062149801333, 118.8338629270736675, 0.8901742599232486119 ) ) ;
#20364=CARTESIAN_POINT ( 'NONE',  ( 0.3254831797250597458, 1.427361272777448509, 4.610396533461925905 ) ) ;
#20365=CARTESIAN_POINT ( 'NONE',  ( 21.58117366275196503, 150.4657531037631486, 1.865176240683389830 ) ) ;
#20368=CARTESIAN_POINT ( 'NONE',  ( 4.979196860906016653, 118.3881331334009985, -0.8414419690753369707 ) ) ;
#20369=CARTESIAN_POINT ( 'NONE',  ( -0.6580430243309095539, -8.493043821084315326, 4.585212396833119541 ) ) ;
#20370=CARTESIAN_POINT ( 'NONE',  ( -0.3562832388057288191, 117.2097358735305050, -0.4069867078728326426 ) ) ;
#20373=CARTESIAN_POINT ( 'NONE',  ( -15.83367336760682242, 146.2622375132148989, 0.01472612784998108409 ) ) ;
#20374=CARTESIAN_POINT ( 'NONE',  ( 5.498554953534677381, -14.76196523188227872, 3.265392988355040327 ) ) ;
#20378=CARTESIAN_POINT ( 'NONE',  ( 18.75244783997680642, 140.8526363637247982, 2.516729932275435289 ) ) ;
#20379=LINE ( 'NONE', #30400, #37291 ) ;
#20380=DIRECTION ( 'NONE',  ( 0.9998004120163608288, 0.000000000000000000, 0.01997839162482749342 ) ) ;
#20381=CARTESIAN_POINT ( 'NONE',  ( -22.55594873278735690, 149.0203452686010337, 0.8552431815872720833 ) ) ;
#20382=CARTESIAN_POINT ( 'NONE',  ( 5.057590804293729647, 14.82039226405042243, -6.742867120243351664 ) ) ;
#20383=CARTESIAN_POINT ( 'NONE',  ( 1.480437121830054492, 120.3785564700922492, 0.4209679054048331426 ) ) ;
#20386=CARTESIAN_POINT ( 'NONE',  ( 23.19190728264271684, 146.6831645211815101, -0.2733909575703941663 ) ) ;
#20393=CARTESIAN_POINT ( 'NONE',  ( -4.373713130305017849, 118.1839426225389929, 0.4384037898859596272 ) ) ;
#20394=CARTESIAN_POINT ( 'NONE',  ( 0.1058213901577373939, 105.9761915687788729, -5.295735085525933528 ) ) ;
#20395=ADVANCED_FACE ( 'NONE', ( #28214 ), #31189, .F. ) ;
#20398=CARTESIAN_POINT ( 'NONE',  ( -8.321911373758148045, 119.8826751762191947, -1.444119111808247036 ) ) ;
#20399=CARTESIAN_POINT ( 'NONE',  ( -5.752478121743209272, 118.4424948052634647, -0.6632437998952303015 ) ) ;
#20400=CARTESIAN_POINT ( 'NONE',  ( 4.592985736287271692, 118.0632451551486639, 0.7326753542377543171 ) ) ;
#20401=CARTESIAN_POINT ( 'NONE',  ( -13.94748453383795983, 150.2679186505038160, -1.219128122479325338 ) ) ;
#20402=CARTESIAN_POINT ( 'NONE',  ( -0.6559789189618892014, 115.7031633261756127, -1.758493996336355059 ) ) ;
#20403=CARTESIAN_POINT ( 'NONE',  ( 2.608821018174404927, 117.3993834728566270, -1.321848261876171327 ) ) ;
#20404=CARTESIAN_POINT ( 'NONE',  ( 5.270289556066540371, 116.2365830367532595, -0.9655167061512665017 ) ) ;
#20405=CARTESIAN_POINT ( 'NONE',  ( -16.63795227869236015, 147.2809512400332608, -1.774228895505126413 ) ) ;
#20406=CARTESIAN_POINT ( 'NONE',  ( -5.247413993112555630, 104.6144662015457385, -1.481417380683311968 ) ) ;
#20408=DIRECTION ( 'NONE',  ( -0.9998004120163608288, 0.000000000000000000, -0.01997839162482749342 ) ) ;
#20409=CARTESIAN_POINT ( 'NONE',  ( -0.6434349170078753621, 156.3034662015460583, 0.09435672052066400306 ) ) ;
#20411=CARTESIAN_POINT ( 'NONE',  ( 4.560443946511397506, -11.68866997254031936, 0.6947937310338139216 ) ) ;
#20412=CARTESIAN_POINT ( 'NONE',  ( 15.61264994714010079, 121.4606353739761744, 1.010464550865948663 ) ) ;
#20414=CARTESIAN_POINT ( 'NONE',  ( 3.405374690515594605, -14.89039384781155917, 1.812165507210882209 ) ) ;
#20415=AXIS2_PLACEMENT_3D ( 'NONE', #31396, #9656, #3921 ) ;
#20416=CARTESIAN_POINT ( 'NONE',  ( -4.259301615573863664, 119.5670751559891585, 0.7808790134437381125 ) ) ;
#20417=CARTESIAN_POINT ( 'NONE',  ( 0.9474642044963531573, -6.343762114497205395, -0.2236011429025598352 ) ) ;
#20418=CARTESIAN_POINT ( 'NONE',  ( -23.10841651933913354, 148.9583646262859133, -1.191549328111825456 ) ) ;
#20420=CARTESIAN_POINT ( 'NONE',  ( -0.7486558104752240039, 25.82057725623272759, -0.6268360674696834556 ) ) ;
#20423=CARTESIAN_POINT ( 'NONE',  ( 5.433204070470799785, 117.5340897209903517, 0.8253704096831886439 ) ) ;
#20424=PRODUCT_CONTEXT ( 'NONE', #24331, 'mechanical' ) ;
#20425=CARTESIAN_POINT ( 'NONE',  ( -2.723409340394791212, 120.7183352303693340, 0.2545450062501627420 ) ) ;
#20426=CARTESIAN_POINT ( 'NONE',  ( 2.708195657389492084, -14.88772387794683105, 5.660366118324242635 ) ) ;
#20427=CARTESIAN_POINT ( 'NONE',  ( 16.99563481483657412, 148.6336825499269310, -1.463981761124605985 ) ) ;
#20429=CARTESIAN_POINT ( 'NONE',  ( -12.70837813489441359, 122.8260676081006153, -1.843161107213562966 ) ) ;
#20430=CARTESIAN_POINT ( 'NONE',  ( 4.831188463146562917, 104.6144662015457527, 0.2218974365694108553 ) ) ;
#20431=CARTESIAN_POINT ( 'NONE',  ( 3.198224922426783579, -14.19254063666773291, 2.189163805996276579 ) ) ;
#20432=CARTESIAN_POINT ( 'NONE',  ( -4.932018240231780482, 117.5375708271148767, -1.014072823415046454 ) ) ;
#20433=CARTESIAN_POINT ( 'NONE',  ( 7.821695933845084880, 154.6216606121152495, -0.03501689623823063535 ) ) ;
#20434=VERTEX_POINT ( 'NONE', #32040 ) ;
#20436=DIRECTION ( 'NONE',  ( 4.017660918040594346E-17, -1.000000000000000000, -2.376309959284834438E-19 ) ) ;
#20438=CARTESIAN_POINT ( 'NONE',  ( -11.74288454345109756, 118.7273140689154616, -0.2346507796901759757 ) ) ;
#20441=CARTESIAN_POINT ( 'NONE',  ( 16.13169674176108970, 121.3783152868344075, 0.08747489889995967161 ) ) ;
#20444=CARTESIAN_POINT ( 'NONE',  ( 2.066596093631920983, -15.63843245996494957, 5.503614811026269038 ) ) ;
#20445=CARTESIAN_POINT ( 'NONE',  ( 5.035933200060415338, 117.3993844219003648, -0.5513780243448201945 ) ) ;
#20446=CARTESIAN_POINT ( 'NONE',  ( 0.7352267002175607580, 35.04949881550903967, -0.1714435552774139504 ) ) ;
#20447=CARTESIAN_POINT ( 'NONE',  ( 13.02489573621943286, 155.4510764517707742, 2.156236249524808635 ) ) ;
#20449=CARTESIAN_POINT ( 'NONE',  ( -3.861838729977780993, 14.11015702457025078, 7.483763204152318771 ) ) ;
#20450=CARTESIAN_POINT ( 'NONE',  ( 8.638409582537143194, 118.5547056413952873, -0.7669449099685430316 ) ) ;
#20451=CARTESIAN_POINT ( 'NONE',  ( -0.7907262360441658089, 106.8474934270474392, -4.937153267606968932 ) ) ;
#20453=CARTESIAN_POINT ( 'NONE',  ( -1.569970522942491176, 106.5487815437991515, -5.038282329708090757 ) ) ;
#20454=FACE_OUTER_BOUND ( 'NONE', #14710, .T. ) ;
#20455=CARTESIAN_POINT ( 'NONE',  ( 2.229080734463354307, 9.364070591990056869, -4.050418370856919914 ) ) ;
#20457=CARTESIAN_POINT ( 'NONE',  ( -4.829921688775540289, 118.5264896598256854, 0.7637249497284026578 ) ) ;
#20458=CARTESIAN_POINT ( 'NONE',  ( 3.036083976128487016, -13.30543680819082297, 1.158518541688273729 ) ) ;
#20459=CARTESIAN_POINT ( 'NONE',  ( 1.638321535317228239, 108.1711930243730109, -4.327427591587794886 ) ) ;
#20460=CARTESIAN_POINT ( 'NONE',  ( -22.74771312706173276, 149.7444054411783441, 0.5134062617908414783 ) ) ;
#20461=CARTESIAN_POINT ( 'NONE',  ( -3.521685918548247418, 29.33394459973516888, 3.031038535435704340 ) ) ;
#20463=ORIENTED_EDGE ( 'NONE', *, *, #30257, .T. ) ;
#20464=CARTESIAN_POINT ( 'NONE',  ( -2.362993923122841178, 104.6144662015455111, -4.208660904431277494 ) ) ;
#20465=CARTESIAN_POINT ( 'NONE',  ( 4.689621780486535663, -15.62538141832135707, 3.172200491054990579 ) ) ;
#20466=CARTESIAN_POINT ( 'NONE',  ( -20.46656357041398877, 147.8414448467482600, 1.666390110339677877 ) ) ;
#20469=CARTESIAN_POINT ( 'NONE',  ( 0.8139239711521952803, 26.85569158835278003, 0.5393279072465841928 ) ) ;
#20470=ORIENTED_EDGE ( 'NONE', *, *, #41179, .T. ) ;
#20472=CARTESIAN_POINT ( 'NONE',  ( 0.2949767777649464628, 114.7739974199301116, 2.049407731665748855 ) ) ;
#20473=B_SPLINE_SURFACE_WITH_KNOTS ( 'NONE', 1, 3, ( 
 ( #40844, #11646, #18233, #5282, #24630, #15042 ),
 ( #21422, #21632, #34450, #9096, #31235, #28259 ) ),
 .UNSPECIFIED., .F., .F., .F.,
 ( 2, 2 ),
 ( 4, 2, 4 ),
 ( 0.000000000000000000, 1.000000000000000000 ),
 ( 0.000000000000000000, 0.5000000000000000000, 1.000000000000000000 ),
 .UNSPECIFIED. ) ;
#20474=CARTESIAN_POINT ( 'NONE',  ( -10.33346200648618840, 123.4707319107414492, 0.9080611472405732965 ) ) ;
#20475=CARTESIAN_POINT ( 'NONE',  ( -4.974001918040873882, 117.3966124607983659, -0.9751453929904890794 ) ) ;
#20476=CARTESIAN_POINT ( 'NONE',  ( 4.045847121365343746, 157.1622345443605582, -1.633529996401409612 ) ) ;
#20478=CARTESIAN_POINT ( 'NONE',  ( -20.59518377851929571, 148.5655811199389689, -2.440016074255365819 ) ) ;
#20479=CARTESIAN_POINT ( 'NONE',  ( 5.332935397695203861, 104.6144662015457243, 0.1065647409268305201 ) ) ;
#20480=CARTESIAN_POINT ( 'NONE',  ( 4.319275104837216439, 118.2117203735061395, -0.3219079343282689187 ) ) ;
#20481=CARTESIAN_POINT ( 'NONE',  ( 4.503927054024090992, 120.9948550335633115, -0.2290337153283756866 ) ) ;
#20483=CARTESIAN_POINT ( 'NONE',  ( 3.263309282894114371, -14.66069363451780205, 2.445366243406764006 ) ) ;
#20486=CARTESIAN_POINT ( 'NONE',  ( 1.368391094521330897, 11.37271669962338372, 4.434453701053673313 ) ) ;
#20487=CARTESIAN_POINT ( 'NONE',  ( 17.20807765352988028, 147.1820577694790018, 2.053081559533530331 ) ) ;
#20488=CARTESIAN_POINT ( 'NONE',  ( -0.1611612690460884623, 32.88059107141324944, 1.736765093886240008 ) ) ;
#20490=CARTESIAN_POINT ( 'NONE',  ( -3.234384296441582762, 11.31316835407710819, -3.315160845070126427 ) ) ;
#20491=CARTESIAN_POINT ( 'NONE',  ( 14.67383990354511702, 148.8475317811793559, 0.3438330757172307628 ) ) ;
#20492=CARTESIAN_POINT ( 'NONE',  ( -5.274544067074300457, 115.7029491485454002, 0.8135768287290441325 ) ) ;
#20494=CARTESIAN_POINT ( 'NONE',  ( -5.555076865044160428, 116.7283850868982711, -0.3026861340469938488 ) ) ;
#20501=CARTESIAN_POINT ( 'NONE',  ( 7.354229849910361771, -2.730604093522916109, 4.103208822889532925 ) ) ;
#20502=DIRECTION ( 'NONE',  ( -0.9998004120163608288, 0.000000000000000000, -0.01997839162482747608 ) ) ;
#20506=CARTESIAN_POINT ( 'NONE',  ( -15.31729018078755722, 120.6995131204970875, 0.01165691202436099257 ) ) ;
#20507=EDGE_LOOP ( 'NONE', ( #30535, #34084, #39458, #8985 ) ) ;
#20512=CARTESIAN_POINT ( 'NONE',  ( -15.78392762965212448, 146.2390805666957192, -0.3668625800963856709 ) ) ;
#20513=CARTESIAN_POINT ( 'NONE',  ( 2.292478802652971659, -15.50831694688660534, 5.896745190559482985 ) ) ;
#20514=CARTESIAN_POINT ( 'NONE',  ( -3.107221341096740197, 117.9340107969418341, 0.6831876054667452847 ) ) ;
#20515=CARTESIAN_POINT ( 'NONE',  ( -4.191205975170537279, 21.45845178295031630, -1.961646697876042511 ) ) ;
#20516=CARTESIAN_POINT ( 'NONE',  ( 21.37844900359467815, 132.5159896776619917, 0.8378797052005131363 ) ) ;
#20517=CARTESIAN_POINT ( 'NONE',  ( 2.050826208811672657, -15.68011782295399037, 5.762527612234801921 ) ) ;
#20519=CARTESIAN_POINT ( 'NONE',  ( 0.1793159252905947298, -3.154364953387045034, 0.9593126492898319535 ) ) ;
#20520=CARTESIAN_POINT ( 'NONE',  ( -3.280774808778091245, 159.4678586119998442, -0.2050961497903012465 ) ) ;
#20521=DIRECTION ( 'NONE',  ( -5.206863593109713661E-17, 1.000000000000000000, -1.077750396879097183E-30 ) ) ;
#20523=CARTESIAN_POINT ( 'NONE',  ( 5.533816750157554587, 116.9218703105320429, 0.5587418741630174601 ) ) ;
#20524=CARTESIAN_POINT ( 'NONE',  ( -5.414978495245632573, 156.5090806470891209, 1.537019876316040090 ) ) ;
#20526=CARTESIAN_POINT ( 'NONE',  ( 6.794677088231689588, 118.4250403807481575, 1.128628347181275915 ) ) ;
#20527=CARTESIAN_POINT ( 'NONE',  ( 13.71253074539970562, 123.6869008171703541, -1.368039988124472695 ) ) ;
#20528=B_SPLINE_CURVE_WITH_KNOTS ( 'NONE', 3,
 ( #6232, #31789, #13242, #19203, #35833, #32211, #35204, #6649, #26014, #3044, #16002, #25803, #38405, #9622, #22590, #29211, #3459, #35622, #6436, #19410, #32417, #3247, #16422, #38188 ),
 .UNSPECIFIED., .F., .F.,
 ( 4, 2, 2, 2, 2, 2, 2, 2, 2, 2, 2, 4 ),
 ( 0.0005723024039399593997, 0.003660507319800902683, 0.006748712235661846401, 0.008292814693592298961, 0.009064865922557507893, 0.009836917151522718561, 0.01060896838048792923, 0.01138101960945313816, 0.01215307083841834883, 0.01253909645290095763, 0.01273210926014226724, 0.01292512206738357684 ),
 .UNSPECIFIED. ) ;
#20529=CARTESIAN_POINT ( 'NONE',  ( 0.7131539557513479899, -7.844638678481905103, 0.6656887750258669856 ) ) ;
#20530=CARTESIAN_POINT ( 'NONE',  ( -15.28824200187838755, 154.8698957928756954, -2.015933685939941267 ) ) ;
#20533=CARTESIAN_POINT ( 'NONE',  ( 15.97699994813249091, 148.2453349897154737, -0.9478121846735142464 ) ) ;
#20534=CARTESIAN_POINT ( 'NONE',  ( 7.846913280328204010, 122.2669436912714929, 0.7513606219076406356 ) ) ;
#20535=VERTEX_POINT ( 'NONE', #35883 ) ;
#20536=CARTESIAN_POINT ( 'NONE',  ( -16.38646240326728432, 135.1966315799913900, -2.295807278541857954 ) ) ;
#20537=CARTESIAN_POINT ( 'NONE',  ( 4.918313631922730522, -15.33159817589810281, -0.1794070962640156031 ) ) ;
#20539=CARTESIAN_POINT ( 'NONE',  ( -4.528805603826046244, 118.1086152786259333, -0.6811083559245456609 ) ) ;
#20542=CARTESIAN_POINT ( 'NONE',  ( 17.12878219156693760, 140.2562023718666353, 2.330665938063504417 ) ) ;
#20543=DIRECTION ( 'NONE',  ( -0.01997839162482749342, -1.040247600000944484E-18, 0.9998004120163608288 ) ) ;
#20545=CARTESIAN_POINT ( 'NONE',  ( 0.2937963077018297398, 116.4254261620736344, -0.006796306282692754844 ) ) ;
#20546=CARTESIAN_POINT ( 'NONE',  ( 8.109546976224176973, 7.201272144248561879, 2.403482862635152539 ) ) ;
#20547=CARTESIAN_POINT ( 'NONE',  ( 3.687801383043704639, 120.9852966486377710, 0.2688355818071224701 ) ) ;
#20548=CARTESIAN_POINT ( 'NONE',  ( 22.54293160324719381, 149.6594668941642681, -0.7271591872719224137 ) ) ;
#20550=CARTESIAN_POINT ( 'NONE',  ( -6.578476689077728991E-14, 85.18346620154574111, -5.002419396613184919E-18 ) ) ;
#20551=TOROIDAL_SURFACE ( 'NONE', #2234, 5.080000000000005400, 0.5080000000000000071 ) ;
#20553=CARTESIAN_POINT ( 'NONE',  ( -18.63219679753396107, 154.1293031355326946, -0.2996243416495529832 ) ) ;
#20554=ORIENTED_EDGE ( 'NONE', *, *, #41179, .F. ) ;
#20556=CARTESIAN_POINT ( 'NONE',  ( -6.814076468830258193, 121.3873156153395456, -0.8343114639089803664 ) ) ;
#20557=DIRECTION ( 'NONE',  ( 4.017660918040594346E-17, -1.000000000000000000, -2.376309959284832031E-19 ) ) ;
#20560=CARTESIAN_POINT ( 'NONE',  ( -14.79492108907976267, 148.8567844064068026, -0.8802232212986719206 ) ) ;
#20561=CARTESIAN_POINT ( 'NONE',  ( 3.942998349758990440, -14.41637075870405482, 4.944918514907367779 ) ) ;
#20562=CARTESIAN_POINT ( 'NONE',  ( -14.41840636618848670, 121.0470547900126519, 0.7241072410554124650 ) ) ;
#20564=CARTESIAN_POINT ( 'NONE',  ( 17.26848747421918873, 122.7565812399420651, 0.3979830900422688944 ) ) ;
#20567=CARTESIAN_POINT ( 'NONE',  ( -0.5496829067194369811, 0.7180641350488168317, -4.598301960397928489 ) ) ;
#20569=CARTESIAN_POINT ( 'NONE',  ( -20.50094783971104917, 129.0975500345852822, -0.4299227524276373891 ) ) ;
#20571=AXIS2_PLACEMENT_3D ( 'NONE', #11179, #27781, #24164 ) ;
#20574=CARTESIAN_POINT ( 'NONE',  ( 8.133763292779583765, 120.8066077149993163, 1.378299465333653107 ) ) ;
#20575=CARTESIAN_POINT ( 'NONE',  ( 4.471266627501615076, -5.469457446779734333, -1.220754042301255948 ) ) ;
#20576=CARTESIAN_POINT ( 'NONE',  ( 15.93415399606955951, 122.8751182158008959, 1.397711951582541801 ) ) ;
#20578=CARTESIAN_POINT ( 'NONE',  ( 18.49784594330472842, 151.8926627062091086, -1.576652458532300960 ) ) ;
#20579=CARTESIAN_POINT ( 'NONE',  ( -1.722957355399680202, -2.895624787512894649, -4.295268622497145472 ) ) ;
#20580=CARTESIAN_POINT ( 'NONE',  ( -1.323305960456944597, 159.4649289425152858, -0.7771481453362865111 ) ) ;
#20582=CARTESIAN_POINT ( 'NONE',  ( -11.18446751737367428, 128.1157469881088105, -0.03160020415517764830 ) ) ;
#20583=CARTESIAN_POINT ( 'NONE',  ( 5.915669078949217230, -14.48123931593440972, 2.327441804047190033 ) ) ;
#20587=CARTESIAN_POINT ( 'NONE',  ( 13.34589015847587135, 154.0568829568526041, 2.281985820853443592 ) ) ;
#20588=CARTESIAN_POINT ( 'NONE',  ( -6.606029807653651701E-14, 92.04146620154574521, -3.372746026535634231E-18 ) ) ;
#20589=DIRECTION ( 'NONE',  ( 0.01997839162482749689, 1.040247600000945640E-18, -0.9998004120163610509 ) ) ;
#20591=CARTESIAN_POINT ( 'NONE',  ( -11.13388036866237663, 119.2389763063149388, 0.6860836662663823970 ) ) ;
#20592=CARTESIAN_POINT ( 'NONE',  ( 2.488832714281139946, 5.747567886007050042, -8.044950587805361764 ) ) ;
#20593=EDGE_CURVE ( 'NONE', #28199, #40141, #9205, .T. ) ;
#20594=CARTESIAN_POINT ( 'NONE',  ( 6.473539731754311077, 155.4519854478747902, 1.179574399179393662 ) ) ;
#20595=CARTESIAN_POINT ( 'NONE',  ( -6.654617103318593247E-14, 104.6144662015457243, 1.534725424433578570E-31 ) ) ;
#20596=CARTESIAN_POINT ( 'NONE',  ( 22.15286039372319493, 136.9573810088325843, -0.3857095667871863753 ) ) ;
#20597=CARTESIAN_POINT ( 'NONE',  ( -3.174366308152013705, 104.6144662015457243, -0.06343139340882732180 ) ) ;
#20602=CARTESIAN_POINT ( 'NONE',  ( -4.424064652446513257, 118.1653673812831471, 0.4722651929950075766 ) ) ;
#20603=CARTESIAN_POINT ( 'NONE',  ( 0.6542085308957266143, 106.0197932915460228, -5.259646073629641094 ) ) ;
#20606=CARTESIAN_POINT ( 'NONE',  ( 8.380735907288704212, 119.8444783950307198, -1.107720622939692756 ) ) ;
#20607=CARTESIAN_POINT ( 'NONE',  ( -0.1506203121293892555, 105.8833743670705445, -5.338473058816376238 ) ) ;
#20609=CARTESIAN_POINT ( 'NONE',  ( 4.627536327950492634, 118.0321392792698560, 0.7764583414207147927 ) ) ;
#20610=CARTESIAN_POINT ( 'NONE',  ( -9.347632431636418104, 123.5785764018267514, -0.8560492856234916959 ) ) ;
#20611=CARTESIAN_POINT ( 'NONE',  ( -0.5151781122927419077, 115.7029491485453434, -1.762078896387328397 ) ) ;
#20613=EDGE_CURVE ( 'NONE', #11942, #24980, #25088, .T. ) ;
#20614=CARTESIAN_POINT ( 'NONE',  ( -4.507778648822867495, 31.37953541088120346, -1.025544427737863362 ) ) ;
#20615=CARTESIAN_POINT ( 'NONE',  ( -10.24488040547501733, 123.7737839053064022, -1.229789271442949472 ) ) ;
#20619=CARTESIAN_POINT ( 'NONE',  ( 7.903630729593992932, 122.1168884809556232, -0.5501188935066759766 ) ) ;
#20620=CARTESIAN_POINT ( 'NONE',  ( -11.72060482218064337, 130.2300814166513305, -0.06371650795576043469 ) ) ;
#20621=DIRECTION ( 'NONE',  ( 4.017660918040594346E-17, -1.000000000000000000, -2.376309959284834438E-19 ) ) ;
#20622=CARTESIAN_POINT ( 'NONE',  ( 1.940752395788238660, 116.9162416783649689, 0.4172132017389483805 ) ) ;
#20623=CARTESIAN_POINT ( 'NONE',  ( -4.808149584360944750, 104.6144662015457243, 0.4147572885131461939 ) ) ;
#20624=CARTESIAN_POINT ( 'NONE',  ( 3.348477204222540138, -14.79883842983281639, 1.177367440313774605 ) ) ;
#20625=CARTESIAN_POINT ( 'NONE',  ( -7.522503210159361409, 120.3045338523282197, 1.038419263833407546 ) ) ;
#20626=CARTESIAN_POINT ( 'NONE',  ( -0.9136164112762927836, -2.447138680932527066, -0.3421040304710446511 ) ) ;
#20627=CARTESIAN_POINT ( 'NONE',  ( -22.36400590086645579, 150.5530013069706285, -1.293239838729947078 ) ) ;
#20629=CARTESIAN_POINT ( 'NONE',  ( -0.2091969695887432312, -7.904008462454454431, -0.9542532860826526964 ) ) ;
#20631=EDGE_CURVE ( 'NONE', #23570, #27974, #4141, .T. ) ;
#20633=CARTESIAN_POINT ( 'NONE',  ( 6.891280466594640330, 121.8252198949890186, 0.2939903263561804425 ) ) ;
#20634=CARTESIAN_POINT ( 'NONE',  ( -16.05525886874805863, 145.8417561620165372, 0.5351738620951718151 ) ) ;
#20635=CARTESIAN_POINT ( 'NONE',  ( 2.601617458372238900, -15.08031326607275879, 5.801161347629554044 ) ) ;
#20636=CARTESIAN_POINT ( 'NONE',  ( 16.16280394421523070, 139.8573806175465961, -1.392748567604541687 ) ) ;
#20638=CARTESIAN_POINT ( 'NONE',  ( -12.10717961583478441, 122.5392882283422864, -1.794329550371803972 ) ) ;
#20639=CARTESIAN_POINT ( 'NONE',  ( 3.600447276656479900, 115.7029491485453150, 1.622454299057154881 ) ) ;
#20640=CARTESIAN_POINT ( 'NONE',  ( 2.491201389814710065, -14.86453887000410745, 4.964479704013470496 ) ) ;
#20641=CARTESIAN_POINT ( 'NONE',  ( -4.947191892140043734, 117.5302764761379990, -0.9660299176223910989 ) ) ;
#20642=CARTESIAN_POINT ( 'NONE',  ( 5.280870373041073762, 121.3253820001177417, -0.01155303659100754415 ) ) ;
#20645=CARTESIAN_POINT ( 'NONE',  ( 6.532233579562727321, 157.6773268839678508, 1.915660460402585752 ) ) ;
#20646=DIRECTION ( 'NONE',  ( -0.9998004120163608288, 0.000000000000000000, -0.01997839162482747608 ) ) ;
#20651=CARTESIAN_POINT ( 'NONE',  ( 5.733252156539616173, 159.1225378944267845, -0.03759195597257673077 ) ) ;
#20652=EDGE_CURVE ( 'NONE', #1790, #3203, #6480, .T. ) ;
#20655=EDGE_CURVE ( 'NONE', #15693, #24814, #7413, .T. ) ;
#20656=CARTESIAN_POINT ( 'NONE',  ( 1.793193054604032222, -15.65090912328376227, 5.542963820967112376 ) ) ;
#20659=CARTESIAN_POINT ( 'NONE',  ( 19.59170213216421175, 150.6586468064772646, 2.354958926090490845 ) ) ;
#20660=ORIENTED_EDGE ( 'NONE', *, *, #20697, .F. ) ;
#20661=CARTESIAN_POINT ( 'NONE',  ( -2.821688713678647709, 20.15627898171042176, -7.936949992814660071 ) ) ;
#20662=CARTESIAN_POINT ( 'NONE',  ( -2.408872516888110216, 117.3686073472606921, -0.7136685935690528781 ) ) ;
#20663=CARTESIAN_POINT ( 'NONE',  ( -2.259516459295737079, 118.2243428780609662, -0.9293431707136510234 ) ) ;
#20665=AXIS2_PLACEMENT_3D ( 'NONE', #12738, #32128, #35751 ) ;
#20668=CARTESIAN_POINT ( 'NONE',  ( -0.01254005783143666460, 120.1716774721351157, 0.6275557724548824767 ) ) ;
#20669=CARTESIAN_POINT ( 'NONE',  ( 2.551540157903699146, -0.3564265548712530207, -3.854280124997286450 ) ) ;
#20672=CARTESIAN_POINT ( 'NONE',  ( 3.381076509412870301, -13.31623885458479961, 2.121725202727857695 ) ) ;
#20673=CARTESIAN_POINT ( 'NONE',  ( 5.132724724882859135, 121.7269124416356192, -0.09984968675566523177 ) ) ;
#20674=CARTESIAN_POINT ( 'NONE',  ( -8.141728797601244239, 117.8329967196738153, 0.4384511054415166087 ) ) ;
#20675=EDGE_CURVE ( 'NONE', #23570, #12906, #31517, .T. ) ;
#20676=CARTESIAN_POINT ( 'NONE',  ( -2.501798531443050422, 32.04972782698715861, 4.390535724770350257 ) ) ;
#20678=EDGE_LOOP ( 'NONE', ( #31232, #21232, #11573, #2656 ) ) ;
#20679=CARTESIAN_POINT ( 'NONE',  ( -4.842539706364327401, 104.6144662015370272, -2.263382849314995671 ) ) ;
#20681=CARTESIAN_POINT ( 'NONE',  ( 4.270102617218862306, -15.70017440876955739, 3.434341872514240723 ) ) ;
#20682=CARTESIAN_POINT ( 'NONE',  ( -14.84283187390168379, 125.6006210965460781, 1.448481940162723358 ) ) ;
#20683=CARTESIAN_POINT ( 'NONE',  ( -2.070226828232369254, -8.352695179381779411, -4.151654383260235726 ) ) ;
#20685=VERTEX_POINT ( 'NONE', #529 ) ;
#20687=CARTESIAN_POINT ( 'NONE',  ( 3.074626428557167390, 123.1875568577169560, 0.1788317054798709282 ) ) ;
#20689=CARTESIAN_POINT ( 'NONE',  ( -11.70197428064591527, 126.1299551460304542, 0.9179571146301048756 ) ) ;
#20691=( BOUNDED_SURFACE ( )  B_SPLINE_SURFACE ( 3, 3, ( 
 ( #23933, #7770, #26511, #20733, #16702, #33757, #7145, #1173, #39943, #3956, #14136, #966, #4583, #30543, #29917, #756, #20307, #20102, #26725, #27138, #40362, #549, #33126, #10532, #10735, #23501, #36528, #26931, #33333, #4163, #31597, #11365, #41190, #5000, #34172, #14552, #27971, #15394, #12212, #28400, #2433, #41405, #24773, #21559, #27762, #25202, #21143, #21350, #34587, #17958, #18371, #2007, #40981, #24988, #11570, #34375, #37560, #40772, #30958, #24556, #5416, #38206, #1798, #8812, #18163, #28185, #31166, #37988, #37771, #11993, #21986, #14761, #9023, #4794, #34797, #8386, #40567, #11783, #5630, #17745, #8176, #5208, #24351, #27560, #14969, #30745, #8595, #31378, #2222, #21771, #15182, #18588, #1595, #37357, #32229, #71, #25418, #26241, #28608, #3060, #41617, #12426, #26030, #3263, #38419, #38626, #39039, #10057, #13257, #19426, #39250, #18793, #5840, #16017, #35019, #22398, #31806, #9846, #29445, #3479, #2643, #28818, #15603, #29016, #9231, #35422, #22189, #22814, #284, #16438, #35219, #41833, #6045, #19007, #32011, #32432, #2850, #15811, #16223, #13040, #12627, #35851, #25615, #29230, #9428, #6665, #42036, #6249, #38828, #19218, #19628, #32643, #12832, #25819, #9638, #22606, #35638, #6453, #33496, #17492, #1120, #17290, #17074, #30488, #32858, #33284, #39888, #27090, #7719, #29658, #30279, #23237, #10265, #3690, #4114, #33707, #1331, #4528, #20683, #14289, #913, #10685, #3904, #27299, #39463, #39677, #23666, #36272, #36686, #20257, #30076, #14089, #29868, #10480, #13678, #16867, #7092, #707 ),
 ( #36477, #40098, #13887, #4326, #40313, #33073, #23028, #36058, #10894, #20054, #16651, #26880, #23882, #6872, #26459, #26669, #498, #13471, #23449, #19845, #7297, #7508, #20469, #36901, #4947, #31326, #7923, #4741, #8334, #18323, #1543, #2383, #17694, #21304, #30694, #14498, #2170, #21509, #27513, #14709, #15128, #28348, #31539, #37726, #15343, #37105, #40521, #24722, #34333, #5161, #28131, #17907, #40722, #1750, #34121, #11312, #30911, #27921, #18534, #24299, #41141, #24503, #34543, #37509, #11947, #31120, #5369, #11107, #21096, #24096, #37936, #24938, #37305, #8122, #18116, #8761, #21721, #27713, #11518, #1957, #20889, #14917, #33913, #40928, #11733, #8550, #34746, #5578, #19374, #38155, #34965, #38570, #6405, #31754, #32589, #5788, #9382, #18743, #2596, #32380, #9588, #15556, #2802, #3211, #16389, #19581, #25770, #3422, #25153, #12160, #22346, #41357, #28765, #8969, #16171, #35798, #9799, #21936, #35168, #28558, #41567, #12376, #38777, #22766, #25363, #22558, #29176, #38367, #22, #6612, #35588, #9181, #12988, #35369, #22138, #3008, #41778, #25982, #38990, #5995, #18957, #31963, #15762, #12578, #6199, #25565, #19170, #32174, #15967, #28965, #41982, #12780, #39626, #4067, #33447, #14040, #36007, #23619, #29612, #16604, #39198, #10432, #40053, #36853, #10846, #27045, #23832, #7252, #17026, #10214, #7671, #3640, #3854, #30024, #20008, #33658, #20629, #22978, #865, #4483, #29395, #29821, #20212, #235, #33238, #659, #13211, #13838, #26193, #6819, #447, #26618, #10006, #19789, #32809, #26835, #39842, #13419 ),
 ( #23402, #26407, #33025, #39411, #23184, #10639, #36639, #36433, #13627, #7461, #20420, #4275, #17238, #30233, #16819, #36220, #1072, #7041, #5114, #15080, #17860, #40676, #34489, #34695, #27251, #11266, #17650, #11468, #31069, #30860, #2117, #1706, #24670, #8501, #21052, #20841, #11683, #37679, #8079, #40267, #8710, #14453, #28081, #5320, #14660, #34286, #18272, #14871, #37060, #41092, #30652, #17443, #21458, #27464, #40475, #27664, #11899, #33866, #24888, #7878, #1286, #37885, #14244, #21672, #40882, #27873, #30441, #11062, #8286, #24457, #31274, #24046, #18067, #4695, #34078, #24252, #1496, #37260, #37461, #4905, #21256, #1908, #6940, #19487, #5742, #9906, #10121, #25309, #18694, #28508, #15292, #3324, #3545, #23092, #13535, #32496, #16291, #41304, #13319, #29295, #138, #29513, #26305, #39314, #13105, #26097, #9134, #12109, #39103, #12322, #35916, #3757, #6512, #22878, #36126, #23303, #28297, #41516, #31704, #6726, #19694, #32711, #32927, #16506, #19911, #16715, #22668, #8917, #352, #29718, #38315, #25099, #39529, #2546, #560, #26523, #10333, #5525, #18482, #31488, #38102, #2333, #15507, #21883, #34910, #35701, #36539, #39953, #27358, #26736, #30552, #766, #7156, #1391, #20115, #11166, #40161, #27149, #37159, #40370, #20529, #13944, #10954, #23941, #4392, #24150, #17136, #20317, #10543, #23512, #33558, #33344, #7358, #36958, #4592, #26942, #4174, #17348, #7781, #30138, #979, #10747, #33137, #23728, #20742, #33767, #36341, #7568, #36747, #39745, #30336, #3967, #16928, #1183, #17551, #29928, #13742, #14146 ),
 ( #14347, #10243, #39654, #13448, #38805, #16631, #13237, #19405, #36035, #32621, #23214, #20032, #3242, #32412, #22793, #9617, #16201, #39225, #475, #26646, #36247, #26436, #684, #23428, #39440, #7068, #28996, #33051, #10458, #3881, #22585, #29638, #26221, #29206, #6850, #3454, #16846, #29846, #49, #13015, #35828, #35617, #26009, #10035, #13656, #36457, #7276, #32206, #23007, #3039, #42013, #263, #19819, #15997, #12809, #6431, #25799, #39018, #9826, #6644, #32836, #19608, #16416, #29422, #3665, #3713, #17309, #7113, #13493, #36496, #26898, #26693, #40118, #39700, #20486, #4347, #16885, #16672, #7525, #33513, #3925, #36082, #4551, #10289, #10912, #1141, #13699, #30095, #30298, #10704, #32881, #23901, #26479, #13277, #14107, #23259, #36294, #10500, #7736, #29677, #36918, #520, #39271, #20702, #10077, #17511, #36704, #23683, #30508, #33728, #4133, #23470, #27106, #26261, #936, #23048, #29886, #20072, #39483, #33094, #33303, #724, #7316, #6896, #19866, #20276, #17092, #13906, #39910, #21115, #14522, #24322, #11126, #40743, #40950, #5389, #8785, #27732, #14730, #37121, #34141, #5602, #11967, #7943, #1978, #41161, #37960, #1770, #21322, #14306, #31139, #17715, #14940, #11540, #37529, #21530, #8144, #30931, #4968, #37328, #30714, #17926, #18134, #21743, #1566, #18344, #24524, #24743, #8354, #34562, #34350, #37745, #18557, #11334, #34769, #28155, #31350, #27532, #20912, #5182, #2193, #24959, #4763, #40539, #33935, #24113, #27942, #1349, #11755, #8569, #15151, #27319, #40332, #10179, #28370, #25176, #28789, #39377 ),
 ( #23148, #413, #38177, #35190, #36187, #7218, #10396, #16568, #23368, #15364, #2404, #41801, #36401, #18980, #31563, #7006, #26582, #624, #41377, #25387, #18766, #12183, #8991, #29578, #13593, #21959, #13382, #19975, #34989, #32991, #39592, #26369, #5810, #3819, #12599, #31775, #35390, #31984, #16782, #29785, #2616, #15576, #22160, #28581, #41589, #38593, #12397, #38390, #9201, #6016, #25586, #2822, #15781, #9401, #6784, #22365, #19752, #32774, #3604, #20382, #7424, #29987, #1254, #30823, #27627, #1669, #37224, #8043, #30199, #14209, #1039, #14624, #36605, #36815, #4239, #40639, #11433, #33408, #17825, #27216, #16987, #23794, #37426, #17201, #30615, #27424, #30405, #4451, #1458, #40437, #11228, #40230, #17409, #7634, #26800, #33622, #27010, #7841, #24421, #20592, #24214, #4029, #10602, #21016, #14004, #40019, #11025, #33830, #24006, #4867, #37026, #34039, #20179, #20804, #23582, #14417, #33203, #10813, #827, #13802, #4658, #39809, #17614, #8673, #25061, #25276, #5707, #27838, #5914, #8469, #8247, #28477, #5285, #18235, #34660, #2721, #24633, #18876, #40846, #34249, #31885, #5079, #41691, #31670, #18664, #25493, #15678, #41269, #21634, #2511, #15475, #38065, #28682, #41055, #31237, #21424, #34452, #28261, #15044, #2080, #41481, #9099, #5488, #28046, #12074, #12289, #11865, #24854, #37851, #18029, #18448, #38281, #22065, #12501, #31454, #2298, #1872, #15258, #21219, #31031, #14834, #8882, #11648, #37643, #21846, #34874, #35091, #29316, #9721, #23109, #158, #29739, #2926, #38702, #35720, #16735, #35295, #6123 ),
 ( #9509, #6528, #580, #19088, #32091, #13128, #26118, #32948, #15888, #22478, #3777, #13552, #35506, #36145, #32515, #28892, #42118, #38490, #25696, #6745, #3564, #19504, #22686, #19713, #16525, #29534, #3346, #16312, #12911, #41906, #39121, #3132, #9927, #6960, #38909, #370, #22271, #12706, #13336, #32302, #6325, #22896, #35933, #32733, #19931, #26325, #39331, #10138, #25903, #19296, #9309, #16093, #29099, #7175, #17772, #23533, #24166, #14366, #26961, #1203, #1410, #23959, #3986, #37176, #26756, #26542, #4612, #36560, #7376, #10767, #20968, #784, #7999, #16946, #10352, #33990, #23324, #30770, #7798, #36977, #1619, #4818, #17366, #39974, #20760, #33784, #14163, #39549, #17156, #20336, #39766, #10560, #4409, #33361, #4194, #17567, #27376, #23747, #30156, #30355, #30570, #997, #13961, #36766, #36359, #7585, #40386, #11181, #20135, #20546, #33575, #33158, #27170, #29944, #13759, #40181, #10975, #12234, #9045, #14994, #34609, #27580, #5438, #27994, #41427, #18396, #17982, #8833, #21795, #5230, #37381, #5861, #11595, #25225, #2456, #41002, #31405, #31617, #12018, #34199, #38230, #14783, #14575, #34823, #24578, #37584, #11808, #22011, #30979, #35041, #5024, #40588, #18821, #11388, #31828, #38011, #25011, #24373, #8196, #2246, #24799, #5656, #18612, #15205, #21167, #18185, #8412, #27785, #40795, #28208, #21371, #34397, #15419, #28422, #37793, #31186, #41216, #1819, #2031, #8619, #21581, #12448, #42062, #98, #6688, #10080, #29044, #16042, #38441, #35449, #6900, #13280, #9256, #3288, #312, #39274, #3082, #22629 ),
 ( #22838, #23052, #26055, #22213, #29253, #25843, #32036, #6475, #12856, #35877, #32670, #15835, #2873, #6272, #35243, #28842, #9663, #13064, #36086, #19655, #39066, #38852, #19869, #25442, #35665, #19450, #3505, #29470, #6068, #9868, #41855, #12652, #19030, #32459, #26264, #2665, #15624, #16463, #28628, #25641, #16249, #38648, #41641, #9454, #19243, #22421, #32253, #4351, #30099, #26901, #4136, #40123, #23907, #36499, #36297, #27111, #10917, #23474, #13496, #24117, #29889, #30514, #20707, #33306, #7529, #7740, #30302, #10294, #1353, #33098, #32884, #36922, #727, #13704, #17096, #27325, #7118, #14312, #23262, #16676, #40336, #29680, #37126, #14112, #1144, #7947, #11130, #23688, #939, #33732, #4555, #20490, #3717, #7320, #26697, #3928, #16888, #10708, #39703, #10504, #17515, #523, #13909, #20279, #36707, #26482, #39914, #33516, #17312, #39487, #20075, #18349, #24964, #28376, #5186, #34354, #14527, #11544, #25181, #31570, #27536, #21536, #18563, #15370, #21327, #40955, #33939, #11760, #18139, #5607, #24749, #12188, #40543, #21119, #31143, #41383, #17719, #30720, #37749, #8573, #38182, #11340, #4973, #20916, #4767, #34147, #2409, #14944, #1570, #24528, #24326, #8148, #31354, #28161, #1983, #27946, #2198, #41165, #11971, #34566, #5393, #37535, #37332, #15156, #27737, #37964, #17932, #8789, #21747, #30935, #1774, #34774, #14735, #40747, #8359, #22582, #22372, #35825, #9207, #8999, #29202, #6022, #18985, #35397, #3450, #25395, #6641, #28586, #34995, #19605, #5815, #259, #32409, #19401, #26217, #16413, #42009, #9406 ) ),
 .UNSPECIFIED., .T., .F., .T. ) 
 B_SPLINE_SURFACE_WITH_KNOTS ( ( 4, 3, 4 ),
 ( 4, 1, 1, 1, 1, 1, 1, 1, 1, 1, 1, 1, 1, 1, 1, 1, 1, 1, 1, 1, 1, 1, 1, 1, 1, 1, 1, 1, 1, 1, 1, 1, 1, 1, 1, 1, 1, 1, 1, 1, 1, 1, 1, 1, 1, 1, 1, 1, 1, 1, 1, 1, 1, 1, 1, 1, 1, 1, 1, 1, 1, 1, 1, 1, 1, 1, 1, 1, 1, 1, 1, 1, 1, 1, 1, 1, 1, 1, 1, 1, 1, 1, 1, 1, 1, 1, 1, 1, 1, 1, 1, 1, 1, 1, 1, 1, 1, 1, 1, 1, 1, 1, 1, 1, 1, 1, 1, 1, 1, 1, 1, 1, 1, 1, 1, 1, 1, 1, 1, 1, 1, 1, 1, 1, 1, 1, 1, 1, 1, 1, 1, 1, 1, 1, 1, 1, 1, 1, 1, 1, 1, 1, 1, 1, 1, 1, 1, 1, 1, 1, 1, 1, 1, 1, 1, 1, 1, 1, 1, 1, 1, 1, 1, 1, 1, 1, 1, 1, 1, 1, 1, 1, 1, 1, 1, 1, 1, 1, 1, 1, 1, 1, 1, 1, 1, 1, 1, 1, 1, 1, 1, 1, 3, 4 ),
 ( 0.000000000000000000, 0.5000000000000000000, 1.000000000000000000 ),
 ( 0.000000000000000000, 0.007812500000000423273, 0.01388888888888889506, 0.01562500000000000000, 0.02343749999999998959, 0.02777777777777778317, 0.03125000000000092981, 0.03906249999999999306, 0.04166666666666667823, 0.04687500000000000000, 0.05468749999999999306, 0.05555555555555556635, 0.06249999999999997918, 0.06944444444444446141, 0.07031250000000000000, 0.07812500000000000000, 0.08333333333333334259, 0.08593749999999998612, 0.09374999999999603095, 0.09722222222222223764, 0.1015625000000000139, 0.1093750000000000000, 0.1111111111111111188, 0.1171875000000000000, 0.1250000000000000000, 0.1328125000000000000, 0.1388888888888889228, 0.1406250000000000000, 0.1484375000000000000, 0.1527777777777778179, 0.1562500000000039690, 0.1640625000000000000, 0.1666666666666666852, 0.1718750000000000000, 0.1796875000000000000, 0.1805555555555555802, 0.1875000000000000000, 0.1944444444444444753, 0.1953125000000000000, 0.2031250000000000000, 0.2083333333333333703, 0.2109375000000000000, 0.2187499999999960310, 0.2222222222222222376, 0.2265625000000000000, 0.2343750000000000000, 0.2361111111111111327, 0.2421875000000000000, 0.2500000000000000000, 0.2578125000000000000, 0.2638888888888888951, 0.2656250000000000000, 0.2734375000000000000, 0.2777777777777777346, 0.2812500000000039968, 0.2890625000000000000, 0.2916666666666665741, 0.2968750000000000000, 0.3046875000000000000, 0.3055555555555554692, 0.3125000000000000000, 0.3194444444444443088, 0.3203125000000000000, 0.3281250000000000000, 0.3333333333333332038, 0.3359375000000000000, 0.3437499999999960587, 0.3472222222222220434, 0.3515625000000000000, 0.3593750000000000000, 0.3611111111111109384, 0.3671875000000000000, 0.3750000000000000000, 0.3828125000000000000, 0.3888888888888886175, 0.3906250000000000000, 0.3984375000000000000, 0.4027777777777775126, 0.4062500000000039968, 0.4140625000000000000, 0.4166666666666663521, 0.4218750000000000000, 0.4296875000000000000, 0.4305555555555552472, 0.4375000000000000000, 0.4444444444444440867, 0.4453125000000000000, 0.4531250000000000000, 0.4583333333333329818, 0.4609375000000000000, 0.4687499999999960587, 0.4722222222222218768, 0.4765625000000000000, 0.4843750000000000000, 0.4861111111111107719, 0.4921875000000000000, 0.5000000000000000000, 0.5078125000000000000, 0.5138888888888886175, 0.5156250000000000000, 0.5234375000000000000, 0.5277777777777775681, 0.5312500000000039968, 0.5390625000000000000, 0.5416666666666664076, 0.5468750000000000000, 0.5546875000000000000, 0.5555555555555553582, 0.5625000000000000000, 0.5694444444444443088, 0.5703125000000000000, 0.5781250000000000000, 0.5833333333333331483, 0.5859375000000000000, 0.5937499999999960032, 0.5972222222222220989, 0.6015625000000000000, 0.6093750000000000000, 0.6111111111111110494, 0.6171875000000000000, 0.6250000000000000000, 0.6328125000000000000, 0.6388888888888888395, 0.6406250000000000000, 0.6484375000000000000, 0.6527777777777777901, 0.6562500000000039968, 0.6640625000000000000, 0.6666666666666666297, 0.6718750000000000000, 0.6796875000000000000, 0.6805555555555555802, 0.6875000000000000000, 0.6944444444444445308, 0.6953125000000000000, 0.7031250000000000000, 0.7083333333333333703, 0.7109375000000000000, 0.7187499999999960032, 0.7222222222222223209, 0.7265625000000000000, 0.7343750000000000000, 0.7361111111111111605, 0.7421875000000000000, 0.7500000000000000000, 0.7578125000000000000, 0.7638888888888889506, 0.7656250000000000000, 0.7734375000000000000, 0.7777777777777779011, 0.7812500000000039968, 0.7890625000000000000, 0.7916666666666668517, 0.7968750000000000000, 0.8046875000000000000, 0.8055555555555556912, 0.8125000000000000000, 0.8194444444444446418, 0.8203125000000000000, 0.8281250000000000000, 0.8333333333333335924, 0.8359375000000000000, 0.8437499999999960032, 0.8472222222222224319, 0.8515625000000000000, 0.8593750000000000000, 0.8611111111111113825, 0.8671875000000000000, 0.8750000000000000000, 0.8828125000000000000, 0.8888888888888891726, 0.8906250000000000000, 0.8984375000000000000, 0.9027777777777781232, 0.9062500000000039968, 0.9140625000000000000, 0.9166666666666670737, 0.9218750000000000000, 0.9296875000000000000, 0.9305555555555559133, 0.9375000000000000000, 0.9444444444444447528, 0.9453125000000000000, 0.9531250000000000000, 0.9583333333333335924, 0.9609375000000000000, 0.9687499999999991118, 0.9722222222222224319, 0.9765625000000000000, 0.9843750000000000000, 0.9861111111111111605, 0.9921874999999995559, 1.000000000000000000, 1.000012325855852646 ),
 .UNSPECIFIED. ) 
 GEOMETRIC_REPRESENTATION_ITEM ( )  RATIONAL_B_SPLINE_SURFACE ( (
 ( 1.000000000000000000, 1.000000000000000000, 1.000000000000000000, 1.000000000000000000, 1.000000000000000000, 1.000000000000000000, 0.9999999999999998890, 0.9999999999999997780, 1.000000000000000000, 1.000000000000000000, 1.000000000000000000, 1.000000000000000000, 1.000000000000000000, 1.000000000000000000, 0.9999999999999998890, 1.000000000000000000, 1.000000000000000222, 1.000000000000000000, 1.000000000000000000, 1.000000000000000000, 1.000000000000000000, 1.000000000000000000, 0.9999999999999998890, 0.9999999999999997780, 1.000000000000000000, 1.000000000000000222, 1.000000000000000000, 1.000000000000000000, 1.000000000000000000, 1.000000000000000000, 0.9999999999999998890, 0.9999999999999997780, 1.000000000000000000, 0.9999999999999998890, 0.9999999999999997780, 1.000000000000000000, 1.000000000000000222, 1.000000000000000222, 1.000000000000000000, 1.000000000000000000, 1.000000000000000222, 1.000000000000000000, 0.9999999999999997780, 1.000000000000000000, 1.000000000000000000, 1.000000000000000000, 1.000000000000000000, 1.000000000000000000, 1.000000000000000000, 1.000000000000000222, 1.000000000000000222, 1.000000000000000000, 1.000000000000000000, 1.000000000000000222, 1.000000000000000222, 1.000000000000000222, 1.000000000000000000, 1.000000000000000000, 1.000000000000000222, 1.000000000000000000, 1.000000000000000000, 1.000000000000000222, 1.000000000000000000, 1.000000000000000000, 1.000000000000000222, 1.000000000000000000, 1.000000000000000000, 0.9999999999999997780, 0.9999999999999998890, 1.000000000000000000, 1.000000000000000000, 1.000000000000000000, 1.000000000000000000, 1.000000000000000222, 1.000000000000000222, 1.000000000000000000, 1.000000000000000000, 1.000000000000000222, 1.000000000000000222, 1.000000000000000222, 1.000000000000000000, 1.000000000000000000, 1.000000000000000222, 1.000000000000000000, 1.000000000000000000, 1.000000000000000222, 1.000000000000000000, 1.000000000000000000, 1.000000000000000222, 1.000000000000000000, 1.000000000000000000, 0.9999999999999997780, 0.9999999999999998890, 1.000000000000000000, 1.000000000000000000, 1.000000000000000000, 1.000000000000000000, 1.000000000000000222, 1.000000000000000222, 1.000000000000000000, 1.000000000000000000, 1.000000000000000222, 1.000000000000000222, 1.000000000000000222, 1.000000000000000000, 1.000000000000000000, 1.000000000000000222, 1.000000000000000000, 0.9999999999999998890, 1.000000000000000222, 1.000000000000000000, 1.000000000000000000, 1.000000000000000222, 1.000000000000000000, 1.000000000000000000, 1.000000000000000222, 1.000000000000000000, 1.000000000000000000, 1.000000000000000000, 1.000000000000000000, 1.000000000000000000, 1.000000000000000222, 1.000000000000000222, 1.000000000000000000, 1.000000000000000000, 1.000000000000000222, 1.000000000000000222, 1.000000000000000222, 1.000000000000000000, 1.000000000000000222, 1.000000000000000222, 1.000000000000000000, 1.000000000000000000, 1.000000000000000222, 1.000000000000000000, 1.000000000000000000, 1.000000000000000222, 1.000000000000000000, 1.000000000000000000, 1.000000000000000222, 1.000000000000000222, 1.000000000000000000, 1.000000000000000000, 1.000000000000000222, 1.000000000000000000, 1.000000000000000222, 1.000000000000000222, 1.000000000000000000, 1.000000000000000000, 1.000000000000000222, 1.000000000000000222, 1.000000000000000222, 1.000000000000000000, 1.000000000000000000, 1.000000000000000222, 1.000000000000000000, 0.9999999999999998890, 1.000000000000000222, 1.000000000000000000, 1.000000000000000000, 1.000000000000000222, 1.000000000000000000, 1.000000000000000000, 1.000000000000000222, 1.000000000000000000, 1.000000000000000000, 1.000000000000000000, 1.000000000000000000, 1.000000000000000000, 1.000000000000000222, 1.000000000000000222, 1.000000000000000000, 1.000000000000000000, 1.000000000000000222, 1.000000000000000222, 1.000000000000000222, 1.000000000000000000, 1.000000000000000000, 1.000000000000000222, 1.000000000000000000, 1.000000000000000000, 1.000000000000000222, 1.000000000000000000, 1.000000000000000000, 1.000000000000000222, 1.000000000000000000, 0.9999999999999996669, 0.9999999999999996669, 1.000000000000000000, 1.000000000000000222, 1.000000000000000000, 1.000000000000000000, 1.000000000000000000, 1.000000000000000000, 1.000000000000000000, 1.000000000000000000, 1.000000000000000000, 1.000000000000000000),
 ( 0.3333333333333333703, 0.3333333333333333703, 0.3333333333333333703, 0.3333333333333334259, 0.3333333333333334259, 0.3333333333333334259, 0.3333333333333333703, 0.3333333333333333148, 0.3333333333333333703, 0.3333333333333333703, 0.3333333333333333148, 0.3333333333333333703, 0.3333333333333333703, 0.3333333333333334814, 0.3333333333333333703, 0.3333333333333333703, 0.3333333333333334259, 0.3333333333333333703, 0.3333333333333333148, 0.3333333333333333703, 0.3333333333333333703, 0.3333333333333333703, 0.3333333333333333703, 0.3333333333333333703, 0.3333333333333333148, 0.3333333333333334259, 0.3333333333333333703, 0.3333333333333333703, 0.3333333333333333703, 0.3333333333333334259, 0.3333333333333333703, 0.3333333333333333703, 0.3333333333333333703, 0.3333333333333333703, 0.3333333333333333148, 0.3333333333333333703, 0.3333333333333334259, 0.3333333333333333703, 0.3333333333333333703, 0.3333333333333333703, 0.3333333333333333703, 0.3333333333333333703, 0.3333333333333333703, 0.3333333333333333703, 0.3333333333333333703, 0.3333333333333333148, 0.3333333333333333703, 0.3333333333333333703, 0.3333333333333333703, 0.3333333333333334259, 0.3333333333333333703, 0.3333333333333333703, 0.3333333333333333703, 0.3333333333333333703, 0.3333333333333333703, 0.3333333333333334259, 0.3333333333333333703, 0.3333333333333333703, 0.3333333333333333703, 0.3333333333333333703, 0.3333333333333334259, 0.3333333333333333703, 0.3333333333333333703, 0.3333333333333333703, 0.3333333333333333703, 0.3333333333333333703, 0.3333333333333333703, 0.3333333333333333148, 0.3333333333333333148, 0.3333333333333333148, 0.3333333333333333703, 0.3333333333333333703, 0.3333333333333333148, 0.3333333333333334259, 0.3333333333333333703, 0.3333333333333333703, 0.3333333333333333703, 0.3333333333333333703, 0.3333333333333333703, 0.3333333333333333703, 0.3333333333333333703, 0.3333333333333333703, 0.3333333333333333703, 0.3333333333333334259, 0.3333333333333334259, 0.3333333333333333703, 0.3333333333333333703, 0.3333333333333333703, 0.3333333333333333703, 0.3333333333333333703, 0.3333333333333333703, 0.3333333333333333703, 0.3333333333333333148, 0.3333333333333333148, 0.3333333333333333703, 0.3333333333333333703, 0.3333333333333333148, 0.3333333333333334259, 0.3333333333333333703, 0.3333333333333333703, 0.3333333333333333703, 0.3333333333333333703, 0.3333333333333333703, 0.3333333333333333703, 0.3333333333333333703, 0.3333333333333333703, 0.3333333333333333703, 0.3333333333333333703, 0.3333333333333333703, 0.3333333333333333148, 0.3333333333333333703, 0.3333333333333333703, 0.3333333333333333703, 0.3333333333333333703, 0.3333333333333333148, 0.3333333333333333703, 0.3333333333333333703, 0.3333333333333333148, 0.3333333333333333703, 0.3333333333333333703, 0.3333333333333333148, 0.3333333333333334259, 0.3333333333333333703, 0.3333333333333333703, 0.3333333333333333703, 0.3333333333333333703, 0.3333333333333333703, 0.3333333333333334259, 0.3333333333333333703, 0.3333333333333333703, 0.3333333333333334259, 0.3333333333333334259, 0.3333333333333334259, 0.3333333333333333703, 0.3333333333333333703, 0.3333333333333333703, 0.3333333333333333703, 0.3333333333333333703, 0.3333333333333333703, 0.3333333333333333703, 0.3333333333333333703, 0.3333333333333333703, 0.3333333333333334259, 0.3333333333333333703, 0.3333333333333333148, 0.3333333333333334259, 0.3333333333333333703, 0.3333333333333333703, 0.3333333333333333703, 0.3333333333333333703, 0.3333333333333333703, 0.3333333333333334259, 0.3333333333333333703, 0.3333333333333333703, 0.3333333333333333703, 0.3333333333333334259, 0.3333333333333333703, 0.3333333333333333703, 0.3333333333333333703, 0.3333333333333333703, 0.3333333333333333703, 0.3333333333333333703, 0.3333333333333333148, 0.3333333333333334259, 0.3333333333333333703, 0.3333333333333333148, 0.3333333333333333703, 0.3333333333333333703, 0.3333333333333333703, 0.3333333333333334259, 0.3333333333333333703, 0.3333333333333333703, 0.3333333333333333703, 0.3333333333333333703, 0.3333333333333333703, 0.3333333333333334259, 0.3333333333333333703, 0.3333333333333333703, 0.3333333333333333703, 0.3333333333333333703, 0.3333333333333334259, 0.3333333333333333703, 0.3333333333333333703, 0.3333333333333333703, 0.3333333333333333703, 0.3333333333333333703, 0.3333333333333333703, 0.3333333333333333148, 0.3333333333333333703, 0.3333333333333333703, 0.3333333333333333703, 0.3333333333333333703, 0.3333333333333333148, 0.3333333333333333703, 0.3333333333333333703, 0.3333333333333333703, 0.3333333333333333703, 0.3333333333333333703),
 ( 0.3333333333333333703, 0.3333333333333333703, 0.3333333333333333703, 0.3333333333333334259, 0.3333333333333334259, 0.3333333333333334259, 0.3333333333333333703, 0.3333333333333333148, 0.3333333333333333703, 0.3333333333333333703, 0.3333333333333333148, 0.3333333333333333703, 0.3333333333333333703, 0.3333333333333334814, 0.3333333333333333703, 0.3333333333333333703, 0.3333333333333334259, 0.3333333333333333703, 0.3333333333333333148, 0.3333333333333333703, 0.3333333333333333703, 0.3333333333333333703, 0.3333333333333333703, 0.3333333333333333703, 0.3333333333333333148, 0.3333333333333334259, 0.3333333333333333703, 0.3333333333333333703, 0.3333333333333333703, 0.3333333333333334259, 0.3333333333333333703, 0.3333333333333333703, 0.3333333333333333703, 0.3333333333333333703, 0.3333333333333333148, 0.3333333333333333703, 0.3333333333333334259, 0.3333333333333333703, 0.3333333333333333703, 0.3333333333333333703, 0.3333333333333333703, 0.3333333333333333703, 0.3333333333333333703, 0.3333333333333333703, 0.3333333333333333703, 0.3333333333333333148, 0.3333333333333333703, 0.3333333333333333703, 0.3333333333333333703, 0.3333333333333334259, 0.3333333333333333703, 0.3333333333333333703, 0.3333333333333333703, 0.3333333333333333703, 0.3333333333333333703, 0.3333333333333334259, 0.3333333333333333703, 0.3333333333333333703, 0.3333333333333333703, 0.3333333333333333703, 0.3333333333333334259, 0.3333333333333333703, 0.3333333333333333703, 0.3333333333333333703, 0.3333333333333333703, 0.3333333333333333703, 0.3333333333333333703, 0.3333333333333333148, 0.3333333333333333148, 0.3333333333333333148, 0.3333333333333333703, 0.3333333333333333703, 0.3333333333333333148, 0.3333333333333334259, 0.3333333333333333703, 0.3333333333333333703, 0.3333333333333333703, 0.3333333333333333703, 0.3333333333333333703, 0.3333333333333333703, 0.3333333333333333703, 0.3333333333333333703, 0.3333333333333333703, 0.3333333333333334259, 0.3333333333333334259, 0.3333333333333333703, 0.3333333333333333703, 0.3333333333333333703, 0.3333333333333333703, 0.3333333333333333703, 0.3333333333333333703, 0.3333333333333333703, 0.3333333333333333148, 0.3333333333333333148, 0.3333333333333333703, 0.3333333333333333703, 0.3333333333333333148, 0.3333333333333334259, 0.3333333333333333703, 0.3333333333333333703, 0.3333333333333333703, 0.3333333333333333703, 0.3333333333333333703, 0.3333333333333333703, 0.3333333333333333703, 0.3333333333333333703, 0.3333333333333333703, 0.3333333333333333703, 0.3333333333333333703, 0.3333333333333333148, 0.3333333333333333703, 0.3333333333333333703, 0.3333333333333333703, 0.3333333333333333703, 0.3333333333333333148, 0.3333333333333333703, 0.3333333333333333703, 0.3333333333333333148, 0.3333333333333333703, 0.3333333333333333703, 0.3333333333333333148, 0.3333333333333334259, 0.3333333333333333703, 0.3333333333333333703, 0.3333333333333333703, 0.3333333333333333703, 0.3333333333333333703, 0.3333333333333334259, 0.3333333333333333703, 0.3333333333333333703, 0.3333333333333334259, 0.3333333333333334259, 0.3333333333333334259, 0.3333333333333333703, 0.3333333333333333703, 0.3333333333333333703, 0.3333333333333333703, 0.3333333333333333703, 0.3333333333333333703, 0.3333333333333333703, 0.3333333333333333703, 0.3333333333333333703, 0.3333333333333334259, 0.3333333333333333703, 0.3333333333333333148, 0.3333333333333334259, 0.3333333333333333703, 0.3333333333333333703, 0.3333333333333333703, 0.3333333333333333703, 0.3333333333333333703, 0.3333333333333334259, 0.3333333333333333703, 0.3333333333333333703, 0.3333333333333333703, 0.3333333333333334259, 0.3333333333333333703, 0.3333333333333333703, 0.3333333333333333703, 0.3333333333333333703, 0.3333333333333333703, 0.3333333333333333703, 0.3333333333333333148, 0.3333333333333334259, 0.3333333333333333703, 0.3333333333333333148, 0.3333333333333333703, 0.3333333333333333703, 0.3333333333333333703, 0.3333333333333334259, 0.3333333333333333703, 0.3333333333333333703, 0.3333333333333333703, 0.3333333333333333703, 0.3333333333333333703, 0.3333333333333334259, 0.3333333333333333703, 0.3333333333333333703, 0.3333333333333333703, 0.3333333333333333703, 0.3333333333333334259, 0.3333333333333333703, 0.3333333333333333703, 0.3333333333333333703, 0.3333333333333333703, 0.3333333333333333703, 0.3333333333333333703, 0.3333333333333333148, 0.3333333333333333703, 0.3333333333333333703, 0.3333333333333333703, 0.3333333333333333703, 0.3333333333333333148, 0.3333333333333333703, 0.3333333333333333703, 0.3333333333333333703, 0.3333333333333333703, 0.3333333333333333703),
 ( 1.000000000000000000, 1.000000000000000000, 1.000000000000000000, 1.000000000000000000, 1.000000000000000000, 1.000000000000000000, 0.9999999999999998890, 0.9999999999999997780, 1.000000000000000000, 1.000000000000000000, 1.000000000000000000, 1.000000000000000000, 1.000000000000000000, 1.000000000000000000, 0.9999999999999998890, 1.000000000000000000, 1.000000000000000222, 1.000000000000000000, 1.000000000000000000, 1.000000000000000000, 1.000000000000000000, 1.000000000000000000, 0.9999999999999998890, 0.9999999999999997780, 1.000000000000000000, 1.000000000000000222, 1.000000000000000000, 1.000000000000000000, 1.000000000000000000, 1.000000000000000000, 0.9999999999999998890, 0.9999999999999997780, 1.000000000000000000, 0.9999999999999998890, 0.9999999999999997780, 1.000000000000000000, 1.000000000000000222, 1.000000000000000222, 1.000000000000000000, 1.000000000000000000, 1.000000000000000222, 1.000000000000000000, 0.9999999999999997780, 1.000000000000000000, 1.000000000000000000, 1.000000000000000000, 1.000000000000000000, 1.000000000000000000, 1.000000000000000000, 1.000000000000000222, 1.000000000000000222, 1.000000000000000000, 1.000000000000000000, 1.000000000000000222, 1.000000000000000222, 1.000000000000000222, 1.000000000000000000, 1.000000000000000000, 1.000000000000000222, 1.000000000000000000, 1.000000000000000000, 1.000000000000000222, 1.000000000000000000, 1.000000000000000000, 1.000000000000000222, 1.000000000000000000, 1.000000000000000000, 0.9999999999999997780, 0.9999999999999998890, 1.000000000000000000, 1.000000000000000000, 1.000000000000000000, 1.000000000000000000, 1.000000000000000222, 1.000000000000000222, 1.000000000000000000, 1.000000000000000000, 1.000000000000000222, 1.000000000000000222, 1.000000000000000222, 1.000000000000000000, 1.000000000000000000, 1.000000000000000222, 1.000000000000000000, 1.000000000000000000, 1.000000000000000222, 1.000000000000000000, 1.000000000000000000, 1.000000000000000222, 1.000000000000000000, 1.000000000000000000, 0.9999999999999997780, 0.9999999999999998890, 1.000000000000000000, 1.000000000000000000, 1.000000000000000000, 1.000000000000000000, 1.000000000000000222, 1.000000000000000222, 1.000000000000000000, 1.000000000000000000, 1.000000000000000222, 1.000000000000000222, 1.000000000000000222, 1.000000000000000000, 1.000000000000000000, 1.000000000000000222, 1.000000000000000000, 0.9999999999999998890, 1.000000000000000222, 1.000000000000000000, 1.000000000000000000, 1.000000000000000222, 1.000000000000000000, 1.000000000000000000, 1.000000000000000222, 1.000000000000000000, 1.000000000000000000, 1.000000000000000000, 1.000000000000000000, 1.000000000000000000, 1.000000000000000222, 1.000000000000000222, 1.000000000000000000, 1.000000000000000000, 1.000000000000000222, 1.000000000000000222, 1.000000000000000222, 1.000000000000000000, 1.000000000000000222, 1.000000000000000222, 1.000000000000000000, 1.000000000000000000, 1.000000000000000222, 1.000000000000000000, 1.000000000000000000, 1.000000000000000222, 1.000000000000000000, 1.000000000000000000, 1.000000000000000222, 1.000000000000000222, 1.000000000000000000, 1.000000000000000000, 1.000000000000000222, 1.000000000000000000, 1.000000000000000222, 1.000000000000000222, 1.000000000000000000, 1.000000000000000000, 1.000000000000000222, 1.000000000000000222, 1.000000000000000222, 1.000000000000000000, 1.000000000000000000, 1.000000000000000222, 1.000000000000000000, 0.9999999999999998890, 1.000000000000000222, 1.000000000000000000, 1.000000000000000000, 1.000000000000000222, 1.000000000000000000, 1.000000000000000000, 1.000000000000000222, 1.000000000000000000, 1.000000000000000000, 1.000000000000000000, 1.000000000000000000, 1.000000000000000000, 1.000000000000000222, 1.000000000000000222, 1.000000000000000000, 1.000000000000000000, 1.000000000000000222, 1.000000000000000222, 1.000000000000000222, 1.000000000000000000, 1.000000000000000000, 1.000000000000000222, 1.000000000000000000, 1.000000000000000000, 1.000000000000000222, 1.000000000000000000, 1.000000000000000000, 1.000000000000000222, 1.000000000000000000, 0.9999999999999996669, 0.9999999999999996669, 1.000000000000000000, 1.000000000000000222, 1.000000000000000000, 1.000000000000000000, 1.000000000000000000, 1.000000000000000000, 1.000000000000000000, 1.000000000000000000, 1.000000000000000000, 1.000000000000000000),
 ( 0.3333333333333333703, 0.3333333333333333703, 0.3333333333333333703, 0.3333333333333334259, 0.3333333333333334259, 0.3333333333333334259, 0.3333333333333333703, 0.3333333333333333148, 0.3333333333333333703, 0.3333333333333333703, 0.3333333333333333148, 0.3333333333333333703, 0.3333333333333333703, 0.3333333333333334814, 0.3333333333333333703, 0.3333333333333333703, 0.3333333333333334259, 0.3333333333333333703, 0.3333333333333333148, 0.3333333333333333703, 0.3333333333333333703, 0.3333333333333333703, 0.3333333333333333703, 0.3333333333333333703, 0.3333333333333333148, 0.3333333333333334259, 0.3333333333333333703, 0.3333333333333333703, 0.3333333333333333703, 0.3333333333333334259, 0.3333333333333333703, 0.3333333333333333703, 0.3333333333333333703, 0.3333333333333333703, 0.3333333333333333148, 0.3333333333333333703, 0.3333333333333334259, 0.3333333333333333703, 0.3333333333333333703, 0.3333333333333333703, 0.3333333333333333703, 0.3333333333333333703, 0.3333333333333333703, 0.3333333333333333703, 0.3333333333333333703, 0.3333333333333333148, 0.3333333333333333703, 0.3333333333333333703, 0.3333333333333333703, 0.3333333333333334259, 0.3333333333333333703, 0.3333333333333333703, 0.3333333333333333703, 0.3333333333333333703, 0.3333333333333333703, 0.3333333333333334259, 0.3333333333333333703, 0.3333333333333333703, 0.3333333333333333703, 0.3333333333333333703, 0.3333333333333334259, 0.3333333333333333703, 0.3333333333333333703, 0.3333333333333333703, 0.3333333333333333703, 0.3333333333333333703, 0.3333333333333333703, 0.3333333333333333148, 0.3333333333333333148, 0.3333333333333333148, 0.3333333333333333703, 0.3333333333333333703, 0.3333333333333333148, 0.3333333333333334259, 0.3333333333333333703, 0.3333333333333333703, 0.3333333333333333703, 0.3333333333333333703, 0.3333333333333333703, 0.3333333333333333703, 0.3333333333333333703, 0.3333333333333333703, 0.3333333333333333703, 0.3333333333333334259, 0.3333333333333334259, 0.3333333333333333703, 0.3333333333333333703, 0.3333333333333333703, 0.3333333333333333703, 0.3333333333333333703, 0.3333333333333333703, 0.3333333333333333703, 0.3333333333333333148, 0.3333333333333333148, 0.3333333333333333703, 0.3333333333333333703, 0.3333333333333333148, 0.3333333333333334259, 0.3333333333333333703, 0.3333333333333333703, 0.3333333333333333703, 0.3333333333333333703, 0.3333333333333333703, 0.3333333333333333703, 0.3333333333333333703, 0.3333333333333333703, 0.3333333333333333703, 0.3333333333333333703, 0.3333333333333333703, 0.3333333333333333148, 0.3333333333333333703, 0.3333333333333333703, 0.3333333333333333703, 0.3333333333333333703, 0.3333333333333333148, 0.3333333333333333703, 0.3333333333333333703, 0.3333333333333333148, 0.3333333333333333703, 0.3333333333333333703, 0.3333333333333333148, 0.3333333333333334259, 0.3333333333333333703, 0.3333333333333333703, 0.3333333333333333703, 0.3333333333333333703, 0.3333333333333333703, 0.3333333333333334259, 0.3333333333333333703, 0.3333333333333333703, 0.3333333333333334259, 0.3333333333333334259, 0.3333333333333334259, 0.3333333333333333703, 0.3333333333333333703, 0.3333333333333333703, 0.3333333333333333703, 0.3333333333333333703, 0.3333333333333333703, 0.3333333333333333703, 0.3333333333333333703, 0.3333333333333333703, 0.3333333333333334259, 0.3333333333333333703, 0.3333333333333333148, 0.3333333333333334259, 0.3333333333333333703, 0.3333333333333333703, 0.3333333333333333703, 0.3333333333333333703, 0.3333333333333333703, 0.3333333333333334259, 0.3333333333333333703, 0.3333333333333333703, 0.3333333333333333703, 0.3333333333333334259, 0.3333333333333333703, 0.3333333333333333703, 0.3333333333333333703, 0.3333333333333333703, 0.3333333333333333703, 0.3333333333333333703, 0.3333333333333333148, 0.3333333333333334259, 0.3333333333333333703, 0.3333333333333333148, 0.3333333333333333703, 0.3333333333333333703, 0.3333333333333333703, 0.3333333333333334259, 0.3333333333333333703, 0.3333333333333333703, 0.3333333333333333703, 0.3333333333333333703, 0.3333333333333333703, 0.3333333333333334259, 0.3333333333333333703, 0.3333333333333333703, 0.3333333333333333703, 0.3333333333333333703, 0.3333333333333334259, 0.3333333333333333703, 0.3333333333333333703, 0.3333333333333333703, 0.3333333333333333703, 0.3333333333333333703, 0.3333333333333333703, 0.3333333333333333148, 0.3333333333333333703, 0.3333333333333333703, 0.3333333333333333703, 0.3333333333333333703, 0.3333333333333333148, 0.3333333333333333703, 0.3333333333333333703, 0.3333333333333333703, 0.3333333333333333703, 0.3333333333333333703),
 ( 0.3333333333333333703, 0.3333333333333333703, 0.3333333333333333703, 0.3333333333333334259, 0.3333333333333334259, 0.3333333333333334259, 0.3333333333333333703, 0.3333333333333333148, 0.3333333333333333703, 0.3333333333333333703, 0.3333333333333333148, 0.3333333333333333703, 0.3333333333333333703, 0.3333333333333334814, 0.3333333333333333703, 0.3333333333333333703, 0.3333333333333334259, 0.3333333333333333703, 0.3333333333333333148, 0.3333333333333333703, 0.3333333333333333703, 0.3333333333333333703, 0.3333333333333333703, 0.3333333333333333703, 0.3333333333333333148, 0.3333333333333334259, 0.3333333333333333703, 0.3333333333333333703, 0.3333333333333333703, 0.3333333333333334259, 0.3333333333333333703, 0.3333333333333333703, 0.3333333333333333703, 0.3333333333333333703, 0.3333333333333333148, 0.3333333333333333703, 0.3333333333333334259, 0.3333333333333333703, 0.3333333333333333703, 0.3333333333333333703, 0.3333333333333333703, 0.3333333333333333703, 0.3333333333333333703, 0.3333333333333333703, 0.3333333333333333703, 0.3333333333333333148, 0.3333333333333333703, 0.3333333333333333703, 0.3333333333333333703, 0.3333333333333334259, 0.3333333333333333703, 0.3333333333333333703, 0.3333333333333333703, 0.3333333333333333703, 0.3333333333333333703, 0.3333333333333334259, 0.3333333333333333703, 0.3333333333333333703, 0.3333333333333333703, 0.3333333333333333703, 0.3333333333333334259, 0.3333333333333333703, 0.3333333333333333703, 0.3333333333333333703, 0.3333333333333333703, 0.3333333333333333703, 0.3333333333333333703, 0.3333333333333333148, 0.3333333333333333148, 0.3333333333333333148, 0.3333333333333333703, 0.3333333333333333703, 0.3333333333333333148, 0.3333333333333334259, 0.3333333333333333703, 0.3333333333333333703, 0.3333333333333333703, 0.3333333333333333703, 0.3333333333333333703, 0.3333333333333333703, 0.3333333333333333703, 0.3333333333333333703, 0.3333333333333333703, 0.3333333333333334259, 0.3333333333333334259, 0.3333333333333333703, 0.3333333333333333703, 0.3333333333333333703, 0.3333333333333333703, 0.3333333333333333703, 0.3333333333333333703, 0.3333333333333333703, 0.3333333333333333148, 0.3333333333333333148, 0.3333333333333333703, 0.3333333333333333703, 0.3333333333333333148, 0.3333333333333334259, 0.3333333333333333703, 0.3333333333333333703, 0.3333333333333333703, 0.3333333333333333703, 0.3333333333333333703, 0.3333333333333333703, 0.3333333333333333703, 0.3333333333333333703, 0.3333333333333333703, 0.3333333333333333703, 0.3333333333333333703, 0.3333333333333333148, 0.3333333333333333703, 0.3333333333333333703, 0.3333333333333333703, 0.3333333333333333703, 0.3333333333333333148, 0.3333333333333333703, 0.3333333333333333703, 0.3333333333333333148, 0.3333333333333333703, 0.3333333333333333703, 0.3333333333333333148, 0.3333333333333334259, 0.3333333333333333703, 0.3333333333333333703, 0.3333333333333333703, 0.3333333333333333703, 0.3333333333333333703, 0.3333333333333334259, 0.3333333333333333703, 0.3333333333333333703, 0.3333333333333334259, 0.3333333333333334259, 0.3333333333333334259, 0.3333333333333333703, 0.3333333333333333703, 0.3333333333333333703, 0.3333333333333333703, 0.3333333333333333703, 0.3333333333333333703, 0.3333333333333333703, 0.3333333333333333703, 0.3333333333333333703, 0.3333333333333334259, 0.3333333333333333703, 0.3333333333333333148, 0.3333333333333334259, 0.3333333333333333703, 0.3333333333333333703, 0.3333333333333333703, 0.3333333333333333703, 0.3333333333333333703, 0.3333333333333334259, 0.3333333333333333703, 0.3333333333333333703, 0.3333333333333333703, 0.3333333333333334259, 0.3333333333333333703, 0.3333333333333333703, 0.3333333333333333703, 0.3333333333333333703, 0.3333333333333333703, 0.3333333333333333703, 0.3333333333333333148, 0.3333333333333334259, 0.3333333333333333703, 0.3333333333333333148, 0.3333333333333333703, 0.3333333333333333703, 0.3333333333333333703, 0.3333333333333334259, 0.3333333333333333703, 0.3333333333333333703, 0.3333333333333333703, 0.3333333333333333703, 0.3333333333333333703, 0.3333333333333334259, 0.3333333333333333703, 0.3333333333333333703, 0.3333333333333333703, 0.3333333333333333703, 0.3333333333333334259, 0.3333333333333333703, 0.3333333333333333703, 0.3333333333333333703, 0.3333333333333333703, 0.3333333333333333703, 0.3333333333333333703, 0.3333333333333333148, 0.3333333333333333703, 0.3333333333333333703, 0.3333333333333333703, 0.3333333333333333703, 0.3333333333333333148, 0.3333333333333333703, 0.3333333333333333703, 0.3333333333333333703, 0.3333333333333333703, 0.3333333333333333703),
 ( 1.000000000000000000, 1.000000000000000000, 1.000000000000000000, 1.000000000000000000, 1.000000000000000000, 1.000000000000000000, 0.9999999999999998890, 0.9999999999999997780, 1.000000000000000000, 1.000000000000000000, 1.000000000000000000, 1.000000000000000000, 1.000000000000000000, 1.000000000000000000, 0.9999999999999998890, 1.000000000000000000, 1.000000000000000222, 1.000000000000000000, 1.000000000000000000, 1.000000000000000000, 1.000000000000000000, 1.000000000000000000, 0.9999999999999998890, 0.9999999999999997780, 1.000000000000000000, 1.000000000000000222, 1.000000000000000000, 1.000000000000000000, 1.000000000000000000, 1.000000000000000000, 0.9999999999999998890, 0.9999999999999997780, 1.000000000000000000, 0.9999999999999998890, 0.9999999999999997780, 1.000000000000000000, 1.000000000000000222, 1.000000000000000222, 1.000000000000000000, 1.000000000000000000, 1.000000000000000222, 1.000000000000000000, 0.9999999999999997780, 1.000000000000000000, 1.000000000000000000, 1.000000000000000000, 1.000000000000000000, 1.000000000000000000, 1.000000000000000000, 1.000000000000000222, 1.000000000000000222, 1.000000000000000000, 1.000000000000000000, 1.000000000000000222, 1.000000000000000222, 1.000000000000000222, 1.000000000000000000, 1.000000000000000000, 1.000000000000000222, 1.000000000000000000, 1.000000000000000000, 1.000000000000000222, 1.000000000000000000, 1.000000000000000000, 1.000000000000000222, 1.000000000000000000, 1.000000000000000000, 0.9999999999999997780, 0.9999999999999998890, 1.000000000000000000, 1.000000000000000000, 1.000000000000000000, 1.000000000000000000, 1.000000000000000222, 1.000000000000000222, 1.000000000000000000, 1.000000000000000000, 1.000000000000000222, 1.000000000000000222, 1.000000000000000222, 1.000000000000000000, 1.000000000000000000, 1.000000000000000222, 1.000000000000000000, 1.000000000000000000, 1.000000000000000222, 1.000000000000000000, 1.000000000000000000, 1.000000000000000222, 1.000000000000000000, 1.000000000000000000, 0.9999999999999997780, 0.9999999999999998890, 1.000000000000000000, 1.000000000000000000, 1.000000000000000000, 1.000000000000000000, 1.000000000000000222, 1.000000000000000222, 1.000000000000000000, 1.000000000000000000, 1.000000000000000222, 1.000000000000000222, 1.000000000000000222, 1.000000000000000000, 1.000000000000000000, 1.000000000000000222, 1.000000000000000000, 0.9999999999999998890, 1.000000000000000222, 1.000000000000000000, 1.000000000000000000, 1.000000000000000222, 1.000000000000000000, 1.000000000000000000, 1.000000000000000222, 1.000000000000000000, 1.000000000000000000, 1.000000000000000000, 1.000000000000000000, 1.000000000000000000, 1.000000000000000222, 1.000000000000000222, 1.000000000000000000, 1.000000000000000000, 1.000000000000000222, 1.000000000000000222, 1.000000000000000222, 1.000000000000000000, 1.000000000000000222, 1.000000000000000222, 1.000000000000000000, 1.000000000000000000, 1.000000000000000222, 1.000000000000000000, 1.000000000000000000, 1.000000000000000222, 1.000000000000000000, 1.000000000000000000, 1.000000000000000222, 1.000000000000000222, 1.000000000000000000, 1.000000000000000000, 1.000000000000000222, 1.000000000000000000, 1.000000000000000222, 1.000000000000000222, 1.000000000000000000, 1.000000000000000000, 1.000000000000000222, 1.000000000000000222, 1.000000000000000222, 1.000000000000000000, 1.000000000000000000, 1.000000000000000222, 1.000000000000000000, 0.9999999999999998890, 1.000000000000000222, 1.000000000000000000, 1.000000000000000000, 1.000000000000000222, 1.000000000000000000, 1.000000000000000000, 1.000000000000000222, 1.000000000000000000, 1.000000000000000000, 1.000000000000000000, 1.000000000000000000, 1.000000000000000000, 1.000000000000000222, 1.000000000000000222, 1.000000000000000000, 1.000000000000000000, 1.000000000000000222, 1.000000000000000222, 1.000000000000000222, 1.000000000000000000, 1.000000000000000000, 1.000000000000000222, 1.000000000000000000, 1.000000000000000000, 1.000000000000000222, 1.000000000000000000, 1.000000000000000000, 1.000000000000000222, 1.000000000000000000, 0.9999999999999996669, 0.9999999999999996669, 1.000000000000000000, 1.000000000000000222, 1.000000000000000000, 1.000000000000000000, 1.000000000000000000, 1.000000000000000000, 1.000000000000000000, 1.000000000000000000, 1.000000000000000000, 1.000000000000000000) ) ) 
 REPRESENTATION_ITEM ( '' )  SURFACE ( )  );
#20692=CARTESIAN_POINT ( 'NONE',  ( 18.44328704050455769, 144.7751241387205425, -1.717333923880829616 ) ) ;
#20693=CARTESIAN_POINT ( 'NONE',  ( -6.734570810858633294, 118.9580315507705706, -1.247721039026444378 ) ) ;
#20694=PLANE ( 'NONE',  #5250 ) ;
#20695=CARTESIAN_POINT ( 'NONE',  ( 4.265934612124557823, 118.2243144435457936, -0.2925027961061675286 ) ) ;
#20696=CARTESIAN_POINT ( 'NONE',  ( 13.89276580153818230, 150.2454140652271803, -0.5485491450630708421 ) ) ;
#20697=EDGE_CURVE ( 'NONE', #35234, #12250, #40073, .T. ) ;
#20699=CARTESIAN_POINT ( 'NONE',  ( 3.113553847179573175, -14.91884098843750195, 3.610284256090800170 ) ) ;
#20700=CARTESIAN_POINT ( 'NONE',  ( -4.828569062062975092, 117.4060461567800786, 1.008118597039231235 ) ) ;
#20702=CARTESIAN_POINT ( 'NONE',  ( 3.363087486136625337, 4.875765145370108300, -3.182472177310056605 ) ) ;
#20703=CARTESIAN_POINT ( 'NONE',  ( 16.93203274801135905, 148.0818255213264365, 2.041866944467892964 ) ) ;
#20704=CARTESIAN_POINT ( 'NONE',  ( 2.958531772299236362, 39.20946620154573026, 1.329372033065076231 ) ) ;
#20705=CARTESIAN_POINT ( 'NONE',  ( -6.675377558974173731, 121.2389289720308199, 0.07470202506228494632 ) ) ;
#20707=CARTESIAN_POINT ( 'NONE',  ( 4.419457123578296454, 17.78516144714274105, -1.360477052881604143 ) ) ;
#20708=CARTESIAN_POINT ( 'NONE',  ( 8.793090887880877560, 123.6850765633735421, 0.2090564433599598482 ) ) ;
#20709=CARTESIAN_POINT ( 'NONE',  ( -2.105106575660352419, 106.4592691022973270, 4.917738869260992907 ) ) ;
#20712=CARTESIAN_POINT ( 'NONE',  ( 8.796521542695449725, 117.7070916852149907, 0.01881401154734642714 ) ) ;
#20715=CARTESIAN_POINT ( 'NONE',  ( -1.247394927440314882, 105.9869000721035661, 5.191483356333327137 ) ) ;
#20716=CARTESIAN_POINT ( 'NONE',  ( -3.682264917456324227, 91.53346620154573543, -0.07358041635423968885 ) ) ;
#20717=CARTESIAN_POINT ( 'NONE',  ( 5.949252453048933909, -3.155934468320678921, 5.972130579448434951 ) ) ;
#20718=CARTESIAN_POINT ( 'NONE',  ( -6.654617103318593247E-14, 104.6144662015457243, 1.534725424433578570E-31 ) ) ;
#20721=CARTESIAN_POINT ( 'NONE',  ( -4.987188648064493357, 117.3993836136597366, -0.9009750914350973527 ) ) ;
#20722=CARTESIAN_POINT ( 'NONE',  ( -22.92015980622324989, 150.1344166263168347, -0.006220127847215065238 ) ) ;
#20725=CARTESIAN_POINT ( 'NONE',  ( -6.064028428014071714, 121.4341838187324782, -0.1213693123384972511 ) ) ;
#20726=VERTEX_POINT ( 'NONE', #22843 ) ;
#20728=CARTESIAN_POINT ( 'NONE',  ( -9.016099448416641238, 124.0612890738674992, -0.1356653335066258237 ) ) ;
#20729=CARTESIAN_POINT ( 'NONE',  ( 3.231152580208111580, -15.43077800403741584, 5.551260886339890455 ) ) ;
#20730=CARTESIAN_POINT ( 'NONE',  ( -11.94841889513460664, 120.7721054874162974, 1.107169436317064770 ) ) ;
#20731=CARTESIAN_POINT ( 'NONE',  ( 23.12143742665057289, 148.7607265879045144, 1.192451864686425722 ) ) ;
#20732=CARTESIAN_POINT ( 'NONE',  ( 21.63845757858504726, 150.4657531037631486, -1.001545151475623951 ) ) ;
#20733=CARTESIAN_POINT ( 'NONE',  ( -4.050807963365556930, 30.95410787014092335, -2.229501126309402448 ) ) ;
#20734=CARTESIAN_POINT ( 'NONE',  ( -20.67395311655602086, 152.5754960671270055, -0.6363119977773274982 ) ) ;
#20736=CARTESIAN_POINT ( 'NONE',  ( 4.973439878603004516, 117.3975399628824903, 0.9753616027188249937 ) ) ;
#20737=VERTEX_POINT ( 'NONE', #32676 ) ;
#20738=CARTESIAN_POINT ( 'NONE',  ( -8.775993782722990133, 117.8320326000692830, 0.2360534736673538525 ) ) ;
#20739=CARTESIAN_POINT ( 'NONE',  ( -5.099922610524069810, 119.9665122172617231, 0.7872683264543848258 ) ) ;
#20741=CARTESIAN_POINT ( 'NONE',  ( 12.68516923343323910, 122.7135068550949200, -1.328447112472142644 ) ) ;
#20742=CARTESIAN_POINT ( 'NONE',  ( -0.4041098725243945644, -13.24273492701920141, -0.8882236940730178221 ) ) ;
#20743=CARTESIAN_POINT ( 'NONE',  ( -13.72986513748895732, 121.3979351292862816, -1.556522170903472890 ) ) ;
#20746=CARTESIAN_POINT ( 'NONE',  ( 15.38818086081963976, 149.0334586719817764, -0.9521378535654881903 ) ) ;
#20747=CARTESIAN_POINT ( 'NONE',  ( -2.884051542275779756, 156.0957788938021054, -0.05763021347587621995 ) ) ;
#20748=CIRCLE ( 'NONE', #16671, 3.683000000000001162 ) ;
#20750=CARTESIAN_POINT ( 'NONE',  ( -11.58692091624697973, 123.4149316504530702, -1.682406715187617419 ) ) ;
#20751=CARTESIAN_POINT ( 'NONE',  ( 4.596189786833723367, -15.64549520875656263, 3.377287787771500849 ) ) ;
#20753=CARTESIAN_POINT ( 'NONE',  ( -4.364856043270152419, 118.1847667706781095, -0.6011001361930394804 ) ) ;
#20756=CARTESIAN_POINT ( 'NONE',  ( 17.79834178490394336, 144.5560955566678558, 2.349204209454023307 ) ) ;
#20758=CARTESIAN_POINT ( 'NONE',  ( 21.90559427349690935, 151.4293160993575498, 0.4377259060014666026 ) ) ;
#20760=CARTESIAN_POINT ( 'NONE',  ( -8.175057852536518510, 12.81247082500981094, 2.033924511151908199 ) ) ;
#20761=CARTESIAN_POINT ( 'NONE',  ( 11.34253674425776204, 128.2076764602477681, 0.6137764907266788361 ) ) ;
#20762=CARTESIAN_POINT ( 'NONE',  ( 5.863496024706776666, 117.4684171610355747, -0.5179920176435334200 ) ) ;
#20764=CARTESIAN_POINT ( 'NONE',  ( 1.075792877641968071, 115.6909491485452719, 1.747631130524746279 ) ) ;
#20766=CARTESIAN_POINT ( 'NONE',  ( -20.47124607682640729, 129.0748834149669904, -0.3487454591146176841 ) ) ;
#20770=CARTESIAN_POINT ( 'NONE',  ( 6.898830447510338360, 121.7080221937641369, -0.3537813070057239107 ) ) ;
#20772=ORIENTED_EDGE ( 'NONE', *, *, #13097, .F. ) ;
#20773=CARTESIAN_POINT ( 'NONE',  ( 0.2373273420099217268, 115.6909491485452719, -1.758352294689179196 ) ) ;
#20774=CARTESIAN_POINT ( 'NONE',  ( -4.329655997251418142, 155.8404949922767742, -0.5159277680907118357 ) ) ;
#20775=CARTESIAN_POINT ( 'NONE',  ( 4.667506617707346983, -11.86120359225895093, 0.9697133514482669803 ) ) ;
#20776=CARTESIAN_POINT ( 'NONE',  ( -14.56950268504908941, 121.1548589120785095, 0.7262516135598525713 ) ) ;
#20778=CARTESIAN_POINT ( 'NONE',  ( 15.43849248880384906, 120.7004057517279989, 0.4663222373074407678 ) ) ;
#20779=ORIENTED_EDGE ( 'NONE', *, *, #19063, .F. ) ;
#20780=CARTESIAN_POINT ( 'NONE',  ( 0.09481320634720795393, -4.229605868409334057, 4.636458411128852930 ) ) ;
#20781=CARTESIAN_POINT ( 'NONE',  ( -15.95982161465190430, 121.0385544001969436, -0.3359599701671935890 ) ) ;
#20785=CARTESIAN_POINT ( 'NONE',  ( -5.117521106717683566, 119.2591321592902744, 0.9016134253432759316 ) ) ;
#20786=CARTESIAN_POINT ( 'NONE',  ( -4.070821798575407158, -9.904843093959119216, 2.245307785351264407 ) ) ;
#20787=CARTESIAN_POINT ( 'NONE',  ( 7.998778050759611347, 118.2752802814886053, 1.041156008592528659 ) ) ;
#20789=CARTESIAN_POINT ( 'NONE',  ( 0.4390033025490695517, 118.1045761740670201, -0.5613618447453815330 ) ) ;
#20790=CARTESIAN_POINT ( 'NONE',  ( 3.440871586586784936, -6.993729544307834445, 3.087053954803492761 ) ) ;
#20791=CARTESIAN_POINT ( 'NONE',  ( -22.50377699857072145, 149.0203452686010337, -1.755643737887156997 ) ) ;
#20792=EDGE_LOOP ( 'NONE', ( #31818, #11684, #22277, #14636, #173 ) ) ;
#20793=VERTEX_POINT ( 'NONE', #6905 ) ;
#20794=CARTESIAN_POINT ( 'NONE',  ( -9.165091971927694203, 123.9989874199980022, 0.04717021870285753593 ) ) ;
#20795=CARTESIAN_POINT ( 'NONE',  ( 6.089492611447847814, -14.32660765653466584, 1.811095812122764270 ) ) ;
#20800=CARTESIAN_POINT ( 'NONE',  ( 19.16322371038626571, 147.9830121424878939, 2.503561316673066806 ) ) ;
#20803=CARTESIAN_POINT ( 'NONE',  ( -4.866704567515652613, 117.3073154462328063, 0.4935321157908419409 ) ) ;
#20804=CARTESIAN_POINT ( 'NONE',  ( 6.390864997528122871, 2.724353428444007630, 5.482255947279437436 ) ) ;
#20805=CARTESIAN_POINT ( 'NONE',  ( 15.74774640517356517, 148.1776054874778197, 1.420244701258234210 ) ) ;
#20807=CARTESIAN_POINT ( 'NONE',  ( 20.50889283491256876, 152.5656283612522657, -0.2944088047499978655 ) ) ;
#20813=CARTESIAN_POINT ( 'NONE',  ( -4.116168481435051874, 118.2429491485453354, 0.1886889149009219058 ) ) ;
#20814=CARTESIAN_POINT ( 'NONE',  ( 1.247284263955336758, 105.9875614017104368, -5.191247707446073889 ) ) ;
#20818=CARTESIAN_POINT ( 'NONE',  ( 8.325909852675222211, 120.1128631755567113, -1.118201085292081176 ) ) ;
#20819=CARTESIAN_POINT ( 'NONE',  ( -5.298772840285949748, 116.6867539651165373, -1.022742042655826022 ) ) ;
#20820=CARTESIAN_POINT ( 'NONE',  ( 4.381205243309556963, 118.1833089681223470, 0.5842985504508096950 ) ) ;
#20821=CARTESIAN_POINT ( 'NONE',  ( -6.352854517228420761, 155.4084287100276072, -1.029490774253102536 ) ) ;
#20822=CARTESIAN_POINT ( 'NONE',  ( -0.4623567408945805646, 115.7034747641299930, -1.762870502475438972 ) ) ;
#20823=CARTESIAN_POINT ( 'NONE',  ( -3.682264917456322895, 69.94346620154573202, -0.07358041635423923088 ) ) ;
#20826=CARTESIAN_POINT ( 'NONE',  ( 4.844936406558457698, 112.7696648386057632, -2.375766922042533036 ) ) ;
#20827=CARTESIAN_POINT ( 'NONE',  ( 0.01887828017110892292, 156.5412816204240301, -0.9447463363288812754 ) ) ;
#20830=AXIS2_PLACEMENT_3D ( 'NONE', #22693, #25700, #16316 ) ;
#20832=CARTESIAN_POINT ( 'NONE',  ( -15.26787271661999235, 148.0267594272436895, -0.1054338715682280742 ) ) ;
#20833=CARTESIAN_POINT ( 'NONE',  ( 4.850929972935443146, 117.7610086971114356, 0.9074237114610381738 ) ) ;
#20834=CARTESIAN_POINT ( 'NONE',  ( 20.30524341716966319, 152.5255278361454145, 1.346157490925044664 ) ) ;
#20836=CARTESIAN_POINT ( 'NONE',  ( 3.411949332026259274, -14.94726182254324520, 2.206293558762954188 ) ) ;
#20837=CARTESIAN_POINT ( 'NONE',  ( 21.17434475962598484, 141.7209635633906259, -1.395834004474946655 ) ) ;
#20838=CARTESIAN_POINT ( 'NONE',  ( -11.50356673920490991, 154.6851215890897038, 1.708948620147628938 ) ) ;
#20839=CARTESIAN_POINT ( 'NONE',  ( -0.9685753864191435358, -11.31243604255521085, 0.1179740209226832204 ) ) ;
#20840=CARTESIAN_POINT ( 'NONE',  ( -11.45183593531622535, 118.8698716516685465, -0.7694570404682199438 ) ) ;
#20841=CARTESIAN_POINT ( 'NONE',  ( 0.3309596775784566236, 20.21946177965197222, 0.9160044982600296093 ) ) ;
#20845=CARTESIAN_POINT ( 'NONE',  ( -12.13795026801536814, 151.9817061558079274, 0.5567646394148116906 ) ) ;
#20846=CARTESIAN_POINT ( 'NONE',  ( 4.964329757808820354, -12.46733462535230785, 1.954119038396571417 ) ) ;
#20847=CARTESIAN_POINT ( 'NONE',  ( 17.00008652715106194, 148.0818255213264365, -1.363822447394348991 ) ) ;
#20849=CARTESIAN_POINT ( 'NONE',  ( 3.612019075414997893, 115.7029516305954360, 1.621388860772168039 ) ) ;
#20850=CARTESIAN_POINT ( 'NONE',  ( 2.739926266261139887, -12.91893237176182296, 0.2921503600690461555 ) ) ;
#20851=CARTESIAN_POINT ( 'NONE',  ( -4.806730152592563421, 117.4761099757325269, -1.179797647331112698 ) ) ;
#20852=CARTESIAN_POINT ( 'NONE',  ( 7.800806202324914729, 154.6345575486818404, 0.04849676858278741121 ) ) ;
#20854=CARTESIAN_POINT ( 'NONE',  ( 8.895965109948861027, 157.0267672960688969, 2.032209471265452816 ) ) ;
#20855=CARTESIAN_POINT ( 'NONE',  ( 3.155936729621069858, 108.2677041351691543, 4.292818659978050455 ) ) ;
#20856=AXIS2_PLACEMENT_3D ( 'NONE', #38062, #37423, #14621 ) ;
#20857=CARTESIAN_POINT ( 'NONE',  ( -2.958531772299361595, 50.13146620154573441, -1.329372033065077119 ) ) ;
#20860=AXIS2_PLACEMENT_3D ( 'NONE', #13712, #19879, #32893 ) ;
#20861=CARTESIAN_POINT ( 'NONE',  ( 15.44479738614495901, 120.7004057517279989, 0.1507993925391201140 ) ) ;
#20863=CARTESIAN_POINT ( 'NONE',  ( 1.931211713635406113, -15.24862219501368976, 5.987091862552307298 ) ) ;
#20864=FACE_OUTER_BOUND ( 'NONE', #24458, .T. ) ;
#20865=CARTESIAN_POINT ( 'NONE',  ( 1.957912617769093755, 35.96399040732271857, -0.5992445403938203574 ) ) ;
#20867=CARTESIAN_POINT ( 'NONE',  ( 4.699679879530964222, 158.1906701298835856, 1.765476639684188109 ) ) ;
#20869=CARTESIAN_POINT ( 'NONE',  ( 8.424193198035354158, 17.36166136180145259, -0.6763034115371487909 ) ) ;
#20870=CARTESIAN_POINT ( 'NONE',  ( -5.483011483344768955, 117.5783348333330594, -0.9732951423285314263 ) ) ;
#20871=CARTESIAN_POINT ( 'NONE',  ( -3.014030426305907895, 115.9530684888725460, -1.587286815012125984 ) ) ;
#20874=CARTESIAN_POINT ( 'NONE',  ( -6.374728672999452917E-14, 124.9344662015457317, 7.707042028354222152E-17 ) ) ;
#20876=CARTESIAN_POINT ( 'NONE',  ( -3.640175008984333882, 11.51306413504884318, -2.862805987297033727 ) ) ;
#20878=CARTESIAN_POINT ( 'NONE',  ( -4.772317898405468384, 118.5264896598256854, 0.8398864596484367784 ) ) ;
#20879=CARTESIAN_POINT ( 'NONE',  ( 3.771727509258866906, -13.52648377956064429, 3.452274064300702605 ) ) ;
#20880=CARTESIAN_POINT ( 'NONE',  ( 3.226952561781350592, 118.4615047536228047, -0.6622324852003673712 ) ) ;
#20882=CARTESIAN_POINT ( 'NONE',  ( -1.879194370357706756, 31.42354579518680424, 3.981814511614891305 ) ) ;
#20884=AXIS2_PLACEMENT_3D ( 'NONE', #3984, #33573, #17565 ) ;
#20885=ORIENTED_EDGE ( 'NONE', *, *, #25293, .T. ) ;
#20886=CARTESIAN_POINT ( 'NONE',  ( -4.754641576874411690, 104.6144662015456959, -0.8423218056084632588 ) ) ;
#20887=CARTESIAN_POINT ( 'NONE',  ( 4.918985584458519966, -15.36470173770705649, 0.08744857223284302483 ) ) ;
#20888=CARTESIAN_POINT ( 'NONE',  ( -0.01147819631912393862, 118.5605975114896609, 0.5744158801423954186 ) ) ;
#20889=CARTESIAN_POINT ( 'NONE',  ( -0.9542339719106045504, 13.68595756868040603, 0.2091889690632084686 ) ) ;
#20893=FACE_OUTER_BOUND ( 'NONE', #35697, .T. ) ;
#20895=CARTESIAN_POINT ( 'NONE',  ( 4.585195778441632619, 124.9344662015457459, 0.09162312381275027062 ) ) ;
#20896=CARTESIAN_POINT ( 'NONE',  ( -0.006810764310395450195, 120.3493709785083183, 0.3408384964863782063 ) ) ;
#20898=EDGE_CURVE ( 'NONE', #35171, #32704, #29839, .T. ) ;
#20899=CARTESIAN_POINT ( 'NONE',  ( 4.692195371935813597, 117.9823393671588434, -0.6749937859069751189 ) ) ;
#20900=CARTESIAN_POINT ( 'NONE',  ( 11.57150582532048411, 123.3156264706956478, -1.212837404772455052 ) ) ;
#20901=CARTESIAN_POINT ( 'NONE',  ( -20.10299018766040291, 141.3454246894093274, -2.438971827487009136 ) ) ;
#20905=CARTESIAN_POINT ( 'NONE',  ( 4.250116660506480848, 118.2249359311486643, -0.3102634091937140348 ) ) ;
#20906=CARTESIAN_POINT ( 'NONE',  ( 3.676778326629012827, 120.9289264519876070, -0.1742216996082329161 ) ) ;
#20907=ORIENTED_EDGE ( 'NONE', *, *, #38026, .F. ) ;
#20908=CARTESIAN_POINT ( 'NONE',  ( 2.670684053127368784, -15.04618456763519241, 4.548342027319769443 ) ) ;
#20909=FACE_OUTER_BOUND ( 'NONE', #11610, .T. ) ;
#20910=AXIS2_PLACEMENT_3D ( 'NONE', #26567, #36587, #23349 ) ;
#20912=CARTESIAN_POINT ( 'NONE',  ( -3.074427775304182209, -11.96646105551300643, -3.469969274305642060 ) ) ;
#20913=CARTESIAN_POINT ( 'NONE',  ( 2.572680461994239831, 120.1437993944865354, 0.5932419562244882760 ) ) ;
#20914=CARTESIAN_POINT ( 'NONE',  ( -3.521407940696402505, 28.96769372650263819, 2.403306918834325678 ) ) ;
#20915=CARTESIAN_POINT ( 'NONE',  ( -5.259129974998975499, 118.7524313932052991, 0.4270625282899582764 ) ) ;
#20916=CARTESIAN_POINT ( 'NONE',  ( 2.551540157903699146, -0.3564265548712530207, -3.854280124997286450 ) ) ;
#20917=CARTESIAN_POINT ( 'NONE',  ( 7.796516423212079161, 154.6345575486818404, 0.2631748570402916432 ) ) ;
#20920=CARTESIAN_POINT ( 'NONE',  ( 8.795815767003183794, 117.7122569620870962, 0.001127142753954061974 ) ) ;
#20923=CARTESIAN_POINT ( 'NONE',  ( -0.1064799869811723365, 105.7853621660184444, 5.332934571178563843 ) ) ;
#20925=CARTESIAN_POINT ( 'NONE',  ( 8.109546976224176973, 7.201272144248561879, 2.403482862635152539 ) ) ;
#20927=PLANE ( 'NONE',  #31397 ) ;
#20929=CARTESIAN_POINT ( 'NONE',  ( 0.0006472084742222537247, 124.6436471961814476, -0.03238895860161178364 ) ) ;
#20930=CARTESIAN_POINT ( 'NONE',  ( -23.16228472148477380, 149.2833505036244048, 0.1324855245534191928 ) ) ;
#20934=ORIENTED_EDGE ( 'NONE', *, *, #17108, .T. ) ;
#20936=CARTESIAN_POINT ( 'NONE',  ( -2.836071964827412639, 121.0300505300837415, -0.05667146733340956699 ) ) ;
#20937=CARTESIAN_POINT ( 'NONE',  ( 4.377062889037126148, -14.98224217357194199, 4.840108967533193862 ) ) ;
#20938=CARTESIAN_POINT ( 'NONE',  ( -12.83522892222240053, 121.3369795956499928, 1.134461614517290551 ) ) ;
#20940=CARTESIAN_POINT ( 'NONE',  ( 14.56950268504896151, 121.1548589120785095, -0.7262516135598524603 ) ) ;
#20942=CARTESIAN_POINT ( 'NONE',  ( -13.56676737375339137, 119.6371495169912436, -0.4909217195147885238 ) ) ;
#20944=ORIENTED_EDGE ( 'NONE', *, *, #14881, .F. ) ;
#20946=CARTESIAN_POINT ( 'NONE',  ( -6.603469437764838190, 120.5225452898634728, 0.8609044167644233081 ) ) ;
#20949=CARTESIAN_POINT ( 'NONE',  ( 18.66004122726566195, 149.2887123452801745, -1.736808470001686810 ) ) ;
#20950=CARTESIAN_POINT ( 'NONE',  ( -14.23594795111950084, 121.8555783441548073, -1.592150851459066319 ) ) ;
#20954=CARTESIAN_POINT ( 'NONE',  ( 2.657114488131237628, 120.4390018212493914, -0.3871174720959879578 ) ) ;
#20955=CARTESIAN_POINT ( 'NONE',  ( 7.788927721206574617, 122.5994874646387984, 0.3062633923827431381 ) ) ;
#20957=CARTESIAN_POINT ( 'NONE',  ( -11.70444740893367275, 123.2143981803894093, -1.719255905491489544 ) ) ;
#20958=CARTESIAN_POINT ( 'NONE',  ( 4.348370292662268710, -15.56902811939260545, 2.317716755344581880 ) ) ;
#20960=DIRECTION ( 'NONE',  ( -4.017660918040594346E-17, 1.000000000000000000, 2.376309959284832031E-19 ) ) ;
#20961=CARTESIAN_POINT ( 'NONE',  ( -4.266443719422126968, 118.2131497807364724, -0.5314359833645941888 ) ) ;
#20963=CARTESIAN_POINT ( 'NONE',  ( -4.975714317725813629, 117.5352226273689240, 0.7922778689861946777 ) ) ;
#20964=CARTESIAN_POINT ( 'NONE',  ( 16.10024230344501461, 135.1141785778430346, 2.240991319914668711 ) ) ;
#20966=CARTESIAN_POINT ( 'NONE',  ( 18.81756541077860589, 125.3161215262879580, 0.3201835051929645126 ) ) ;
#20968=CARTESIAN_POINT ( 'NONE',  ( 6.048790893839320226, 16.06121166075865148, 5.875566521300903844 ) ) ;
#20969=CARTESIAN_POINT ( 'NONE',  ( 14.79492108907963477, 148.8567844064068026, 0.8802232212986721427 ) ) ;
#20973=CIRCLE ( 'NONE', #31880, 0.5080000000000002292 ) ;
#20976=CARTESIAN_POINT ( 'NONE',  ( -9.807059279560077059, 117.9968303279965340, -0.1034500883390724879 ) ) ;
#20979=CARTESIAN_POINT ( 'NONE',  ( 7.917148831097427397, 122.0549026337326808, -0.5915961107884312176 ) ) ;
#20980=FACE_BOUND ( 'NONE', #26313, .T. ) ;
#20982=CARTESIAN_POINT ( 'NONE',  ( 0.5726544197577119188, 115.7031858585135637, -1.740669147351574075 ) ) ;
#20983=CARTESIAN_POINT ( 'NONE',  ( -15.75631923737921092, 146.9135488020124001, -0.6449975968329648701 ) ) ;
#20984=CARTESIAN_POINT ( 'NONE',  ( 4.871446434089309108, -12.86987818651588711, 2.618604111146097591 ) ) ;
#20985=CARTESIAN_POINT ( 'NONE',  ( -7.412489149516535036, 158.3992165788449711, 1.135539963648920070 ) ) ;
#20986=CARTESIAN_POINT ( 'NONE',  ( 1.627035472719924547, 117.3993836203816556, -1.397827203978000865 ) ) ;
#20987=CARTESIAN_POINT ( 'NONE',  ( 2.764936593379123675, 116.5678055239024644, 0.1631480333911173308 ) ) ;
#20988=CARTESIAN_POINT ( 'NONE',  ( 8.739549413732950356, 123.6764625261342587, 0.2181624419688201200 ) ) ;
#20990=CARTESIAN_POINT ( 'NONE',  ( 0.2723526006440308844, 25.78125159710042169, 0.9401034630801221592 ) ) ;
#20991=CARTESIAN_POINT ( 'NONE',  ( -23.11076619426189538, 149.9001102426712748, -0.4874744954944869590 ) ) ;
#20996=CARTESIAN_POINT ( 'NONE',  ( -8.335421588164685147, 120.0665240995501364, 1.118669443656532758 ) ) ;
#20997=CARTESIAN_POINT ( 'NONE',  ( 4.571311019248293306, -6.119132638730012452, 0.7325351754658009362 ) ) ;
#20998=CARTESIAN_POINT ( 'NONE',  ( 13.94627971010872614, 121.2764344996515717, 1.482775695869144705 ) ) ;
#21000=CARTESIAN_POINT ( 'NONE',  ( 1.145842520592908365, 158.4310823543925721, -1.558676969884219332 ) ) ;
#21001=CARTESIAN_POINT ( 'NONE',  ( 2.990331240142678482, -7.206181497205274233, 3.547999066060627094 ) ) ;
#21002=CARTESIAN_POINT ( 'NONE',  ( -6.860783072103511238, 117.8105958006179890, -0.8866969874100999460 ) ) ;
#21003=CARTESIAN_POINT ( 'NONE',  ( 4.975302499479774987, 117.5352015494678142, -0.7925089078733521530 ) ) ;
#21004=EDGE_CURVE ( 'NONE', #24227, #36646, #26466, .T. ) ;
#21006=CARTESIAN_POINT ( 'NONE',  ( -9.747124062405315925, 124.8671652961716489, 0.04776528062357104226 ) ) ;
#21008=CARTESIAN_POINT ( 'NONE',  ( 2.113928706699719218, -15.46215275738946282, 5.949113654003534535 ) ) ;
#21010=DIRECTION ( 'NONE',  ( 0.9998004120163608288, 0.000000000000000000, 0.01997839162482749342 ) ) ;
#21012=CARTESIAN_POINT ( 'NONE',  ( 4.155191945500637196, 119.0775769483117870, 1.003333751211267888 ) ) ;
#21015=CARTESIAN_POINT ( 'NONE',  ( -3.898136962790746285, 117.1932757116604762, 0.4670938640342006676 ) ) ;
#21016=CARTESIAN_POINT ( 'NONE',  ( 6.464508713081113633, 4.871470569706378484, -5.424950676754816570 ) ) ;
#21017=CARTESIAN_POINT ( 'NONE',  ( 13.80305775881199537, 134.3516747369166069, 1.357216474725372768 ) ) ;
#21019=CARTESIAN_POINT ( 'NONE',  ( 10.65151157945274996, 157.9324367681937815, -0.3596066298475817935 ) ) ;
#21020=DIRECTION ( 'NONE',  ( 4.017660918040594346E-17, -1.000000000000000000, -2.376309959284834438E-19 ) ) ;
#21026=CARTESIAN_POINT ( 'NONE',  ( -4.122399503745135974, 118.2429491485453497, 0.1816704820238574380 ) ) ;
#21027=CARTESIAN_POINT ( 'NONE',  ( 3.324910422824467915, 108.2677041351605141, -4.163315910313021284 ) ) ;
#21028=EDGE_LOOP ( 'NONE', ( #25216, #1300 ) ) ;
#21031=CARTESIAN_POINT ( 'NONE',  ( -4.092897794381019416, 119.2344987732284807, -0.9253235121601953717 ) ) ;
#21033=CARTESIAN_POINT ( 'NONE',  ( 0.1065646865915093611, 105.8844662015456777, -5.332932678536313809 ) ) ;
#21034=CARTESIAN_POINT ( 'NONE',  ( 4.441684112726699496, 118.1590229626581419, 0.6063474506374556539 ) ) ;
#21035=CARTESIAN_POINT ( 'NONE',  ( -9.461503173624157270, 123.8597080710187015, -0.7891915900027407504 ) ) ;
#21036=CARTESIAN_POINT ( 'NONE',  ( 0.3668836553635324571, 118.1651003658195833, -0.8808146135302142854 ) ) ;
#21038=CARTESIAN_POINT ( 'NONE',  ( 3.211436584971100849, 28.15539441671475274, -3.345526564039049688 ) ) ;
#21039=CARTESIAN_POINT ( 'NONE',  ( -2.605661685743515310, 120.2926465633240127, -0.5460719465365780900 ) ) ;
#21043=CARTESIAN_POINT ( 'NONE',  ( -8.838968381400917451, 123.8898104212950670, -0.04432116756960934739 ) ) ;
#21044=CARTESIAN_POINT ( 'NONE',  ( -6.263959367015712765, 28.84083519579221999, 0.1566845698765544637 ) ) ;
#21045=CARTESIAN_POINT ( 'NONE',  ( 9.626009506019130413, 118.2334930433176652, 0.7695227696168691622 ) ) ;
#21047=CARTESIAN_POINT ( 'NONE',  ( 2.350639260211558668, -15.10312717587823705, 4.966175652281853203 ) ) ;
#21048=CARTESIAN_POINT ( 'NONE',  ( 3.062634247293183787, 117.6993298527280984, -0.6308921261198919828 ) ) ;
#21049=CARTESIAN_POINT ( 'NONE',  ( -5.904616261062859195, 156.9788419092994047, 1.696979819435221470 ) ) ;
#21050=CARTESIAN_POINT ( 'NONE',  ( 0.4928529169951482158, -8.289340824275994279, 0.8415213476199340237 ) ) ;
#21051=CARTESIAN_POINT ( 'NONE',  ( -8.152918552588374723, 117.7057695168643932, -0.6423243676978416250 ) ) ;
#21052=CARTESIAN_POINT ( 'NONE',  ( 0.4517697234110209514, 20.42248995698831493, 0.8659212905253524939 ) ) ;
#21053=ORIENTED_EDGE ( 'NONE', *, *, #8699, .T. ) ;
#21055=CARTESIAN_POINT ( 'NONE',  ( -9.439557112687712248, 123.9587481073520223, 0.3264598115655272248 ) ) ;
#21056=CARTESIAN_POINT ( 'NONE',  ( 2.266344692909419312, -15.23424214381746644, 5.932772278557574275 ) ) ;
#21057=CARTESIAN_POINT ( 'NONE',  ( 5.874057931648818176, 120.5744318282211651, -0.7168624585904721513 ) ) ;
#21059=CARTESIAN_POINT ( 'NONE',  ( 2.094145466755243934, 115.7021055795812572, 1.712902155792607406 ) ) ;
#21060=CARTESIAN_POINT ( 'NONE',  ( 3.215637690559757456, -14.25221971482225314, 3.321654998001884795 ) ) ;
#21061=CARTESIAN_POINT ( 'NONE',  ( -4.781726760622166061, 117.4742263818998680, -1.189410900997683651 ) ) ;
#21062=CARTESIAN_POINT ( 'NONE',  ( 7.567922279963275045, 122.4257779438054285, 0.07478732235760103542 ) ) ;
#21065=CARTESIAN_POINT ( 'NONE',  ( 10.23541510771056906, 120.3038588096988803, 1.551695437301547242 ) ) ;
#21066=CARTESIAN_POINT ( 'NONE',  ( 4.038844528162431224, 111.0901538136610611, 3.207827241414232144 ) ) ;
#21069=CARTESIAN_POINT ( 'NONE',  ( -6.426369768295692736E-14, 159.6054662015457382, 1.032716915552223178E-16 ) ) ;
#21070=CARTESIAN_POINT ( 'NONE',  ( 16.83721787035668171, 155.2408147041404050, 0.1288212628531383852 ) ) ;
#21072=CARTESIAN_POINT ( 'NONE',  ( 1.720506426491690055, -15.42054776992238274, 5.887968618877454041 ) ) ;
#21074=CARTESIAN_POINT ( 'NONE',  ( -2.938663822924134639, 31.60055309655552946, 0.8891835726407014695 ) ) ;
#21075=CARTESIAN_POINT ( 'NONE',  ( -4.818183171710055390, 117.8426606599154667, 0.7484465901436401225 ) ) ;
#21077=CARTESIAN_POINT ( 'NONE',  ( 5.586884702347363785, 104.6144662015457243, 0.1116392523995368424 ) ) ;
#21079=CARTESIAN_POINT ( 'NONE',  ( -5.733800310741941963, 118.6806198687866214, -1.226522746645787088 ) ) ;
#21080=CARTESIAN_POINT ( 'NONE',  ( -0.8148005656458301438, 107.7619142660649203, -4.566897024910153924 ) ) ;
#21081=CARTESIAN_POINT ( 'NONE',  ( 4.940360603511367188, 117.5341859490524996, 0.9905126371005529284 ) ) ;
#21083=CARTESIAN_POINT ( 'NONE',  ( -0.01046636458954068247, 120.7331730230139755, 0.5237796829256087250 ) ) ;
#21084=CARTESIAN_POINT ( 'NONE',  ( 4.523211737919912601, 7.414965188139293950, 0.9565071382433593117 ) ) ;
#21086=CARTESIAN_POINT ( 'NONE',  ( -5.031308904535771731, 113.7220012594890619, -1.867310441168415158 ) ) ;
#21087=B_SPLINE_CURVE_WITH_KNOTS ( 'NONE', 3,
 ( #6767, #13578, #3799, #32755, #19322, #35742, #32326, #6146, #3155, #16761, #29768 ),
 .UNSPECIFIED., .F., .F.,
 ( 4, 1, 1, 1, 1, 1, 1, 1, 4 ),
 ( 0.000000000000000000, 0.1250000000000006939, 0.2500000000000013878, 0.3750000000000020539, 0.5000000000000027756, 0.6250000000000061062, 0.7499999999999986677, 0.8750000000000019984, 1.000000000000000000 ),
 .UNSPECIFIED. ) ;
#21088=CARTESIAN_POINT ( 'NONE',  ( 3.509037099356659084, -13.47856448578629873, 2.732507022889707038 ) ) ;
#21089=CARTESIAN_POINT ( 'NONE',  ( 3.375001179497614689, 119.3320731715853782, -0.4843141097021076980 ) ) ;
#21090=CARTESIAN_POINT ( 'NONE',  ( 2.383981540283352629, 36.81846344528510429, 1.803752045214197297 ) ) ;
#21091=CARTESIAN_POINT ( 'NONE',  ( -0.7849891123721223218, 115.7029491485453434, 1.726829941792507483 ) ) ;
#21092=ORIENTED_EDGE ( 'NONE', *, *, #32590, .T. ) ;
#21094=CARTESIAN_POINT ( 'NONE',  ( 1.925067723532086994, -15.61332249492565438, 5.452854070638914585 ) ) ;
#21095=CARTESIAN_POINT ( 'NONE',  ( -1.091998727716720241, 158.1148137021529578, 1.603323485041850294 ) ) ;
#21096=CARTESIAN_POINT ( 'NONE',  ( 0.4504873307288463358, 16.48674109716143477, 0.8651787211232140340 ) ) ;
#21097=ADVANCED_FACE ( 'NONE', ( #30520 ), #26956, .F. ) ;
#21100=CARTESIAN_POINT ( 'NONE',  ( -4.112981969563189288, 27.92417664812854738, 0.5059177812967017296 ) ) ;
#21101=CARTESIAN_POINT ( 'NONE',  ( 2.258874542396673846, 118.3648483361698851, 0.8858652710056679203 ) ) ;
#21102=CARTESIAN_POINT ( 'NONE',  ( -16.33516936551327703, 148.1602266505728380, 1.109112510451941924 ) ) ;
#21104=CARTESIAN_POINT ( 'NONE',  ( 4.732466489211092586, 117.9644445172183538, -0.6135672020651322667 ) ) ;
#21105=CARTESIAN_POINT ( 'NONE',  ( 7.569905091580497292, 156.0351187175861867, -1.610277000873165054 ) ) ;
#21106=CARTESIAN_POINT ( 'NONE',  ( -15.97272115206789955, 153.3736753708079732, -2.320099718173297187 ) ) ;
#21109=CARTESIAN_POINT ( 'NONE',  ( 4.248835768063355722, 118.2248660469010559, -0.3116667286827642380 ) ) ;
#21110=CARTESIAN_POINT ( 'NONE',  ( 13.73699108721713458, 150.2158912636999730, -0.3005180155469768244 ) ) ;
#21112=CARTESIAN_POINT ( 'NONE',  ( 2.349528287245666647, -15.15257587461875310, 4.947206973663434759 ) ) ;
#21115=CARTESIAN_POINT ( 'NONE',  ( -4.603752034695621553, -0.9465464349810851497, 0.4006815057252178236 ) ) ;
#21116=CARTESIAN_POINT ( 'NONE',  ( 12.90748236152450623, 128.4900567078429390, 1.625332807165861260 ) ) ;
#21117=CARTESIAN_POINT ( 'NONE',  ( 2.971218050981001113, 39.20946620154573736, 0.6944987714346865237 ) ) ;
#21118=CARTESIAN_POINT ( 'NONE',  ( -4.048024155119399836, 117.4230540797109938, 0.8140401526052126746 ) ) ;
#21119=CARTESIAN_POINT ( 'NONE',  ( -3.426874451426485724, 1.805113900313119357, -3.130497002818263930 ) ) ;
#21120=CARTESIAN_POINT ( 'NONE',  ( 11.85559104777363082, 130.3381101163291760, 0.2804367443601422649 ) ) ;
#21124=CARTESIAN_POINT ( 'NONE',  ( 2.170629307524321927, 116.6785980183682625, -0.3802400742865192917 ) ) ;
#21127=CARTESIAN_POINT ( 'NONE',  ( 1.824656174747253168, -15.25388738520313225, 5.420764384989097628 ) ) ;
#21128=CARTESIAN_POINT ( 'NONE',  ( 4.559522851259544041, 6.111780172613243245, 7.100340242056582873 ) ) ;
#21129=CARTESIAN_POINT ( 'NONE',  ( 5.332923298845091864, 115.7029491485453150, 0.1071700043820369153 ) ) ;
#21131=CARTESIAN_POINT ( 'NONE',  ( 2.102813808753936087, -15.18136450426021256, 5.202461169095355942 ) ) ;
#21132=CARTESIAN_POINT ( 'NONE',  ( 0.07831152689291247249, 109.4728569552520838, -3.919029035233798641 ) ) ;
#21133=CARTESIAN_POINT ( 'NONE',  ( -0.9570688389944551622, 116.7004868406603322, 0.2253703713229212591 ) ) ;
#21134=VERTEX_POINT ( 'NONE', #31047 ) ;
#21139=CARTESIAN_POINT ( 'NONE',  ( -10.39928917620371784, 153.1223395828141918, -0.2078025466733117443 ) ) ;
#21140=CARTESIAN_POINT ( 'NONE',  ( 3.037190435423921642, -15.45437603076259236, 5.639675387367293347 ) ) ;
#21141=CARTESIAN_POINT ( 'NONE',  ( -2.760819571866494293, 158.5977336698458089, 1.488126253378572406 ) ) ;
#21142=CARTESIAN_POINT ( 'NONE',  ( 21.83270838041246975, 150.5404744109896171, -0.8586010584139893709 ) ) ;
#21143=CARTESIAN_POINT ( 'NONE',  ( -4.191205975170537279, 21.45845178295031630, -1.961646697876042511 ) ) ;
#21144=CARTESIAN_POINT ( 'NONE',  ( -13.43369120214920365, 119.6710471929552000, -0.6668731667128946494 ) ) ;
#21149=CARTESIAN_POINT ( 'NONE',  ( -5.873575024772843101, 120.4133487461328826, 0.7716123655894260303 ) ) ;
#21150=CARTESIAN_POINT ( 'NONE',  ( 5.078986093043053707, 98.39146620154573952, 0.1014902294541244060 ) ) ;
#21151=CARTESIAN_POINT ( 'NONE',  ( 6.044862153450403675, 157.1185343457808301, -1.711190705598350403 ) ) ;
#21152=CARTESIAN_POINT ( 'NONE',  ( -1.092003032498587212, 117.6437429425539420, -0.5722403007656916563 ) ) ;
#21154=ADVANCED_FACE ( 'NONE', ( #1886 ), #6071, .F. ) ;
#21155=CARTESIAN_POINT ( 'NONE',  ( 10.90887028606290876, 153.1125297277760069, -0.8016274872379887118 ) ) ;
#21157=CARTESIAN_POINT ( 'NONE',  ( -11.19992112824931496, 154.5781333488962446, -2.119767339128325823 ) ) ;
#21158=CARTESIAN_POINT ( 'NONE',  ( 4.206901174280650579, -15.33509931759592604, 0.05204670666830889247 ) ) ;
#21159=CARTESIAN_POINT ( 'NONE',  ( -4.444388996687162141, 118.1581009083410976, -0.6033315295914259968 ) ) ;
#21161=CARTESIAN_POINT ( 'NONE',  ( -4.971548125946218200, 117.4753602155310404, 0.8635831801788802498 ) ) ;
#21162=CARTESIAN_POINT ( 'NONE',  ( 11.03566430468803361, 123.0430266451958232, 1.599512106649902510 ) ) ;
#21163=EDGE_CURVE ( 'NONE', #30281, #24814, #8097, .T. ) ;
#21164=FACE_OUTER_BOUND ( 'NONE', #41645, .T. ) ;
#21166=CARTESIAN_POINT ( 'NONE',  ( 23.11179153581189993, 149.9001102426712748, 0.4361622115260940236 ) ) ;
#21167=CARTESIAN_POINT ( 'NONE',  ( -3.982871878373832164, -5.105173558950587775, 7.419718595111914894 ) ) ;
#21168=CARTESIAN_POINT ( 'NONE',  ( 9.239529650026105045, 153.8817031120973411, 0.7017441744976311568 ) ) ;
#21172=CARTESIAN_POINT ( 'NONE',  ( -2.802975543813512882, 117.9394509414842531, 1.218220532187687999 ) ) ;
#21174=CARTESIAN_POINT ( 'NONE',  ( 3.946153427423682469, 118.7629491485453741, 1.103408776148272930 ) ) ;
#21175=ADVANCED_FACE ( 'NONE', ( #34467 ), #315, .T. ) ;
#21178=CARTESIAN_POINT ( 'NONE',  ( -15.18069129733363098, 156.1124880001465556, -0.1695137023582057034 ) ) ;
#21181=CARTESIAN_POINT ( 'NONE',  ( 7.883489662030576994, 122.2086137271560062, -0.4845574022495899302 ) ) ;
#21182=CARTESIAN_POINT ( 'NONE',  ( -8.060916924639437653, 121.3839393899242936, 0.8986322262797288296 ) ) ;
#21183=CARTESIAN_POINT ( 'NONE',  ( 0.02551629667430791934, 118.7629491485454025, -1.276939826302095682 ) ) ;
#21184=CARTESIAN_POINT ( 'NONE',  ( -12.03016689884997525, 130.4833683797432684, -0.5359549021282030701 ) ) ;
#21185=CARTESIAN_POINT ( 'NONE',  ( 2.867264926914522949, -14.81558118910870903, 5.578245215537346979 ) ) ;
#21187=CARTESIAN_POINT ( 'NONE',  ( -5.164160201466208022, 158.7070047875298826, 1.240540739692759020 ) ) ;
#21188=FACE_OUTER_BOUND ( 'NONE', #6933, .T. ) ;
#21189=AXIS2_PLACEMENT_3D ( 'NONE', #41276, #24429, #12082 ) ;
#21190=CARTESIAN_POINT ( 'NONE',  ( 9.792313404876027860, 118.0024801742749929, 0.3345192158099828950 ) ) ;
#21191=CARTESIAN_POINT ( 'NONE',  ( 15.52593806990746472, 147.5347896062808957, 0.3770146343057313443 ) ) ;
#21193=CARTESIAN_POINT ( 'NONE',  ( -0.9394305312890779414, 22.53537758578342931, -0.2615529312561373776 ) ) ;
#21194=CARTESIAN_POINT ( 'NONE',  ( -1.421330246821875587, 159.6054662015457666, -0.04208995589191817654 ) ) ;
#21199=ORIENTED_EDGE ( 'NONE', *, *, #1448, .F. ) ;
#21200=CARTESIAN_POINT ( 'NONE',  ( -3.563367352916122499, 117.8600736429027478, 0.7435805097010282916 ) ) ;
#21201=CARTESIAN_POINT ( 'NONE',  ( -5.327983418387242764, 105.1224763138612843, 0.2702714856519077280 ) ) ;
#21202=CARTESIAN_POINT ( 'NONE',  ( 21.61975215418284790, 149.3076860495818323, 2.139488579489919218 ) ) ;
#21204=CARTESIAN_POINT ( 'NONE',  ( 20.06821085608255473, 149.3093937917295762, -1.664735353294634068 ) ) ;
#21205=CARTESIAN_POINT ( 'NONE',  ( -5.272568914482754998, 19.56627864152888208, 6.568537450970175939 ) ) ;
#21206=CARTESIAN_POINT ( 'NONE',  ( -22.55218723263380909, 148.5212373274837319, -1.758973660241909487 ) ) ;
#21207=CARTESIAN_POINT ( 'NONE',  ( 4.933441418498765607, 117.6566197977928852, -0.7552850541079862978 ) ) ;
#21209=CARTESIAN_POINT ( 'NONE',  ( -15.77919907218852025, 145.7191243368997675, 0.01646358168407728237 ) ) ;
#21210=CARTESIAN_POINT ( 'NONE',  ( 6.028374245061780989, -14.54558069259788411, 1.726931113533916040 ) ) ;
#21215=CARTESIAN_POINT ( 'NONE',  ( 6.656653968793884601, 119.6463993818898359, 1.283952750486249794 ) ) ;
#21217=CARTESIAN_POINT ( 'NONE',  ( -3.682264917456323783, 85.18346620154574111, -0.07358041635423968885 ) ) ;
#21218=CARTESIAN_POINT ( 'NONE',  ( -3.315449255180983545, 124.9344662015457743, -0.06625056644921972770 ) ) ;
#21219=CARTESIAN_POINT ( 'NONE',  ( -5.217102898550305845, -11.97038331068927342, -6.647077075081065267 ) ) ;
#21220=CARTESIAN_POINT ( 'NONE',  ( 9.561025033427959841, 123.8224200044116827, 0.8726585919039498984 ) ) ;
#21221=CARTESIAN_POINT ( 'NONE',  ( -4.787902336757507094, 118.5930653697794384, -0.9393770334760460639 ) ) ;
#21222=CARTESIAN_POINT ( 'NONE',  ( 15.31827776641168271, 121.1074504348956964, -0.3839962087354598652 ) ) ;
#21226=EDGE_CURVE ( 'NONE', #30442, #26111, #639, .T. ) ;
#21228=CARTESIAN_POINT ( 'NONE',  ( -6.538677740023618411E-14, 75.27746620154573520, -7.356392042280733227E-18 ) ) ;
#21229=CARTESIAN_POINT ( 'NONE',  ( -4.270517806291405982, 118.2236137968261716, 0.2873848592035506688 ) ) ;
#21230=AXIS2_PLACEMENT_3D ( 'NONE', #5229, #8618, #37377 ) ;
#21232=ORIENTED_EDGE ( 'NONE', *, *, #40967, .T. ) ;
#21234=CARTESIAN_POINT ( 'NONE',  ( -6.140969379225402314, 119.6263759229288155, -1.248624756452694884 ) ) ;
#21236=CARTESIAN_POINT ( 'NONE',  ( 4.226304903563289805, 118.2242387644281365, 0.4878455849994780547 ) ) ;
#21237=CARTESIAN_POINT ( 'NONE',  ( -6.479597433594425304, 121.6155390319085683, -0.5171962410403524446 ) ) ;
#21241=CARTESIAN_POINT ( 'NONE',  ( -0.3239230800893593276, 29.42979164457532804, -4.628216972995994993 ) ) ;
#21242=CARTESIAN_POINT ( 'NONE',  ( -16.69533394573253915, 146.9696287467501179, -1.777152765835339654 ) ) ;
#21246=CARTESIAN_POINT ( 'NONE',  ( 6.071556415024221387, 121.4181341445724911, 0.3301129433361331689 ) ) ;
#21247=CARTESIAN_POINT ( 'NONE',  ( -0.2796867633624597893, 20.41853924017881283, 4.627572958784220702 ) ) ;
#21248=CARTESIAN_POINT ( 'NONE',  ( 15.26873630740953480, 121.3917326167944708, 1.149126527656483265 ) ) ;
#21250=CARTESIAN_POINT ( 'NONE',  ( 2.856221160286674277, -14.96258862872340600, 4.237710179968991575 ) ) ;
#21251=CARTESIAN_POINT ( 'NONE',  ( 21.00062727315619782, 150.0074445146613584, -1.385517290469731044 ) ) ;
#21252=CARTESIAN_POINT ( 'NONE',  ( -11.86655615995746693, 122.9427978038690270, 1.277170931065712667 ) ) ;
#21253=CARTESIAN_POINT ( 'NONE',  ( -4.137704358559117779, 17.39492794009094823, -2.099109474953318788 ) ) ;
#21254=CARTESIAN_POINT ( 'NONE',  ( -1.924101685567954689, 116.8467566806161386, -0.3833193769953582852 ) ) ;
#21256=CARTESIAN_POINT ( 'NONE',  ( -0.01433812918766144522, 10.07226683256953947, 0.9740319587662029654 ) ) ;
#21259=CARTESIAN_POINT ( 'NONE',  ( -1.677891416185295803, 156.3096136994911092, 0.5101806352362401320 ) ) ;
#21260=CARTESIAN_POINT ( 'NONE',  ( 5.886196856236641572, -12.36517754215322995, 0.8550893866892870232 ) ) ;
#21261=CARTESIAN_POINT ( 'NONE',  ( 17.27635908418598021, 147.1820577694790018, -1.364000445115660654 ) ) ;
#21263=CARTESIAN_POINT ( 'NONE',  ( 1.783695439853289377, 115.7029489856815019, 1.723415406732235811 ) ) ;
#21265=VERTEX_POINT ( 'NONE', #38710 ) ;
#21266=CARTESIAN_POINT ( 'NONE',  ( 3.381076509412870301, -13.31623885458479961, 2.121725202727857695 ) ) ;
#21267=CARTESIAN_POINT ( 'NONE',  ( -4.830385371082315693, 117.7605833166150404, -0.9792491193852199682 ) ) ;
#21268=CARTESIAN_POINT ( 'NONE',  ( 0.6421132086018013219, 120.9975462804897433, -0.01250379197263685321 ) ) ;
#21271=CARTESIAN_POINT ( 'NONE',  ( 7.739031927414979251, 119.2688035297948659, 1.343379870322972458 ) ) ;
#21274=CARTESIAN_POINT ( 'NONE',  ( 0.004910662370358964517, 159.5928157220454295, -0.2457496255665020946 ) ) ;
#21275=CARTESIAN_POINT ( 'NONE',  ( 5.806485631242116696, 116.9771394561422539, -0.05772921648981169107 ) ) ;
#21277=AXIS2_PLACEMENT_3D ( 'NONE', #20002, #36002, #26188 ) ;
#21278=CARTESIAN_POINT ( 'NONE',  ( 1.643874335733584768, -15.34739276353720783, 5.606459198667521626 ) ) ;
#21281=CARTESIAN_POINT ( 'NONE',  ( -4.706055329038499657, 117.9791134883193848, 0.6571109466785158837 ) ) ;
#21282=ORIENTED_EDGE ( 'NONE', *, *, #38382, .T. ) ;
#21285=CARTESIAN_POINT ( 'NONE',  ( 8.584051096561029937, 118.8309510801975932, -0.8814915625618818806 ) ) ;
#21286=CARTESIAN_POINT ( 'NONE',  ( -4.467639297143111143, 123.9529229959338608, -0.1358511699341444778 ) ) ;
#21287=CARTESIAN_POINT ( 'NONE',  ( 4.868692240912165126, 117.7191721330082572, 0.9439216475803462458 ) ) ;
#21289=CARTESIAN_POINT ( 'NONE',  ( -0.7907195946117820951, 120.5370721568272216, 0.4966358104988965461 ) ) ;
#21291=CARTESIAN_POINT ( 'NONE',  ( -0.8472427164685307766, -8.777537934218566207, -4.544909406875613733 ) ) ;
#21292=CARTESIAN_POINT ( 'NONE',  ( 4.997288873896878592, 117.4043910709748104, -0.8233982764724142589 ) ) ;
#21294=CARTESIAN_POINT ( 'NONE',  ( 3.107604131292615257, -12.52806217606054773, 0.6782401946156415562 ) ) ;
#21295=CARTESIAN_POINT ( 'NONE',  ( 2.433495328593811902, 107.4436264546101967, -4.557236999380250175 ) ) ;
#21296=CARTESIAN_POINT ( 'NONE',  ( -0.9149567752697735923, 32.47697140010484418, 3.785418454572507141 ) ) ;
#21297=CARTESIAN_POINT ( 'NONE',  ( -0.6166778457948044467, 115.7029855731295811, 1.738056368063223944 ) ) ;
#21298=CARTESIAN_POINT ( 'NONE',  ( 3.400481176189167343, 25.78150505744974552, 3.158589348000393482 ) ) ;
#21300=CARTESIAN_POINT ( 'NONE',  ( -5.282606327573863503, 104.6144662015414184, -0.7587477978234113962 ) ) ;
#21301=CARTESIAN_POINT ( 'NONE',  ( 3.676215660907734328, -15.61639409997438221, 3.572853394304201569 ) ) ;
#21302=CARTESIAN_POINT ( 'NONE',  ( -17.46034360794361007, 151.5007859583534753, 1.733980983366192552 ) ) ;
#21303=CARTESIAN_POINT ( 'NONE',  ( 0.7683055643446228267, 21.07255974867073078, 0.6014680952941496850 ) ) ;
#21304=CARTESIAN_POINT ( 'NONE',  ( -0.6395729929254629909, 24.25746453972198680, 0.7366970655621520869 ) ) ;
#21305=ORIENTED_EDGE ( 'NONE', *, *, #12262, .T. ) ;
#21307=CARTESIAN_POINT ( 'NONE',  ( 0.7055264248721295761, 108.7514562038770976, 4.178308661695779413 ) ) ;
#21308=CARTESIAN_POINT ( 'NONE',  ( -6.522410937005572507, 121.2869106855140018, 0.5334890203407733900 ) ) ;
#21310=CARTESIAN_POINT ( 'NONE',  ( 4.687054664522481318, 118.0074822305351319, -0.5902932124156423654 ) ) ;
#21311=CARTESIAN_POINT ( 'NONE',  ( 14.27712035414119107, 128.5469532985352714, -1.439506347022430299 ) ) ;
#21313=CARTESIAN_POINT ( 'NONE',  ( -20.07331991451315645, 148.0303212619860744, -2.505472171123445335 ) ) ;
#21315=CARTESIAN_POINT ( 'NONE',  ( -6.441001096823943506, 29.32969738650800551, -0.01017983961634279927 ) ) ;
#21317=CARTESIAN_POINT ( 'NONE',  ( 9.493134470504843492, 124.1929984354129175, -0.2364027771656554699 ) ) ;
#21319=CARTESIAN_POINT ( 'NONE',  ( 3.028202472743143581, -14.11696900735987015, 1.123381337427139526 ) ) ;
#21322=CARTESIAN_POINT ( 'NONE',  ( 4.264856162967361364, -5.269518785209044154, -1.792273654951743067 ) ) ;
#21323=CARTESIAN_POINT ( 'NONE',  ( 3.288791919378179163, 156.3062290909284116, 1.149731754608032785 ) ) ;
#21324=CARTESIAN_POINT ( 'NONE',  ( -2.690315046239569075, 30.48488075981191159, 3.827843980145978264 ) ) ;
#21325=CARTESIAN_POINT ( 'NONE',  ( -4.642736441617746124, 114.7252160460498516, 1.690332539979629622 ) ) ;
#21327=CARTESIAN_POINT ( 'NONE',  ( -3.998286381996895233, 3.741657206818807424, 2.332027183294827832 ) ) ;
#21328=CARTESIAN_POINT ( 'NONE',  ( 6.499560145427067503, 121.7799842514348541, 0.1589113151347880393 ) ) ;
#21329=CARTESIAN_POINT ( 'NONE',  ( 8.368836169178564433, 3.587476746713724740, 1.217019533931793074 ) ) ;
#21331=CARTESIAN_POINT ( 'NONE',  ( 5.529029624460691572, 116.9734914006921684, -0.4280831465535851477 ) ) ;
#21334=CARTESIAN_POINT ( 'NONE',  ( 5.274109024393328404, 115.7029491485453150, -0.8140283081321303404 ) ) ;
#21335=CARTESIAN_POINT ( 'NONE',  ( 3.595709101656964890, 5.917279480223868404, 7.636340781540109646 ) ) ;
#21336=CARTESIAN_POINT ( 'NONE',  ( 2.526652830164346053, 118.1588881379252456, 0.8392714833404777419 ) ) ;
#21337=DIRECTION ( 'NONE',  ( -0.9998036453533934997, -0.0004114442613340082121, -0.01981164939336589603 ) ) ;
#21339=CARTESIAN_POINT ( 'NONE',  ( 1.058771226886385586, 124.8229041592835387, 0.01153269281271733331 ) ) ;
#21340=CARTESIAN_POINT ( 'NONE',  ( -15.29680631459152806, 120.8527393138689376, 0.2092734171533192633 ) ) ;
#21342=DIRECTION ( 'NONE',  ( -4.017660918040594346E-17, 1.000000000000000000, 2.376309959284834438E-19 ) ) ;
#21345=CARTESIAN_POINT ( 'NONE',  ( -9.538359384048678891, 124.8019839352694476, -0.1905991205270209377 ) ) ;
#21346=CARTESIAN_POINT ( 'NONE',  ( 4.127870218248371970, -15.50624122109489633, 4.747786349039386344 ) ) ;
#21347=CARTESIAN_POINT ( 'NONE',  ( -13.89335097268686070, 122.2371923977168109, 1.173247377384143642 ) ) ;
#21348=AXIS2_PLACEMENT_3D ( 'NONE', #29141, #7009, #3823 ) ;
#21349=CARTESIAN_POINT ( 'NONE',  ( 21.93433297169870144, 150.0588410196355937, -0.9994452811612329901 ) ) ;
#21350=CARTESIAN_POINT ( 'NONE',  ( -3.854280124997887746, 21.23357344512866973, -2.551540157904111261 ) ) ;
#21351=CARTESIAN_POINT ( 'NONE',  ( -15.70536794749891385, 121.0099257824619627, -0.6352152019007782924 ) ) ;
#21353=CARTESIAN_POINT ( 'NONE',  ( -5.563975647486109288, 116.7001730204267460, -0.05417444520887694515 ) ) ;
#21355=CARTESIAN_POINT ( 'NONE',  ( -0.009931517865296061315, 119.6374844068871397, 0.4970137656763587430 ) ) ;
#21357=CARTESIAN_POINT ( 'NONE',  ( 9.796729639280824742, 120.9522862504114897, -1.196371290339073079 ) ) ;
#21358=CARTESIAN_POINT ( 'NONE',  ( -19.95554629013501469, 150.7967616730061593, -2.267143661507363017 ) ) ;
#21360=CARTESIAN_POINT ( 'NONE',  ( 0.01341678693497577735, 156.4123495908283985, -0.6714308817992609146 ) ) ;
#21361=ORIENTED_EDGE ( 'NONE', *, *, #34966, .F. ) ;
#21362=CARTESIAN_POINT ( 'NONE',  ( -4.244755607818407661, 119.7015364213435333, -0.9259100998607278088 ) ) ;
#21363=CARTESIAN_POINT ( 'NONE',  ( 4.529877808639974468, -15.43662617131508163, 0.9000745948097405025 ) ) ;
#21365=CARTESIAN_POINT ( 'NONE',  ( -4.458822442788735074, 118.1301844220468240, -0.7147248541670323529 ) ) ;
#21367=CARTESIAN_POINT ( 'NONE',  ( -4.838325046627658388, 117.5445662390599466, 0.9681270212778525508 ) ) ;
#21368=CARTESIAN_POINT ( 'NONE',  ( 17.88897823598637160, 147.4621342421176848, 2.293131556269223381 ) ) ;
#21371=CARTESIAN_POINT ( 'NONE',  ( -8.418590987418564708, -6.603242653765095227, 0.8142584484527041200 ) ) ;
#21372=CARTESIAN_POINT ( 'NONE',  ( 8.994301780669024637, 123.6974368934138226, 0.4925676131310584571 ) ) ;
#21376=CARTESIAN_POINT ( 'NONE',  ( -1.621065714518569623, 117.9394518546463075, 1.312504281541743367 ) ) ;
#21377=CARTESIAN_POINT ( 'NONE',  ( 1.565376701539133553, 118.7629491485454025, 1.245871636779464886 ) ) ;
#21380=EDGE_CURVE ( 'NONE', #28325, #28199, #12737, .T. ) ;
#21381=CARTESIAN_POINT ( 'NONE',  ( -15.16801640535331153, 156.1230782244120121, -0.1031879763837424829 ) ) ;
#21384=CARTESIAN_POINT ( 'NONE',  ( 6.895111204100116353, 121.6823721895668058, -0.3746929160640417034 ) ) ;
#21385=CARTESIAN_POINT ( 'NONE',  ( -8.614520148391088483, 118.6763556054875863, 0.8198081090888234002 ) ) ;
#21387=CARTESIAN_POINT ( 'NONE',  ( 0.08719654901811217662, 115.7029491485439507, -1.760460446363953047 ) ) ;
#21388=CARTESIAN_POINT ( 'NONE',  ( -8.617107517140190964, 123.3364012560002578, -0.3915851211929421982 ) ) ;
#21389=CARTESIAN_POINT ( 'NONE',  ( 4.239944546232853106, -14.55591092887127758, 4.867068800921800609 ) ) ;
#21390=CARTESIAN_POINT ( 'NONE',  ( -4.918710253155017753, 117.7409041207840090, 0.6764595669667289313 ) ) ;
#21392=CARTESIAN_POINT ( 'NONE',  ( 21.54627550604352493, 132.6250929350426020, 0.6335863061179136668 ) ) ;
#21393=CARTESIAN_POINT ( 'NONE',  ( 2.845126842128428812, 121.0294355418728998, 0.09108657199543482297 ) ) ;
#21394=CARTESIAN_POINT ( 'NONE',  ( -5.036492167631829275, 117.3993844946803478, 0.5480994846027128498 ) ) ;
#21395=CARTESIAN_POINT ( 'NONE',  ( -0.3664848240473963514, 30.73350494673895739, -0.9073219246443798847 ) ) ;
#21396=CARTESIAN_POINT ( 'NONE',  ( -15.65298122355244637, 120.8241032224722176, -0.4173319239378794898 ) ) ;
#21399=ORIENTED_EDGE ( 'NONE', *, *, #15940, .F. ) ;
#21400=CARTESIAN_POINT ( 'NONE',  ( 6.192180060147616238, 119.1566478384643375, 1.251899301844930035 ) ) ;
#21401=CARTESIAN_POINT ( 'NONE',  ( -5.332935397695336199, 105.1224662015457199, -0.1065647409268299373 ) ) ;
#21402=CARTESIAN_POINT ( 'NONE',  ( 21.42793111275534201, 141.8478887571778273, 2.143904907781018387 ) ) ;
#21404=CARTESIAN_POINT ( 'NONE',  ( 4.766456943369734134, 158.1906701298835856, -1.576320697809042715 ) ) ;
#21405=CARTESIAN_POINT ( 'NONE',  ( -0.09930934064637705894, -13.04092083763876175, -4.623607705436294957 ) ) ;
#21406=CARTESIAN_POINT ( 'NONE',  ( -19.72970310060717480, 132.0165317526581816, -1.843001364771305717 ) ) ;
#21407=CARTESIAN_POINT ( 'NONE',  ( 4.907479179103392930, 117.6706796365961054, -0.8186149998474543388 ) ) ;
#21409=CARTESIAN_POINT ( 'NONE',  ( 2.923657115617320112, 107.8178375082508609, 4.476818208047827596 ) ) ;
#21411=ORIENTED_EDGE ( 'NONE', *, *, #33934, .T. ) ;
#21412=CARTESIAN_POINT ( 'NONE',  ( -15.66469409602200891, 147.2250547476223801, -0.08357164438766989667 ) ) ;
#21413=CARTESIAN_POINT ( 'NONE',  ( -14.20181026158660309, 125.7140216354555804, -2.028863013303968899 ) ) ;
#21415=CARTESIAN_POINT ( 'NONE',  ( 3.829091000068871598, -15.41100336169511031, 5.152250049158875633 ) ) ;
#21417=EDGE_CURVE ( 'NONE', #41007, #3899, #35305, .T. ) ;
#21418=CARTESIAN_POINT ( 'NONE',  ( -0.5318626099109079464, 118.1651004811886594, -0.8919322041951796010 ) ) ;
#21420=CARTESIAN_POINT ( 'NONE',  ( 8.179471065859045709, 156.5149677146980309, 2.065073912022258984 ) ) ;
#21421=DIRECTION ( 'NONE',  ( -4.017660918040594346E-17, 1.000000000000000000, 2.376309959284834438E-19 ) ) ;
#21422=CARTESIAN_POINT ( 'NONE',  ( -4.761160981199589415, 118.7629491485453599, -0.9360238318275121427 ) ) ;
#21423=CARTESIAN_POINT ( 'NONE',  ( -2.822804308802561835, 121.9077826007922312, 0.1826741318641921241 ) ) ;
#21424=CARTESIAN_POINT ( 'NONE',  ( 6.742867120194277142, -6.769607736128188336, 5.057590804256700601 ) ) ;
#21425=CARTESIAN_POINT ( 'NONE',  ( 16.29504633872591768, 146.4745453488731357, 1.441742819671184783 ) ) ;
#21426=CARTESIAN_POINT ( 'NONE',  ( -4.787809760100155465, 118.5930653697794384, -0.9398806957526995021 ) ) ;
#21427=CARTESIAN_POINT ( 'NONE',  ( 22.26937170471349603, 150.7043692363948537, -0.4001190995498105640 ) ) ;
#21433=CARTESIAN_POINT ( 'NONE',  ( -4.308292265359691342, 118.2138082877722240, 0.3344837457086672350 ) ) ;
#21434=CARTESIAN_POINT ( 'NONE',  ( -1.794468298957929475, 116.4672891243423578, -0.03585774721038182539 ) ) ;
#21437=CARTESIAN_POINT ( 'NONE',  ( 8.304983337102498808, 120.2147944736314713, -1.116985254693862784 ) ) ;
#21438=DIRECTION ( 'NONE',  ( 5.206863593109713661E-17, -1.000000000000000000, 1.077750396879097183E-30 ) ) ;
#21439=CARTESIAN_POINT ( 'NONE',  ( 4.342787850355605883, 118.1821923640319625, 0.6217834867231702978 ) ) ;
#21440=CARTESIAN_POINT ( 'NONE',  ( -15.99655225346421972, 147.0154580547469152, -1.170958206671063762 ) ) ;
#21442=CARTESIAN_POINT ( 'NONE',  ( 4.713631738767327661, 116.7564862437112794, 0.09418957996065571714 ) ) ;
#21444=CARTESIAN_POINT ( 'NONE',  ( -3.957843245660688680, 22.95775517496322848, 2.395914033147342970 ) ) ;
#21447=EDGE_CURVE ( 'NONE', #3703, #36577, #5117, .T. ) ;
#21448=CARTESIAN_POINT ( 'NONE',  ( 5.078986093043054595, 68.92746620154572668, 0.1014902294541237815 ) ) ;
#21449=CARTESIAN_POINT ( 'NONE',  ( -7.806212186347956106, 122.5473094838618522, 0.09301756479190019522 ) ) ;
#21451=CARTESIAN_POINT ( 'NONE',  ( 21.82912119472381107, 136.8312970274703844, 1.482621438090450328 ) ) ;
#21452=CARTESIAN_POINT ( 'NONE',  ( -2.763989507385018918, 104.6144662015456817, -3.966747042067132245 ) ) ;
#21453=CARTESIAN_POINT ( 'NONE',  ( 2.755344442395651683, -14.11966664619605716, -0.1083093155031689958 ) ) ;
#21454=CARTESIAN_POINT ( 'NONE',  ( 9.525696296010659481, 157.4068808874136209, -1.471446521238429117 ) ) ;
#21455=CARTESIAN_POINT ( 'NONE',  ( -3.942276470047367809, 157.0187206368471209, 1.592783893122187378 ) ) ;
#21456=CARTESIAN_POINT ( 'NONE',  ( -4.488006035213030209, 18.49445617864287073, 1.146732334616328286 ) ) ;
#21457=CARTESIAN_POINT ( 'NONE',  ( -15.72348727998161877, 121.4292885696920621, -0.9291061361373527117 ) ) ;
#21458=CARTESIAN_POINT ( 'NONE',  ( -0.7860673829865619799, 16.32342451650498916, -0.5763570944834206511 ) ) ;
#21459=ORIENTED_EDGE ( 'NONE', *, *, #33247, .F. ) ;
#21462=CARTESIAN_POINT ( 'NONE',  ( -6.226794683659868213, 155.3658059236344684, 0.5518929715360438859 ) ) ;
#21463=CARTESIAN_POINT ( 'NONE',  ( 4.651167782940357931, -13.82644354294225408, 4.017274338905189701 ) ) ;
#21464=CARTESIAN_POINT ( 'NONE',  ( 5.207149668175573787, 156.3268443366877989, -1.412139582428342033 ) ) ;
#21466=CARTESIAN_POINT ( 'NONE',  ( 2.487003399377340163, 115.7030328857400150, 1.696587098641219926 ) ) ;
#21469=CARTESIAN_POINT ( 'NONE',  ( 3.171691571413298050, -13.57474810710837509, 1.775319381694977716 ) ) ;
#21470=CARTESIAN_POINT ( 'NONE',  ( -4.670922868269323125, 117.8935129453105759, -0.9879990057292081795 ) ) ;
#21471=CARTESIAN_POINT ( 'NONE',  ( 5.940729632618738876, 121.5467800236367424, 0.09028238529180381000 ) ) ;
#21473=CARTESIAN_POINT ( 'NONE',  ( 4.596153127770110203, 158.0471523224993859, 1.806220157282541372 ) ) ;
#21476=CARTESIAN_POINT ( 'NONE',  ( 0.03066982525775523508, 157.3074135339440147, -1.534843470138540278 ) ) ;
#21477=CARTESIAN_POINT ( 'NONE',  ( 2.803048170062486300, 116.6385632091030544, -0.1397181956995449670 ) ) ;
#21479=CARTESIAN_POINT ( 'NONE',  ( 1.713575183690340786, -15.32738180877292500, 5.454580614592902776 ) ) ;
#21480=CARTESIAN_POINT ( 'NONE',  ( -6.589702033682734540E-14, 87.97746620154572383, -4.338478393988997516E-18 ) ) ;
#21483=CARTESIAN_POINT ( 'NONE',  ( -4.645946495889221595, 117.9566612795834999, 0.7540674584965481042 ) ) ;
#21485=EDGE_LOOP ( 'NONE', ( #41310, #788, #32521, #1641, #10773, #5660, #28093, #6676, #25193 ) ) ;
#21486=ORIENTED_EDGE ( 'NONE', *, *, #7115, .F. ) ;
#21487=CARTESIAN_POINT ( 'NONE',  ( -0.5121017581959355081, 118.7629491485454025, 1.259106457356409470 ) ) ;
#21489=CARTESIAN_POINT ( 'NONE',  ( -5.628064490234534922, 118.3591030996166751, -1.176039089841854235 ) ) ;
#21490=CARTESIAN_POINT ( 'NONE',  ( -1.876195077988602078, 107.8038693663528278, -4.521701016168464093 ) ) ;
#21491=CARTESIAN_POINT ( 'NONE',  ( 4.781282322697058440, 117.4742075776832309, 1.189488429716421658 ) ) ;
#21493=CARTESIAN_POINT ( 'NONE',  ( -0.7818436192038892285, 120.2878791493615296, 0.5419007644741468122 ) ) ;
#21496=DIRECTION ( 'NONE',  ( -0.9998004120163610509, -4.016384292689131511E-17, -0.01997839162482749689 ) ) ;
#21497=CARTESIAN_POINT ( 'NONE',  ( 2.740927916200229131, -14.67636064986481337, 4.771625012207401539 ) ) ;
#21498=CARTESIAN_POINT ( 'NONE',  ( 6.089625701343383213, 119.5347744825833871, -0.2725575997743531209 ) ) ;
#21499=CARTESIAN_POINT ( 'NONE',  ( 7.784012320790350437, 122.6313477007501689, 0.1555430920740328848 ) ) ;
#21500=CARTESIAN_POINT ( 'NONE',  ( -6.335520854202698615, 28.81365682905730097, 0.1643347731004514700 ) ) ;
#21501=CARTESIAN_POINT ( 'NONE',  ( -0.9196057312421086483, 115.7029491485453718, 1.717296384394745079 ) ) ;
#21502=CARTESIAN_POINT ( 'NONE',  ( 2.229080734463354307, 9.364070591990056869, -4.050418370856919914 ) ) ;
#21503=CARTESIAN_POINT ( 'NONE',  ( 15.60595500976382333, 121.0226940419799462, 0.7351363234501834265 ) ) ;
#21505=CARTESIAN_POINT ( 'NONE',  ( 2.600103240316629538, 104.6144662015457243, -4.075503436606891405 ) ) ;
#21506=CARTESIAN_POINT ( 'NONE',  ( 3.404406166340397277, -15.64019586361782643, 4.053891870528842922 ) ) ;
#21507=CARTESIAN_POINT ( 'NONE',  ( -2.527692779614401086, 158.0185616612000956, 1.624164342510255210 ) ) ;
#21508=CARTESIAN_POINT ( 'NONE',  ( -0.7014129483091587902, 16.11884676413550466, -0.6771123631929140130 ) ) ;
#21509=CARTESIAN_POINT ( 'NONE',  ( -0.9370761106581132482, 23.39645565634240043, 0.2812775048015344614 ) ) ;
#21510=ORIENTED_EDGE ( 'NONE', *, *, #5258, .T. ) ;
#21511=VERTEX_POINT ( 'NONE', #34001 ) ;
#21513=CARTESIAN_POINT ( 'NONE',  ( 1.155499320159395937, 111.9985432423065959, 2.960082065640199822 ) ) ;
#21515=CARTESIAN_POINT ( 'NONE',  ( -4.803469898345708700, 156.0326374431741385, 1.047298710704739344 ) ) ;
#21517=EDGE_CURVE ( 'NONE', #12283, #11359, #13550, .T. ) ;
#21518=CARTESIAN_POINT ( 'NONE',  ( 3.214659515886821861, -12.19625089790456229, 0.4983212145216010525 ) ) ;
#21519=CARTESIAN_POINT ( 'NONE',  ( 17.58824906652080600, 148.8653046532945723, -1.619734885946522596 ) ) ;
#21520=CARTESIAN_POINT ( 'NONE',  ( -3.174067013697543072, 118.4902560533893592, -0.8904294910640481175 ) ) ;
#21523=CARTESIAN_POINT ( 'NONE',  ( 4.074910602682932925, 118.2429491485453354, -0.1454311599470142491 ) ) ;
#21524=CARTESIAN_POINT ( 'NONE',  ( 9.391698128491960063, 124.2036136473707018, -0.1363215471561607384 ) ) ;
#21526=ORIENTED_EDGE ( 'NONE', *, *, #14406, .F. ) ;
#21527=CARTESIAN_POINT ( 'NONE',  ( 2.768784035434307178, -15.00486597294339930, 4.394545281259884639 ) ) ;
#21528=CARTESIAN_POINT ( 'NONE',  ( -6.578476689077728991E-14, 85.18346620154574111, -5.002419396613184919E-18 ) ) ;
#21530=CARTESIAN_POINT ( 'NONE',  ( 3.857898856315107761, -6.768822978661375167, 2.551181839177400601 ) ) ;
#21531=CARTESIAN_POINT ( 'NONE',  ( 5.849275934571454449, 120.8872308857076519, 0.8185814695607154245 ) ) ;
#21532=CARTESIAN_POINT ( 'NONE',  ( -2.900060555911446070, 29.50094634256690540, 2.476086984555808002 ) ) ;
#21533=CARTESIAN_POINT ( 'NONE',  ( -5.086085965935806641, 114.3657942991566472, 1.756424186875608751 ) ) ;
#21534=VECTOR ( 'NONE', #2395, 1000.000000000000000 ) ;
#21536=CARTESIAN_POINT ( 'NONE',  ( -2.406711483539481389, 4.503775517365914638, 3.979180414515509412 ) ) ;
#21537=CARTESIAN_POINT ( 'NONE',  ( 0.6438746309740379647, 120.9974662015465867, 0.01286614746332127857 ) ) ;
#21538=CARTESIAN_POINT ( 'NONE',  ( 0.6424836204703546771, -8.070646579680392563, 8.395564330620057802 ) ) ;
#21540=CARTESIAN_POINT ( 'NONE',  ( -8.754227852576507374, 117.8550674546482071, -0.6168156700147224836 ) ) ;
#21541=CIRCLE ( 'NONE', #30410, 5.080000000000006288 ) ;
#21542=CARTESIAN_POINT ( 'NONE',  ( -0.1664298668079876309, 110.3683645023726427, -3.586750284817682211 ) ) ;
#21544=CARTESIAN_POINT ( 'NONE',  ( 4.537321141924904211, 26.63107350737006840, 0.8823464973398146283 ) ) ;
#21545=CARTESIAN_POINT ( 'NONE',  ( 0.6963533560661814281, 117.3993842961302363, 1.488888644047975607 ) ) ;
#21546=CARTESIAN_POINT ( 'NONE',  ( -6.538176131568015962E-14, 82.13546620154573930, -1.207165459078370276E-19 ) ) ;
#21548=CARTESIAN_POINT ( 'NONE',  ( 0.3790891741044132290, 120.5507043431651510, -0.5490176968301535565 ) ) ;
#21549=CARTESIAN_POINT ( 'NONE',  ( -21.14621813959900010, 132.3956117394162106, 0.2431941713936564553 ) ) ;
#21551=ORIENTED_EDGE ( 'NONE', *, *, #15701, .F. ) ;
#21555=CARTESIAN_POINT ( 'NONE',  ( -5.945776936743828678, 121.5465042053001667, -0.1188107733588233128 ) ) ;
#21556=CARTESIAN_POINT ( 'NONE',  ( 4.355571528211143573, -15.30747929803376373, 4.711715777764150737 ) ) ;
#21557=CARTESIAN_POINT ( 'NONE',  ( -15.93384955644688183, 125.3951846505478329, 1.286024093939968305 ) ) ;
#21558=CARTESIAN_POINT ( 'NONE',  ( 22.39452804842985500, 149.5981344557702641, -0.8550856607202135251 ) ) ;
#21559=CARTESIAN_POINT ( 'NONE',  ( -4.631227783250409402, 22.10816835407601744, -0.05711764529929251599 ) ) ;
#21560=CARTESIAN_POINT ( 'NONE',  ( -4.777924661806649986, 116.8922783744782379, -0.3800144224740276133 ) ) ;
#21562=EDGE_LOOP ( 'NONE', ( #29488, #33708, #39054, #14328 ) ) ;
#21563=CARTESIAN_POINT ( 'NONE',  ( 8.795381777531829925, 117.6899729038807720, 0.2515276502602432074 ) ) ;
#21565=CARTESIAN_POINT ( 'NONE',  ( -5.108784305046479624, 120.0747842884402132, 0.7604166522187121302 ) ) ;
#21567=CARTESIAN_POINT ( 'NONE',  ( 16.46135582144558285, 131.4813445454897192, -1.641276044305394866 ) ) ;
#21568=CARTESIAN_POINT ( 'NONE',  ( -4.008523173341965951, 118.0179939250997023, -0.8984863180294770935 ) ) ;
#21570=STYLED_ITEM ( 'NONE', ( #16656 ), #22381 ) ;
#21572=CARTESIAN_POINT ( 'NONE',  ( 8.258026456251805314, 154.6505398758502849, -0.7900859392159012007 ) ) ;
#21574=CARTESIAN_POINT ( 'NONE',  ( -10.13131171838204203, 122.2967958330617648, -1.512676856611740561 ) ) ;
#21575=CARTESIAN_POINT ( 'NONE',  ( 3.762885361805711870, -15.68952731832974656, 3.843115198823321865 ) ) ;
#21576=CARTESIAN_POINT ( 'NONE',  ( -4.112774970794720986, 118.2429491485453070, -0.3453283136715148416 ) ) ;
#21579=CARTESIAN_POINT ( 'NONE',  ( 17.92322948971676766, 147.1528319293316542, 2.295422193410857847 ) ) ;
#21581=CARTESIAN_POINT ( 'NONE',  ( -2.033853377119958061, -8.777475726645231902, -8.175041553700232555 ) ) ;
#21582=CARTESIAN_POINT ( 'NONE',  ( 0.6270554149910597674, 120.8998192842950488, 0.1385313962210439065 ) ) ;
#21586=CARTESIAN_POINT ( 'NONE',  ( 0.1066493941974573784, 105.7853621660184444, -5.332931186019219005 ) ) ;
#21587=CARTESIAN_POINT ( 'NONE',  ( -7.839438867670176059, 122.3085338874637671, -0.7152514657530811837 ) ) ;
#21588=( GEOMETRIC_REPRESENTATION_CONTEXT ( 3 ) GLOBAL_UNCERTAINTY_ASSIGNED_CONTEXT ( ( #23544 ) ) GLOBAL_UNIT_ASSIGNED_CONTEXT ( ( #41838, #3065, #35427 ) ) REPRESENTATION_CONTEXT ( 'NONE', 'WORKASPACE' ) );
#21591=CARTESIAN_POINT ( 'NONE',  ( -1.417759636995488570, 159.6040221172770259, 0.05833233067434092506 ) ) ;
#21594=CARTESIAN_POINT ( 'NONE',  ( 7.864380575010578411, 122.2948005240338603, -0.4127209565927187351 ) ) ;
#21596=CARTESIAN_POINT ( 'NONE',  ( -7.886551735270039387, 122.1946728851204398, 0.4945421293698979981 ) ) ;
#21598=CARTESIAN_POINT ( 'NONE',  ( 4.375075790391449004, 118.7629491485369613, -0.8820669128659245350 ) ) ;
#21599=CARTESIAN_POINT ( 'NONE',  ( -8.927705404389175925, 123.7033391712731145, -0.4040904458349091621 ) ) ;
#21600=CARTESIAN_POINT ( 'NONE',  ( 5.886196856236641572, -12.36517754215322995, 0.8550893866892870232 ) ) ;
#21601=CARTESIAN_POINT ( 'NONE',  ( -21.83857928711807261, 148.7205309135917730, 1.274413580488712450 ) ) ;
#21603=CARTESIAN_POINT ( 'NONE',  ( 22.82515744214346753, 150.4067493646842593, 0.6093393687072348186 ) ) ;
#21604=CARTESIAN_POINT ( 'NONE',  ( 5.317159844422477910, 121.3518965702581340, 0.1425998613045213748 ) ) ;
#21606=CARTESIAN_POINT ( 'NONE',  ( 0.8793282038724897776, 27.06027571872007442, 0.4248793764785103177 ) ) ;
#21607=CARTESIAN_POINT ( 'NONE',  ( -22.98214253804999530, 150.1595482613961110, -0.5361612621683793378 ) ) ;
#21611=ORIENTED_EDGE ( 'NONE', *, *, #35816, .F. ) ;
#21612=CARTESIAN_POINT ( 'NONE',  ( 3.990160187250827217, 118.2607540442166680, 0.9787250380842466013 ) ) ;
#21613=CARTESIAN_POINT ( 'NONE',  ( -6.513165593194060347E-14, 68.92746620154572668, -8.865348866426607246E-18 ) ) ;
#21614=CARTESIAN_POINT ( 'NONE',  ( 6.827620370265914396, 118.1252062928739832, 1.028125137227138275 ) ) ;
#21615=CARTESIAN_POINT ( 'NONE',  ( 16.30903692877109279, 153.4734386769207504, -1.632589361097313230 ) ) ;
#21616=CARTESIAN_POINT ( 'NONE',  ( -6.181412921142831252, 19.34218365691531361, 5.729511908899769246 ) ) ;
#21617=CARTESIAN_POINT ( 'NONE',  ( -17.71751426720061318, 153.9999837190418930, -1.728000864493653754 ) ) ;
#21618=CARTESIAN_POINT ( 'NONE',  ( 4.737242769783595264, 117.7521409222561601, -0.9001186629912181214 ) ) ;
#21619=ADVANCED_FACE ( 'NONE', ( #20980, #17578 ), #36989, .F. ) ;
#21620=CARTESIAN_POINT ( 'NONE',  ( 6.094139411021942898, 119.5248422734510427, 0.5163842741021833493 ) ) ;
#21622=CARTESIAN_POINT ( 'NONE',  ( -9.234582554329520576, 124.2544328994657405, -0.09881537413615858190 ) ) ;
#21623=CARTESIAN_POINT ( 'NONE',  ( -11.65353862096132609, 154.7938929448963279, -2.201148936174281534 ) ) ;
#21624=CARTESIAN_POINT ( 'NONE',  ( 5.208953926857062378, -15.24612122244077561, 3.266433406317167165 ) ) ;
#21628=EDGE_CURVE ( 'NONE', #31017, #39680, #24383, .T. ) ;
#21630=CARTESIAN_POINT ( 'NONE',  ( 18.70459055478403343, 148.4604323410545987, 2.472120825861215732 ) ) ;
#21632=CARTESIAN_POINT ( 'NONE',  ( -4.812426554072069429, 118.7629491485389650, -0.6571134116375234591 ) ) ;
#21633=CARTESIAN_POINT ( 'NONE',  ( -0.2204105866772946287, 106.6745790697264056, 5.009819746185714351 ) ) ;
#21634=CARTESIAN_POINT ( 'NONE',  ( 7.953355231451894269, -5.272462086923463076, -2.798479926915725891 ) ) ;
#21635=CARTESIAN_POINT ( 'NONE',  ( 9.704918697729759458, 124.0009531390599591, 0.8840593909831664376 ) ) ;
#21636=CARTESIAN_POINT ( 'NONE',  ( -5.239701418611189432, 115.6909491485453003, -1.023982712389454930 ) ) ;
#21637=CARTESIAN_POINT ( 'NONE',  ( 8.157450159232084275, 117.7673425867732249, -0.3794901880580578424 ) ) ;
#21642=CARTESIAN_POINT ( 'NONE',  ( -4.499111063581361591, 31.49064988344817806, -0.6933409209711203225 ) ) ;
#21645=CARTESIAN_POINT ( 'NONE',  ( -4.280837819800595412, 118.2124897020258771, 0.3640674451363055120 ) ) ;
#21646=CARTESIAN_POINT ( 'NONE',  ( -9.822473411059320370, 117.9943479623217399, -0.1962763949404990327 ) ) ;
#21649=CARTESIAN_POINT ( 'NONE',  ( -8.223115700291321772, 120.3649693293168639, -1.438891654778712281 ) ) ;
#21650=CARTESIAN_POINT ( 'NONE',  ( 5.329288917532060132, 116.0444662015457453, 0.2890495193807575691 ) ) ;
#21651=CARTESIAN_POINT ( 'NONE',  ( 0.004916276843087831992, 120.6356583033945782, -0.2460305967400713556 ) ) ;
#21652=CARTESIAN_POINT ( 'NONE',  ( 4.973935731622961320, 117.4065895991867734, -0.8875407820844548601 ) ) ;
#21653=CARTESIAN_POINT ( 'NONE',  ( 0.02808993187329204833, 117.9496053154548321, -1.405735122999207887 ) ) ;
#21656=CARTESIAN_POINT ( 'NONE',  ( -2.614655561276646889, 23.60746518810343986, 3.812863311767609620 ) ) ;
#21661=CARTESIAN_POINT ( 'NONE',  ( -7.793391099074982620, 122.5980884063560836, -0.02750199203433729284 ) ) ;
#21663=CARTESIAN_POINT ( 'NONE',  ( -0.9239673467531356321, 25.61616486456964736, -4.531977062890359065 ) ) ;
#21664=CARTESIAN_POINT ( 'NONE',  ( 0.9938236163260620870, 116.9791385580615781, 0.3849800449318574458 ) ) ;
#21665=CARTESIAN_POINT ( 'NONE',  ( -3.891925687308367632, 104.6144662015454401, -2.872084872932638699 ) ) ;
#21666=CARTESIAN_POINT ( 'NONE',  ( 2.908198840139253338, -13.99431844974620454, 0.6722015529863232253 ) ) ;
#21667=CARTESIAN_POINT ( 'NONE',  ( 14.09802512849270073, 121.9525460547650226, -1.083329899170117461 ) ) ;
#21668=CARTESIAN_POINT ( 'NONE',  ( -5.624295920984248909, 156.7050554705274408, 1.628980406729419350 ) ) ;
#21670=CARTESIAN_POINT ( 'NONE',  ( 4.353980591602404360, 23.44215234368072487, -1.583070106892425111 ) ) ;
#21671=CARTESIAN_POINT ( 'NONE',  ( -13.19686234056499430, 119.7880570645780978, -0.9111371353940662665 ) ) ;
#21672=CARTESIAN_POINT ( 'NONE',  ( 0.5639076275445228381, 13.94848098472073161, -0.7944722417661187475 ) ) ;
#21675=CARTESIAN_POINT ( 'NONE',  ( -15.59522120955195845, 147.8873989650969918, 0.4103944809294446383 ) ) ;
#21676=CARTESIAN_POINT ( 'NONE',  ( 3.183750377336629356, -15.03749083096926675, 5.611903928707999256 ) ) ;
#21677=CARTESIAN_POINT ( 'NONE',  ( 10.11798836042633454, 123.5826510519420509, -0.8100524519737970497 ) ) ;
#21678=ORIENTED_EDGE ( 'NONE', *, *, #8732, .T. ) ;
#21679=CARTESIAN_POINT ( 'NONE',  ( 0.5848834147048422860, 115.7029859896981634, 1.760412536671860817 ) ) ;
#21680=CARTESIAN_POINT ( 'NONE',  ( -4.851553261282356644, 117.6732321342373524, -1.041740536389639482 ) ) ;
#21681=CARTESIAN_POINT ( 'NONE',  ( 2.829134042005047256, 121.0305217392013759, 0.03030232591675486795 ) ) ;
#21683=CARTESIAN_POINT ( 'NONE',  ( 9.988019213705062072, 120.6268241347409855, 1.591717657363032723 ) ) ;
#21685=CARTESIAN_POINT ( 'NONE',  ( -6.583861033951825950E-14, 91.02546620154572565, 1.480257718193877056E-29 ) ) ;
#21686=CARTESIAN_POINT ( 'NONE',  ( 0.03153870137009017610, 158.4432089348667319, -1.578325583784927932 ) ) ;
#21688=CARTESIAN_POINT ( 'NONE',  ( 22.95349865178509674, 150.1476136049543868, 0.1290964995630298762 ) ) ;
#21691=CARTESIAN_POINT ( 'NONE',  ( 2.073162808081137509, -15.12483991451984977, 5.841363716764139902 ) ) ;
#21692=FACE_OUTER_BOUND ( 'NONE', #16710, .T. ) ;
#21693=DIRECTION ( 'NONE',  ( 4.017660918040594346E-17, -1.000000000000000000, -2.376309959284834438E-19 ) ) ;
#21694=CARTESIAN_POINT ( 'NONE',  ( -4.783754133273223630, 117.8482099188709071, 0.7929052515055885486 ) ) ;
#21697=DIRECTION ( 'NONE',  ( -4.017660918040594346E-17, 1.000000000000000000, 2.376309959284832031E-19 ) ) ;
#21699=CARTESIAN_POINT ( 'NONE',  ( -5.828253901312384855, 118.9244088370469257, -1.251152115012297728 ) ) ;
#21700=CARTESIAN_POINT ( 'NONE',  ( -6.983605877934339290, 124.9344662015457175, -0.1395490654994193946 ) ) ;
#21701=CARTESIAN_POINT ( 'NONE',  ( 4.857949651814833736, 117.7455164169167290, 0.9241763922800549924 ) ) ;
#21703=CARTESIAN_POINT ( 'NONE',  ( -0.08519874065577472122, 108.5751225745497948, 4.263693374914214296 ) ) ;
#21704=CARTESIAN_POINT ( 'NONE',  ( 0.6989348986720191892, -4.029744825116962303, 4.573446973323917142 ) ) ;
#21705=ADVANCED_FACE ( 'NONE', ( #12249 ), #39172, .T. ) ;
#21706=CARTESIAN_POINT ( 'NONE',  ( 4.958342374402591624, 117.4102150217221237, -0.9055978162701078249 ) ) ;
#21708=CARTESIAN_POINT ( 'NONE',  ( 3.494528270914563528, -13.06595970051097133, 2.012497701936279082 ) ) ;
#21709=CARTESIAN_POINT ( 'NONE',  ( 7.426015305410854417, 123.6670498955208473, 0.1137005639190687006 ) ) ;
#21710=CARTESIAN_POINT ( 'NONE',  ( -1.409834354326183314, 119.9358631726476574, -0.5453972335014173334 ) ) ;
#21711=CARTESIAN_POINT ( 'NONE',  ( -6.065589077789664607, 121.4348142148880214, -0.1208730379670850952 ) ) ;
#21712=CARTESIAN_POINT ( 'NONE',  ( -5.871471797037544071, 31.01275966357848901, 2.875548327037550589 ) ) ;
#21713=CARTESIAN_POINT ( 'NONE',  ( -0.6339378988202717391, 115.7029520820172905, 1.736981566562831425 ) ) ;
#21714=CARTESIAN_POINT ( 'NONE',  ( 4.076717266748975277, 8.489475128091552136, -2.202413229635628689 ) ) ;
#21715=CARTESIAN_POINT ( 'NONE',  ( 18.42221188220377215, 125.1790410860780298, 0.8413473246917885229 ) ) ;
#21717=CARTESIAN_POINT ( 'NONE',  ( 4.563830193338946017, 104.6144662015380931, -2.766517067423098553 ) ) ;
#21718=CARTESIAN_POINT ( 'NONE',  ( 4.512298201359578265, -15.31825885905126228, -0.4677400858729020006 ) ) ;
#21719=CARTESIAN_POINT ( 'NONE',  ( -2.466025220844247468, 157.8629595415303584, 1.630325060746250720 ) ) ;
#21720=CARTESIAN_POINT ( 'NONE',  ( 0.7508863055360318617, -11.68651920905074348, 0.6198408032357946018 ) ) ;
#21721=CARTESIAN_POINT ( 'NONE',  ( -0.6963090749671848600, 14.53960050853193842, 0.6834203841726373962 ) ) ;
#21723=AXIS2_PLACEMENT_3D ( 'NONE', #6114, #19077, #32082 ) ;
#21725=DIRECTION ( 'NONE',  ( -4.017660918040594346E-17, 1.000000000000000000, 2.376309959284834438E-19 ) ) ;
#21726=CARTESIAN_POINT ( 'NONE',  ( 2.208446607403821371, 108.4767889311100362, 4.246804138318780453 ) ) ;
#21728=CARTESIAN_POINT ( 'NONE',  ( -16.31827467517383923, 146.7930872653447523, 0.7884962901916311440 ) ) ;
#21729=DIRECTION ( 'NONE',  ( 0.9998004120163609398, 0.000000000000000000, 0.01997839162482749689 ) ) ;
#21731=CARTESIAN_POINT ( 'NONE',  ( 2.390819523577490280, -14.89105559343156848, 5.112470274569719919 ) ) ;
#21732=CARTESIAN_POINT ( 'NONE',  ( 12.98417868877897163, 125.9520529675768898, -1.303718779035868192 ) ) ;
#21733=CARTESIAN_POINT ( 'NONE',  ( -7.694773992301706222, 119.4405053107883958, -1.366649582720010025 ) ) ;
#21735=CARTESIAN_POINT ( 'NONE',  ( -15.78437780952707215, 146.2378312303354448, -0.3154094333657934679 ) ) ;
#21736=CARTESIAN_POINT ( 'NONE',  ( -6.536164027931061327, 29.86201144190116707, 0.1241447379370549109 ) ) ;
#21737=CARTESIAN_POINT ( 'NONE',  ( 5.244198393876475350, 121.2166884500396833, -0.1799464770355447274 ) ) ;
#21739=CARTESIAN_POINT ( 'NONE',  ( 2.350639260211558668, -15.10312717587823705, 4.966175652281853203 ) ) ;
#21740=DIRECTION ( 'NONE',  ( -0.9998004120163608288, 0.000000000000000000, -0.01997839162482749342 ) ) ;
#21741=CARTESIAN_POINT ( 'NONE',  ( 4.855108373332432947, 117.7629957853780667, 0.8790759234368952235 ) ) ;
#21743=CARTESIAN_POINT ( 'NONE',  ( -0.6580430243309095539, -8.493043821084315326, 4.585212396833119541 ) ) ;
#21744=CARTESIAN_POINT ( 'NONE',  ( 6.788801044988693967, 155.5980657034081105, 1.487835262196284036 ) ) ;
#21746=CARTESIAN_POINT ( 'NONE',  ( -0.3628555246835991066, 105.8844662015457629, 5.327769491516690437 ) ) ;
#21747=CARTESIAN_POINT ( 'NONE',  ( -4.187759052228169132, -5.978784877027076838, 2.003160513425938483 ) ) ;
#21748=CARTESIAN_POINT ( 'NONE',  ( -7.220045317357707698E-14, 120.9974662015457341, -1.901466176754077691E-16 ) ) ;
#21749=CARTESIAN_POINT ( 'NONE',  ( 6.390864997528122871, 2.724353428444007630, 5.482255947279437436 ) ) ;
#21751=CARTESIAN_POINT ( 'NONE',  ( -5.498207759818521723, 117.0463165232320364, -0.7052634562340454050 ) ) ;
#21752=CARTESIAN_POINT ( 'NONE',  ( -0.3633380039126155592, 121.5961256765096152, -0.3912981906941392363 ) ) ;
#21754=CARTESIAN_POINT ( 'NONE',  ( -6.158966240078259879, 30.49883854570459718, 2.286114001711006871 ) ) ;
#21755=CARTESIAN_POINT ( 'NONE',  ( 1.580769961479467911, 28.79261460129497863, -4.363931058323818668 ) ) ;
#21760=CARTESIAN_POINT ( 'NONE',  ( 0.3809694336148531368, 120.1716774721349168, -0.6201936767135831641 ) ) ;
#21761=CARTESIAN_POINT ( 'NONE',  ( -13.37627446016234600, 119.7032035076741465, 0.2201875619950501017 ) ) ;
#21764=ORIENTED_EDGE ( 'NONE', *, *, #4010, .F. ) ;
#21766=CARTESIAN_POINT ( 'NONE',  ( -15.72520672816718523, 146.8976288387275133, -0.2472165429730639463 ) ) ;
#21767=CARTESIAN_POINT ( 'NONE',  ( 6.028374245061780989, -14.54558069259788411, 1.726931113533916040 ) ) ;
#21768=CARTESIAN_POINT ( 'NONE',  ( -14.64490033095734134, 154.5799843816573684, 1.633817034445554039 ) ) ;
#21770=CARTESIAN_POINT ( 'NONE',  ( 17.54374246740519538, 153.9260871938423065, -1.166327135487699618 ) ) ;
#21771=CARTESIAN_POINT ( 'NONE',  ( -4.012847786888796620, 11.73797844546971270, -2.294585225469591983 ) ) ;
#21772=CARTESIAN_POINT ( 'NONE',  ( -8.183336086940967036, 117.5993832199734328, -0.5018928202873275124 ) ) ;
#21775=CARTESIAN_POINT ( 'NONE',  ( -5.563655970165373610, 116.7104814527052667, 0.001055824976130279166 ) ) ;
#21776=CARTESIAN_POINT ( 'NONE',  ( -6.550797450135577910E-14, 84.67546620154573134, 2.164564701558966795E-29 ) ) ;
#21777=CARTESIAN_POINT ( 'NONE',  ( -9.926448497735856691, 122.5082557396031291, 1.019319756893169338 ) ) ;
#21779=CARTESIAN_POINT ( 'NONE',  ( 2.404146712672410757, 157.7073581658784178, -1.626633079703769136 ) ) ;
#21781=CARTESIAN_POINT ( 'NONE',  ( -19.67869083727186919, 136.1149058410947532, -2.266608711299009649 ) ) ;
#21783=CARTESIAN_POINT ( 'NONE',  ( 8.389933090069224164, 122.6561726160659731, -0.4454891811124966350 ) ) ;
#21785=CARTESIAN_POINT ( 'NONE',  ( -1.354060893033618429, 119.5584937100158243, -0.6194060083641331760 ) ) ;
#21786=CARTESIAN_POINT ( 'NONE',  ( 4.220783105811589664, -15.35787857112312693, 0.3368293509108917783 ) ) ;
#21787=CARTESIAN_POINT ( 'NONE',  ( -4.144796762172593851, 118.2390927319115832, -0.4001549744010635123 ) ) ;
#21788=CIRCLE ( 'NONE', #23844, 5.080000000000006288 ) ;
#21790=CARTESIAN_POINT ( 'NONE',  ( -4.932064943850939187, 117.4109299206517818, 0.9378731322835484052 ) ) ;
#21791=CARTESIAN_POINT ( 'NONE',  ( 11.09706570755277788, 123.3376105302527037, 1.576947150105312501 ) ) ;
#21794=AXIS2_PLACEMENT_3D ( 'NONE', #30852, #14652, #27656 ) ;
#21795=CARTESIAN_POINT ( 'NONE',  ( -8.432237393326710517, 2.893158626077577900, 0.2611430682616783239 ) ) ;
#21796=CARTESIAN_POINT ( 'NONE',  ( -0.004910621514806326471, 156.3161161488371533, 0.2457475809811482670 ) ) ;
#21797=CARTESIAN_POINT ( 'NONE',  ( 2.722315517715700572, 118.0959538166519849, -0.8461704532092527709 ) ) ;
#21798=DIRECTION ( 'NONE',  ( -0.9998004120163609398, 0.000000000000000000, -0.01997839162482749689 ) ) ;
#21800=CARTESIAN_POINT ( 'NONE',  ( -0.2177282545546737058, 118.1588900835526914, 0.9015745107222330468 ) ) ;
#21803=CARTESIAN_POINT ( 'NONE',  ( -7.784012322544769269, 122.6313477034873074, -0.1555430911242075831 ) ) ;
#21806=CARTESIAN_POINT ( 'NONE',  ( -22.98049992366342309, 150.1579452496398801, -0.3057203305217676137 ) ) ;
#21807=B_SPLINE_CURVE_WITH_KNOTS ( 'NONE', 3,
 ( #27380, #10979, #7801, #29743, #33161, #8002 ),
 .UNSPECIFIED., .F., .F.,
 ( 4, 2, 4 ),
 ( 0.01688307072824751093, 0.01716653801739397023, 0.01745000530654042953 ),
 .UNSPECIFIED. ) ;
#21808=ORIENTED_EDGE ( 'NONE', *, *, #36085, .T. ) ;
#21810=CARTESIAN_POINT ( 'NONE',  ( 6.041926471666161369, 121.4447802455698877, 0.08406784148116053235 ) ) ;
#21811=CARTESIAN_POINT ( 'NONE',  ( -7.920006352636957736, 122.0419191725281678, 0.5993308652498723355 ) ) ;
#21813=CARTESIAN_POINT ( 'NONE',  ( 0.8976087670000849617, 115.7028554113044123, -1.718884712376715251 ) ) ;
#21814=CARTESIAN_POINT ( 'NONE',  ( -7.577119205441469774, 122.4179301937671767, -0.2905534069474315917 ) ) ;
#21815=CARTESIAN_POINT ( 'NONE',  ( 2.821817058828279823, -15.16010343277639194, 5.768636546787819341 ) ) ;
#21816=CARTESIAN_POINT ( 'NONE',  ( -13.46300103848319196, 120.9245410081625209, 0.9131080906212013515 ) ) ;
#21818=CARTESIAN_POINT ( 'NONE',  ( 15.78464309758866690, 121.0087326939336378, 0.5477818752361017784 ) ) ;
#21819=CARTESIAN_POINT ( 'NONE',  ( 9.098285506954120194, 153.9557200233357435, 0.2398147890565895668 ) ) ;
#21821=CARTESIAN_POINT ( 'NONE',  ( 0.9647673288271847447, 27.50405299253531410, 0.1566625405351598777 ) ) ;
#21822=CARTESIAN_POINT ( 'NONE',  ( -1.417643301182503368, 159.6052071245950970, -0.07209812905978379982 ) ) ;
#21823=CARTESIAN_POINT ( 'NONE',  ( -3.682264917456324227, 88.99346620154574339, -0.07358041635423923088 ) ) ;
#21824=EDGE_LOOP ( 'NONE', ( #13420, #24654, #42111, #41499 ) ) ;
#21825=CARTESIAN_POINT ( 'NONE',  ( 4.084276569795989964, 118.3417739162233744, 0.9965765103875263708 ) ) ;
#21826=CARTESIAN_POINT ( 'NONE',  ( 4.135298993362768627, -14.76517611359900961, -2.065434832541708676 ) ) ;
#21827=CARTESIAN_POINT ( 'NONE',  ( 21.74240605069414300, 146.0876064316611860, 2.155783927327832306 ) ) ;
#21828=CARTESIAN_POINT ( 'NONE',  ( 15.41274837478107784, 125.4902479783272184, -1.384083614372567661 ) ) ;
#21829=CARTESIAN_POINT ( 'NONE',  ( -8.411989387141455055, 18.26859176889432490, 0.3690887223902433734 ) ) ;
#21830=CARTESIAN_POINT ( 'NONE',  ( -19.75679031132836272, 152.3633698111425758, -1.804147069793666347 ) ) ;
#21831=CARTESIAN_POINT ( 'NONE',  ( 4.843357629187326374, 117.6435499053430931, -0.9176853102465485357 ) ) ;
#21833=CARTESIAN_POINT ( 'NONE',  ( 4.730021378956775102, 112.7831754354443348, 2.563638443952895862 ) ) ;
#21834=CARTESIAN_POINT ( 'NONE',  ( -1.606403942294512222, 120.9755568995931156, 0.03214495494220275668 ) ) ;
#21835=CARTESIAN_POINT ( 'NONE',  ( -4.182621382392013309, 157.4559852174668322, -1.843664507743932202 ) ) ;
#21836=CARTESIAN_POINT ( 'NONE',  ( 4.016706779461339138, -15.37834506377831723, 5.009826762111060816 ) ) ;
#21837=AXIS2_PLACEMENT_3D ( 'NONE', #25531, #38532, #19750 ) ;
#21839=CARTESIAN_POINT ( 'NONE',  ( -3.159512914937968819, 117.3993812128981347, -1.388958443500331263 ) ) ;
#21841=CARTESIAN_POINT ( 'NONE',  ( 18.41737859239631803, 149.0103496150362901, 2.461622840412570845 ) ) ;
#21845=CARTESIAN_POINT ( 'NONE',  ( -0.5468943487521297220, 107.2171362991012842, 4.774625097732313250 ) ) ;
#21846=CARTESIAN_POINT ( 'NONE',  ( 1.420544585151703343, -13.23898594424576203, -8.332176651214544094 ) ) ;
#21847=CARTESIAN_POINT ( 'NONE',  ( -0.004916276843216625669, 120.6356583033945782, 0.2460305967400715221 ) ) ;
#21849=CARTESIAN_POINT ( 'NONE',  ( 15.64055365641533690, 121.4606353739761744, -0.3859511643760804023 ) ) ;
#21851=AXIS2_PLACEMENT_3D ( 'NONE', #13863, #40497, #26858 ) ;
#21853=DIRECTION ( 'NONE',  ( -5.206863593109713661E-17, 1.000000000000000000, -1.077750396879097183E-30 ) ) ;
#21854=AXIS2_PLACEMENT_3D ( 'NONE', #31461, #15265, #11441 ) ;
#21855=EDGE_CURVE ( 'NONE', #10591, #34625, #40715, .T. ) ;
#21858=CARTESIAN_POINT ( 'NONE',  ( 2.063686733023939901, -15.30319371230426917, 5.972472134935500776 ) ) ;
#21859=CARTESIAN_POINT ( 'NONE',  ( -4.123368102914265698, 118.2429491485453354, 0.1806032781032593237 ) ) ;
#21860=CARTESIAN_POINT ( 'NONE',  ( 5.232282628590676943, 115.9099169135977689, -1.117942969498063155 ) ) ;
#21861=ORIENTED_EDGE ( 'NONE', *, *, #10863, .T. ) ;
#21863=CARTESIAN_POINT ( 'NONE',  ( -8.148487026236251651, 120.7334362890933477, -1.392358570714556487 ) ) ;
#21864=DIRECTION ( 'NONE',  ( 4.017660918040594346E-17, -1.000000000000000000, -2.376309959284834438E-19 ) ) ;
#21865=CARTESIAN_POINT ( 'NONE',  ( -8.043896744444055003, 154.6119571123129788, -0.8805139685443125197 ) ) ;
#21867=CARTESIAN_POINT ( 'NONE',  ( 0.01782678998956764571, 118.1651004037419881, -0.8921253700480482607 ) ) ;
#21869=CARTESIAN_POINT ( 'NONE',  ( 4.419457123578296454, 17.78516144714274105, -1.360477052881604143 ) ) ;
#21874=CARTESIAN_POINT ( 'NONE',  ( 6.073146511589309071, 121.4483376143599287, 0.1695659588288715436 ) ) ;
#21876=CARTESIAN_POINT ( 'NONE',  ( 22.50793294095875652, 142.2972183020237367, 1.640122747091714128 ) ) ;
#21878=CARTESIAN_POINT ( 'NONE',  ( 2.460727335429193197, -15.06314154744310585, 4.845259171755021299 ) ) ;
#21879=CARTESIAN_POINT ( 'NONE',  ( 6.834340443517000985, 118.4250403807481575, -0.8562881416378697041 ) ) ;
#21880=CARTESIAN_POINT ( 'NONE',  ( -11.06957317628273785, 122.5598569164413334, 1.209814958810230934 ) ) ;
#21881=CARTESIAN_POINT ( 'NONE',  ( -4.282102574861781363, 27.11529131024228434, -1.748715980913516876 ) ) ;
#21882=CARTESIAN_POINT ( 'NONE',  ( -0.3355986945388581555, 116.9201722098172382, -0.3169108175686566886 ) ) ;
#21883=CARTESIAN_POINT ( 'NONE',  ( -0.2078495401522961472, -3.970246887572310257, -0.9510052327550873041 ) ) ;
#21884=ORIENTED_EDGE ( 'NONE', *, *, #19063, .T. ) ;
#21886=CARTESIAN_POINT ( 'NONE',  ( -13.37097581265842905, 134.1388935151753401, 0.4393653360420519682 ) ) ;
#21887=CARTESIAN_POINT ( 'NONE',  ( 4.916912942907655903, -13.49232782388964935, 3.465564004687308408 ) ) ;
#21888=CARTESIAN_POINT ( 'NONE',  ( 2.625396581831431320, 120.2926465633240127, -0.4415429531236469418 ) ) ;
#21889=EDGE_LOOP ( 'NONE', ( #13776, #9518, #30950, #28918 ) ) ;
#21890=CARTESIAN_POINT ( 'NONE',  ( 1.253061391183938555, 115.7029074980223271, 1.740285132395945178 ) ) ;
#21891=CIRCLE ( 'NONE', #3569, 5.588000000000006295 ) ;
#21893=CARTESIAN_POINT ( 'NONE',  ( -4.876515041417334828, 117.7132576400690027, -0.9240722683427993189 ) ) ;
#21895=CARTESIAN_POINT ( 'NONE',  ( 15.77133435453283461, 146.5691041611200660, 0.3151487940933137555 ) ) ;
#21896=VERTEX_POINT ( 'NONE', #41870 ) ;
#21897=CARTESIAN_POINT ( 'NONE',  ( 19.60096582671575405, 145.2539617268756729, 2.527680105953240552 ) ) ;
#21898=DIRECTION ( 'NONE',  ( -5.206863593109713661E-17, 1.000000000000000000, -1.077750396879097183E-30 ) ) ;
#21900=CARTESIAN_POINT ( 'NONE',  ( 4.996532045110951614, 117.4672001989742398, -0.7808144642989416351 ) ) ;
#21902=CARTESIAN_POINT ( 'NONE',  ( 17.03046551078681148, 122.6950552906510694, 0.003367075177501197957 ) ) ;
#21903=CARTESIAN_POINT ( 'NONE',  ( -6.008977632366433015E-14, 69.43546620154573645, 9.241195598681324794E-17 ) ) ;
#21906=CARTESIAN_POINT ( 'NONE',  ( 1.774262667879180411, -15.10206561957146221, 5.641947496857006250 ) ) ;
#21910=CARTESIAN_POINT ( 'NONE',  ( -4.749506590746891632, 117.9455148129567164, 0.6338826763805054387 ) ) ;
#21911=ORIENTED_EDGE ( 'NONE', *, *, #19130, .F. ) ;
#21913=LINE ( 'NONE', #21077, #22699 ) ;
#21914=CARTESIAN_POINT ( 'NONE',  ( 5.671516376864802034, 118.3593096970241305, -0.9503249289038079306 ) ) ;
#21915=CARTESIAN_POINT ( 'NONE',  ( -3.549733929830021673, 110.1236525333376619, -3.577684766704721575 ) ) ;
#21916=CARTESIAN_POINT ( 'NONE',  ( 4.859873572602068315, 117.5461019621290575, 1.119800123233829270 ) ) ;
#21917=CARTESIAN_POINT ( 'NONE',  ( 2.568134854143032442, -15.02010252187911554, 4.714990346623905815 ) ) ;
#21918=CARTESIAN_POINT ( 'NONE',  ( -0.4232488410869896800, 124.9344662015457317, -0.008457519121176893320 ) ) ;
#21923=CARTESIAN_POINT ( 'NONE',  ( 4.093446853122521212, 111.5999093057820772, -2.867423493935855827 ) ) ;
#21924=CARTESIAN_POINT ( 'NONE',  ( -17.41367791652951880, 147.5992144370567871, -2.159268082968857971 ) ) ;
#21926=CARTESIAN_POINT ( 'NONE',  ( 7.002510704594238966, 121.9568449727899520, 0.1399268299516837899 ) ) ;
#21929=CARTESIAN_POINT ( 'NONE',  ( 4.513502956352341222, 8.064680226961385756, -0.9949261897555528034 ) ) ;
#21930=CARTESIAN_POINT ( 'NONE',  ( 22.38168272118564062, 137.0915487549672491, 1.023064006592828479 ) ) ;
#21932=CARTESIAN_POINT ( 'NONE',  ( 1.938810462764684051, 105.1240917556268641, -4.970498420434350528 ) ) ;
#21933=CARTESIAN_POINT ( 'NONE',  ( 3.857521300888583582, -15.67877420849868386, 3.673684628067402702 ) ) ;
#21934=CARTESIAN_POINT ( 'NONE',  ( -6.702632528927957800, 119.6463993818898359, 1.017002412926887533 ) ) ;
#21935=CARTESIAN_POINT ( 'NONE',  ( -0.1630216852218501489, 24.74361041950371032, -0.9604350664704873752 ) ) ;
#21936=CARTESIAN_POINT ( 'NONE',  ( -0.4248780512631177841, 5.470267980206036107, 0.8793239699972363876 ) ) ;
#21939=ORIENTED_EDGE ( 'NONE', *, *, #17360, .T. ) ;
#21941=CARTESIAN_POINT ( 'NONE',  ( 0.09082259786502508425, 105.9597790263619146, 5.306270932934927131 ) ) ;
#21942=CARTESIAN_POINT ( 'NONE',  ( -8.467456592458740161, 122.5794309061019618, 0.5337204191277992171 ) ) ;
#21944=CARTESIAN_POINT ( 'NONE',  ( 3.884801864383396808, -13.20605796264157128, 2.953397552313849150 ) ) ;
#21945=CARTESIAN_POINT ( 'NONE',  ( 7.383627470571713758, 120.8389031223305352, -0.9130476668403028073 ) ) ;
#21946=CARTESIAN_POINT ( 'NONE',  ( -19.91185195753441661, 145.3736917597469471, -2.515063280254572042 ) ) ;
#21948=CARTESIAN_POINT ( 'NONE',  ( 8.557792064668554133, 118.7566837416166692, 1.194711599118532863 ) ) ;
#21949=CARTESIAN_POINT ( 'NONE',  ( -0.8575334777045592327, 37.18052207920313634, 1.701599969488736930 ) ) ;
#21951=CARTESIAN_POINT ( 'NONE',  ( 4.305249565653697985, 155.8363458669846864, -0.2390946120805818864 ) ) ;
#21953=CARTESIAN_POINT ( 'NONE',  ( -0.4669360306570718988, 105.9268256211375103, -5.319786075441130357 ) ) ;
#21954=CARTESIAN_POINT ( 'NONE',  ( -6.501940248589056060E-14, 66.13346620154574396, -9.529289869050788486E-18 ) ) ;
#21955=ADVANCED_FACE ( 'NONE', ( #15640 ), #33958, .F. ) ;
#21958=ADVANCED_FACE ( 'NONE', ( #27912 ), #25897, .T. ) ;
#21959=CARTESIAN_POINT ( 'NONE',  ( 7.984751813625430295, 22.47881364768745271, 2.830840501157275924 ) ) ;
#21960=CARTESIAN_POINT ( 'NONE',  ( 16.88761465400175155, 147.3835828867039766, 1.922606999130501482 ) ) ;
#21961=DIRECTION ( 'NONE',  ( -0.9998004120163609398, 0.000000000000000000, -0.01997839162482749689 ) ) ;
#21962=CARTESIAN_POINT ( 'NONE',  ( 4.725057015249740644, 116.7592613395855352, 0.05262260997884649766 ) ) ;
#21963=CARTESIAN_POINT ( 'NONE',  ( -6.300894124712325350, 120.0808430858776887, 0.2013153013476513264 ) ) ;
#21966=CARTESIAN_POINT ( 'NONE',  ( 15.26262975078991779, 148.0175730704188481, 0.3049836654608578113 ) ) ;
#21968=CARTESIAN_POINT ( 'NONE',  ( 5.527521262545286085, 2.498091250051501344, 6.371381250375013572 ) ) ;
#21969=CARTESIAN_POINT ( 'NONE',  ( 2.167983032549695821, 116.6620882976681628, -0.3727921820594300439 ) ) ;
#21970=CARTESIAN_POINT ( 'NONE',  ( 0.05238710762246717723, 113.0327356262574341, -2.621665085262795181 ) ) ;
#21972=CARTESIAN_POINT ( 'NONE',  ( -7.401523468229766145, -5.981721843848114339, 4.095665678060115944 ) ) ;
#21973=CARTESIAN_POINT ( 'NONE',  ( -0.02812206864257424735, 117.9394488565463064, 1.407343427015907311 ) ) ;
#21976=CARTESIAN_POINT ( 'NONE',  ( 0.6988325576870501044, 114.3327162918516962, -2.155465965906839809 ) ) ;
#21977=CARTESIAN_POINT ( 'NONE',  ( -5.638719538426442135, 159.1014311945586712, 0.3820744581509935567 ) ) ;
#21982=CARTESIAN_POINT ( 'NONE',  ( -11.79229084918624082, 130.2874513316071443, -0.1788083452990229527 ) ) ;
#21983=CARTESIAN_POINT ( 'NONE',  ( 2.291706021380962355, -15.53059561260056221, 5.887745402940570472 ) ) ;
#21984=CARTESIAN_POINT ( 'NONE',  ( -16.30903692877122424, 153.4734386769207504, 1.632589361097313230 ) ) ;
#21985=CARTESIAN_POINT ( 'NONE',  ( 3.058359628041792622, 159.2229145144301867, -0.9584471420995392954 ) ) ;
#21986=CARTESIAN_POINT ( 'NONE',  ( 3.121479725567877228, 16.06095178295013071, 3.416230322513892137 ) ) ;
#21987=CARTESIAN_POINT ( 'NONE',  ( 0.004910662370358964517, 159.5928157220454295, -0.2457496255665020946 ) ) ;
#21990=EDGE_CURVE ( 'NONE', #39565, #35799, #18314, .T. ) ;
#21991=VERTEX_POINT ( 'NONE', #6190 ) ;
#21992=CARTESIAN_POINT ( 'NONE',  ( 0.3920235582991468126, 123.4679809879532542, 0.1617017839830492132 ) ) ;
#21993=CARTESIAN_POINT ( 'NONE',  ( -6.486711254249450261E-14, 72.48346620154573827, 1.207165459670006807E-19 ) ) ;
#21994=CARTESIAN_POINT ( 'NONE',  ( -11.97328186178021170, 153.4554508723442439, 1.471200310048991655 ) ) ;
#21996=CARTESIAN_POINT ( 'NONE',  ( 19.00246547725214086, 147.5601278813269914, -1.724645192979526342 ) ) ;
#21997=CARTESIAN_POINT ( 'NONE',  ( -21.11954758237303764, 149.1058327099893290, -2.305704729659639796 ) ) ;
#22000=CARTESIAN_POINT ( 'NONE',  ( 8.995803412248823960, 123.1852847016406685, -0.4677080646552714271 ) ) ;
#22001=ORIENTED_EDGE ( 'NONE', *, *, #21004, .F. ) ;
#22002=CARTESIAN_POINT ( 'NONE',  ( -3.791208754741646647, 156.9018388488748883, -1.699278904607348872 ) ) ;
#22003=CARTESIAN_POINT ( 'NONE',  ( 3.668568818830479028, -15.43917834477946727, 2.972162690469843049 ) ) ;
#22004=CARTESIAN_POINT ( 'NONE',  ( -4.151500737348964520, 118.2394118959124114, -0.3932187221707064695 ) ) ;
#22007=CARTESIAN_POINT ( 'NONE',  ( -4.786196459852546603, 117.6677270402089022, 0.9346353507170748198 ) ) ;
#22008=CARTESIAN_POINT ( 'NONE',  ( 17.39571694528370216, 144.3974720067888313, 2.245075470287479558 ) ) ;
#22009=CARTESIAN_POINT ( 'NONE',  ( 3.009276887026298031, 39.20946620154573026, -1.210121013456480599 ) ) ;
#22010=CIRCLE ( 'NONE', #280, 0.5080000000000002292 ) ;
#22011=CARTESIAN_POINT ( 'NONE',  ( 7.936949992814905208, -1.433721018288910853, -2.821688713676304250 ) ) ;
#22012=CARTESIAN_POINT ( 'NONE',  ( 1.583718294068441557, 120.9073379818811134, 0.1636693232558003586 ) ) ;
#22019=CARTESIAN_POINT ( 'NONE',  ( -7.954217475012978156, 121.7102781429355076, -1.090678254656372692 ) ) ;
#22023=CARTESIAN_POINT ( 'NONE',  ( -9.797860116730056745, 118.0024801742749929, -0.05693907317356646652 ) ) ;
#22026=CARTESIAN_POINT ( 'NONE',  ( 5.965796276062810044, 121.4109386283128771, -0.03877683265643106642 ) ) ;
#22027=CARTESIAN_POINT ( 'NONE',  ( -7.788361016000392212, 122.6175610729407452, -0.07939682847776179109 ) ) ;
#22029=CARTESIAN_POINT ( 'NONE',  ( 1.218872564666173997, 115.7029483217724390, -1.696103018937654028 ) ) ;
#22030=CARTESIAN_POINT ( 'NONE',  ( -9.288927291931168284, 124.2653519604415067, -0.3477528771403739505 ) ) ;
#22032=CARTESIAN_POINT ( 'NONE',  ( 5.673176617818914913, -13.06232935199844114, 2.160669506476638357 ) ) ;
#22033=CARTESIAN_POINT ( 'NONE',  ( -1.132512924677574029, 117.7697124030934077, 0.5521475598058978029 ) ) ;
#22035=CARTESIAN_POINT ( 'NONE',  ( 23.30750959433825287, 148.8446908248229477, 0.7975424382754977559 ) ) ;
#22036=CARTESIAN_POINT ( 'NONE',  ( 15.37822400800898137, 147.8362807140078417, 0.4405641715785962309 ) ) ;
#22038=CARTESIAN_POINT ( 'NONE',  ( -0.7839530942921373313, 14.33508526448824760, 0.5845576647881698396 ) ) ;
#22039=CARTESIAN_POINT ( 'NONE',  ( -0.2950350728690642188, 116.4333835968663919, -0.04389667002116224431 ) ) ;
#22040=DIRECTION ( 'NONE',  ( 5.206863593109713661E-17, -1.000000000000000000, 1.077750396879097183E-30 ) ) ;
#22042=ORIENTED_EDGE ( 'NONE', *, *, #25382, .T. ) ;
#22043=CARTESIAN_POINT ( 'NONE',  ( 2.276210869248295854, 116.3688137149352571, 0.2778600029539394223 ) ) ;
#22044=CARTESIAN_POINT ( 'NONE',  ( 3.793251108634954516, -14.54000584982637001, -2.652246991476435056 ) ) ;
#22045=CARTESIAN_POINT ( 'NONE',  ( 2.096789228655988158, 117.6567184779878232, 0.6641637518095837578 ) ) ;
#22046=CARTESIAN_POINT ( 'NONE',  ( 6.741493414765732162, 119.3011930948910759, -1.016225879973854607 ) ) ;
#22048=CARTESIAN_POINT ( 'NONE',  ( -0.4402761300873825334, 6.286315195291644287, -8.460265346311377499 ) ) ;
#22049=CARTESIAN_POINT ( 'NONE',  ( -1.049200951577276664, 117.3444111807523882, -0.5008604537731422557 ) ) ;
#22050=CARTESIAN_POINT ( 'NONE',  ( 4.719955967559978482, 117.8401570591244507, -0.8449457312083641369 ) ) ;
#22051=CARTESIAN_POINT ( 'NONE',  ( 5.245364206137161922, 116.4655405006298849, 1.092799426751067005 ) ) ;
#22052=CARTESIAN_POINT ( 'NONE',  ( -11.84655969407690534, 151.9972573545839225, -0.1156591128142183539 ) ) ;
#22053=CARTESIAN_POINT ( 'NONE',  ( -18.91595150393233027, 147.0452383304005082, -2.485053599041413985 ) ) ;
#22055=CARTESIAN_POINT ( 'NONE',  ( 5.769960013412655186, -14.74427453315851899, 2.495425615322755419 ) ) ;
#22057=CARTESIAN_POINT ( 'NONE',  ( 5.239248437989107110, 115.6909491485453145, 1.024417804751308836 ) ) ;
#22061=CARTESIAN_POINT ( 'NONE',  ( 18.91595150393219882, 147.0452383304005082, 2.485053599041414429 ) ) ;
#22063=FACE_OUTER_BOUND ( 'NONE', #31600, .T. ) ;
#22064=CARTESIAN_POINT ( 'NONE',  ( -0.1065646865916160119, 105.8844662015457061, 5.332932678536314697 ) ) ;
#22065=CARTESIAN_POINT ( 'NONE',  ( -8.418873817481639321, -10.66996252118913091, -0.4581590610697409693 ) ) ;
#22066=CARTESIAN_POINT ( 'NONE',  ( 0.6009856513685500889, 120.6441756478195089, 0.2688776736664574285 ) ) ;
#22067=CARTESIAN_POINT ( 'NONE',  ( 22.18008199020988158, 150.6715983490228723, -0.5179974990882317831 ) ) ;
#22070=CARTESIAN_POINT ( 'NONE',  ( -8.795391115079340238, 117.6899447938497048, -0.2513484674950453024 ) ) ;
#22072=CARTESIAN_POINT ( 'NONE',  ( -16.31694223957266843, 121.4173703750124531, -0.3260513381110075604 ) ) ;
#22074=CARTESIAN_POINT ( 'NONE',  ( -4.450428981627350566, 119.5746151482181148, -0.9239258634587167451 ) ) ;
#22075=CARTESIAN_POINT ( 'NONE',  ( -5.332935397695335311, 104.6144662015457385, -0.1065647409268299373 ) ) ;
#22076=CARTESIAN_POINT ( 'NONE',  ( -0.6714861817528541277, 156.3445873232922736, -0.4416347707370365527 ) ) ;
#22078=CARTESIAN_POINT ( 'NONE',  ( 21.90516586211584737, 151.4314113202728436, 0.4630247046772880681 ) ) ;
#22080=CARTESIAN_POINT ( 'NONE',  ( 2.229080734463354307, 9.364070591990056869, -4.050418370856919914 ) ) ;
#22081=CARTESIAN_POINT ( 'NONE',  ( -5.314278422745059238, 105.1224610256965235, 0.4583187270701644667 ) ) ;
#22085=CARTESIAN_POINT ( 'NONE',  ( -6.993440844384329225, 121.9489362634231924, -0.08176518772864471707 ) ) ;
#22087=CARTESIAN_POINT ( 'NONE',  ( 16.15135472115366611, 155.1612327564137388, 1.525667687477715306 ) ) ;
#22088=CARTESIAN_POINT ( 'NONE',  ( -4.760791928307794407, 104.6144662015457385, -0.8517687557738815585 ) ) ;
#22089=CARTESIAN_POINT ( 'NONE',  ( 4.703170801235237342, 114.7515816609199533, 1.852262375087519120 ) ) ;
#22090=CARTESIAN_POINT ( 'NONE',  ( 15.16136233027289393, 154.7927800759015042, -1.480671785937533347 ) ) ;
#22091=CARTESIAN_POINT ( 'NONE',  ( -10.44084688387123627, 122.0805278159965610, 1.176281030686837425 ) ) ;
#22092=CARTESIAN_POINT ( 'NONE',  ( 3.308978306493741250, 24.09187545982852541, -3.235542752117448018 ) ) ;
#22093=CARTESIAN_POINT ( 'NONE',  ( -15.50015290592197381, 121.4967652112180048, -1.085784428920436362 ) ) ;
#22096=CARTESIAN_POINT ( 'NONE',  ( -15.99817776903328692, 146.0164801329953548, 0.4101439804456899485 ) ) ;
#22097=CARTESIAN_POINT ( 'NONE',  ( 4.834931622272050866, -13.60668467239417545, 3.655623996717635382 ) ) ;
#22098=CARTESIAN_POINT ( 'NONE',  ( 17.03734119261599744, 146.7604995623492243, -1.248076303867124093 ) ) ;
#22099=CARTESIAN_POINT ( 'NONE',  ( -4.845000436079312855, 117.7309513030204613, -0.9913659128643448337 ) ) ;
#22100=CARTESIAN_POINT ( 'NONE',  ( 10.18105065676961729, 125.9743313966586129, 0.2034416216762105212 ) ) ;
#22101=MECHANICAL_DESIGN_GEOMETRIC_PRESENTATION_REPRESENTATION('',(#41885),#31649);
#22103=CARTESIAN_POINT ( 'NONE',  ( 18.46656456646925548, 135.7714211226372640, 2.417028963773544259 ) ) ;
#22104=CARTESIAN_POINT ( 'NONE',  ( 14.67500508080551924, 148.8517222229471315, 0.2932415260855780748 ) ) ;
#22106=CARTESIAN_POINT ( 'NONE',  ( 4.921840205057578466, 117.4109437077822946, -0.9481957113721782848 ) ) ;
#22107=CARTESIAN_POINT ( 'NONE',  ( 15.11282490002045087, 156.1437908837410191, -0.09152821140687288082 ) ) ;
#22111=CARTESIAN_POINT ( 'NONE',  ( 1.762577841197611406, -15.17375865732635631, 5.852863657745463577 ) ) ;
#22114=CARTESIAN_POINT ( 'NONE',  ( -4.580516980462806309, 118.0858134742356782, 0.5548273466755001548 ) ) ;
#22115=B_SPLINE_SURFACE_WITH_KNOTS ( 'NONE', 3, 3, ( 
 ( #37090, #10247, #30473, #1317, #39658, #30263, #7280, #20036, #13660, #1104, #14071, #27075 ),
 ( #1941, #40910, #24919, #11501, #34316, #8531, #37492, #5556, #8316, #21491, #12140, #34106 ),
 ( #40504, #14900, #21081, #27697, #24702, #28111, #21916, #14692, #25132, #31519, #34726, #4933 ),
 ( #27903, #18513, #2363, #15322, #17891, #5145, #11715, #30894, #38135, #18099, #34523, #5349 ),
 ( #40705, #37916, #1528, #11299, #37708, #11927, #37288, #8949, #24283, #18303, #8107, #1734 ),
 ( #15108, #24487, #21287, #8740, #4727, #17679, #31305, #30680, #14484, #27497, #2149, #31102 ),
 ( #41121, #21701, #28329, #41337, #26173, #28745, #22121, #2577, #15538, #32361, #3401, #39178 ),
 ( #12968, #31734, #25961, #15949, #22540, #19355, #9570, #18938, #35567, #35150, #32568, #28946 ),
 ( #38551, #9985, #5975, #3189, #2, #2987, #19149, #16151, #38968, #9778, #41963, #32154 ),
 ( #41548, #6181, #41758, #6385, #16369, #35352, #22745, #18724, #25343, #35776, #12559, #31946 ),
 ( #29155, #12762, #19559, #25751, #6591, #29374, #9364, #38346, #213, #28540, #34946, #13188 ),
 ( #5770, #12355, #2784, #9164, #15740, #38759, #25548, #22327, #846, #4257, #40248, #33008 ),
 ( #7234, #17424, #39394, #20609, #428, #6801, #26602, #35986, #32790, #16800, #33429, #22958 ),
 ( #13819, #23383, #20400, #17220, #39825, #1269, #13611, #3836, #23167, #36201, #26817, #29802 ),
 ( #30216, #23811, #36416, #7022, #10619, #27027, #642, #19990, #39608, #3620, #20194, #1056 ),
 ( #30422, #33219, #4047, #10412, #23601, #16585, #17007, #29594, #36622, #33640, #14226, #30007 ),
 ( #19770, #7442, #14020, #7652, #40035, #27233, #10830, #36833, #4467, #13399, #26387, #10196 ),
 ( #4674, #21034, #24231, #1687, #18249, #28060, #24438, #41071, #7859, #40655, #34266, #37659 ),
 ( #33846, #40861, #27441, #14432, #20820, #11448, #31255, #11880, #2096, #8483, #21439, #37241 ),
 ( #8059, #15061, #1476, #17840, #5094, #40456, #18047, #27642, #37441, #24649, #34056, #30839 ),
 ( #4886, #34468, #14641, #31048, #24869, #11246, #5301, #17632, #8265, #21236, #1887, #14849 ),
 ( #11041, #27854, #11663, #24025, #37041, #30632, #4608, #26538, #32941, #10556, #19924, #16729 ),
 ( #17362, #24162, #14360, #39970, #7372, #4405, #1199, #23741, #27373, #39761, #29940, #7170 ),
 ( #26955, #13755, #3982, #30349, #7794, #20331, #20128, #10760, #10969, #26751, #33154, #779 ) ),
 .UNSPECIFIED., .F., .F., .F.,
 ( 4, 2, 2, 2, 2, 2, 2, 2, 2, 2, 2, 4 ),
 ( 4, 2, 1, 2, 1, 2, 4 ),
 ( 0.000000000000000000, 0.1320084156805522713, 0.1980126235208284069, 0.2640168313611045425, 0.3918685259135502030, 0.4557943731897730055, 0.5197202204659958635, 0.5807706587133798504, 0.6418210969607638372, 0.7639219734555318109, 0.8819609867277659054, 1.000000000000000000 ),
 ( 0.000000000000000000, 0.1250000000000000000, 0.2500000000000000000, 0.5000000000000000000, 0.7500000000000000000, 0.8750000000000000000, 1.000000000000000000 ),
 .UNSPECIFIED. ) ;
#22117=ORIENTED_EDGE ( 'NONE', *, *, #29282, .T. ) ;
#22118=CARTESIAN_POINT ( 'NONE',  ( -2.791966037470495987, 115.6909491485424581, -1.685616604675346908 ) ) ;
#22119=CARTESIAN_POINT ( 'NONE',  ( 8.388245728505863141, 119.8075375339928854, -1.104450739913065638 ) ) ;
#22120=CARTESIAN_POINT ( 'NONE',  ( -7.618479139564732883, 124.9344662015457317, -0.1522353441811853947 ) ) ;
#22121=CARTESIAN_POINT ( 'NONE',  ( 4.783303902122270301, 117.7666275948723893, 1.035273760934583898 ) ) ;
#22122=CARTESIAN_POINT ( 'NONE',  ( -0.1698098321967818070, 106.7790779034713324, 4.970076682467829521 ) ) ;
#22123=CARTESIAN_POINT ( 'NONE',  ( 4.560362914109654220, -11.68884639558073069, 0.6953251057713033534 ) ) ;
#22126=CARTESIAN_POINT ( 'NONE',  ( 5.582679110870555128, 119.7830797108918688, -0.2735363082852447780 ) ) ;
#22127=CARTESIAN_POINT ( 'NONE',  ( -10.85577430263316145, 123.7747955097422476, -1.451053175688577168 ) ) ;
#22128=CARTESIAN_POINT ( 'NONE',  ( 0.7910183541139823582, 37.90597915310805632, -1.254447098105976321 ) ) ;
#22129=CARTESIAN_POINT ( 'NONE',  ( -6.158966240078259879, 30.49883854570459718, 2.286114001711006871 ) ) ;
#22131=CARTESIAN_POINT ( 'NONE',  ( 3.121479725567877228, 16.06095178295013071, 3.416230322513892137 ) ) ;
#22132=CARTESIAN_POINT ( 'NONE',  ( 18.29650779608093458, 125.1624627582897915, 0.9465853942869046911 ) ) ;
#22134=CARTESIAN_POINT ( 'NONE',  ( 1.603816410906297341, 104.6144662015457811, -4.552900351846083105 ) ) ;
#22135=CARTESIAN_POINT ( 'NONE',  ( 3.614876661864775187, -15.45153451277975165, 3.150551394879585132 ) ) ;
#22136=CARTESIAN_POINT ( 'NONE',  ( -17.50667431346024117, 135.4862447717955547, 1.719380121689204399 ) ) ;
#22137=CARTESIAN_POINT ( 'NONE',  ( -0.4694259674403166716, 18.92165170904731397, 0.8533247626313392731 ) ) ;
#22138=CARTESIAN_POINT ( 'NONE',  ( -0.1494942157332288524, 1.595350521021342782, -0.9636992805340545143 ) ) ;
#22140=ORIENTED_EDGE ( 'NONE', *, *, #32940, .T. ) ;
#22142=CARTESIAN_POINT ( 'NONE',  ( 3.137457178757887988, 117.8122656274855871, 0.9631651297103498433 ) ) ;
#22143=CARTESIAN_POINT ( 'NONE',  ( -15.86865214134244795, 143.7482200480382346, 0.8098737496861397878 ) ) ;
#22144=CARTESIAN_POINT ( 'NONE',  ( -11.03183784343237583, 128.0124916018596650, -0.2204423744267034746 ) ) ;
#22145=CARTESIAN_POINT ( 'NONE',  ( 1.990724735134854262, -15.09768785095407040, 5.370787383207776600 ) ) ;
#22146=CARTESIAN_POINT ( 'NONE',  ( 10.63443090528964241, 122.8495954190337898, -1.101905667251144250 ) ) ;
#22147=CARTESIAN_POINT ( 'NONE',  ( -15.45413117217014332, 153.1703808545849483, -2.356132421238607222 ) ) ;
#22149=EDGE_CURVE ( 'NONE', #27091, #9260, #29164, .T. ) ;
#22150=CARTESIAN_POINT ( 'NONE',  ( 8.762167414255284115, 117.8147271796869973, 0.5760304689628181762 ) ) ;
#22151=CARTESIAN_POINT ( 'NONE',  ( -0.3512404605478313679, 38.00633005727588198, 1.239100654724479167 ) ) ;
#22152=CARTESIAN_POINT ( 'NONE',  ( 15.85578974452665335, 145.9541952667573810, -0.1379097727432555265 ) ) ;
#22154=CARTESIAN_POINT ( 'NONE',  ( -2.546031358067248451, 107.1167599116761124, -4.680030732370826563 ) ) ;
#22160=CARTESIAN_POINT ( 'NONE',  ( -8.001679540263406665, 18.69059125004590172, 2.668541714186715819 ) ) ;
#22161=CARTESIAN_POINT ( 'NONE',  ( 12.60153737394475648, 128.4643691153342218, 1.495224527512394985 ) ) ;
#22163=CARTESIAN_POINT ( 'NONE',  ( 0.0007535234281856949918, 116.4338605912342786, -0.03770939363766601798 ) ) ;
#22164=CARTESIAN_POINT ( 'NONE',  ( -6.897523911742089453, 121.8252198949890186, 0.01845719934638757193 ) ) ;
#22167=CARTESIAN_POINT ( 'NONE',  ( 13.57054970571769914, 121.9345505566020194, 1.704910367088877221 ) ) ;
#22168=EDGE_CURVE ( 'NONE', #40141, #38260, #6158, .T. ) ;
#22169=CARTESIAN_POINT ( 'NONE',  ( 7.658903097349539557, 3.149683656735901671, 3.518291596705641400 ) ) ;
#22170=CARTESIAN_POINT ( 'NONE',  ( 2.173545817240357003, 116.6950714377704372, -0.3876481791814581634 ) ) ;
#22171=CARTESIAN_POINT ( 'NONE',  ( -0.3562073053189366845, 119.8383472832136931, -0.7014361403029916175 ) ) ;
#22174=CARTESIAN_POINT ( 'NONE',  ( 8.369638709285570854, -11.69152869469262157, 0.7709884470677680346 ) ) ;
#22175=CARTESIAN_POINT ( 'NONE',  ( 2.723865133717724873, 118.1588879269519197, 0.8291662895598204130 ) ) ;
#22177=CARTESIAN_POINT ( 'NONE',  ( 3.187143392547471255, -14.52651900126690876, 3.212499789951002604 ) ) ;
#22179=CARTESIAN_POINT ( 'NONE',  ( 1.058122102717250934, 124.9344662015457459, 0.02114379780294225672 ) ) ;
#22180=CARTESIAN_POINT ( 'NONE',  ( -23.00823290520148845, 149.2143936249396461, 0.3942700086401352277 ) ) ;
#22186=CARTESIAN_POINT ( 'NONE',  ( 3.601051898931722395, -15.74651769575186044, 4.782909482641136911 ) ) ;
#22187=CARTESIAN_POINT ( 'NONE',  ( -9.025716902756052207, 119.5326672034033777, 1.052790416315139144 ) ) ;
#22188=CARTESIAN_POINT ( 'NONE',  ( 21.68724320794224525, 149.9601031839316079, -1.147785971009648076 ) ) ;
#22189=CARTESIAN_POINT ( 'NONE',  ( -4.478778176974228309, 3.316883148187759645, 1.141857468124592101 ) ) ;
#22195=CARTESIAN_POINT ( 'NONE',  ( -0.01386859376762973779, 119.8383472832138779, 0.6940411431075129700 ) ) ;
#22197=CARTESIAN_POINT ( 'NONE',  ( -5.207149668175701684, 156.3268443366877989, 1.412139582428342255 ) ) ;
#22199=CARTESIAN_POINT ( 'NONE',  ( 5.055620027408425088, 119.3892302351119810, -0.8859254200104712540 ) ) ;
#22200=CARTESIAN_POINT ( 'NONE',  ( -21.01875934457266837, 148.7375953542188256, -2.355668865594946926 ) ) ;
#22202=CARTESIAN_POINT ( 'NONE',  ( 16.18586682243763875, 146.0959698922748942, -0.6488728679227168117 ) ) ;
#22204=CARTESIAN_POINT ( 'NONE',  ( -7.368974454111360650, 120.7277362223577768, -1.240556355415273648 ) ) ;
#22205=CARTESIAN_POINT ( 'NONE',  ( 2.947576629936649706, -15.31278845794613375, 4.223034005107467515 ) ) ;
#22206=CARTESIAN_POINT ( 'NONE',  ( -4.237174196529505110, 118.2251025442845673, -0.4770184348334939872 ) ) ;
#22209=CARTESIAN_POINT ( 'NONE',  ( -4.907998571170089086, 117.7148545784633882, 0.7335003228574443757 ) ) ;
#22210=CARTESIAN_POINT ( 'NONE',  ( 9.109784082438006081, 121.7740273863187923, 1.385347505406782309 ) ) ;
#22213=CARTESIAN_POINT ( 'NONE',  ( -4.050807963365556930, 30.95410787014092335, -2.229501126309402448 ) ) ;
#22214=CARTESIAN_POINT ( 'NONE',  ( 5.276193270648691147, 121.3253820001177417, 0.2225082926070589828 ) ) ;
#22216=TOROIDAL_SURFACE ( 'NONE', #34509, 5.080000000000005400, 0.5080000000000000071 ) ;
#22219=EDGE_CURVE ( 'NONE', #25673, #1100, #1436, .T. ) ;
#22220=CARTESIAN_POINT ( 'NONE',  ( -0.2349146782472707473, 117.9394520961335360, 1.402130674019514966 ) ) ;
#22226=CARTESIAN_POINT ( 'NONE',  ( -9.784355093145462590, 118.0142902678875885, 0.004515160920743777929 ) ) ;
#22229=CARTESIAN_POINT ( 'NONE',  ( -6.925176729217432658, 121.9065058997480122, -0.3750947163342890356 ) ) ;
#22231=CARTESIAN_POINT ( 'NONE',  ( 4.901772867295396630, 117.4071509163661204, -0.9681717027652592122 ) ) ;
#22232=VERTEX_POINT ( 'NONE', #8274 ) ;
#22233=CARTESIAN_POINT ( 'NONE',  ( 2.051901541566586218, 115.7029480913673751, -1.635851152962789934 ) ) ;
#22234=CARTESIAN_POINT ( 'NONE',  ( -12.91493749300788885, 133.8340822528099636, -0.3749514369420003934 ) ) ;
#22235=CARTESIAN_POINT ( 'NONE',  ( 2.103176148521523459, -15.33886314497087611, 5.964097425510020756 ) ) ;
#22236=CARTESIAN_POINT ( 'NONE',  ( -19.06828360855658744, 152.1029585079319020, 1.398049597035978087 ) ) ;
#22238=CARTESIAN_POINT ( 'NONE',  ( 20.65160272637281480, 152.5811724025633112, 0.7328296130731980496 ) ) ;
#22241=CARTESIAN_POINT ( 'NONE',  ( 7.992875830012473592, 122.8474187487093872, 0.2833331899898612893 ) ) ;
#22243=CARTESIAN_POINT ( 'NONE',  ( -0.9731698936423014423, 13.46246454747003618, 0.06867709314994872860 ) ) ;
#22244=CARTESIAN_POINT ( 'NONE',  ( 0.001319893060087149817, 116.4580521601689185, -0.06605284600166357045 ) ) ;
#22245=CARTESIAN_POINT ( 'NONE',  ( -5.586884702347497900, 123.6644662015457214, -0.1116392523995361624 ) ) ;
#22247=ORIENTED_EDGE ( 'NONE', *, *, #11287, .F. ) ;
#22248=CARTESIAN_POINT ( 'NONE',  ( -2.788466383568154239, 117.1109391571273619, 0.5482988353915653201 ) ) ;
#22251=CARTESIAN_POINT ( 'NONE',  ( 21.43631064271305320, 148.9071063441643048, 2.241374363660425750 ) ) ;
#22252=CARTESIAN_POINT ( 'NONE',  ( 20.17069300908746854, 147.5185649274072830, -1.704009200980389771 ) ) ;
#22253=CARTESIAN_POINT ( 'NONE',  ( 7.425401986171529245, 12.64277321918224040, 4.020893088955488359 ) ) ;
#22254=EDGE_CURVE ( 'NONE', #19060, #26787, #2534, .T. ) ;
#22255=CARTESIAN_POINT ( 'NONE',  ( -14.80859988127097715, 121.7713424311148032, -1.438396347550856991 ) ) ;
#22256=CARTESIAN_POINT ( 'NONE',  ( 4.817834478233289808, 117.8426053691435840, -0.7486223446464784770 ) ) ;
#22257=CARTESIAN_POINT ( 'NONE',  ( 7.136594729663718439, 122.4194348751405101, 0.2521576392032937597 ) ) ;
#22259=CARTESIAN_POINT ( 'NONE',  ( -14.20283082469480007, 138.9094276006951247, -0.1579304324436907880 ) ) ;
#22260=CARTESIAN_POINT ( 'NONE',  ( -13.34589015847600102, 154.0568829568526041, -2.281985820853443592 ) ) ;
#22261=CARTESIAN_POINT ( 'NONE',  ( 3.172349117095228710, -15.63690262102951323, 5.390679387232247599 ) ) ;
#22264=B_SPLINE_CURVE_WITH_KNOTS ( 'NONE', 3,
 ( #23467, #36494, #7313, #16883, #32450, #35659, #16669, #33302, #29884, #3282, #23256, #20273, #26477, #35869, #17090, #22623, #39059, #16243, #30092, #10286, #12851, #6894, #25837, #91, #517, #722, #32663, #9862, #304, #13056, #19862, #22833, #32878, #36290 ),
 .UNSPECIFIED., .F., .F.,
 ( 4, 2, 2, 2, 2, 2, 2, 2, 2, 2, 2, 2, 2, 2, 2, 2, 4 ),
 ( 0.01745000530654042953, 0.01846956716767890472, 0.01948912902881738338, 0.02050869088995585857, 0.02152825275109433376, 0.02356737647337128760, 0.02458693833450976279, 0.02560650019564823798, 0.02662606205678671317, 0.02764562391792518836, 0.02866518577906366355, 0.02917496670963290462, 0.02968474764020214221, 0.03070430950134062087, 0.03172387136247909606, 0.03274343322361757125, 0.03376299508475605338 ),
 .UNSPECIFIED. ) ;
#22265=ORIENTED_EDGE ( 'NONE', *, *, #1230, .F. ) ;
#22266=CARTESIAN_POINT ( 'NONE',  ( 16.04699077284479003, 131.4332636412663931, 2.269269673164717283 ) ) ;
#22267=CARTESIAN_POINT ( 'NONE',  ( 2.666490510518176649, -13.49855353256042712, 0.05227394649444803282 ) ) ;
#22269=AXIS2_PLACEMENT_3D ( 'NONE', #16551, #17184, #30183 ) ;
#22270=CARTESIAN_POINT ( 'NONE',  ( -1.209846520933468339, 108.5039085404744981, 4.223631676023018144 ) ) ;
#22271=CARTESIAN_POINT ( 'NONE',  ( -4.342437030201590886, 23.60747082334219371, 7.218840658967335067 ) ) ;
#22272=CARTESIAN_POINT ( 'NONE',  ( 15.99655225346408649, 147.0154580547469152, 1.170958206671064206 ) ) ;
#22273=CARTESIAN_POINT ( 'NONE',  ( 14.76838793310957421, 156.1040168620350244, -0.6600470674582793462 ) ) ;
#22276=CARTESIAN_POINT ( 'NONE',  ( -0.8838529761741459323, 116.4325158421065680, -0.01766148591713742610 ) ) ;
#22277=ORIENTED_EDGE ( 'NONE', *, *, #8685, .F. ) ;
#22278=CARTESIAN_POINT ( 'NONE',  ( 6.353751754745901259, 119.9757864133673735, -0.9602761413627547427 ) ) ;
#22280=CARTESIAN_POINT ( 'NONE',  ( -4.372087114477377412, 155.8497297829079571, -0.6179351164228050752 ) ) ;
#22282=CARTESIAN_POINT ( 'NONE',  ( 21.67415503129002019, 132.7302833492884417, 0.4548691923922799640 ) ) ;
#22283=ADVANCED_FACE ( 'NONE', ( #38509 ), #41712, .T. ) ;
#22284=EDGE_LOOP ( 'NONE', ( #31498, #13691, #13583, #10784 ) ) ;
#22285=CARTESIAN_POINT ( 'NONE',  ( -0.5093740622119584671, 14.76157059199007016, 4.595130897425484306 ) ) ;
#22287=CARTESIAN_POINT ( 'NONE',  ( -4.854959790655453133, 117.4058051295649534, 0.9982048359480585331 ) ) ;
#22289=CARTESIAN_POINT ( 'NONE',  ( -3.174366308152011928, 76.29346620154572634, -0.06343139340882730792 ) ) ;
#22290=CARTESIAN_POINT ( 'NONE',  ( -7.988165842219651758, 121.7257876813687858, 0.7681561951654892750 ) ) ;
#22292=CARTESIAN_POINT ( 'NONE',  ( 0.4327634382839667393, 5.975216699623356220, -4.620561613140377055 ) ) ;
#22293=CARTESIAN_POINT ( 'NONE',  ( 17.90421410101168576, 154.0540368679750998, 1.594113676345344954 ) ) ;
#22296=CARTESIAN_POINT ( 'NONE',  ( 6.947343058555276230, 158.0090104422344268, -1.506406725519187972 ) ) ;
#22297=CARTESIAN_POINT ( 'NONE',  ( -3.394752741017290631, 119.5845705363850442, 0.6980748167159184225 ) ) ;
#22298=CARTESIAN_POINT ( 'NONE',  ( 4.198131962423935271, 12.64715247731088787, 1.959332076845688553 ) ) ;
#22299=CARTESIAN_POINT ( 'NONE',  ( -16.47501798513129145, 155.2380866766625047, -1.211716152346587361 ) ) ;
#22302=CARTESIAN_POINT ( 'NONE',  ( -0.003756957834544885893, 120.7746249494737896, 0.1880135328902414193 ) ) ;
#22303=CARTESIAN_POINT ( 'NONE',  ( 4.135482704272881449, -14.73569165307708673, 5.015242562682193039 ) ) ;
#22304=DIRECTION ( 'NONE',  ( -0.9998004120163609398, 0.000000000000000000, -0.01997839162482749689 ) ) ;
#22305=CARTESIAN_POINT ( 'NONE',  ( -4.661795382597888171, 117.9824458133873861, -0.8615256122207085587 ) ) ;
#22306=CARTESIAN_POINT ( 'NONE',  ( 14.16569067496505774, 138.8670163227233161, 0.2830642121559648339 ) ) ;
#22308=CARTESIAN_POINT ( 'NONE',  ( 18.80649797369231280, 150.3568762430427910, 2.459390564378663768 ) ) ;
#22310=CARTESIAN_POINT ( 'NONE',  ( 7.784012320830338005, 122.6313477005580665, 0.1555430910899518460 ) ) ;
#22311=CARTESIAN_POINT ( 'NONE',  ( -0.01289612358334801118, 159.5048567107479585, 0.6453747585945883714 ) ) ;
#22312=CARTESIAN_POINT ( 'NONE',  ( 4.812211268859890367, 117.4735958283970234, -1.001561189053170153 ) ) ;
#22313=CARTESIAN_POINT ( 'NONE',  ( 4.773421586889285528, 116.8420656028321218, -0.1264526730306985980 ) ) ;
#22317=CARTESIAN_POINT ( 'NONE',  ( 1.961397211334666046, -15.23659401288117365, 5.381129598871191355 ) ) ;
#22320=CARTESIAN_POINT ( 'NONE',  ( -4.567146515290242625, 118.0741377463749160, 0.6112040792829432911 ) ) ;
#22321=ORIENTED_EDGE ( 'NONE', *, *, #15211, .T. ) ;
#22325=CARTESIAN_POINT ( 'NONE',  ( 5.944196296451716321, 119.0874165451813695, -1.025244264899787483 ) ) ;
#22326=CARTESIAN_POINT ( 'NONE',  ( -4.757567707637590182, 116.6039038697339549, -1.126183464948452562 ) ) ;
#22327=CARTESIAN_POINT ( 'NONE',  ( 4.589873572828570225, 118.0230325535246010, 0.8585248486873602314 ) ) ;
#22329=CARTESIAN_POINT ( 'NONE',  ( 2.350639260211558668, -15.10312717587823705, 4.966175652281853203 ) ) ;
#22330=CARTESIAN_POINT ( 'NONE',  ( -3.199116795994628948, 156.2293907256693331, -0.9954876105832137778 ) ) ;
#22331=CARTESIAN_POINT ( 'NONE',  ( -2.393320966970525987, 115.7029491485454002, -1.700712295284147579 ) ) ;
#22332=CARTESIAN_POINT ( 'NONE',  ( -0.3678760602612873298, 105.9882361710916427, 5.283425915285953067 ) ) ;
#22333=FACE_OUTER_BOUND ( 'NONE', #4906, .T. ) ;
#22334=CARTESIAN_POINT ( 'NONE',  ( 2.668012146925189398, 107.2306503360107541, -4.624472725681509466 ) ) ;
#22335=CARTESIAN_POINT ( 'NONE',  ( -13.40752216115205542, 152.3772590505219569, -2.011877943007317704 ) ) ;
#22337=CARTESIAN_POINT ( 'NONE',  ( -4.259326390738950252, 31.70363750509472212, 4.262602491460973475 ) ) ;
#22338=CARTESIAN_POINT ( 'NONE',  ( -3.636814527154180521, 115.7029495058465045, 1.480691701714403452 ) ) ;
#22339=CARTESIAN_POINT ( 'NONE',  ( 3.700881553190929374, 8.714383148187751615, -2.768892949411812854 ) ) ;
#22340=CARTESIAN_POINT ( 'NONE',  ( 5.580240031299299908, 159.0849926622337023, 0.6989143883095926268 ) ) ;
#22341=ORIENTED_EDGE ( 'NONE', *, *, #30040, .F. ) ;
#22342=CARTESIAN_POINT ( 'NONE',  ( 4.210806622510559372, 104.6144662015456817, -2.365042981711354297 ) ) ;
#22343=CARTESIAN_POINT ( 'NONE',  ( 3.487342509456591522, -15.13654059619573644, 2.575171134517089566 ) ) ;
#22344=CARTESIAN_POINT ( 'NONE',  ( -19.58589350844871291, 147.2819018089465715, 1.740056086200069796 ) ) ;
#22345=CARTESIAN_POINT ( 'NONE',  ( 0.7587898337924254832, 1.856531735440085207, 0.6142162870750064174 ) ) ;
#22346=CARTESIAN_POINT ( 'NONE',  ( 0.5069063945870452281, 6.992850521020996801, 0.8331330811856124674 ) ) ;
#22348=ORIENTED_EDGE ( 'NONE', *, *, #26444, .F. ) ;
#22349=FACE_OUTER_BOUND ( 'NONE', #15492, .T. ) ;
#22350=CARTESIAN_POINT ( 'NONE',  ( 1.726955742647716674, 108.8931014686503289, 4.100893600158903141 ) ) ;
#22351=CARTESIAN_POINT ( 'NONE',  ( -3.602148172789818581, 120.6468399921648711, 0.3585086490597838016 ) ) ;
#22352=CARTESIAN_POINT ( 'NONE',  ( -10.18105065676974519, 125.9743313966586129, -0.2034416216762104657 ) ) ;
#22353=CARTESIAN_POINT ( 'NONE',  ( 2.851896361732738860, -14.59419570037479019, 4.638016276237491020 ) ) ;
#22354=CARTESIAN_POINT ( 'NONE',  ( 3.432158483474355037, 119.7942873563901713, -0.6544105580379840914 ) ) ;
#22355=CARTESIAN_POINT ( 'NONE',  ( -19.66043293732255748, 148.5147687316951135, -2.511426770373370587 ) ) ;
#22357=CARTESIAN_POINT ( 'NONE',  ( -2.948382749353948729, 50.63946620154572997, -1.837270642369388307 ) ) ;
#22358=CARTESIAN_POINT ( 'NONE',  ( -4.834131565410835663, 32.86531471714831554, 2.080611622871570088 ) ) ;
#22359=CARTESIAN_POINT ( 'NONE',  ( 13.12764272666522558, 133.9996589410087324, -0.1750096343312397829 ) ) ;
#22364=CARTESIAN_POINT ( 'NONE',  ( 4.889213426004227259, 117.7581299865985471, -0.6851927402696675884 ) ) ;
#22365=CARTESIAN_POINT ( 'NONE',  ( 0.7350785369229140276, 15.66647056970591301, -8.407117359194836936 ) ) ;
#22366=CARTESIAN_POINT ( 'NONE',  ( 7.769844292199929114, 122.1031240515655298, 0.8163738826679364236 ) ) ;
#22367=DIRECTION ( 'NONE',  ( 4.017660918040594346E-17, -1.000000000000000000, -2.376309959284834438E-19 ) ) ;
#22368=CARTESIAN_POINT ( 'NONE',  ( 20.50175740331280139, 129.0975500345852822, 0.3894088793431775830 ) ) ;
#22370=CARTESIAN_POINT ( 'NONE',  ( -5.267339127473358751, 116.4790307410953289, 0.8814195561379957189 ) ) ;
#22372=CARTESIAN_POINT ( 'NONE',  ( -3.178183004559932190, -7.902942162671289239, -3.366045245292264010 ) ) ;
#22373=CARTESIAN_POINT ( 'NONE',  ( -0.09153888643297225514, 38.16702564188061331, -1.140315812098650960 ) ) ;
#22374=CARTESIAN_POINT ( 'NONE',  ( 20.51891680819867503, 149.8464234248869786, 2.337676305755668871 ) ) ;
#22375=CARTESIAN_POINT ( 'NONE',  ( 8.184481992144968743, -14.99546276350015717, -2.142971516962156819 ) ) ;
#22376=CARTESIAN_POINT ( 'NONE',  ( -5.482088966821565990, 117.2431503203738714, -0.8245388645859690335 ) ) ;
#22377=CARTESIAN_POINT ( 'NONE',  ( -0.3576380314658750836, 120.7331730230137623, -0.5311352847986057224 ) ) ;
#22380=CARTESIAN_POINT ( 'NONE',  ( -3.947475993436067920, 104.6144662015413616, 3.604255196807834682 ) ) ;
#22381=ADVANCED_BREP_SHAPE_REPRESENTATION ( '', ( #38535, #3275 ), #21588 ) ;
#22382=CARTESIAN_POINT ( 'NONE',  ( -2.201963191602333225, 30.07953629247752758, -4.075912811544394998 ) ) ;
#22384=CARTESIAN_POINT ( 'NONE',  ( 2.958531772299236362, 39.20946620154573736, 1.329372033065076453 ) ) ;
#22385=CARTESIAN_POINT ( 'NONE',  ( 1.854781166956293248, -15.20994639552496253, 5.427130820981656001 ) ) ;
#22387=CARTESIAN_POINT ( 'NONE',  ( 1.590100404673003398, 118.0223913815010377, -0.9765506547304492191 ) ) ;
#22388=CARTESIAN_POINT ( 'NONE',  ( -5.848384816632850480, 117.2350771734024164, 0.3616545339607749043 ) ) ;
#22390=ORIENTED_EDGE ( 'NONE', *, *, #27142, .T. ) ;
#22393=ORIENTED_EDGE ( 'NONE', *, *, #13864, .T. ) ;
#22394=PLANE ( 'NONE',  #26722 ) ;
#22395=CARTESIAN_POINT ( 'NONE',  ( 2.745816630209086728, -15.73397280162352985, 5.435574744647863277 ) ) ;
#22396=CARTESIAN_POINT ( 'NONE',  ( -11.63724909022846177, 121.0393782313542346, 1.189926691809807036 ) ) ;
#22397=CARTESIAN_POINT ( 'NONE',  ( 22.03832501185533488, 149.1257232373000647, -1.146528549967842148 ) ) ;
#22398=CARTESIAN_POINT ( 'NONE',  ( 1.719524320724281852, 5.915668354077112667, 4.300554535892874064 ) ) ;
#22402=CARTESIAN_POINT ( 'NONE',  ( -0.1041500444723911512, 106.1822392402443143, 5.212094112990278028 ) ) ;
#22404=CARTESIAN_POINT ( 'NONE',  ( -14.44833386134795283, 131.1674235819977241, 1.369607862251506658 ) ) ;
#22406=CARTESIAN_POINT ( 'NONE',  ( 0.5101717508067669105, 119.1670848682014281, -0.5756831679880033414 ) ) ;
#22407=CARTESIAN_POINT ( 'NONE',  ( -9.341440546823601920, 157.3305555497073271, -1.901068499721874971 ) ) ;
#22410=CARTESIAN_POINT ( 'NONE',  ( 16.19917940306794790, 146.4165046419237228, -0.6472847106673340623 ) ) ;
#22412=CARTESIAN_POINT ( 'NONE',  ( -0.5205939700077546473, 119.6443647996702566, -0.5336935438815135768 ) ) ;
#22413=CARTESIAN_POINT ( 'NONE',  ( 2.733372102295486439, -15.34075898222114809, 4.536119796583970576 ) ) ;
#22414=CARTESIAN_POINT ( 'NONE',  ( -4.242447431898493271, 118.2250608216800032, -0.4715757167317731202 ) ) ;
#22416=DIRECTION ( 'NONE',  ( 0.9998004120163608288, 0.000000000000000000, 0.01997839162482749342 ) ) ;
#22418=CARTESIAN_POINT ( 'NONE',  ( -4.815137252779631893, 117.6728645535923903, 0.9184442549704321390 ) ) ;
#22419=CARTESIAN_POINT ( 'NONE',  ( 5.840731033150115437, 120.5744318282211651, 0.9509518217554208119 ) ) ;
#22421=CARTESIAN_POINT ( 'NONE',  ( -4.420329592304260480, 21.65838872207745425, -1.398650104627336743 ) ) ;
#22422=CARTESIAN_POINT ( 'NONE',  ( 2.787004648571185683, 120.9517662584847102, 0.1965090384792946565 ) ) ;
#22425=ORIENTED_EDGE ( 'NONE', *, *, #31016, .T. ) ;
#22429=CARTESIAN_POINT ( 'NONE',  ( -8.255892650435239233, 120.2042668886316505, -1.447829519518265551 ) ) ;
#22432=CARTESIAN_POINT ( 'NONE',  ( -23.31467963135047583, 142.7201128741078833, -0.1336249016415856083 ) ) ;
#22435=CARTESIAN_POINT ( 'NONE',  ( -5.947743514043456692, 121.4056990298405339, -0.2736948476934324970 ) ) ;
#22437=CARTESIAN_POINT ( 'NONE',  ( 0.7498611054318164992, 115.7030496223163567, -1.729246923944893322 ) ) ;
#22439=CARTESIAN_POINT ( 'NONE',  ( -7.814053207648073318, 154.6216606121152495, -0.3474563751001364942 ) ) ;
#22440=CARTESIAN_POINT ( 'NONE',  ( 4.669346286639404653, -14.72966438191931893, 4.552848284282712044 ) ) ;
#22441=CARTESIAN_POINT ( 'NONE',  ( -13.91986491619295663, 121.5005676099359846, 1.010465608187345321 ) ) ;
#22443=CARTESIAN_POINT ( 'NONE',  ( 23.40831777029523053, 146.8136392739129974, 0.6999192077533369361 ) ) ;
#22444=CARTESIAN_POINT ( 'NONE',  ( 2.854181719429574215, 121.0288205536620580, 0.1255016766574598708 ) ) ;
#22445=CARTESIAN_POINT ( 'NONE',  ( 4.765727645999143114, 118.5266822147775940, -0.8411891241973677991 ) ) ;
#22446=CARTESIAN_POINT ( 'NONE',  ( -0.8857237343455648393, 3.096269703755229141, -0.4102451188256627801 ) ) ;
#22447=CARTESIAN_POINT ( 'NONE',  ( -21.89464077100150163, 151.4392833230981239, -0.5893027811483438905 ) ) ;
#22449=EDGE_CURVE ( 'NONE', #10681, #9538, #5935, .T. ) ;
#22451=VERTEX_POINT ( 'NONE', #9121 ) ;
#22452=CARTESIAN_POINT ( 'NONE',  ( -2.376166872315972345, 116.5345204588131480, 0.3007191275596990954 ) ) ;
#22455=CARTESIAN_POINT ( 'NONE',  ( 12.23848595143944351, 156.6574886424908470, 1.779988832801368659 ) ) ;
#22456=CARTESIAN_POINT ( 'NONE',  ( 12.70950188986275187, 122.0451665396574725, -1.271450951352564251 ) ) ;
#22457=CARTESIAN_POINT ( 'NONE',  ( 5.111951166545567027, 11.99449087320206431, 6.736519543253151276 ) ) ;
#22458=CARTESIAN_POINT ( 'NONE',  ( -15.75167367066978485, 155.0373533369262589, -1.797107981590890358 ) ) ;
#22459=CARTESIAN_POINT ( 'NONE',  ( 4.887170171423926845, 117.7483457736543500, -0.7389058998312844073 ) ) ;
#22461=CARTESIAN_POINT ( 'NONE',  ( -7.558302675500311985, 122.4263405438208991, -0.1204446389788524086 ) ) ;
#22464=CARTESIAN_POINT ( 'NONE',  ( -1.279006062070071170, 119.0230276286704054, -0.6822954352362460284 ) ) ;
#22465=CARTESIAN_POINT ( 'NONE',  ( 3.361984464572039144, -15.63109852379819564, 5.271848418269179604 ) ) ;
#22467=CIRCLE ( 'NONE', #27270, 3.683000000000001162 ) ;
#22470=B_SPLINE_SURFACE_WITH_KNOTS ( 'NONE', 3, 3, ( 
 ( #24516, #8346, #15356, #15568, #2185, #24736, #11959, #38381, #18549, #37739, #34759, #34980, #15143, #41581, #8562, #25169, #21315 ),
 ( #5802, #5380, #8982, #22151, #21949, #34344, #35182, #18757, #12389, #37952, #31977, #24951, #8776, #5174, #14933, #21736, #31553 ),
 ( #2397, #25782, #19388, #9601, #13000, #39422, #39211, #26207, #13224, #29406, #3023, #10019, #23197, #3865, #13433, #25579, #36231 ),
 ( #25993, #19803, #9394, #26419, #39002, #3224, #6213, #9813, #20019, #22358, #6625, #38585, #460, #19184, #246, #35600, #35383 ),
 ( #10227, #15979, #32603, #22779, #6417, #32392, #35, #28976, #32189, #16185, #41996, #35810, #12793, #19592, #38790, #7052, #29624 ),
 ( #16830, #29189, #3436, #16401, #22991, #33037, #22570, #36017, #6832, #32821, #3650, #41792, #16617, #12590, #17660, #27475, #11278 ) ),
 .UNSPECIFIED., .F., .F., .F.,
 ( 4, 2, 4 ),
 ( 4, 1, 1, 1, 1, 1, 1, 1, 1, 1, 1, 1, 1, 1, 4 ),
 ( 0.000000000000000000, 0.5000000000000000000, 1.000000000000000000 ),
 ( 0.000000000000000000, 0.08300113939718137268, 0.1732806554784933895, 0.2717672377176819087, 0.3752096606209606167, 0.4787223716043260135, 0.5772295444745598747, 0.6668133826162351285, 0.7470991451079272982, 0.7815930070524458317, 0.8169452614683294644, 0.8547689062991584708, 0.8968063284581728745, 0.9447228702782888288, 1.000000000000000000 ),
 .UNSPECIFIED. ) ;
#22471=CARTESIAN_POINT ( 'NONE',  ( 5.832110448082596044, 156.9788419092994047, 1.931507550941140794 ) ) ;
#22472=CARTESIAN_POINT ( 'NONE',  ( -15.19943428492320869, 148.1072807477730748, -0.3037208696559880461 ) ) ;
#22476=CARTESIAN_POINT ( 'NONE',  ( -3.375001179497743031, 119.3320731715853782, 0.4843141097021078090 ) ) ;
#22478=CARTESIAN_POINT ( 'NONE',  ( -2.299398447937291756, 29.65396322172144039, -8.101725167555347440 ) ) ;
#22479=CARTESIAN_POINT ( 'NONE',  ( 4.418888662852166860, 155.8637389808261275, 0.7167756870077641729 ) ) ;
#22480=CARTESIAN_POINT ( 'NONE',  ( 8.141728797601116341, 117.8329967196738153, -0.4384511054415164422 ) ) ;
#22481=CARTESIAN_POINT ( 'NONE',  ( 4.822993300437530273, 117.8022149080996570, 0.9221314676250721432 ) ) ;
#22482=DIRECTION ( 'NONE',  ( -4.017660918040594346E-17, 1.000000000000000000, 2.376309959284834438E-19 ) ) ;
#22483=CARTESIAN_POINT ( 'NONE',  ( -0.2937963077019585811, 116.4254261620736344, 0.006796306282692864999 ) ) ;
#22486=CARTESIAN_POINT ( 'NONE',  ( -8.178145033566243782, 120.5865709611434369, -1.415302197751513225 ) ) ;
#22487=CARTESIAN_POINT ( 'NONE',  ( 5.819807902803178834, -14.34990091593344808, 2.641378012185163104 ) ) ;
#22488=CARTESIAN_POINT ( 'NONE',  ( -10.60367000503898538, 126.1357510980948575, -0.6849044484263042687 ) ) ;
#22489=CARTESIAN_POINT ( 'NONE',  ( 4.222548444470398010, -13.63200092856201096, 3.862739453107805421 ) ) ;
#22492=CARTESIAN_POINT ( 'NONE',  ( 20.69909148798420517, 152.5508394022679113, 0.4136171090298729758 ) ) ;
#22494=CARTESIAN_POINT ( 'NONE',  ( 4.513502956352341222, 8.064680226961385756, -0.9949261897555528034 ) ) ;
#22495=CARTESIAN_POINT ( 'NONE',  ( -11.74288454345109756, 118.7273140689154616, -0.2346507796901759757 ) ) ;
#22496=CARTESIAN_POINT ( 'NONE',  ( -21.90559427349733213, 151.4293160993572940, -0.4377259060014722092 ) ) ;
#22497=CARTESIAN_POINT ( 'NONE',  ( -0.1064799869812408512, 105.7853621660184444, 5.332934571178566507 ) ) ;
#22499=CARTESIAN_POINT ( 'NONE',  ( -6.115548012816138801, 121.1758403914483466, 0.4341407379041746784 ) ) ;
#22500=CARTESIAN_POINT ( 'NONE',  ( -4.168830513765062307, 9.198770455692846681, 1.997586429550192166 ) ) ;
#22501=CARTESIAN_POINT ( 'NONE',  ( 22.05995121575384843, 150.4421090420883900, 1.612468304426259325 ) ) ;
#22502=CARTESIAN_POINT ( 'NONE',  ( -0.07831152689652476351, 109.4728569552520838, 3.919029035233729363 ) ) ;
#22503=CARTESIAN_POINT ( 'NONE',  ( 2.906309357581933650, -13.72804873580029472, 0.7610837935892840189 ) ) ;
#22504=CARTESIAN_POINT ( 'NONE',  ( 4.041216738202956016, 118.0179939250997023, -0.7376333572805301442 ) ) ;
#22506=CARTESIAN_POINT ( 'NONE',  ( -4.168830513765062307, 9.198770455692846681, 1.997586429550192166 ) ) ;
#22507=CARTESIAN_POINT ( 'NONE',  ( -1.940752395788367446, 116.9162416783649689, -0.4172132017389482694 ) ) ;
#22508=ORIENTED_EDGE ( 'NONE', *, *, #1230, .T. ) ;
#22510=CARTESIAN_POINT ( 'NONE',  ( -14.89139266796671635, 148.8756053271976327, 0.4181552259878851818 ) ) ;
#22511=CARTESIAN_POINT ( 'NONE',  ( 6.095337826619875443, -12.40160515274643593, 0.5428006832284221206 ) ) ;
#22512=CARTESIAN_POINT ( 'NONE',  ( -6.615214180512292604E-14, 94.32746620154571815, -2.829521569843129660E-18 ) ) ;
#22513=CARTESIAN_POINT ( 'NONE',  ( -4.535049786513674519, 118.0744006754055562, -0.7972472874695084588 ) ) ;
#22514=CARTESIAN_POINT ( 'NONE',  ( 7.044606587285096033, 122.0729346620515088, 0.1407680048458705979 ) ) ;
#22516=CARTESIAN_POINT ( 'NONE',  ( 14.77311812546545156, 125.6006210965460781, 2.040279103193882282 ) ) ;
#22517=DIRECTION ( 'NONE',  ( -0.9998004120163609398, -5.205824365704083189E-17, -0.01997839162482749689 ) ) ;
#22518=DIRECTION ( 'NONE',  ( -4.017660918040594346E-17, 1.000000000000000000, 2.376309959284834438E-19 ) ) ;
#22520=CARTESIAN_POINT ( 'NONE',  ( -14.14567801931327118, 120.5239346615589540, 0.5295366371686062168 ) ) ;
#22522=CARTESIAN_POINT ( 'NONE',  ( 0.0005468344958371703160, 156.3034662015456604, -0.02736583427618478198 ) ) ;
#22523=CARTESIAN_POINT ( 'NONE',  ( 15.06072413439829027, 156.1474796653986630, -0.2161187639505615099 ) ) ;
#22532=CARTESIAN_POINT ( 'NONE',  ( -4.605735037197680626, 118.0200015956283863, 0.6870595234115985939 ) ) ;
#22535=ORIENTED_EDGE ( 'NONE', *, *, #35079, .F. ) ;
#22537=( BOUNDED_SURFACE ( )  B_SPLINE_SURFACE ( 3, 2, ( 
 ( #26604, #13614, #33011 ),
 ( #37044, #33849, #7862 ),
 ( #27237, #36419, #7445 ),
 ( #40251, #1272, #29806 ),
 ( #39611, #10833, #23604 ),
 ( #4470, #33223, #13823 ),
 ( #20403, #14023, #23387 ),
 ( #4677, #7237, #30426 ),
 ( #36625, #20197, #4050 ),
 ( #7656, #26392, #17011 ),
 ( #11044, #24029, #30010 ),
 ( #16803, #10199, #849 ),
 ( #39828, #10622, #27030 ),
 ( #17634, #30636, #36836 ),
 ( #33433, #17427, #4260 ),
 ( #17223, #33643, #39397 ),
 ( #8061, #11666, #21036 ),
 ( #5508, #24872, #34060 ),
 ( #18466, #31686, #40658 ),
 ( #4888, #21653, #21867 ) ),
 .UNSPECIFIED., .F., .F., .T. ) 
 B_SPLINE_SURFACE_WITH_KNOTS ( ( 4, 2, 2, 2, 2, 2, 2, 2, 2, 4 ),
 ( 3, 3 ),
 ( -2.835263634875403419E-05, 0.001133586441676013700, 0.001714555980688397662, 0.002295525519700781624, 0.003457464597725549114, 0.003747949367231741095, 0.004038434136737933076, 0.004183676521491029067, 0.004328918906244125057, 0.004619403675750317038 ),
 ( 0.000000000000000000, 0.7115407172542784764 ),
 .UNSPECIFIED. ) 
 GEOMETRIC_REPRESENTATION_ITEM ( )  RATIONAL_B_SPLINE_SURFACE ( (
 ( 1.000000000000000000, 0.8295190889138120971, 0.9016463973324821968),
 ( 1.000000000000000000, 0.8295190889138120971, 0.9016463973324821968),
 ( 1.000000000000000000, 0.8295191357741429350, 0.9016464243670769818),
 ( 1.000000000000000000, 0.8295190646856472894, 0.9016463833548040707),
 ( 1.000000000000000000, 0.8295185271377292224, 0.9016460732334303785),
 ( 1.000000000000000000, 0.8295186176601453409, 0.9016461254574927864),
 ( 1.000000000000000000, 0.8295190559657723561, 0.9016463783241464025),
 ( 1.000000000000000000, 0.8295191606352591007, 0.9016464387099165645),
 ( 1.000000000000000000, 0.8295190986999689819, 0.9016464029782977896),
 ( 1.000000000000000000, 0.8295190867078258146, 0.9016463960598077865),
 ( 1.000000000000000000, 0.8295190998541304150, 0.9016464036441549368),
 ( 1.000000000000000000, 0.8295190811289877564, 0.9016463928412725704),
 ( 1.000000000000000000, 0.8295192486502576124, 0.9016464894874032243),
 ( 1.000000000000000000, 0.8295190462722409341, 0.9016463727317682864),
 ( 1.000000000000000000, 0.8295188582200193617, 0.9016462642409502903),
 ( 1.000000000000000000, 0.8295187249109206018, 0.9016461873324561616),
 ( 1.000000000000000000, 0.8295190035458798183, 0.9016463480821370613),
 ( 1.000000000000000000, 0.8295192259831494219, 0.9016464764103275797),
 ( 1.000000000000000000, 0.8295190889132049161, 0.9016463973321320324),
 ( 1.000000000000000000, 0.8295190889132049161, 0.9016463973321320324) ) ) 
 REPRESENTATION_ITEM ( '' )  SURFACE ( )  );
#22538=CARTESIAN_POINT ( 'NONE',  ( 8.447822738470250670, 119.5131637967545259, -1.065025361500244072 ) ) ;
#22539=CARTESIAN_POINT ( 'NONE',  ( -5.888892352462247182, 118.9932487913337411, -0.5850130909721117378 ) ) ;
#22540=CARTESIAN_POINT ( 'NONE',  ( 4.784214230320843697, 117.8428681949036729, 0.9402043361855015879 ) ) ;
#22541=CARTESIAN_POINT ( 'NONE',  ( 2.906309357581933650, -13.72804873580029472, 0.7610837935892840189 ) ) ;
#22542=CARTESIAN_POINT ( 'NONE',  ( -3.584950684498069418, 120.6468399921648711, -0.5021239885730617303 ) ) ;
#22544=CARTESIAN_POINT ( 'NONE',  ( -0.6265688110002558542, 106.0241047940699559, 5.258438125228670046 ) ) ;
#22545=CARTESIAN_POINT ( 'NONE',  ( 5.755298473670368509, 118.4539739381501988, -0.4326931426192709429 ) ) ;
#22546=CARTESIAN_POINT ( 'NONE',  ( -6.534901955149031494, 120.8223817900871495, -1.022280983926979303 ) ) ;
#22548=CARTESIAN_POINT ( 'NONE',  ( -0.01887972822151516225, 159.3676309965788960, 0.9448188026860502298 ) ) ;
#22550=CARTESIAN_POINT ( 'NONE',  ( 4.440276399826426967, -1.430929408009915083, -1.287880193523989636 ) ) ;
#22551=CARTESIAN_POINT ( 'NONE',  ( 5.825324126169723726, 117.1711376449269721, 0.5405197603966794828 ) ) ;
#22552=ORIENTED_EDGE ( 'NONE', *, *, #25321, .T. ) ;
#22554=CARTESIAN_POINT ( 'NONE',  ( 3.555255404795384599, -15.46298345743583802, 3.323699395844104565 ) ) ;
#22555=CARTESIAN_POINT ( 'NONE',  ( -19.37548274631734557, 145.1342744731992127, 1.755133555010167656 ) ) ;
#22556=CARTESIAN_POINT ( 'NONE',  ( 0.6214172073067296687, 11.15065110656550118, 0.7500636867869169278 ) ) ;
#22558=CARTESIAN_POINT ( 'NONE',  ( -0.9676832378731173856, 3.540085264489355676, -0.1409938603398425416 ) ) ;
#22562=CARTESIAN_POINT ( 'NONE',  ( 3.138057391968664067, 117.6701293611589278, 1.012097185230346419 ) ) ;
#22564=CARTESIAN_POINT ( 'NONE',  ( -10.66674206690823468, 124.7671305375842934, 0.7411263988551110016 ) ) ;
#22565=CARTESIAN_POINT ( 'NONE',  ( 3.901187470525758094, -13.68826627043556776, 3.907672046116945186 ) ) ;
#22566=CARTESIAN_POINT ( 'NONE',  ( 1.391675519083714674, 119.6596719632383383, -0.5469696729655012524 ) ) ;
#22567=CARTESIAN_POINT ( 'NONE',  ( 0.01152893261308097703, 118.7114655739656257, -0.5769549317675698452 ) ) ;
#22568=DIRECTION ( 'NONE',  ( 4.017660918040594346E-17, -1.000000000000000000, -2.376309959284834438E-19 ) ) ;
#22569=CARTESIAN_POINT ( 'NONE',  ( 8.232931626680233705, 120.3169219327360508, 1.441413524645123623 ) ) ;
#22570=CARTESIAN_POINT ( 'NONE',  ( -2.579283729523311752, 34.63205429821886838, 0.7922911722492691489 ) ) ;
#22571=CARTESIAN_POINT ( 'NONE',  ( 14.35733687469664410, 139.0340687859245463, -0.1707862337897577132 ) ) ;
#22576=CARTESIAN_POINT ( 'NONE',  ( 3.584950684497941076, 120.6468399921648711, 0.5021239885730618413 ) ) ;
#22578=CARTESIAN_POINT ( 'NONE',  ( 0.3004615168031275485, 116.4565202671238069, -0.06108086412306412694 ) ) ;
#22579=CARTESIAN_POINT ( 'NONE',  ( -0.8832484628483068256, 105.9424719104300436, 5.282093952356136768 ) ) ;
#22581=DIRECTION ( 'NONE',  ( 0.01997839162482749689, 1.040247600000945640E-18, -0.9998004120163610509 ) ) ;
#22582=CARTESIAN_POINT ( 'NONE',  ( -3.594857975007920814, -7.703025367003809798, -2.923569511714296798 ) ) ;
#22583=CARTESIAN_POINT ( 'NONE',  ( -4.530671860764704739, 32.23439806600806889, 0.8345080972855752899 ) ) ;
#22584=CARTESIAN_POINT ( 'NONE',  ( -0.02874440110946640745, 158.8294072187990196, 1.438487372358303373 ) ) ;
#22585=CARTESIAN_POINT ( 'NONE',  ( 2.264360804680111805, 21.29314879275315064, 4.027482774281332389 ) ) ;
#22586=CARTESIAN_POINT ( 'NONE',  ( -7.958381229837070414, -11.09356959825496247, -2.748999415197344476 ) ) ;
#22587=CARTESIAN_POINT ( 'NONE',  ( -5.485516209714965008, 117.1863486007777766, -0.7935004768815202558 ) ) ;
#22588=CARTESIAN_POINT ( 'NONE',  ( -2.988627099741104853, 122.7580772961051707, -0.2146329844597061054 ) ) ;
#22589=CARTESIAN_POINT ( 'NONE',  ( 0.01793833495430298061, 118.1627382089642566, -0.8977079103094813828 ) ) ;
#22590=CARTESIAN_POINT ( 'NONE',  ( 1.769773243241540950, 106.5493969454534522, -4.971304634441370496 ) ) ;
#22591=CARTESIAN_POINT ( 'NONE',  ( -0.2386208842475691927, 105.1223928365816391, 5.340289220565798800 ) ) ;
#22592=CARTESIAN_POINT ( 'NONE',  ( -4.563195415240126174, 21.88328375387019165, -0.7336086519975816289 ) ) ;
#22593=FACE_OUTER_BOUND ( 'NONE', #30468, .T. ) ;
#22595=CARTESIAN_POINT ( 'NONE',  ( 3.116451998213339625, -14.00698646007624149, 1.619014592372306716 ) ) ;
#22596=CARTESIAN_POINT ( 'NONE',  ( 1.626581124784194143, 119.3928400758114918, -0.6183738137425958126 ) ) ;
#22597=CARTESIAN_POINT ( 'NONE',  ( -4.817281438370394575, 117.0090399748681875, 0.3002870190743006651 ) ) ;
#22598=AXIS2_PLACEMENT_3D ( 'NONE', #15783, #28791, #41803 ) ;
#22602=CARTESIAN_POINT ( 'NONE',  ( -3.113414239748029111, 30.98679946927233431, 0.04088859964249514506 ) ) ;
#22603=CARTESIAN_POINT ( 'NONE',  ( 3.743762692837560468, -15.60843739440008449, 4.988928788737716502 ) ) ;
#22604=CARTESIAN_POINT ( 'NONE',  ( -11.48785675552158381, 156.2473422840488979, 1.634126210350451691 ) ) ;
#22605=CARTESIAN_POINT ( 'NONE',  ( 9.403995501905139776, 118.7255599110314961, -0.7521618898589477187 ) ) ;
#22606=CARTESIAN_POINT ( 'NONE',  ( 3.064284189169764971, -3.155149710853871525, 3.465721614369133174 ) ) ;
#22610=CARTESIAN_POINT ( 'NONE',  ( -0.001862839608873425017, 124.0591982226671490, 0.09322411149286721765 ) ) ;
#22611=CARTESIAN_POINT ( 'NONE',  ( -11.67916898317110785, 124.4569610989641859, 1.132436424213030035 ) ) ;
#22613=CARTESIAN_POINT ( 'NONE',  ( 12.69690185265270266, 124.0847267554996591, -1.337322108705696566 ) ) ;
#22614=CARTESIAN_POINT ( 'NONE',  ( -18.59893286765449005, 151.9584835496716266, -2.273025404440324859 ) ) ;
#22618=CARTESIAN_POINT ( 'NONE',  ( 4.591905152882217678, 118.0813191133225217, -0.5393609360573334843 ) ) ;
#22619=CARTESIAN_POINT ( 'NONE',  ( 16.15477348297510574, 145.8839827664328368, -0.6502963436359732174 ) ) ;
#22621=CARTESIAN_POINT ( 'NONE',  ( -10.58192191572921637, 122.8495954190337898, -1.525858888728604645 ) ) ;
#22622=CARTESIAN_POINT ( 'NONE',  ( 1.983586949722073500, -15.35435952563934947, 5.265070481109153988 ) ) ;
#22623=CARTESIAN_POINT ( 'NONE',  ( -0.5136306012015983136, 105.1226572023712009, -5.319725606971133836 ) ) ;
#22626=CARTESIAN_POINT ( 'NONE',  ( -4.862062482173646671, 117.7349268748283322, 0.8245466556072992281 ) ) ;
#22627=CARTESIAN_POINT ( 'NONE',  ( 3.575075884023247053, 156.6183338678525558, 1.521800568792661235 ) ) ;
#22629=CARTESIAN_POINT ( 'NONE',  ( 8.369515367582838650, -11.69187915512254783, 0.7729349465547848963 ) ) ;
#22630=CARTESIAN_POINT ( 'NONE',  ( 9.242391706085484770, 124.1957968681474824, 0.3461533994140004178 ) ) ;
#22634=VECTOR ( 'NONE', #31050, 1000.000000000000227 ) ;
#22637=CARTESIAN_POINT ( 'NONE',  ( -8.537794462167497045, 118.8508514274944332, -1.228900455792910407 ) ) ;
#22642=CARTESIAN_POINT ( 'NONE',  ( -11.62351318166555458, 118.7506923092098674, 0.05658863777226878777 ) ) ;
#22645=ORIENTED_EDGE ( 'NONE', *, *, #40941, .F. ) ;
#22647=CARTESIAN_POINT ( 'NONE',  ( 6.037966007429210968, 121.4449702037965295, 0.07866225072108197491 ) ) ;
#22649=CARTESIAN_POINT ( 'NONE',  ( 3.151445404061590683, 115.7029491485452866, -1.538701385061280069 ) ) ;
#22650=CARTESIAN_POINT ( 'NONE',  ( -9.132214679254637701, 153.9061766533773152, -0.3822102345680641888 ) ) ;
#22651=CARTESIAN_POINT ( 'NONE',  ( 6.072898904334845582, -12.55662260458653634, 0.7994981368886315831 ) ) ;
#22652=CARTESIAN_POINT ( 'NONE',  ( -6.847865590701599281, 118.2876074772933492, 0.8134140678991771400 ) ) ;
#22655=CARTESIAN_POINT ( 'NONE',  ( 13.56676737375326347, 119.6371495169912436, 0.4909217195147886348 ) ) ;
#22656=CARTESIAN_POINT ( 'NONE',  ( 2.871147452325312432, 156.1036873960511286, 0.1443595091093279881 ) ) ;
#22658=CARTESIAN_POINT ( 'NONE',  ( 0.1941685572964340079, 16.06069190514159928, 0.9568941237268799860 ) ) ;
#22659=CARTESIAN_POINT ( 'NONE',  ( -23.34655412193315982, 148.8653451956335516, -0.6207958181910344653 ) ) ;
#22661=CARTESIAN_POINT ( 'NONE',  ( -5.237832120027546168, 115.7029491485453718, -1.023639123012231034 ) ) ;
#22663=CARTESIAN_POINT ( 'NONE',  ( 2.467838008569906982, 116.7125891676179492, 0.4911571291703088482 ) ) ;
#22664=ORIENTED_EDGE ( 'NONE', *, *, #10739, .T. ) ;
#22666=CARTESIAN_POINT ( 'NONE',  ( 4.913347341789697786, 118.0342071775839941, 0.9606804153092149967 ) ) ;
#22667=CARTESIAN_POINT ( 'NONE',  ( 8.792330854012570640, 120.0394951565550343, -1.134075770671235217 ) ) ;
#22668=CARTESIAN_POINT ( 'NONE',  ( -0.4837089014371968032, -0.2951250844416551944, 0.8451309203121293301 ) ) ;
#22669=CARTESIAN_POINT ( 'NONE',  ( -4.414756536061148928, 7.050034479431100287, -7.184669936685727620 ) ) ;
#22670=CARTESIAN_POINT ( 'NONE',  ( -9.289280848106855615, 118.8811571165754941, -1.201727579052786377 ) ) ;
#22671=CARTESIAN_POINT ( 'NONE',  ( 4.663464417680016183, 117.9609724899354859, -0.7408843369873798768 ) ) ;
#22673=CARTESIAN_POINT ( 'NONE',  ( -4.224755116450005232, 155.8535809751167562, -0.04780361979672655831 ) ) ;
#22675=CARTESIAN_POINT ( 'NONE',  ( -6.619107555072970328, 119.9895581359321994, -1.245414878088068056 ) ) ;
#22676=CARTESIAN_POINT ( 'NONE',  ( 4.276943344491330734, -15.69687736684960377, 3.951204673509490117 ) ) ;
#22678=CARTESIAN_POINT ( 'NONE',  ( 4.787409750893364624, 118.5931160184169073, 0.9399879859136054394 ) ) ;
#22681=ORIENTED_EDGE ( 'NONE', *, *, #7621, .T. ) ;
#22682=CARTESIAN_POINT ( 'NONE',  ( 2.442377090744232149, 119.5064228623769225, 0.7372000016323178029 ) ) ;
#22684=AXIS2_PLACEMENT_3D ( 'NONE', #21903, #25330, #41111 ) ;
#22685=CARTESIAN_POINT ( 'NONE',  ( -4.548929788228186943, 119.7344140837147819, 0.3435137807816315836 ) ) ;
#22686=CARTESIAN_POINT ( 'NONE',  ( 8.431793794909870243, 26.85621209503467455, -0.1224882448600171925 ) ) ;
#22687=CARTESIAN_POINT ( 'NONE',  ( 5.232823448427218693, 121.2166884500396833, 0.3893023073710020210 ) ) ;
#22689=CARTESIAN_POINT ( 'NONE',  ( 7.773589648320840872, 158.6130819278358501, -0.6584978287542903042 ) ) ;
#22693=CARTESIAN_POINT ( 'NONE',  ( -6.555005513994535572E-14, 79.34146620154574236, -6.390659674827382268E-18 ) ) ;
#22695=CARTESIAN_POINT ( 'NONE',  ( -1.798461198689529583, 116.4670535197835051, -0.02282230188723645067 ) ) ;
#22697=CARTESIAN_POINT ( 'NONE',  ( 6.372047788406695723, 120.0155008613895262, -0.9547430740777989033 ) ) ;
#22698=CARTESIAN_POINT ( 'NONE',  ( 22.46755768833288158, 150.8526571111528654, 0.4489552724284878171 ) ) ;
#22699=VECTOR ( 'NONE', #15105, 1000.000000000000000 ) ;
#22700=CARTESIAN_POINT ( 'NONE',  ( -8.208845571667785279, 122.7966848691156514, -0.5426025200548864058 ) ) ;
#22701=CARTESIAN_POINT ( 'NONE',  ( 2.073997095138572000, -14.95492255878227894, 5.604884748988061105 ) ) ;
#22702=CARTESIAN_POINT ( 'NONE',  ( -5.125197423627203541, 116.9874462378649156, 0.2390140417207006485 ) ) ;
#22703=CARTESIAN_POINT ( 'NONE',  ( 6.896076486346172096, 117.1676486657671177, 0.1523180551073342603 ) ) ;
#22704=ORIENTED_EDGE ( 'NONE', *, *, #20655, .T. ) ;
#22705=CARTESIAN_POINT ( 'NONE',  ( -4.603678009535974169, 12.38766144714272066, -0.4343361176327051321 ) ) ;
#22707=CARTESIAN_POINT ( 'NONE',  ( 0.8498849898440922201, 105.1231291862523562, 5.276109398275504958 ) ) ;
#22708=CARTESIAN_POINT ( 'NONE',  ( -4.801770124674531459, 117.3993836138989479, 1.016061141329191786 ) ) ;
#22709=CARTESIAN_POINT ( 'NONE',  ( 3.686126148285236770, 108.9297438659294670, 3.861031192209934737 ) ) ;
#22710=CARTESIAN_POINT ( 'NONE',  ( 7.821621632655430645, 122.4026362592563260, 0.6204867030296015162 ) ) ;
#22712=CARTESIAN_POINT ( 'NONE',  ( 3.547999066118234346, 14.38381850277834317, -2.990331240093012433 ) ) ;
#22713=CARTESIAN_POINT ( 'NONE',  ( 22.54106487284166960, 146.4122051224262577, 1.767531409769413475 ) ) ;
#22716=CARTESIAN_POINT ( 'NONE',  ( 21.01144550848343684, 149.0309112320384486, -1.514039682450821322 ) ) ;
#22717=CARTESIAN_POINT ( 'NONE',  ( 1.100877510726109954, 5.750359496286542971, -4.487862572965156005 ) ) ;
#22718=CARTESIAN_POINT ( 'NONE',  ( -16.38310316169965830, 155.2191194103077407, -1.312707330359597302 ) ) ;
#22719=EDGE_CURVE ( 'NONE', #10933, #22232, #12266, .T. ) ;
#22721=CARTESIAN_POINT ( 'NONE',  ( -1.588992450109173449, 120.9073379818811134, 0.1002710119552034512 ) ) ;
#22722=CARTESIAN_POINT ( 'NONE',  ( 5.314795342858649185, -13.92002763284938638, 3.476347616104731753 ) ) ;
#22723=CARTESIAN_POINT ( 'NONE',  ( 0.1695430583838596905, 115.7029491485453718, 1.764635982249148638 ) ) ;
#22724=ORIENTED_EDGE ( 'NONE', *, *, #35707, .T. ) ;
#22725=CARTESIAN_POINT ( 'NONE',  ( -0.03256023585726924852, 157.9544661776888290, 1.629447346748784664 ) ) ;
#22727=CYLINDRICAL_SURFACE ( 'NONE', #15037, 5.588000000000006295 ) ;
#22728=CARTESIAN_POINT ( 'NONE',  ( -0.3541790919672200832, 116.9919054422455531, 0.3273860145854424752 ) ) ;
#22729=CARTESIAN_POINT ( 'NONE',  ( 8.185302851676453884, 117.6493956690293317, -0.2478838862282036759 ) ) ;
#22731=CARTESIAN_POINT ( 'NONE',  ( -6.437058721807690810E-14, 62.83146620154573014, 4.519164521849267879E-29 ) ) ;
#22733=CARTESIAN_POINT ( 'NONE',  ( 1.850362377257448232, -15.22409370683930341, 5.412180775546769240 ) ) ;
#22736=CARTESIAN_POINT ( 'NONE',  ( -4.610742620264918656, 118.0210047857977003, 0.6828504890990388931 ) ) ;
#22742=CARTESIAN_POINT ( 'NONE',  ( -3.570975303727345285, 118.7434192143189620, -0.9358452737509639352 ) ) ;
#22744=CARTESIAN_POINT ( 'NONE',  ( -5.011858831344667031, 114.3657942991566472, -1.958205155698268696 ) ) ;
#22745=CARTESIAN_POINT ( 'NONE',  ( 4.659120009405922858, 117.9637684512630500, 0.9018216066107574980 ) ) ;
#22746=CARTESIAN_POINT ( 'NONE',  ( 2.769760999665409340, -14.92388480464812872, 4.423285184949336646 ) ) ;
#22747=CARTESIAN_POINT ( 'NONE',  ( -1.501069045181644634, 120.4980338609919386, -0.3776272143368911149 ) ) ;
#22751=CARTESIAN_POINT ( 'NONE',  ( 5.300219172352869990, 116.7134249176580028, -0.8085863681920514301 ) ) ;
#22752=CARTESIAN_POINT ( 'NONE',  ( -16.85437733762588763, 144.1809451582817587, -2.058110026898293921 ) ) ;
#22754=CARTESIAN_POINT ( 'NONE',  ( -0.02768730785358111679, 158.9256195073445213, 1.385586103196075891 ) ) ;
#22755=CARTESIAN_POINT ( 'NONE',  ( -6.733080298864849599E-14, 123.6644662015457214, 4.141858957710797243E-18 ) ) ;
#22756=CARTESIAN_POINT ( 'NONE',  ( -15.52860580939315227, 147.5347899789022392, -0.2435143895907615208 ) ) ;
#22757=CARTESIAN_POINT ( 'NONE',  ( -4.550674770548566173, 2.667180226961371137, -0.8080508602523946982 ) ) ;
#22758=CARTESIAN_POINT ( 'NONE',  ( 16.67457936879062785, 122.7093839631038463, 0.9722687365115705305 ) ) ;
#22760=CARTESIAN_POINT ( 'NONE',  ( 5.024208363535699107, 104.6144662015413900, -1.824882619888055002 ) ) ;
#22761=CARTESIAN_POINT ( 'NONE',  ( 3.351832917607362461, -15.21525542808549503, 3.277475278119628133 ) ) ;
#22762=CARTESIAN_POINT ( 'NONE',  ( -12.30591244053544564, 123.0735437985678971, 1.316165607245708635 ) ) ;
#22763=CARTESIAN_POINT ( 'NONE',  ( 0.2555639604167124768, 10.49987491555810593, 0.9396316490698124468 ) ) ;
#22764=CARTESIAN_POINT ( 'NONE',  ( -2.832181158176262592, 116.7549172960530939, -0.3515502119895594912 ) ) ;
#22766=CARTESIAN_POINT ( 'NONE',  ( -0.9658880162092680077, 3.969362202269336226, 0.1338930134723784471 ) ) ;
#22767=ORIENTED_EDGE ( 'NONE', *, *, #2212, .T. ) ;
#22770=CARTESIAN_POINT ( 'NONE',  ( -0.1065646865916383690, 105.8844662015456919, 5.332932678536313809 ) ) ;
#22772=AXIS2_PLACEMENT_3D ( 'NONE', #26824, #23819, #19996 ) ;
#22773=CARTESIAN_POINT ( 'NONE',  ( -9.814938192569949038, 124.1138826855306831, 0.4990610963926597754 ) ) ;
#22774=CARTESIAN_POINT ( 'NONE',  ( 2.474817137005230983, -14.89163965485640340, 5.628581999208025266 ) ) ;
#22775=CARTESIAN_POINT ( 'NONE',  ( 15.29320056080882040, 150.6904849259475441, -1.473493523582195097 ) ) ;
#22776=CARTESIAN_POINT ( 'NONE',  ( -1.027076152783870544, 158.1148137021529578, -1.645667644272182484 ) ) ;
#22778=CARTESIAN_POINT ( 'NONE',  ( 8.267145744840583177, 120.1492222882854009, 1.449473100370770817 ) ) ;
#22779=CARTESIAN_POINT ( 'NONE',  ( -0.5377276166119240308, 37.39316116396758360, -0.3507468784153330299 ) ) ;
#22780=CARTESIAN_POINT ( 'NONE',  ( 15.80820582674403951, 146.9282941555416073, -0.1367419433413213647 ) ) ;
#22781=VERTEX_POINT ( 'NONE', #4008 ) ;
#22786=CARTESIAN_POINT ( 'NONE',  ( 22.53108783561238226, 150.7873321363286152, 0.2974592429706746644 ) ) ;
#22787=CARTESIAN_POINT ( 'NONE',  ( -0.3646759018191795265, 105.8822825325953261, 5.328619312200441271 ) ) ;
#22788=DIRECTION ( 'NONE',  ( 0.9998004120163608288, 0.000000000000000000, 0.01997839162482749342 ) ) ;
#22789=DIRECTION ( 'NONE',  ( -4.017660918040594346E-17, 1.000000000000000000, 2.376309959284834438E-19 ) ) ;
#22790=CARTESIAN_POINT ( 'NONE',  ( -0.7874499056167989508, 36.06947511884756352, -0.2613531129797825869 ) ) ;
#22791=CARTESIAN_POINT ( 'NONE',  ( 2.740693480742271149, 158.6924860557018064, 1.553331106148862606 ) ) ;
#22793=CARTESIAN_POINT ( 'NONE',  ( 1.027636191897724816, 24.96647085856908532, -4.506105791511280323 ) ) ;
#22794=CARTESIAN_POINT ( 'NONE',  ( -6.736519641741455899, -9.595509028896938020, 5.111951147309959254 ) ) ;
#22795=CARTESIAN_POINT ( 'NONE',  ( -8.717398971979335442, 118.0183826319925373, -0.7839213143053921362 ) ) ;
#22796=CARTESIAN_POINT ( 'NONE',  ( -3.315449255180983545, 124.9344662015457743, -0.06625056644921928362 ) ) ;
#22797=CARTESIAN_POINT ( 'NONE',  ( 5.511035053980530840, -11.68933965407963704, 0.7135650660036900739 ) ) ;
#22799=CARTESIAN_POINT ( 'NONE',  ( -0.9366858060089110483, 104.6144662015478701, 5.262845480310400781 ) ) ;
#22800=CARTESIAN_POINT ( 'NONE',  ( 3.400481176189167343, 25.78150505744974552, 3.158589348000393482 ) ) ;
#22802=CARTESIAN_POINT ( 'NONE',  ( 2.857130780617909149, -14.87311083204414786, 4.269097905712053276 ) ) ;
#22803=CARTESIAN_POINT ( 'NONE',  ( 2.387353046264464762, 119.4803856251332945, -0.5366433100809052670 ) ) ;
#22804=CARTESIAN_POINT ( 'NONE',  ( -22.26937170471362748, 150.7043692363948537, 0.4001190995498107861 ) ) ;
#22807=EDGE_CURVE ( 'NONE', #450, #38156, #11528, .T. ) ;
#22809=FACE_OUTER_BOUND ( 'NONE', #25581, .T. ) ;
#22810=CARTESIAN_POINT ( 'NONE',  ( 2.631220017305710090, -15.63525587843500553, 5.668892982663133573 ) ) ;
#22811=CARTESIAN_POINT ( 'NONE',  ( -20.44439181834797381, 148.1475078817917961, 1.665223645801947816 ) ) ;
#22812=CARTESIAN_POINT ( 'NONE',  ( 6.847865590701471383, 118.2876074772933492, -0.8134140678991769180 ) ) ;
#22814=CARTESIAN_POINT ( 'NONE',  ( -4.609222696788063622, 3.091975128091568159, 0.4746723485708761459 ) ) ;
#22816=VERTEX_POINT ( 'NONE', #37202 ) ;
#22818=CARTESIAN_POINT ( 'NONE',  ( -0.007670926890914411475, 121.5961256765098284, 0.3838845493044711343 ) ) ;
#22819=( NAMED_UNIT ( * ) SI_UNIT ( $, .STERADIAN. ) SOLID_ANGLE_UNIT ( ) );
#22821=CARTESIAN_POINT ( 'NONE',  ( -0.8674473734594028151, 156.8926940187749324, 1.309446568524254673 ) ) ;
#22822=CARTESIAN_POINT ( 'NONE',  ( 5.071597197228429721, 117.1436960276084278, 0.6009254234287543239 ) ) ;
#22823=CARTESIAN_POINT ( 'NONE',  ( 18.88959041316438459, 148.1672603684278329, -1.723054188180887403 ) ) ;
#22824=CARTESIAN_POINT ( 'NONE',  ( -18.34395142906178222, 131.7683309214445728, -2.187682908440787610 ) ) ;
#22827=CARTESIAN_POINT ( 'NONE',  ( 4.462286611852313456, 118.1590011982771244, -0.4284256476081526599 ) ) ;
#22828=CARTESIAN_POINT ( 'NONE',  ( 13.64865021167016046, 134.2686865373913463, -0.6688813089635637921 ) ) ;
#22829=VECTOR ( 'NONE', #2599, 1000.000000000000227 ) ;
#22831=CARTESIAN_POINT ( 'NONE',  ( -17.71853448156636901, 146.5573550606970628, -2.243325415855147664 ) ) ;
#22832=CARTESIAN_POINT ( 'NONE',  ( 2.429471885602138670, -15.51652123318236676, 4.968198114871331228 ) ) ;
#22833=CARTESIAN_POINT ( 'NONE',  ( -5.287127330377648704, 105.1224767669196183, -0.7827282581152339436 ) ) ;
#22835=CARTESIAN_POINT ( 'NONE',  ( -4.852690634155996108, 117.6441829300342334, 0.9099436388107151608 ) ) ;
#22836=CARTESIAN_POINT ( 'NONE',  ( 2.508893989683063541, 119.8406177399916714, 0.6723988897110715346 ) ) ;
#22838=CARTESIAN_POINT ( 'NONE',  ( -4.559029627765868398, 31.49133049583988253, -0.6947656260628575220 ) ) ;
#22839=CARTESIAN_POINT ( 'NONE',  ( 9.051149985088882133, 123.9289873439938674, 0.3396360471471667752 ) ) ;
#22842=CARTESIAN_POINT ( 'NONE',  ( -5.562698904337072925, 116.6986079444752846, -0.1401370167873323136 ) ) ;
#22843=CARTESIAN_POINT ( 'NONE',  ( 4.799643950526473191, 115.7029491485453292, 1.472414092453835588 ) ) ;
#22846=DIRECTION ( 'NONE',  ( -0.9998004120163609398, -4.016384292689130894E-17, -0.01997839162482749689 ) ) ;
#22848=CARTESIAN_POINT ( 'NONE',  ( -4.074955089416341991, 118.2429491485453354, 0.1454234154749719787 ) ) ;
#22849=CARTESIAN_POINT ( 'NONE',  ( -6.484670282503085616E-14, 71.97546620154574271, 3.533028205012241021E-29 ) ) ;
#22853=CARTESIAN_POINT ( 'NONE',  ( -15.79392588796415353, 121.0087326939336378, -0.08323308591264573508 ) ) ;
#22858=CARTESIAN_POINT ( 'NONE',  ( 6.071239300402657690, 121.4397587287365639, 0.1177787590444958898 ) ) ;
#22859=ORIENTED_EDGE ( 'NONE', *, *, #38592, .T. ) ;
#22861=CARTESIAN_POINT ( 'NONE',  ( -8.071037755103120048, 122.8559727437779827, -0.2401247476687868587 ) ) ;
#22862=CARTESIAN_POINT ( 'NONE',  ( 5.767107246999573889, -13.94705323133380048, 2.761945726399152701 ) ) ;
#22863=CARTESIAN_POINT ( 'NONE',  ( -18.85936551755652246, 131.8417273817641444, 1.350502370828212673 ) ) ;
#22865=CARTESIAN_POINT ( 'NONE',  ( 23.25077945365668342, 149.0206351951634076, 0.9193108337986204415 ) ) ;
#22866=CARTESIAN_POINT ( 'NONE',  ( 8.436454488239842675, 123.3184168920685551, 0.2537209124029990437 ) ) ;
#22867=CARTESIAN_POINT ( 'NONE',  ( 5.065658811076494850, 115.6909491485453145, -1.197684230374509218 ) ) ;
#22868=CARTESIAN_POINT ( 'NONE',  ( 0.8726510978149698561, 7.843753604616166442, 0.4398688123008435147 ) ) ;
#22869=CARTESIAN_POINT ( 'NONE',  ( -23.08789804466238849, 149.8924475812327159, -0.6911741358207282859 ) ) ;
#22873=CARTESIAN_POINT ( 'NONE',  ( 2.765491355666962914, 117.1119770199604631, 0.6595734277189526651 ) ) ;
#22876=CARTESIAN_POINT ( 'NONE',  ( 9.605778978211040098, 157.4977751962898083, 1.777432263976032711 ) ) ;
#22877=CARTESIAN_POINT ( 'NONE',  ( 19.99643065938083453, 145.3736917597469471, -1.717600817134501634 ) ) ;
#22878=CARTESIAN_POINT ( 'NONE',  ( 0.9680108232324700079, 2.729151709021603978, 0.1071397942825247085 ) ) ;
#22879=CARTESIAN_POINT ( 'NONE',  ( -3.310625167495538257, 6.824969433126684137, -7.744297517547710896 ) ) ;
#22880=CARTESIAN_POINT ( 'NONE',  ( -2.895878334088895834, 159.0164033662945258, -1.329837440140976046 ) ) ;
#22881=CARTESIAN_POINT ( 'NONE',  ( 4.894174812879662717, 117.7423131706384112, -0.7196635720700498284 ) ) ;
#22882=CARTESIAN_POINT ( 'NONE',  ( 13.70496720263909829, 119.6480011847203002, 0.2738578607179662505 ) ) ;
#22883=CARTESIAN_POINT ( 'NONE',  ( 15.87656987697858746, 149.2064892436030163, -1.252469198948042539 ) ) ;
#22884=CARTESIAN_POINT ( 'NONE',  ( -8.961118498053046721, 123.9105667600146177, -0.1452814789513759974 ) ) ;
#22886=CARTESIAN_POINT ( 'NONE',  ( -5.693059210196507181, 156.8407539676644546, -1.898889529600695569 ) ) ;
#22887=CARTESIAN_POINT ( 'NONE',  ( 3.555926573287145231, -15.62149673449747489, 5.135790484437000814 ) ) ;
#22893=CARTESIAN_POINT ( 'NONE',  ( -0.01081828683971087710, 119.3136608367422866, 0.5413913113077197803 ) ) ;
#22894=DIRECTION ( 'NONE',  ( -4.017660918040594346E-17, 1.000000000000000000, 2.376309959284834438E-19 ) ) ;
#22895=CARTESIAN_POINT ( 'NONE',  ( -3.467804978690799622, 119.7720183225874138, 0.4097519885510785276 ) ) ;
#22896=CARTESIAN_POINT ( 'NONE',  ( -7.980626778564171353, 22.53057930515566554, 2.691543149341120156 ) ) ;
#22897=CARTESIAN_POINT ( 'NONE',  ( 7.664053125822814394, 122.2986020547093915, 0.5896768268545022895 ) ) ;
#22898=CARTESIAN_POINT ( 'NONE',  ( 8.125192968412290995, 117.9016134627522945, -0.4934282302770852113 ) ) ;
#22899=EDGE_CURVE ( 'NONE', #11900, #20726, #13781, .T. ) ;
#22904=CARTESIAN_POINT ( 'NONE',  ( -0.8920107295036362460, 116.4394364983335493, 0.02072182073814212572 ) ) ;
#22906=CARTESIAN_POINT ( 'NONE',  ( -6.706889091645539480, 120.9727344454672107, -1.004351640261528900 ) ) ;
#22907=CARTESIAN_POINT ( 'NONE',  ( 3.232439242213211994, -15.36757322000031145, 5.574794819488745112 ) ) ;
#22909=CARTESIAN_POINT ( 'NONE',  ( -9.364230102553138479, 123.8909350679826815, -0.6996930829695081622 ) ) ;
#22910=CARTESIAN_POINT ( 'NONE',  ( 3.231995002093183800, -14.34039573884512997, 4.866605245980782257 ) ) ;
#22912=CARTESIAN_POINT ( 'NONE',  ( 0.8860745468265911473, 116.4323782974132513, 0.03055428320029210734 ) ) ;
#22915=CARTESIAN_POINT ( 'NONE',  ( -4.399545650080316506, 2.442302885307133131, -1.471791394725967095 ) ) ;
#22916=CARTESIAN_POINT ( 'NONE',  ( -1.491112615444313949, 105.1235505628452387, 5.131223246399314597 ) ) ;
#22920=CARTESIAN_POINT ( 'NONE',  ( -6.978456853209969779, 121.0120372305622567, 0.7589161456756378099 ) ) ;
#22921=CARTESIAN_POINT ( 'NONE',  ( -3.586339569854333220, 7.474549112184489807, -2.913498476264247294 ) ) ;
#22922=CARTESIAN_POINT ( 'NONE',  ( 17.57666534335605490, 125.1652531886817172, 1.391946913312248180 ) ) ;
#22925=CARTESIAN_POINT ( 'NONE',  ( 11.94841889513447697, 120.7721054874162974, -1.107169436317064770 ) ) ;
#22926=CARTESIAN_POINT ( 'NONE',  ( -3.128764270554720728, 7.249652477310866594, -3.416742352092642321 ) ) ;
#22927=CARTESIAN_POINT ( 'NONE',  ( -22.50793294095888797, 142.2972183020237367, -1.640122747091713906 ) ) ;
#22929=EDGE_CURVE ( 'NONE', #26282, #40423, #19704, .T. ) ;
#22930=CARTESIAN_POINT ( 'NONE',  ( -13.67682410656413516, 150.2105054413494543, 0.1652630162413761539 ) ) ;
#22931=CARTESIAN_POINT ( 'NONE',  ( 6.168037961413951997, -13.40247527924742776, 1.492370457280242091 ) ) ;
#22933=CIRCLE ( 'NONE', #16841, 3.175000000000001155 ) ;
#22934=CARTESIAN_POINT ( 'NONE',  ( -2.753942980615568192, 107.6238140763581441, -4.560544256597707680 ) ) ;
#22937=CARTESIAN_POINT ( 'NONE',  ( 8.537619249161298995, 156.7723266660784986, 2.072230564756332161 ) ) ;
#22939=CARTESIAN_POINT ( 'NONE',  ( -6.503981220335420706E-14, 66.64146620154573952, -9.408573323119121831E-18 ) ) ;
#22940=CARTESIAN_POINT ( 'NONE',  ( -12.94589274040331439, 156.9034992427187376, 0.7570359663163894748 ) ) ;
#22942=CARTESIAN_POINT ( 'NONE',  ( 11.57591774076040103, 118.7825156662901378, -0.1473217720007391485 ) ) ;
#22947=CARTESIAN_POINT ( 'NONE',  ( -4.973570852245686957, 117.3993868453976575, -0.9750598967993134858 ) ) ;
#22951=CARTESIAN_POINT ( 'NONE',  ( -4.547585464732198268, 118.0892030396713039, 0.5918700655309280245 ) ) ;
#22955=CARTESIAN_POINT ( 'NONE',  ( -2.168366069047774403, 118.7629491485468236, -1.225207463359169857 ) ) ;
#22956=CARTESIAN_POINT ( 'NONE',  ( -8.375474303938146292, 119.6239881352457388, -1.418291987643603091 ) ) ;
#22957=CARTESIAN_POINT ( 'NONE',  ( -6.891280466594768228, 121.8252198949890186, -0.2939903263561802760 ) ) ;
#22958=CARTESIAN_POINT ( 'NONE',  ( 4.536752517374653237, 118.0323550597005209, 0.8638088581934265653 ) ) ;
#22960=CARTESIAN_POINT ( 'NONE',  ( -7.153290765950069741, 121.6016026263613838, -0.8513816870021353456 ) ) ;
#22961=CARTESIAN_POINT ( 'NONE',  ( -4.299427874650186610, 115.7036758056284356, -1.546095265231658855 ) ) ;
#22963=CARTESIAN_POINT ( 'NONE',  ( 5.267339127473229965, 116.4790307410953289, -0.8814195561379954968 ) ) ;
#22964=CARTESIAN_POINT ( 'NONE',  ( -16.67506696845916991, 147.9788754379930822, -1.914365833524547256 ) ) ;
#22966=CARTESIAN_POINT ( 'NONE',  ( -0.03245814172817860360, 158.1186941186938952, 1.624338139048501661 ) ) ;
#22967=CARTESIAN_POINT ( 'NONE',  ( 7.819596425025786779, 122.5025573198914230, -0.1851469994925282470 ) ) ;
#22968=CARTESIAN_POINT ( 'NONE',  ( -15.77235285888377270, 146.5682724429268262, -0.2480670253506113976 ) ) ;
#22969=CARTESIAN_POINT ( 'NONE',  ( 4.574821423538755205, -2.080616851812391310, 0.6590154617212384824 ) ) ;
#22970=CARTESIAN_POINT ( 'NONE',  ( 22.23561040172127434, 150.7043692363948537, 1.289434558007280129 ) ) ;
#22971=ORIENTED_EDGE ( 'NONE', *, *, #8699, .F. ) ;
#22973=CARTESIAN_POINT ( 'NONE',  ( 3.116032494879745762, -15.28226460877120374, 3.911124699519683556 ) ) ;
#22974=CARTESIAN_POINT ( 'NONE',  ( -11.94919878421465675, 122.6721150436042223, 1.294096368778067996 ) ) ;
#22975=CARTESIAN_POINT ( 'NONE',  ( -0.7398639285967090196, 8.776656789086558774, 0.6336005302938405581 ) ) ;
#22976=CARTESIAN_POINT ( 'NONE',  ( -3.233108093638920266, 159.4494809562368971, -0.4325382840285660890 ) ) ;
#22978=CARTESIAN_POINT ( 'NONE',  ( -0.06867543354984582959, -8.127513596672324425, -0.9731866935420671050 ) ) ;
#22983=CARTESIAN_POINT ( 'NONE',  ( 4.850755190080882073, 117.2937442104795593, 0.9187341308512859683 ) ) ;
#22985=CARTESIAN_POINT ( 'NONE',  ( -9.599121003648976469, 153.9312916436033447, 0.7969471826422134253 ) ) ;
#22986=CARTESIAN_POINT ( 'NONE',  ( 3.649535173467634674, -14.21384370944696407, 4.751373335446510637 ) ) ;
#22987=CARTESIAN_POINT ( 'NONE',  ( 17.34190353359454306, 148.5513402141484391, -1.530992562556359182 ) ) ;
#22988=CARTESIAN_POINT ( 'NONE',  ( -12.85210230480898375, 122.5866728308148055, -1.831397601346916426 ) ) ;
#22990=CARTESIAN_POINT ( 'NONE',  ( 3.093198985275321444, -14.55695847870221193, 3.716444964235936066 ) ) ;
#22991=CARTESIAN_POINT ( 'NONE',  ( -1.114473875789820934, 36.31367722304656809, -0.2353634988756889146 ) ) ;
#22992=CARTESIAN_POINT ( 'NONE',  ( 1.582738162022832018, 156.2580631240469415, -0.1078144505905371531 ) ) ;
#22995=CARTESIAN_POINT ( 'NONE',  ( 0.9967641087948266865, 106.0888231320409716, 5.244678224992261661 ) ) ;
#22998=CARTESIAN_POINT ( 'NONE',  ( 5.750520748247040181, 159.1178304044242964, 0.06386070104996836860 ) ) ;
#23001=CARTESIAN_POINT ( 'NONE',  ( -3.110646482806300739, 107.8085536575111689, 4.359277737140974551 ) ) ;
#23002=ADVANCED_FACE ( 'NONE', ( #23769 ), #36024, .T. ) ;
#23003=CARTESIAN_POINT ( 'NONE',  ( -4.459494944917585357, 115.6909491485452719, 1.361414471398195714 ) ) ;
#23005=CARTESIAN_POINT ( 'NONE',  ( -4.457266160556883960, 31.52268539727636565, -0.7032076836091958327 ) ) ;
#23006=CARTESIAN_POINT ( 'NONE',  ( 19.77411333694939088, 150.7280352275851101, 2.313572189391364109 ) ) ;
#23007=CARTESIAN_POINT ( 'NONE',  ( -4.137704358559117779, 17.39492794009094823, -2.099109474953318788 ) ) ;
#23008=CARTESIAN_POINT ( 'NONE',  ( -5.217102898550305845, -11.97038331068927342, -6.647077075081065267 ) ) ;
#23009=CARTESIAN_POINT ( 'NONE',  ( -8.722122541997446632, 117.9971651243157424, -0.7652714498589991976 ) ) ;
#23010=CARTESIAN_POINT ( 'NONE',  ( -0.3783624953764856969, 110.0486234891351245, -3.695659563127995373 ) ) ;
#23012=CARTESIAN_POINT ( 'NONE',  ( -1.146254217351140303, 106.2775121091388115, -5.162372565581046402 ) ) ;
#23013=CARTESIAN_POINT ( 'NONE',  ( 2.498149781570049299, 104.6144662015456959, 4.129972621594562909 ) ) ;
#23014=CARTESIAN_POINT ( 'NONE',  ( 4.203610184846851894, 17.99761390031315500, -1.968029828111186319 ) ) ;
#23015=FACE_BOUND ( 'NONE', #1866, .T. ) ;
#23016=CARTESIAN_POINT ( 'NONE',  ( -3.967884321586665042, 117.3993838589258019, -1.334270751278506362 ) ) ;
#23017=CARTESIAN_POINT ( 'NONE',  ( 3.093198985275321444, -14.55695847870221193, 3.716444964235936066 ) ) ;
#23018=CARTESIAN_POINT ( 'NONE',  ( 2.352838477949680929, 119.2037781873646622, -0.5921520780602625988 ) ) ;
#23019=CARTESIAN_POINT ( 'NONE',  ( -5.842267051812750189, 117.1711376449269721, 0.3073735213368162800 ) ) ;
#23023=ORIENTED_EDGE ( 'NONE', *, *, #9514, .F. ) ;
#23025=CARTESIAN_POINT ( 'NONE',  ( 5.309364964326869440, -15.28511724905957969, 2.738662543889408774 ) ) ;
#23026=CARTESIAN_POINT ( 'NONE',  ( -20.10795522872020058, 148.3334041379468715, 1.700709099906817956 ) ) ;
#23027=CARTESIAN_POINT ( 'NONE',  ( 20.59913821282560420, 136.3738900553462372, -1.239205967624167570 ) ) ;
#23028=CARTESIAN_POINT ( 'NONE',  ( -0.1020318426323372635, 30.30579279289823802, -0.9687052925327788166 ) ) ;
#23032=CARTESIAN_POINT ( 'NONE',  ( 1.051265659380868689, 124.5996987749017109, 0.05046802306060386295 ) ) ;
#23033=FILL_AREA_STYLE ('',( #35643 ) ) ;
#23034=CARTESIAN_POINT ( 'NONE',  ( -11.73912714424001180, 153.3684197651487580, 1.370860710263250182 ) ) ;
#23036=CARTESIAN_POINT ( 'NONE',  ( 0.01081828683957167594, 119.3136608367422866, -0.5413913113077197803 ) ) ;
#23038=CARTESIAN_POINT ( 'NONE',  ( -1.153229101629017261, 158.8088198215516229, -1.472604719115122807 ) ) ;
#23040=VERTEX_POINT ( 'NONE', #8023 ) ;
#23041=CARTESIAN_POINT ( 'NONE',  ( 4.603039994573143723, 118.0757665291171037, -0.5234378334457231441 ) ) ;
#23042=CARTESIAN_POINT ( 'NONE',  ( 9.648208730819460399, 124.2480737032941533, -0.3321887029122944091 ) ) ;
#23043=ORIENTED_EDGE ( 'NONE', *, *, #19791, .F. ) ;
#23044=CARTESIAN_POINT ( 'NONE',  ( -17.54535662205675450, 147.9903219242534078, -2.232389162988360543 ) ) ;
#23045=CARTESIAN_POINT ( 'NONE',  ( 3.315889604118840150, -14.76599673617913488, 0.9486971755708663023 ) ) ;
#23046=CARTESIAN_POINT ( 'NONE',  ( -22.46755768833301303, 150.8526571111528654, -0.4489552724284875951 ) ) ;
#23048=CARTESIAN_POINT ( 'NONE',  ( 2.776928087254650013, 2.301956178644051221, 3.707541451904531105 ) ) ;
#23049=CARTESIAN_POINT ( 'NONE',  ( 0.8144440842625040311, 156.8926940187749324, 1.343054762528750112 ) ) ;
#23050=CARTESIAN_POINT ( 'NONE',  ( -3.046231754824817006, 31.09810386281187533, 0.4001267285823237874 ) ) ;
#23052=CARTESIAN_POINT ( 'NONE',  ( -4.507778648822867495, 31.37953541088120346, -1.025544427737863362 ) ) ;
#23053=CARTESIAN_POINT ( 'NONE',  ( 11.85612367793081745, 151.9842433124228762, 0.4520816642129338314 ) ) ;
#23060=DIRECTION ( 'NONE',  ( 0.9998004120163608288, 0.000000000000000000, 0.01997839162482749342 ) ) ;
#23062=CARTESIAN_POINT ( 'NONE',  ( -8.564670675228182262, 118.7243493509376435, -1.182334654099753468 ) ) ;
#23068=CARTESIAN_POINT ( 'NONE',  ( -22.63314285866090003, 150.6357905964555925, -0.1239933314926728036 ) ) ;
#23069=ORIENTED_EDGE ( 'NONE', *, *, #28031, .F. ) ;
#23071=CARTESIAN_POINT ( 'NONE',  ( 6.984995591253446712, 121.9529933140264575, 0.08165562821682262329 ) ) ;
#23072=ORIENTED_EDGE ( 'NONE', *, *, #14420, .T. ) ;
#23074=CARTESIAN_POINT ( 'NONE',  ( -9.566940353391325758, 124.8108731098830049, -0.2265937611309800925 ) ) ;
#23075=CARTESIAN_POINT ( 'NONE',  ( 4.196136289373067818, -14.93657984310306475, 5.004071965215434403 ) ) ;
#23076=CARTESIAN_POINT ( 'NONE',  ( -0.4229338353208662582, 117.8786474493541050, 0.5307671053780920190 ) ) ;
#23077=DIRECTION ( 'NONE',  ( 0.9998004120163608288, 0.000000000000000000, 0.01997839162482749342 ) ) ;
#23078=CARTESIAN_POINT ( 'NONE',  ( 0.3088162040006633968, 116.5752054743899038, 0.1648661904198057415 ) ) ;
#23079=CARTESIAN_POINT ( 'NONE',  ( 2.031162158012311370, -15.69476345269874074, 5.605913305253631407 ) ) ;
#23080=CARTESIAN_POINT ( 'NONE',  ( 4.765335592615821625, 118.5266822147775940, -0.8412684598427435656 ) ) ;
#23081=CARTESIAN_POINT ( 'NONE',  ( 0.9522911014763013604, -10.27702741150894994, -0.2247348558088197723 ) ) ;
#23082=CARTESIAN_POINT ( 'NONE',  ( -8.209937203459384492, 117.5146787832509858, -0.2970838962712566977 ) ) ;
#23086=CARTESIAN_POINT ( 'NONE',  ( 5.544339057385890612, 116.8028365428300361, 0.4221121198209883962 ) ) ;
#23088=CARTESIAN_POINT ( 'NONE',  ( -4.293775319276113223, 119.8084884740358547, 0.7325880323699283103 ) ) ;
#23090=CARTESIAN_POINT ( 'NONE',  ( 10.54454712121190951, 119.9085704333771787, 1.450830856784146139 ) ) ;
#23091=CARTESIAN_POINT ( 'NONE',  ( 8.713776656587251424, 120.2102557752085232, -1.142027078586575595 ) ) ;
#23092=CARTESIAN_POINT ( 'NONE',  ( -0.9360807938713975318, 7.254031735439380846, -0.2770855581244007215 ) ) ;
#23093=CARTESIAN_POINT ( 'NONE',  ( -21.88420111187377870, 149.4141677464492091, -2.022441453707984227 ) ) ;
#23094=CARTESIAN_POINT ( 'NONE',  ( 4.591938001951629822, 118.0392868320003714, -0.6629688387655557902 ) ) ;
#23095=CARTESIAN_POINT ( 'NONE',  ( 10.08214312826198267, 118.0934564804968971, 0.2014652138697922978 ) ) ;
#23097=CARTESIAN_POINT ( 'NONE',  ( 10.43918028506318940, 123.9810924921358151, -0.8290978625009025604 ) ) ;
#23098=CARTESIAN_POINT ( 'NONE',  ( -6.503408402854686798, 121.7799126398724354, -0.1299535771408516782 ) ) ;
#23099=ORIENTED_EDGE ( 'NONE', *, *, #27602, .T. ) ;
#23100=CARTESIAN_POINT ( 'NONE',  ( 0.01081828683958208255, 119.3136608367422866, -0.5413913113077195582 ) ) ;
#23102=CARTESIAN_POINT ( 'NONE',  ( 4.081004676854354862, -15.57459693632588760, 4.681182614216856663 ) ) ;
#23105=CARTESIAN_POINT ( 'NONE',  ( 11.70444740893354485, 123.2143981803894093, 1.719255905491489766 ) ) ;
#23106=CARTESIAN_POINT ( 'NONE',  ( -1.114473875789821378, 36.31367722304657519, -0.2353634988756885538 ) ) ;
#23108=CARTESIAN_POINT ( 'NONE',  ( -4.933025141172056927, 117.5302216577071874, 0.6666291745611304664 ) ) ;
#23109=CARTESIAN_POINT ( 'NONE',  ( 6.556273983038449771, -14.34328088419217728, -5.323198733142235461 ) ) ;
#23110=CARTESIAN_POINT ( 'NONE',  ( 9.476112355320449154, 124.1929984354129175, 0.6154534730440990309 ) ) ;
#23111=CARTESIAN_POINT ( 'NONE',  ( 13.06303874853649738, 119.8917521002241955, -0.5243808535303263740 ) ) ;
#23114=CARTESIAN_POINT ( 'NONE',  ( -6.439805278602227377E-14, 159.6054662015457382, 1.008550168686281963E-16 ) ) ;
#23116=CARTESIAN_POINT ( 'NONE',  ( 6.621162754568407749, 120.6004594848523226, -0.8446542950495584678 ) ) ;
#23117=CARTESIAN_POINT ( 'NONE',  ( 23.11127252101355722, 149.9001116002701224, 0.4618182267416076070 ) ) ;
#23118=CARTESIAN_POINT ( 'NONE',  ( -13.65930421665844641, 150.2105054413494543, -0.7115039165091185946 ) ) ;
#23119=CARTESIAN_POINT ( 'NONE',  ( 3.097180478269691672, -14.43375334869456594, 4.992610980676636778 ) ) ;
#23120=CARTESIAN_POINT ( 'NONE',  ( -0.008308726997795933336, 117.3658353995175503, 0.4158026747930030909 ) ) ;
#23122=CARTESIAN_POINT ( 'NONE',  ( 2.743358099589752630, 116.5337465564440578, 0.09497135926289701491 ) ) ;
#23123=ORIENTED_EDGE ( 'NONE', *, *, #4825, .T. ) ;
#23124=CARTESIAN_POINT ( 'NONE',  ( 1.398650104629075797, 0.06838872207683838189, -4.420329592304430122 ) ) ;
#23125=CARTESIAN_POINT ( 'NONE',  ( -0.1569751959820993303, 105.1223796759901177, 5.342321742714839949 ) ) ;
#23128=CARTESIAN_POINT ( 'NONE',  ( -7.815079368384979297, 122.5103633090772064, 0.1576210380653273735 ) ) ;
#23129=CARTESIAN_POINT ( 'NONE',  ( -4.468841950160419962, 8.124252568732815760, -1.173904233648782158 ) ) ;
#23130=CARTESIAN_POINT ( 'NONE',  ( 1.281755300609836334, 159.3505072347868747, 0.9987438389826047702 ) ) ;
#23132=CARTESIAN_POINT ( 'NONE',  ( 21.15257933310676108, 148.4376209648218321, -1.514591261405503708 ) ) ;
#23133=CARTESIAN_POINT ( 'NONE',  ( 3.912982837994093188, 14.17146771520798332, -2.459658384584827218 ) ) ;
#23134=CARTESIAN_POINT ( 'NONE',  ( -11.27775095430307140, 119.0414093155750379, -0.9684783378491814698 ) ) ;
#23135=AXIS2_PLACEMENT_3D ( 'NONE', #13890, #4117, #16654 ) ;
#23137=CARTESIAN_POINT ( 'NONE',  ( -8.770618086121094947, 123.6813396614493712, -0.1752578222716850986 ) ) ;
#23138=CARTESIAN_POINT ( 'NONE',  ( -15.82110658236432776, 145.7390459690742830, 0.1389873312028087615 ) ) ;
#23139=CARTESIAN_POINT ( 'NONE',  ( 2.112423120037338453, -15.42067558999450583, 5.959086572354191702 ) ) ;
#23142=CARTESIAN_POINT ( 'NONE',  ( 2.906309357581933650, -13.72804873580029472, 0.7610837935892840189 ) ) ;
#23143=VERTEX_POINT ( 'NONE', #5891 ) ;
#23144=CARTESIAN_POINT ( 'NONE',  ( 2.460791562519470066, 158.0185616612000956, 1.723846131599015230 ) ) ;
#23146=CARTESIAN_POINT ( 'NONE',  ( 14.16569067496491563, 138.8670163227227476, 0.2830642121559620583 ) ) ;
#23147=CARTESIAN_POINT ( 'NONE',  ( -22.10675755583041635, 150.4421090420883900, 0.7299123522449004753 ) ) ;
#23148=CARTESIAN_POINT ( 'NONE',  ( -8.392384909494198908, 27.87760190725155951, 0.4359655409547527616 ) ) ;
#23150=CARTESIAN_POINT ( 'NONE',  ( 22.71658102202232854, 150.3666470947781022, -0.1371106802449218731 ) ) ;
#23156=CARTESIAN_POINT ( 'NONE',  ( -4.962974768447578455, 117.4026934023842585, -1.029810944977519460 ) ) ;
#23158=CARTESIAN_POINT ( 'NONE',  ( -5.586884702347496123, 85.69146620154573668, -0.1116392523995361624 ) ) ;
#23159=CARTESIAN_POINT ( 'NONE',  ( -4.558231547695950958, 118.1058047250539005, 0.4915253113856153377 ) ) ;
#23164=CARTESIAN_POINT ( 'NONE',  ( -3.727707540449571866, 118.8936418977788634, -0.9337890276463987060 ) ) ;
#23165=CARTESIAN_POINT ( 'NONE',  ( -5.211883163658477258, 116.1034411669277375, -1.237845179234434045 ) ) ;
#23167=CARTESIAN_POINT ( 'NONE',  ( 4.521618879414620373, 118.0718733995298066, 0.8081141274518772732 ) ) ;
#23168=CARTESIAN_POINT ( 'NONE',  ( -5.192366003377138384, 121.0352659167314755, -0.5503205103620255612 ) ) ;
#23169=CARTESIAN_POINT ( 'NONE',  ( -1.791851930664796644, 115.7029402959327911, -1.723146288102838986 ) ) ;
#23171=CARTESIAN_POINT ( 'NONE',  ( 5.498174961348566647, 117.5088849381099436, -0.6086507346144034436 ) ) ;
#23172=CARTESIAN_POINT ( 'NONE',  ( -14.96631152213295479, 150.5987129668814077, -1.974168424754894957 ) ) ;
#23173=CARTESIAN_POINT ( 'NONE',  ( 4.304052292061569140, 104.6144662015457385, -3.992357259174772466 ) ) ;
#23174=CARTESIAN_POINT ( 'NONE',  ( -0.03066982525788228969, 157.3074135339440147, 1.534843470138540722 ) ) ;
#23176=CARTESIAN_POINT ( 'NONE',  ( -7.540585633152407041, 122.4256904137044302, -0.07081817902877589332 ) ) ;
#23177=CARTESIAN_POINT ( 'NONE',  ( 4.586363120317823672, -1.655842793181455663, -0.6244342276643227718 ) ) ;
#23178=CARTESIAN_POINT ( 'NONE',  ( 20.97948398557565497, 132.3427885975763161, 1.200284224572990777 ) ) ;
#23180=CARTESIAN_POINT ( 'NONE',  ( 3.071204355543858178, -15.18643405355604692, 3.901769932616943493 ) ) ;
#23181=CARTESIAN_POINT ( 'NONE',  ( -19.00012635448491594, 147.0452383304005082, 1.727400128179960026 ) ) ;
#23182=CARTESIAN_POINT ( 'NONE',  ( -0.1482875670852983607, 5.528424516503947395, -0.9633795868741713564 ) ) ;
#23183=CARTESIAN_POINT ( 'NONE',  ( -15.83212890848034426, 121.4040080620525117, -0.8411940925737089181 ) ) ;
#23184=CARTESIAN_POINT ( 'NONE',  ( -0.9630862182390291792, 27.11985920190685917, 0.1463314843619143713 ) ) ;
#23188=CARTESIAN_POINT ( 'NONE',  ( 5.246142718657039516, 116.7267603939287426, 1.018146482794727747 ) ) ;
#23190=CARTESIAN_POINT ( 'NONE',  ( -15.92216882203272377, 147.6644253265642135, 0.6463398217596320050 ) ) ;
#23191=CARTESIAN_POINT ( 'NONE',  ( 4.301541689408341362, -12.13840576482722078, 1.420409876116004222 ) ) ;
#23192=CARTESIAN_POINT ( 'NONE',  ( 10.76607124212182498, 123.2317624570580534, -1.067040512904773752 ) ) ;
#23193=CARTESIAN_POINT ( 'NONE',  ( -11.06681148537632353, 121.4866960210745503, -1.697623966824489461 ) ) ;
#23194=CARTESIAN_POINT ( 'NONE',  ( -4.429613830441260447, 104.6144662015457527, 1.943785857760518043 ) ) ;
#23196=CARTESIAN_POINT ( 'NONE',  ( 3.211984996733021624, -14.06435921420946755, 2.432701253525752172 ) ) ;
#23197=CARTESIAN_POINT ( 'NONE',  ( -6.125448292536311179, 31.19746429541880772, 1.780260802209707949 ) ) ;
#23198=CARTESIAN_POINT ( 'NONE',  ( 4.580760836099185163, 121.1907927009877000, 0.02326454623414945036 ) ) ;
#23200=CARTESIAN_POINT ( 'NONE',  ( -5.232920286240068108, 115.9100003722636956, 1.117763783589812432 ) ) ;
#23201=CARTESIAN_POINT ( 'NONE',  ( -0.1065207248106947446, 105.8844037013955983, 5.332933549509751181 ) ) ;
#23204=EDGE_CURVE ( 'NONE', #31017, #2334, #37164, .T. ) ;
#23206=CARTESIAN_POINT ( 'NONE',  ( 0.001838942458788770306, 116.4858755864912183, -0.09202820039585830891 ) ) ;
#23207=CARTESIAN_POINT ( 'NONE',  ( -5.103137870717271873, 114.3519703858145959, 1.758966173294684854 ) ) ;
#23210=DIRECTION ( 'NONE',  ( -0.9998004120163609398, 0.000000000000000000, -0.01997839162482749689 ) ) ;
#23211=CARTESIAN_POINT ( 'NONE',  ( -1.543289776211116626, 35.18841652350401006, 0.2515601095814950505 ) ) ;
#23213=CARTESIAN_POINT ( 'NONE',  ( 13.54337464129331714, 122.2126086331852974, 1.756000464972328867 ) ) ;
#23214=CARTESIAN_POINT ( 'NONE',  ( -1.512449008193210931, 25.81601926892489018, -4.382106060783010903 ) ) ;
#23215=CARTESIAN_POINT ( 'NONE',  ( -8.302162399154521921, -10.86525386290528594, -1.555404731216454284 ) ) ;
#23216=CARTESIAN_POINT ( 'NONE',  ( -5.532489265500688980, 117.9651905194339605, -1.089543468331991116 ) ) ;
#23217=CARTESIAN_POINT ( 'NONE',  ( -3.074626428557295732, 123.1875568577169560, -0.1788317054798707617 ) ) ;
#23221=CARTESIAN_POINT ( 'NONE',  ( -1.607155361308500563, 104.6144662015456959, 4.551785039662791021 ) ) ;
#23222=AXIS2_PLACEMENT_3D ( 'NONE', #36310, #16900, #29902 ) ;
#23223=CARTESIAN_POINT ( 'NONE',  ( 1.325333094648095011, 19.28447512809159292, -4.440015753949128730 ) ) ;
#23226=CARTESIAN_POINT ( 'NONE',  ( 3.226040172055379518, -13.73821525131127608, 2.149215086980220235 ) ) ;
#23227=CARTESIAN_POINT ( 'NONE',  ( 2.102284131448346027, 122.9394440205640961, -0.1126375150955781085 ) ) ;
#23228=CARTESIAN_POINT ( 'NONE',  ( -14.24059674577823387, 120.4756499382577886, 0.4587616384891654575 ) ) ;
#23229=CARTESIAN_POINT ( 'NONE',  ( 4.922801907822831780, 117.4099815471397363, -0.9489923651248427516 ) ) ;
#23233=CARTESIAN_POINT ( 'NONE',  ( -5.204863647155245410, 115.7029491485453576, 1.024056704596592038 ) ) ;
#23234=CARTESIAN_POINT ( 'NONE',  ( 2.719191112037562252, -15.71471113085404170, 5.040136806425350002 ) ) ;
#23235=CARTESIAN_POINT ( 'NONE',  ( -20.39294766749442900, 148.4497675966422889, 1.664483663417329895 ) ) ;
#23236=CARTESIAN_POINT ( 'NONE',  ( 12.48318382086454115, 120.3283006479967128, -0.8937555771000558202 ) ) ;
#23237=CARTESIAN_POINT ( 'NONE',  ( -4.595132424582489605, -6.828429371805166959, -0.5093739664528403877 ) ) ;
#23240=EDGE_LOOP ( 'NONE', ( #17390, #24896, #25410, #33146 ) ) ;
#23242=CARTESIAN_POINT ( 'NONE',  ( 1.058386756517223137, 124.8229041592835387, 0.03077316225166111877 ) ) ;
#23243=CARTESIAN_POINT ( 'NONE',  ( -14.75676393591426816, 134.6798445586954927, 1.238239479614488214 ) ) ;
#23245=EDGE_CURVE ( 'NONE', #15805, #21511, #10182, .T. ) ;
#23246=CARTESIAN_POINT ( 'NONE',  ( 18.41704236485550439, 146.8095856830544790, -1.664602135862215393 ) ) ;
#23247=CARTESIAN_POINT ( 'NONE',  ( -20.91063213905309937, 147.8517002469272370, -2.402771019925620255 ) ) ;
#23251=CARTESIAN_POINT ( 'NONE',  ( 4.407527007107042039, 118.1629860519386881, -0.4885628053013030825 ) ) ;
#23252=CARTESIAN_POINT ( 'NONE',  ( 3.022581645176192211, 156.1079525116674631, -0.4343475099915217741 ) ) ;
#23254=CARTESIAN_POINT ( 'NONE',  ( -8.183297913989086680, 121.2453320564195280, -1.294587653635731916 ) ) ;
#23255=CARTESIAN_POINT ( 'NONE',  ( 1.980066450162843106, -15.31690195035381663, 5.269506609478212589 ) ) ;
#23256=CARTESIAN_POINT ( 'NONE',  ( 2.447805105500874934, 105.1245809240877662, -4.785117320943135688 ) ) ;
#23259=CARTESIAN_POINT ( 'NONE',  ( -2.065029617914060367, 6.824861272777455135, -4.134893973632223663 ) ) ;
#23260=CARTESIAN_POINT ( 'NONE',  ( 3.657622835216417290, 156.7231754051992425, 1.598616135119148352 ) ) ;
#23261=CARTESIAN_POINT ( 'NONE',  ( -0.3625295811786362621, 32.83794214056845107, 1.283952373590488305 ) ) ;
#23262=CARTESIAN_POINT ( 'NONE',  ( -2.359559261509405204, 14.11188314818778267, 3.974389579228013503 ) ) ;
#23263=CARTESIAN_POINT ( 'NONE',  ( 6.494557633019020670, 121.7745328324513139, 0.2023806202038008484 ) ) ;
#23268=CARTESIAN_POINT ( 'NONE',  ( -2.026290786761661522, 117.3993837374443672, 1.369916322765275529 ) ) ;
#23270=DIRECTION ( 'NONE',  ( -0.9998004120163610509, -4.016384292689131511E-17, -0.01997839162482749689 ) ) ;
#23273=CARTESIAN_POINT ( 'NONE',  ( -4.074955089416341991, 118.2429491485453354, 0.1454234154749719787 ) ) ;
#23277=CARTESIAN_POINT ( 'NONE',  ( -21.39485547647985086, 132.5159896776619917, -0.01683271311856767219 ) ) ;
#23279=ORIENTED_EDGE ( 'NONE', *, *, #13097, .T. ) ;
#23281=CARTESIAN_POINT ( 'NONE',  ( 7.796796354633476867, 122.5849000957118022, -0.007570717282985798234 ) ) ;
#23282=ORIENTED_EDGE ( 'NONE', *, *, #26151, .T. ) ;
#23283=CARTESIAN_POINT ( 'NONE',  ( 3.636484375549583259, 115.7029495056428487, -1.480734918736348105 ) ) ;
#23284=CARTESIAN_POINT ( 'NONE',  ( -13.59043555108506851, 150.2357272821285221, -0.3212980696657036783 ) ) ;
#23285=CARTESIAN_POINT ( 'NONE',  ( 5.669917404453804544, -14.04548127125972101, 2.990483579271598469 ) ) ;
#23286=CARTESIAN_POINT ( 'NONE',  ( -2.840063763404333308, 158.7847427699215928, 1.391859091975727658 ) ) ;
#23287=CARTESIAN_POINT ( 'NONE',  ( 4.203610184846851894, 17.99761390031315500, -1.968029828111186541 ) ) ;
#23289=CARTESIAN_POINT ( 'NONE',  ( 5.814470848032661898, 117.0573985505404693, 0.4185731406947919009 ) ) ;
#23290=CARTESIAN_POINT ( 'NONE',  ( 2.303556031286093653, -15.40459834138439810, 5.802045920756290442 ) ) ;
#23292=CARTESIAN_POINT ( 'NONE',  ( 0.9725752971277935588, -10.50039532299128808, -0.08436647605774086345 ) ) ;
#23293=CARTESIAN_POINT ( 'NONE',  ( -5.792301705315751725, 116.9567987913546006, -0.2385690759321333065 ) ) ;
#23296=ORIENTED_EDGE ( 'NONE', *, *, #9552, .F. ) ;
#23297=CARTESIAN_POINT ( 'NONE',  ( 8.731230164061564381, 117.9563494393051144, 0.7283447773125311109 ) ) ;
#23299=CARTESIAN_POINT ( 'NONE',  ( -12.33128838443264463, 153.5964916033214820, 1.587645809864455471 ) ) ;
#23301=CARTESIAN_POINT ( 'NONE',  ( 17.69400247866221321, 128.5843929717815115, 1.987683303373968702 ) ) ;
#23302=CARTESIAN_POINT ( 'NONE',  ( 12.91500497980660178, 122.5866728308148055, -1.316509475493082171 ) ) ;
#23303=CARTESIAN_POINT ( 'NONE',  ( 0.9007433063219677516, 2.300345052497278608, 0.3717552062572989091 ) ) ;
#23304=CARTESIAN_POINT ( 'NONE',  ( -21.61975215418298291, 149.3076860495818323, -2.139488579489918774 ) ) ;
#23305=CARTESIAN_POINT ( 'NONE',  ( 4.587194918930014964, 118.0383489642607913, -0.6670231109234234790 ) ) ;
#23310=CARTESIAN_POINT ( 'NONE',  ( 4.803469898345580802, 156.0326374431741385, -1.047298710704739122 ) ) ;
#23311=CARTESIAN_POINT ( 'NONE',  ( -2.888995153171277419, 156.0927491134738716, -0.02440385714215712737 ) ) ;
#23313=CARTESIAN_POINT ( 'NONE',  ( -18.63996327081357052, 147.1333978507680627, -2.447832456508666432 ) ) ;
#23314=CARTESIAN_POINT ( 'NONE',  ( 4.914263517198875775, -15.39432152949170352, 0.3857354017804055513 ) ) ;
#23315=CARTESIAN_POINT ( 'NONE',  ( -4.556757383386185190, 31.49269130883712720, -0.6906699653381264126 ) ) ;
#23316=CARTESIAN_POINT ( 'NONE',  ( -4.575423324728332020, 118.0775249002766003, -0.7112773029818583170 ) ) ;
#23319=CARTESIAN_POINT ( 'NONE',  ( 11.19992112824918706, 154.5781333488962446, 2.119767339128326267 ) ) ;
#23322=CARTESIAN_POINT ( 'NONE',  ( 23.11127252101355722, 149.9001116002701224, 0.4618182267416076070 ) ) ;
#23324=CARTESIAN_POINT ( 'NONE',  ( -1.660137282266059611, 14.53371390510571004, 8.268994913937449454 ) ) ;
#23325=CARTESIAN_POINT ( 'NONE',  ( 13.34275001191896415, 134.1388935151753401, 0.9731691531512426385 ) ) ;
#23326=CARTESIAN_POINT ( 'NONE',  ( 20.57308965805791701, 132.2049894596293313, -0.6677571715933801055 ) ) ;
#23327=DIRECTION ( 'NONE',  ( 0.9963166110440661027, 0.000000000000000000, -0.08575086330566526749 ) ) ;
#23329=CARTESIAN_POINT ( 'NONE',  ( 0.6575858438756917446, 118.7629491485454025, 1.273916485320598202 ) ) ;
#23330=CIRCLE ( 'NONE', #12499, 5.588000000000006295 ) ;
#23331=CARTESIAN_POINT ( 'NONE',  ( -5.755666581048902941, 159.1151184437813981, -0.09834937626042344894 ) ) ;
#23333=CARTESIAN_POINT ( 'NONE',  ( 6.848188653798881198, 121.3878566068075173, -0.5633949501833540596 ) ) ;
#23335=CARTESIAN_POINT ( 'NONE',  ( -15.79012389680301709, 146.9282941555416073, -0.7681517710631363682 ) ) ;
#23336=CARTESIAN_POINT ( 'NONE',  ( 4.218352450475082449, -13.04292013931325478, 2.887648331721151873 ) ) ;
#23337=CARTESIAN_POINT ( 'NONE',  ( -20.93040400792228795, 136.4823663107028722, 1.114867025985508464 ) ) ;
#23338=DIRECTION ( 'NONE',  ( -0.9998004120163609398, 0.000000000000000000, -0.01997839162482749689 ) ) ;
#23339=CARTESIAN_POINT ( 'NONE',  ( 1.417643301182374582, 159.6052071245950970, 0.07209812905978400799 ) ) ;
#23341=CARTESIAN_POINT ( 'NONE',  ( -1.861891798414337940, 1.167894131763866250, -4.247245584637167504 ) ) ;
#23342=CARTESIAN_POINT ( 'NONE',  ( -23.45208337669183152, 146.8499405026647651, -0.4686284387228153991 ) ) ;
#23344=CARTESIAN_POINT ( 'NONE',  ( -6.434551728065664555, 119.5454990110429065, 1.003392985923742931 ) ) ;
#23346=CARTESIAN_POINT ( 'NONE',  ( 1.583070580811935191, 1.852152477310867074, 4.353984577079609508 ) ) ;
#23347=CARTESIAN_POINT ( 'NONE',  ( 14.52885936862946004, 121.1548589120785095, 1.307706137645302302 ) ) ;
#23349=DIRECTION ( 'NONE',  ( 0.9998004120163609398, 4.016384292689130894E-17, 0.01997839162482749689 ) ) ;
#23350=CARTESIAN_POINT ( 'NONE',  ( 13.70042256495996824, 122.3361261571837986, -1.218568937077757042 ) ) ;
#23351=AXIS2_PLACEMENT_3D ( 'NONE', #8215, #5045, #1840 ) ;
#23352=CARTESIAN_POINT ( 'NONE',  ( -0.3558933743640902425, 1.202427940091101100, 4.626034787239965418 ) ) ;
#23353=CARTESIAN_POINT ( 'NONE',  ( -20.20545065706726717, 152.4988772720997190, -1.451042778694937363 ) ) ;
#23357=CARTESIAN_POINT ( 'NONE',  ( -15.85578974452678658, 145.9541952667573810, 0.1379097727432557485 ) ) ;
#23358=CARTESIAN_POINT ( 'NONE',  ( 2.083301838685661878, -15.46665383083971257, 5.961979448439955753 ) ) ;
#23361=CARTESIAN_POINT ( 'NONE',  ( -1.903537964721656151, 106.6614287958324354, -4.980401174282360621 ) ) ;
#23363=CARTESIAN_POINT ( 'NONE',  ( 13.39306239354261407, 123.7870877700634509, 1.917211633051635333 ) ) ;
#23366=DIRECTION ( 'NONE',  ( 0.9998004120163608288, 0.000000000000000000, 0.01997839162482760791 ) ) ;
#23367=CARTESIAN_POINT ( 'NONE',  ( -14.96085986107159016, 121.2513550155162960, 0.6271060280491598249 ) ) ;
#23368=CARTESIAN_POINT ( 'NONE',  ( -4.534963259934312596, 26.26729952004485824, -7.114490783490484027 ) ) ;
#23369=CARTESIAN_POINT ( 'NONE',  ( 5.855671506236596713, 121.0368588677253143, 0.7388637662663295469 ) ) ;
#23370=CARTESIAN_POINT ( 'NONE',  ( 4.803851041827788215, 116.9482543694763166, -0.2466672064845015777 ) ) ;
#23374=CARTESIAN_POINT ( 'NONE',  ( 2.104948366110713565, 106.4601199789983212, -4.917459751093059772 ) ) ;
#23377=CARTESIAN_POINT ( 'NONE',  ( -4.432033464645024345, 118.1653844686336186, 0.4638121791032019381 ) ) ;
#23380=CARTESIAN_POINT ( 'NONE',  ( -4.722993557843548018, 118.7629491485454309, -0.9938571727007795564 ) ) ;
#23381=CARTESIAN_POINT ( 'NONE',  ( 6.146672433393463031, 119.5348080636299954, -1.011818472031234206 ) ) ;
#23382=CARTESIAN_POINT ( 'NONE',  ( -5.262805716460127847, 116.4520502601644409, -1.094458988799881682 ) ) ;
#23383=CARTESIAN_POINT ( 'NONE',  ( 4.596454834243283827, 118.0615255785435949, 0.7279963062917687022 ) ) ;
#23384=CARTESIAN_POINT ( 'NONE',  ( -11.86571527151352612, 128.3619849303985632, -1.073981288313974991 ) ) ;
#23385=TOROIDAL_SURFACE ( 'NONE', #21348, 3.683000000000000718, 0.5080000000000000071 ) ;
#23386=CARTESIAN_POINT ( 'NONE',  ( -0.9706191444543458280, 115.7029418442419484, -1.748960127381335994 ) ) ;
#23387=CARTESIAN_POINT ( 'NONE',  ( 2.557047726870576465, 118.1651003891136185, -0.7232189756707855244 ) ) ;
#23388=CARTESIAN_POINT ( 'NONE',  ( 4.861212978143112373, 112.7561542417671916, -2.378900599183503051 ) ) ;
#23389=CARTESIAN_POINT ( 'NONE',  ( -7.227551859934705725, 121.2980461901665308, -1.025750885112893585 ) ) ;
#23390=CARTESIAN_POINT ( 'NONE',  ( -5.336395407662996249, 116.0444662015457169, 0.06658830643601890142 ) ) ;
#23391=CARTESIAN_POINT ( 'NONE',  ( -0.03153870137021549253, 158.4432089348667319, 1.578325583784928376 ) ) ;
#23392=CARTESIAN_POINT ( 'NONE',  ( 8.207314164617031338, 120.6877426416259738, -1.076149196205714587 ) ) ;
#23393=CARTESIAN_POINT ( 'NONE',  ( -15.77438986758538242, 146.5666090065403466, -0.1139034878652071398 ) ) ;
#23394=CARTESIAN_POINT ( 'NONE',  ( 4.634220987317881679, -1.855718946426311078, -0.01876340930339078644 ) ) ;
#23395=CARTESIAN_POINT ( 'NONE',  ( 5.539025187978692699, 159.0643023895801491, 0.7880117631591502247 ) ) ;
#23397=CARTESIAN_POINT ( 'NONE',  ( 2.352443540978347958, -15.20488079220741540, 4.935102241435597392 ) ) ;
#23399=CARTESIAN_POINT ( 'NONE',  ( -3.316780243214269230, 119.1333808041459577, 0.7607270569537705196 ) ) ;
#23400=CARTESIAN_POINT ( 'NONE',  ( 0.6087277426107279288, -8.065848283227245119, 0.7602462886992925606 ) ) ;
#23401=CARTESIAN_POINT ( 'NONE',  ( -21.25299977426499609, 132.4531229209162575, -0.9669248719381910995 ) ) ;
#23402=CARTESIAN_POINT ( 'NONE',  ( -0.7739057699295280868, 27.87760190725158083, 0.5882008851359883383 ) ) ;
#23406=CARTESIAN_POINT ( 'NONE',  ( 2.902940568641189323, 107.8364052097302306, 4.470325690468442303 ) ) ;
#23407=CARTESIAN_POINT ( 'NONE',  ( -12.35517153206337149, 152.0262389575480881, 0.8038591168380521124 ) ) ;
#23408=CARTESIAN_POINT ( 'NONE',  ( 4.310348487322937849, -12.41951052373176090, 1.878555342735434230 ) ) ;
#23409=CARTESIAN_POINT ( 'NONE',  ( 12.55519531044855697, 126.0212559692275249, -1.204658208757142246 ) ) ;
#23411=CARTESIAN_POINT ( 'NONE',  ( -6.111605970564546020, 157.2590385278250267, -1.959406070573513459 ) ) ;
#23413=CARTESIAN_POINT ( 'NONE',  ( 2.107392885931908211, -15.11054218480166433, 5.236909061670549370 ) ) ;
#23414=CARTESIAN_POINT ( 'NONE',  ( -4.910297347208772756, 117.4773399772923170, -1.095285516455568375 ) ) ;
#23415=CARTESIAN_POINT ( 'NONE',  ( 15.75440288366313268, 145.7063497038720925, 0.08391657230255397670 ) ) ;
#23418=FACE_OUTER_BOUND ( 'NONE', #11149, .T. ) ;
#23422=CARTESIAN_POINT ( 'NONE',  ( 23.20816695139192021, 149.6253602407241488, 0.3098579641399932250 ) ) ;
#23423=CARTESIAN_POINT ( 'NONE',  ( -5.379991719817741824, 116.9256180743815179, 0.7442756809649816452 ) ) ;
#23424=CARTESIAN_POINT ( 'NONE',  ( 1.741439286752546556, -15.57054322800294166, 5.502057211990651453 ) ) ;
#23426=CARTESIAN_POINT ( 'NONE',  ( -5.010339283552668554, 117.3993855393351566, -0.7509198670801209285 ) ) ;
#23427=CARTESIAN_POINT ( 'NONE',  ( 20.74782508767430755, 148.9555414352193168, 2.393722347598511657 ) ) ;
#23428=CARTESIAN_POINT ( 'NONE',  ( 4.610398055573782905, 23.01736123548795021, -0.3254830233858732602 ) ) ;
#23429=CARTESIAN_POINT ( 'NONE',  ( -4.329333532990936817, 10.85900946394830413, -7.254296797256971630 ) ) ;
#23430=CARTESIAN_POINT ( 'NONE',  ( -2.454038931915638599, 117.4443284220410533, -0.7335733216053069716 ) ) ;
#23431=CARTESIAN_POINT ( 'NONE',  ( -0.3093948633800919779, 109.1907409294041429, -4.022046774707581207 ) ) ;
#23433=DIRECTION ( 'NONE',  ( -0.9998004120163608288, 0.000000000000000000, -0.01997839162482747608 ) ) ;
#23434=CARTESIAN_POINT ( 'NONE',  ( -0.006734421712100887789, 121.9236798544229003, 0.3370180007451228366 ) ) ;
#23435=CARTESIAN_POINT ( 'NONE',  ( -1.861891798414337940, 1.167894131763866250, -4.247245584637167504 ) ) ;
#23438=CARTESIAN_POINT ( 'NONE',  ( 2.821697343786723877, -14.64683725402170289, 4.582568527534213843 ) ) ;
#23439=CARTESIAN_POINT ( 'NONE',  ( 4.022785008250933991, 122.0441497943765370, -0.1183375255305477575 ) ) ;
#23440=CARTESIAN_POINT ( 'NONE',  ( -7.827178552123696065, 158.6358315003295161, 0.5664908120210209175 ) ) ;
#23442=CARTESIAN_POINT ( 'NONE',  ( 4.999258502396517478, 117.4056799841109466, -0.8307607214361057979 ) ) ;
#23445=CARTESIAN_POINT ( 'NONE',  ( -4.855072294470597072, 115.7029491485453718, 1.279409886141102071 ) ) ;
#23446=CARTESIAN_POINT ( 'NONE',  ( 2.005403748902764516, -15.69871118693741430, 5.609036204238825540 ) ) ;
#23447=CARTESIAN_POINT ( 'NONE',  ( -5.005942668485581670, 118.7197616721209670, 0.8869178833313973165 ) ) ;
#23448=CARTESIAN_POINT ( 'NONE',  ( 19.13467844095158199, 131.8899703912256314, -1.275959715510668779 ) ) ;
#23449=CARTESIAN_POINT ( 'NONE',  ( 0.9754839647580387796, 27.70931421350951496, 0.02445524045744520980 ) ) ;
#23453=CARTESIAN_POINT ( 'NONE',  ( -4.973569738608247803, 117.3993868453981548, -0.9750659555622913643 ) ) ;
#23454=CARTESIAN_POINT ( 'NONE',  ( 1.733652500133013197, 120.5851793143259130, 0.4713357653683603044 ) ) ;
#23456=CARTESIAN_POINT ( 'NONE',  ( -10.16557698404471921, 154.1059161911440469, 1.245122368702753946 ) ) ;
#23457=CARTESIAN_POINT ( 'NONE',  ( 3.070829792790402024, 118.0750053011746985, 0.9656202980712693673 ) ) ;
#23458=CARTESIAN_POINT ( 'NONE',  ( 14.24002733280059374, 152.6618899727951089, -1.673933364105638866 ) ) ;
#23459=CARTESIAN_POINT ( 'NONE',  ( -13.08065502438839189, 121.7804325175133755, -1.718327614618424315 ) ) ;
#23462=CARTESIAN_POINT ( 'NONE',  ( 4.252665683302173427, 118.2250214913236448, -0.3074501678815576566 ) ) ;
#23464=CARTESIAN_POINT ( 'NONE',  ( 3.658657848224157405, 120.8687762150871379, -0.2216941123881816522 ) ) ;
#23466=CARTESIAN_POINT ( 'NONE',  ( 3.405374690515594605, -14.89039384781155917, 1.812165507210882209 ) ) ;
#23467=CARTESIAN_POINT ( 'NONE',  ( 5.314256983240370324, 105.1224655745845382, -0.4585143440169748841 ) ) ;
#23469=AXIS2_PLACEMENT_3D ( 'NONE', #40444, #11236, #11439 ) ;
#23470=CARTESIAN_POINT ( 'NONE',  ( 4.309711357183296343, 3.151582320728117725, 1.677628897243969464 ) ) ;
#23471=CARTESIAN_POINT ( 'NONE',  ( 10.31823449898706180, 154.1877054190025262, 1.778048316349531310 ) ) ;
#23473=CARTESIAN_POINT ( 'NONE',  ( 0.5299325911148425883, 33.81561889908242335, 0.8798404401248783868 ) ) ;
#23474=CARTESIAN_POINT ( 'NONE',  ( 2.488009491785908800, 18.85968022696138391, -3.895047602898422223 ) ) ;
#23475=CARTESIAN_POINT ( 'NONE',  ( 8.071037755102992151, 122.8559727437779827, 0.2401247476687870253 ) ) ;
#23476=CARTESIAN_POINT ( 'NONE',  ( -3.495814013870744308, 108.2588365649876607, 4.019948443012803629 ) ) ;
#23479=CARTESIAN_POINT ( 'NONE',  ( 5.562754537904068819, 116.7283259021707806, -0.08022358443418030338 ) ) ;
#23480=CARTESIAN_POINT ( 'NONE',  ( -0.03519895179131819068, 115.7029491485452866, 1.761499482103557446 ) ) ;
#23484=EDGE_CURVE ( 'NONE', #11121, #2591, #29505, .T. ) ;
#23489=CARTESIAN_POINT ( 'NONE',  ( -23.34493312772039175, 146.7646281656787437, -0.007662864037405678515 ) ) ;
#23492=CARTESIAN_POINT ( 'NONE',  ( 6.064603996746924075, 121.4401124717423528, 0.1114288923163564010 ) ) ;
#23493=ORIENTED_EDGE ( 'NONE', *, *, #11533, .T. ) ;
#23495=CARTESIAN_POINT ( 'NONE',  ( 0.0005023639977569234428, 120.9974662015457056, -0.02514034870427536705 ) ) ;
#23496=CARTESIAN_POINT ( 'NONE',  ( 6.473144302699227026, -13.19137087452153168, 0.2309683151692971392 ) ) ;
#23497=CARTESIAN_POINT ( 'NONE',  ( -20.65103440377624011, 150.0789294893613999, 1.463288793709878854 ) ) ;
#23498=CARTESIAN_POINT ( 'NONE',  ( -0.1328416520900886078, 24.48205809745167372, 4.627450821846854190 ) ) ;
#23499=CARTESIAN_POINT ( 'NONE',  ( 10.73501234801821802, 157.9381345072164038, 0.5669044750022473877 ) ) ;
#23500=CARTESIAN_POINT ( 'NONE',  ( 10.38578193225963275, 153.1602398435892383, 0.3880091275358500402 ) ) ;
#23501=CARTESIAN_POINT ( 'NONE',  ( 3.979181138743986601, 26.09377549647152961, 2.406711837290479661 ) ) ;
#23502=CARTESIAN_POINT ( 'NONE',  ( 0.8800754956866637668, -0.3565347152210476267, -0.4212773433312864690 ) ) ;
#23503=CARTESIAN_POINT ( 'NONE',  ( -16.82892344227272474, 155.2408147041404050, -0.5439083615366221425 ) ) ;
#23505=CARTESIAN_POINT ( 'NONE',  ( 4.962228190351918755, 117.4046759642803863, 1.029882822851095892 ) ) ;
#23507=CARTESIAN_POINT ( 'NONE',  ( -5.551989495070855263, 116.9209052717933446, 0.3361809518408999664 ) ) ;
#23508=CARTESIAN_POINT ( 'NONE',  ( -3.413396786258182658, 119.6896249646678569, 0.6770706109030820707 ) ) ;
#23510=CARTESIAN_POINT ( 'NONE',  ( 20.86684145051964734, 149.6610172957225586, 2.296701127946504606 ) ) ;
#23511=CARTESIAN_POINT ( 'NONE',  ( 5.880668475635486558, 119.2401804501882197, -0.9647153462086464071 ) ) ;
#23512=CARTESIAN_POINT ( 'NONE',  ( -0.4938630982110026046, -9.903502963049303887, 0.8462501600425517134 ) ) ;
#23513=CARTESIAN_POINT ( 'NONE',  ( -12.12330053995824741, 120.5818589831333441, -1.513795679345424361 ) ) ;
#23514=CARTESIAN_POINT ( 'NONE',  ( 4.668726057213791414, 118.0244701076749436, -0.5694989693638285999 ) ) ;
#23516=CARTESIAN_POINT ( 'NONE',  ( 4.831188462585346954, 104.6144662015456959, 0.2218974364397717225 ) ) ;
#23517=CARTESIAN_POINT ( 'NONE',  ( 6.522410937005443721, 121.2869106855140018, -0.5334890203407732789 ) ) ;
#23520=CARTESIAN_POINT ( 'NONE',  ( -5.832110448082723941, 156.9788419092994047, -1.931507550941140572 ) ) ;
#23521=CARTESIAN_POINT ( 'NONE',  ( 2.422525963563016749, -15.70080278133445617, 5.253054914258033392 ) ) ;
#23523=CARTESIAN_POINT ( 'NONE',  ( -4.571919090563273613, 118.0413024280605043, -0.8379947033858301531 ) ) ;
#23528=CARTESIAN_POINT ( 'NONE',  ( 17.85978967527192296, 148.7876888829155746, 2.377023446492704473 ) ) ;
#23529=CARTESIAN_POINT ( 'NONE',  ( -1.820350978615107751, 35.44831059284695129, 0.3018992756893351115 ) ) ;
#23531=CARTESIAN_POINT ( 'NONE',  ( 22.83540780336915432, 150.4058779721138421, 0.4563057931615321361 ) ) ;
#23533=CARTESIAN_POINT ( 'NONE',  ( 1.932697321913770416, 19.28018055242734619, -8.218723488459904303 ) ) ;
#23534=CARTESIAN_POINT ( 'NONE',  ( 15.91553746749626796, 146.9815093338748966, 1.044385907527698665 ) ) ;
#23536=CARTESIAN_POINT ( 'NONE',  ( 17.79905452297344937, 125.1550653296939970, -0.5857557929999462898 ) ) ;
#23540=B_SPLINE_CURVE_WITH_KNOTS ( 'NONE', 3,
 ( #9779, #41964, #18725, #31735, #8951, #22329, #35777, #21917, #19151, #22746, #38347, #32362, #35151, #6592, #32155, #41338, #12763, #2364, #5976, #6182, #2988, #18940, #38760, #31947, #3, #34947, #28330, #15950, #28947, #9571, #22541, #35568, #41759, #3190, #16152 ),
 .UNSPECIFIED., .F., .F.,
 ( 4, 1, 1, 1, 1, 1, 1, 1, 1, 1, 1, 1, 1, 1, 1, 1, 1, 1, 1, 1, 1, 1, 1, 1, 1, 1, 1, 1, 1, 1, 1, 1, 4 ),
 ( 0.000000000000000000, 0.02711375962671787321, 0.05385523109991235263, 0.08027126036152537614, 0.1064096946071439176, 0.1323192412471900226, 0.1580495177521483718, 0.1882118685537063907, 0.2182788543618764954, 0.2483346178351386324, 0.2784631806910429774, 0.3054937156393619513, 0.3327069032348308197, 0.3601597580799023035, 0.3879077415152338837, 0.4160045136367338525, 0.4445017332217630623, 0.4734489055539064517, 0.5028932750457014711, 0.5328797594123376724, 0.5634509204570880003, 0.5946469669818265080, 0.6265057848166851739, 0.6590629893014032792, 0.6923519956652609553, 0.7264041031822485728, 0.7612485893105871426, 0.7986318966073006065, 0.8369441774603861850, 0.8762126957585177900, 0.9164627945539034481, 0.9577180065289634392, 1.000000000000000000 ),
 .UNSPECIFIED. ) ;
#23542=DIRECTION ( 'NONE',  ( 4.017660918040594346E-17, -1.000000000000000000, -2.376309959284834438E-19 ) ) ;
#23544=UNCERTAINTY_MEASURE_WITH_UNIT (LENGTH_MEASURE( 1.000000000000000082E-05 ), #41838, 'distance_accuracy_value', 'NONE');
#23545=CARTESIAN_POINT ( 'NONE',  ( -16.10770497005625757, 121.2391669109744186, -0.2160841345999987839 ) ) ;
#23546=ORIENTED_EDGE ( 'NONE', *, *, #10721, .T. ) ;
#23547=CARTESIAN_POINT ( 'NONE',  ( -8.005205585284276282, 121.4511398066844521, -1.197578517849991586 ) ) ;
#23548=CARTESIAN_POINT ( 'NONE',  ( -8.635102817406197673, 118.5712416014078059, 0.7746300195078978934 ) ) ;
#23551=CARTESIAN_POINT ( 'NONE',  ( -4.529648377621004585, 121.1059516323014549, -0.2990124396216894409 ) ) ;
#23552=CARTESIAN_POINT ( 'NONE',  ( 4.658995561375286698, -13.35466759734559083, 3.413121997863386881 ) ) ;
#23553=CARTESIAN_POINT ( 'NONE',  ( -5.352805660278798783, 158.9031408473208273, 0.9771030980504661345 ) ) ;
#23555=CARTESIAN_POINT ( 'NONE',  ( 3.295257134497863838, 159.4684106755469202, 0.1128235000732134147 ) ) ;
#23557=CARTESIAN_POINT ( 'NONE',  ( -0.5842699607273857954, -4.454521554441356557, 4.585487691134133570 ) ) ;
#23558=CARTESIAN_POINT ( 'NONE',  ( -13.69515342115119694, 119.6466660129326272, -0.2899717296217780294 ) ) ;
#23561=CARTESIAN_POINT ( 'NONE',  ( -6.585129507136150195, 119.8605863436230692, 0.9846512238138591666 ) ) ;
#23562=CARTESIAN_POINT ( 'NONE',  ( -4.540528814728789442, -1.371322978654152092, -0.8806307088788817294 ) ) ;
#23563=CARTESIAN_POINT ( 'NONE',  ( 18.89746971955487709, 128.6554162386474047, 1.621015360058189581 ) ) ;
#23566=CARTESIAN_POINT ( 'NONE',  ( 7.829350110466591239, 119.0983413489662297, -1.000240898550800672 ) ) ;
#23567=CARTESIAN_POINT ( 'NONE',  ( -3.254339884055971854, 0.1279812147911008058, 3.287934741457726684 ) ) ;
#23568=CARTESIAN_POINT ( 'NONE',  ( -17.76144578550761111, 125.1550653296939970, -1.296339218450673014 ) ) ;
#23570=VERTEX_POINT ( 'NONE', #39096 ) ;
#23572=CARTESIAN_POINT ( 'NONE',  ( -11.35800195117484535, 128.2076764602477681, 0.1601657033123586593 ) ) ;
#23573=CARTESIAN_POINT ( 'NONE',  ( 2.466063760571058250, -15.50753052345275940, 5.840068263025540496 ) ) ;
#23575=CARTESIAN_POINT ( 'NONE',  ( -4.304088219600741283, 111.0463454453284555, -3.212841137876927711 ) ) ;
#23577=CARTESIAN_POINT ( 'NONE',  ( 12.33952200554331569, 155.1253022143813496, 2.231822996700852269 ) ) ;
#23581=CARTESIAN_POINT ( 'NONE',  ( -1.996658253870984723, 117.0827246868714013, 0.4092875891974779301 ) ) ;
#23582=CARTESIAN_POINT ( 'NONE',  ( 5.527521262545286085, 2.498091250051501344, 6.371381250375013572 ) ) ;
#23583=CARTESIAN_POINT ( 'NONE',  ( 0.5861964566936646026, 120.4790399057546182, 0.3305540093316995387 ) ) ;
#23584=CYLINDRICAL_SURFACE ( 'NONE', #3605, 3.175000000000001155 ) ;
#23585=CARTESIAN_POINT ( 'NONE',  ( 9.680782865131664749, 118.1749183431956425, -0.3159967629729716343 ) ) ;
#23594=CARTESIAN_POINT ( 'NONE',  ( -4.532383222279214863, 118.1210121875601118, 0.4790102578777305498 ) ) ;
#23595=CARTESIAN_POINT ( 'NONE',  ( 4.556421141688495879, 110.9173483060741887, -2.841207085095037943 ) ) ;
#23597=ORIENTED_EDGE ( 'NONE', *, *, #29018, .F. ) ;
#23599=CARTESIAN_POINT ( 'NONE',  ( -8.299000378089440133, 119.9939463870335743, -1.448799010205415128 ) ) ;
#23600=CARTESIAN_POINT ( 'NONE',  ( -6.114402651314438053, 119.5149100643186983, -0.5171552335003599676 ) ) ;
#23601=CARTESIAN_POINT ( 'NONE',  ( 4.512626992550961447, 118.1142824865469834, 0.7004059809699817452 ) ) ;
#23602=CARTESIAN_POINT ( 'NONE',  ( -7.725927843277678342, 122.1869765257964673, -0.7315739442948009374 ) ) ;
#23603=CARTESIAN_POINT ( 'NONE',  ( -1.123231675714139177, 115.7029491485453292, -1.744269607945097667 ) ) ;
#23604=CARTESIAN_POINT ( 'NONE',  ( 3.145428050085047555, 118.1651001541507355, -0.6645078962191128813 ) ) ;
#23605=CARTESIAN_POINT ( 'NONE',  ( 4.074523107743381445, 109.7948460773305897, -3.525254900318187445 ) ) ;
#23606=CARTESIAN_POINT ( 'NONE',  ( -10.62607977745490295, 123.8807653058400575, -1.354828998092944436 ) ) ;
#23607=CARTESIAN_POINT ( 'NONE',  ( -4.333424916720135300, 104.6144662015457243, 3.954443799498177370 ) ) ;
#23609=CARTESIAN_POINT ( 'NONE',  ( 8.323020013683247953, 120.1269634747937545, -1.118279847563949270 ) ) ;
#23610=CARTESIAN_POINT ( 'NONE',  ( -8.415924194183428853, 123.3149294549902493, -0.04043142641129342241 ) ) ;
#23611=CARTESIAN_POINT ( 'NONE',  ( 4.998195222330234166, 117.4629589511271348, -0.7743079785927495795 ) ) ;
#23612=CARTESIAN_POINT ( 'NONE',  ( -0.005431400947739826145, 116.8580640273661118, 0.2718095133625909043 ) ) ;
#23614=CARTESIAN_POINT ( 'NONE',  ( 1.977593594988821479, -15.25598227308876176, 5.283756247048868815 ) ) ;
#23615=CARTESIAN_POINT ( 'NONE',  ( -18.60513690094820305, 148.0519089404264150, 1.698284372519642371 ) ) ;
#23616=CARTESIAN_POINT ( 'NONE',  ( 0.8497018901738310204, -5.914940278964642140, -0.4796499176142879906 ) ) ;
#23617=CARTESIAN_POINT ( 'NONE',  ( -15.50334291652352370, 121.0440340969820596, -0.8284681841690884063 ) ) ;
#23619=CARTESIAN_POINT ( 'NONE',  ( -0.09873697212813982438, -3.591044343564580910, 0.9733856795103970061 ) ) ;
#23622=CARTESIAN_POINT ( 'NONE',  ( 4.310423192638969780, 113.1344509532474376, 2.465321907391796241 ) ) ;
#23624=CARTESIAN_POINT ( 'NONE',  ( -1.542034982439734581, 120.6610732671444595, 0.2472410911860531690 ) ) ;
#23625=CARTESIAN_POINT ( 'NONE',  ( 4.627184959846470491, -11.70336558297383611, 0.7419505617825855603 ) ) ;
#23626=CARTESIAN_POINT ( 'NONE',  ( 3.718565865971962925, 156.7231754051992425, -1.451222330515914871 ) ) ;
#23627=ORIENTED_EDGE ( 'NONE', *, *, #7122, .F. ) ;
#23628=CARTESIAN_POINT ( 'NONE',  ( -19.50074546578255053, 147.2819018089465715, -2.521100153936117305 ) ) ;
#23629=CARTESIAN_POINT ( 'NONE',  ( -4.722986921643055780, 104.6144662015457527, 1.042082362937506002 ) ) ;
#23630=CARTESIAN_POINT ( 'NONE',  ( 3.212496809824684441, -14.25148094350509353, 2.370051959060230473 ) ) ;
#23631=CARTESIAN_POINT ( 'NONE',  ( -4.863397889133672436, 117.6413937367854174, -1.052647808288214026 ) ) ;
#23632=CARTESIAN_POINT ( 'NONE',  ( 11.86471938700702466, 151.9842433124228762, 0.02191723269355114190 ) ) ;
#23634=ORIENTED_EDGE ( 'NONE', *, *, #31919, .T. ) ;
#23635=CARTESIAN_POINT ( 'NONE',  ( -2.933932892823386318, 107.6238140763627484, 4.446886960255170607 ) ) ;
#23636=CARTESIAN_POINT ( 'NONE',  ( 2.445884319531578033, 107.2200259173994112, 4.733447966000433382 ) ) ;
#23638=CARTESIAN_POINT ( 'NONE',  ( 4.758755041966881372, 116.8068435238802465, -0.07043225793504322152 ) ) ;
#23641=CARTESIAN_POINT ( 'NONE',  ( 1.878570595667757193, -15.26290889022100039, 5.982895072476400955 ) ) ;
#23643=CARTESIAN_POINT ( 'NONE',  ( -2.667392527469405916, 31.33771804890096746, 0.9893360403373154810 ) ) ;
#23644=CARTESIAN_POINT ( 'NONE',  ( 5.842949248259128758, 118.5625182843610617, 1.130067629703343624 ) ) ;
#23646=CARTESIAN_POINT ( 'NONE',  ( -2.728255833603390190, 14.33847684266025801, 7.992727065595903291 ) ) ;
#23647=CARTESIAN_POINT ( 'NONE',  ( 5.529981148835290128, 117.6928892124895896, -0.7912142295696815708 ) ) ;
#23648=CARTESIAN_POINT ( 'NONE',  ( -4.134812325682042378, 122.5143120247930142, -0.2378952825278685956 ) ) ;
#23649=CARTESIAN_POINT ( 'NONE',  ( -6.472048963935522405E-14, 69.43546620154573645, -1.207165458941418601E-19 ) ) ;
#23651=CARTESIAN_POINT ( 'NONE',  ( -5.284088079744258870, 105.1223998609899724, 0.8090923337965348905 ) ) ;
#23653=CARTESIAN_POINT ( 'NONE',  ( 4.440015753948663324, -2.305524871907271400, 1.325333094644747245 ) ) ;
#23657=CARTESIAN_POINT ( 'NONE',  ( 3.398501971686946010, -13.69110397484313246, 2.823423868610629217 ) ) ;
#23658=CARTESIAN_POINT ( 'NONE',  ( 0.2179432916432262890, 106.0530876078258586, -5.262233728842789837 ) ) ;
#23659=CARTESIAN_POINT ( 'NONE',  ( -4.841477346016104910, 117.1414559920645644, 0.3963857013944136476 ) ) ;
#23660=CARTESIAN_POINT ( 'NONE',  ( 4.801256233860562439, 117.4019745851689152, -1.015743786222129907 ) ) ;
#23664=CARTESIAN_POINT ( 'NONE',  ( 2.674787014790545481, -15.76824019788006304, 5.299902074303234123 ) ) ;
#23665=CARTESIAN_POINT ( 'NONE',  ( -2.650128318467547928, 158.3255140430775043, 1.577873239259485860 ) ) ;
#23666=CARTESIAN_POINT ( 'NONE',  ( 2.862861873098513588, -10.07698056833738320, -3.640125809621840069 ) ) ;
#23669=CARTESIAN_POINT ( 'NONE',  ( 1.058122102717250934, 124.9344662015457459, 0.02114379780294273203 ) ) ;
#23670=CARTESIAN_POINT ( 'NONE',  ( -10.06555281207545782, 123.2077283916686525, 0.8929836319946563572 ) ) ;
#23671=CARTESIAN_POINT ( 'NONE',  ( -6.263959367015712765, 28.84083519579221999, 0.1566845698765544637 ) ) ;
#23672=( BOUNDED_CURVE ( )  B_SPLINE_CURVE ( 3, ( #28985, #42002, #25790, #38795, #26853, #30460, #20231 ),
 .UNSPECIFIED., .F., .T. ) 
 B_SPLINE_CURVE_WITH_KNOTS ( ( 4, 3, 4 ),
 ( 0.4997054356531658859, 0.5000000000001099121, 0.5508374472049354376 ),
 .UNSPECIFIED. ) 
 CURVE ( )  GEOMETRIC_REPRESENTATION_ITEM ( )  RATIONAL_B_SPLINE_CURVE ( ( 0.9988224367574590756, 0.9992147264565607312, 0.9996072475374077060, 1.000000000000000000, 0.9322167370602015835, 0.8713253302225519858, 0.8173257794870510962 ) ) 
 REPRESENTATION_ITEM ( '' )  );
#23673=CARTESIAN_POINT ( 'NONE',  ( 10.44084688387110837, 122.0805278159965610, -1.176281030686837203 ) ) ;
#23674=CARTESIAN_POINT ( 'NONE',  ( -13.15656197906106684, 122.1656469061080514, -1.777190774585285071 ) ) ;
#23677=CARTESIAN_POINT ( 'NONE',  ( 4.267851022923248472, 118.2240358439523362, -0.2903317238581183957 ) ) ;
#23678=CARTESIAN_POINT ( 'NONE',  ( 1.653377498379587696, 156.2910218135955631, -0.4236837486942555131 ) ) ;
#23680=CARTESIAN_POINT ( 'NONE',  ( 3.172822981795960562, -14.65879537465078464, 0.2101774045261552148 ) ) ;
#23681=CARTESIAN_POINT ( 'NONE',  ( -4.866602953137410204, 117.4089747018453238, 0.9905608030323003188 ) ) ;
#23683=CARTESIAN_POINT ( 'NONE',  ( 4.531904421025400254, 4.026177021345840323, -0.9239884639389631671 ) ) ;
#23684=CARTESIAN_POINT ( 'NONE',  ( 1.432854634133363891, 120.0849730816093910, 0.5085234606245938593 ) ) ;
#23685=CARTESIAN_POINT ( 'NONE',  ( -1.474725677411676372, 32.11469766029267703, 1.198063404855159275 ) ) ;
#23688=CARTESIAN_POINT ( 'NONE',  ( -4.492784857928645792, 12.16275517495587977, -1.104450737933446725 ) ) ;
#23689=CARTESIAN_POINT ( 'NONE',  ( 15.72575858332438870, 145.6903699455376113, 0.3657738730356401846 ) ) ;
#23690=PLANE ( 'NONE',  #37179 ) ;
#23693=CARTESIAN_POINT ( 'NONE',  ( -8.792762063912906711, 117.6983032061184957, -0.2971417965732215394 ) ) ;
#23698=CARTESIAN_POINT ( 'NONE',  ( 3.113543590025587005, -0.1312883392403825233, -7.836836066719057747 ) ) ;
#23700=FACE_OUTER_BOUND ( 'NONE', #3055, .T. ) ;
#23702=CARTESIAN_POINT ( 'NONE',  ( -4.999405966312342464, 117.3993846663101266, -0.8267122116642939833 ) ) ;
#23703=CARTESIAN_POINT ( 'NONE',  ( -15.95511372484729051, 121.3860667298135070, 0.1093881341078833946 ) ) ;
#23706=CARTESIAN_POINT ( 'NONE',  ( 6.053201463129273208, 121.4432835561000985, 0.09870068995202660456 ) ) ;
#23709=CARTESIAN_POINT ( 'NONE',  ( 3.657801486795293044, 115.7029491485453008, -1.477931297577026459 ) ) ;
#23710=CARTESIAN_POINT ( 'NONE',  ( -11.06205061746909024, 128.0319838675845290, -0.2615737156286699339 ) ) ;
#23711=CARTESIAN_POINT ( 'NONE',  ( 4.841517317049865987, -14.78816330421856051, 4.356870016251622957 ) ) ;
#23713=CARTESIAN_POINT ( 'NONE',  ( -20.94193450296710068, 149.6610172957225586, 1.461262285038966047 ) ) ;
#23714=CARTESIAN_POINT ( 'NONE',  ( -0.8080508600641239658, 24.25718022715097533, 4.550674767031389401 ) ) ;
#23715=CARTESIAN_POINT ( 'NONE',  ( 15.09710430809799853, 156.1437908837410191, 0.6951944926208392106 ) ) ;
#23716=CARTESIAN_POINT ( 'NONE',  ( 15.75500244940657524, 145.8995334253134217, 0.5165061539673916347 ) ) ;
#23717=CARTESIAN_POINT ( 'NONE',  ( 0.6857505489063979720, -9.425274534614802135, -0.6942005185601292094 ) ) ;
#23718=B_SPLINE_CURVE_WITH_KNOTS ( 'NONE', 3,
 ( #6496, #5883, #39089, #15857, #13089, #15646, #25869, #6089 ),
 .UNSPECIFIED., .F., .F.,
 ( 4, 2, 2, 4 ),
 ( 0.000000000000000000, 0.0002285670694212123722, 0.0004571341388424247443, 0.0009142682776848494886 ),
 .UNSPECIFIED. ) ;
#23719=CARTESIAN_POINT ( 'NONE',  ( -18.60568445592648601, 154.1511370093759865, -0.5871577710369983993 ) ) ;
#23723=CARTESIAN_POINT ( 'NONE',  ( 5.529640237942972547, 117.0347480979416019, 0.6524371917319816694 ) ) ;
#23724=CARTESIAN_POINT ( 'NONE',  ( -18.00357552251037063, 146.8415343102147972, 1.578964580512863369 ) ) ;
#23726=CARTESIAN_POINT ( 'NONE',  ( 14.14688762606133388, 122.0820592118662091, 1.654226634644705873 ) ) ;
#23727=CARTESIAN_POINT ( 'NONE',  ( 1.263959281924152966, 118.7146927282448132, -0.6429003683496401500 ) ) ;
#23728=CARTESIAN_POINT ( 'NONE',  ( -0.5179912613141952615, -13.03896268189918217, -0.8249499322734266116 ) ) ;
#23729=CARTESIAN_POINT ( 'NONE',  ( 0.009513433763454561681, 117.6614778598761291, -0.4760911276077178234 ) ) ;
#23731=CARTESIAN_POINT ( 'NONE',  ( 3.853311296320406587, 104.6144662015434932, 3.705097815587511167 ) ) ;
#23733=CARTESIAN_POINT ( 'NONE',  ( 16.49265603038150374, 146.0252812507985141, -0.9509463687623791461 ) ) ;
#23734=CARTESIAN_POINT ( 'NONE',  ( -8.981069108608934926, 123.9698733229553937, -0.1794631345465899919 ) ) ;
#23736=CARTESIAN_POINT ( 'NONE',  ( -9.734001924785522064, 155.3230018269108825, -2.058186707467866139 ) ) ;
#23737=CARTESIAN_POINT ( 'NONE',  ( 4.357275237516622823, -15.68314232965556343, 3.240836981083619062 ) ) ;
#23739=CARTESIAN_POINT ( 'NONE',  ( -4.612168628140729254, 117.9566741055143524, -0.9390375305927243232 ) ) ;
#23741=CARTESIAN_POINT ( 'NONE',  ( 4.107391299159643516, 118.2429491485453497, 0.3509127516616104003 ) ) ;
#23742=CARTESIAN_POINT ( 'NONE',  ( 16.90821003499434383, 140.1729163700083518, 2.280195664865559912 ) ) ;
#23743=CARTESIAN_POINT ( 'NONE',  ( -4.432242455686237648, 32.76553509196318004, 1.287969469385144006 ) ) ;
#23746=CARTESIAN_POINT ( 'NONE',  ( 13.70496720262315193, 119.6480011847128253, 0.2738578607176475055 ) ) ;
#23747=CARTESIAN_POINT ( 'NONE',  ( 0.7770267621822702919, 9.899933826931993863, -8.437367074289049640 ) ) ;
#23748=CARTESIAN_POINT ( 'NONE',  ( 5.901573779631297256, 121.4708175001875077, 0.3521552259516175232 ) ) ;
#23749=CARTESIAN_POINT ( 'NONE',  ( 8.102197167284966639, 117.9965348323767671, -0.5618759090088266683 ) ) ;
#23751=CARTESIAN_POINT ( 'NONE',  ( 0.1669061836184802250, 115.6909491485452719, 1.766429643240662095 ) ) ;
#23752=ADVANCED_FACE ( 'NONE', ( #9694 ), #9922, .T. ) ;
#23753=CARTESIAN_POINT ( 'NONE',  ( -0.0008202526018428905668, 159.6052337359418800, 0.04104879434819971862 ) ) ;
#23756=CARTESIAN_POINT ( 'NONE',  ( 5.532952480631610825, 120.7401383209704733, -0.5099206179826454299 ) ) ;
#23759=CARTESIAN_POINT ( 'NONE',  ( -8.672603809708856915, 123.3259068333282755, -0.4768435845110673976 ) ) ;
#23760=CARTESIAN_POINT ( 'NONE',  ( 3.520038346949750707, -14.46602075298747359, 5.128058278438484052 ) ) ;
#23761=CARTESIAN_POINT ( 'NONE',  ( -17.11036550247955290, 125.2153959547233910, 0.9255656842583632749 ) ) ;
#23763=CARTESIAN_POINT ( 'NONE',  ( 9.813487807256207063, 117.9943556427423488, 0.2419611575297473949 ) ) ;
#23764=VERTEX_POINT ( 'NONE', #10326 ) ;
#23765=CARTESIAN_POINT ( 'NONE',  ( 4.611808778022512989, -11.57686662695173929, 0.3579861242195471194 ) ) ;
#23766=CARTESIAN_POINT ( 'NONE',  ( -23.11127252101368867, 149.9001116002701224, -0.4618182267416073850 ) ) ;
#23769=FACE_OUTER_BOUND ( 'NONE', #37797, .T. ) ;
#23771=CARTESIAN_POINT ( 'NONE',  ( -5.640823739553852079, 119.8537775533140604, 0.8705914987587907161 ) ) ;
#23774=CARTESIAN_POINT ( 'NONE',  ( -4.324967070706027705, -0.5217348546298696821, 1.653223044864502222 ) ) ;
#23775=CARTESIAN_POINT ( 'NONE',  ( 12.63141193514819705, 156.8164516032445306, 1.520932111850479496 ) ) ;
#23778=CARTESIAN_POINT ( 'NONE',  ( 12.83522892222227085, 121.3369795956499928, -1.134461614517290551 ) ) ;
#23779=CARTESIAN_POINT ( 'NONE',  ( -1.319288878716189828, -8.717950886928733212, 4.428293336331323715 ) ) ;
#23780=CARTESIAN_POINT ( 'NONE',  ( -22.54106487284180105, 146.4122051224262577, -1.767531409769413253 ) ) ;
#23781=ORIENTED_EDGE ( 'NONE', *, *, #40789, .T. ) ;
#23783=CARTESIAN_POINT ( 'NONE',  ( -8.132787923797444307, 122.8458379852381910, 0.04721391815988599389 ) ) ;
#23785=CARTESIAN_POINT ( 'NONE',  ( 6.471342906213767066, -13.19865009487615559, 0.2853922585125314715 ) ) ;
#23788=CARTESIAN_POINT ( 'NONE',  ( -0.3349390595691898453, 117.3993832489317128, -1.495620772394688602 ) ) ;
#23790=CARTESIAN_POINT ( 'NONE',  ( 11.78639615006484576, 122.5845257805695923, 1.760937685738447556 ) ) ;
#23793=CARTESIAN_POINT ( 'NONE',  ( -4.883164212476821753, 117.4312795728108227, 0.5545796311387337640 ) ) ;
#23794=CARTESIAN_POINT ( 'NONE',  ( -5.788041011255496748, 9.848169244510268427, 6.116426545680356597 ) ) ;
#23795=CARTESIAN_POINT ( 'NONE',  ( 7.827001302695538953, 121.9903164032602518, 0.9115841697347605299 ) ) ;
#23799=CARTESIAN_POINT ( 'NONE',  ( 19.82178279981176061, 128.7876384977266468, -0.3398896782655024817 ) ) ;
#23805=CARTESIAN_POINT ( 'NONE',  ( -4.361853176623482042, 118.1815349744495762, 0.4500548209967693003 ) ) ;
#23806=CARTESIAN_POINT ( 'NONE',  ( 1.205487064955253595, 106.0888231320280255, -5.200672005475023063 ) ) ;
#23809=CARTESIAN_POINT ( 'NONE',  ( 6.118303280479630679, 119.4740638505368509, -1.016964802927776468 ) ) ;
#23810=CARTESIAN_POINT ( 'NONE',  ( -7.301789825441274751, 123.0387167848234355, -0.2146691528375950508 ) ) ;
#23811=CARTESIAN_POINT ( 'NONE',  ( 4.575203770056261554, 118.0775004785955957, 0.7114012580090923743 ) ) ;
#23812=CARTESIAN_POINT ( 'NONE',  ( -15.16020740373479292, 148.9716719698033387, -1.401450122450045077 ) ) ;
#23813=CARTESIAN_POINT ( 'NONE',  ( -0.3140675500742723947, 115.7030945160809665, -1.764426291103405653 ) ) ;
#23814=AXIS2_PLACEMENT_3D ( 'NONE', #14712, #14921, #5164 ) ;
#23816=CARTESIAN_POINT ( 'NONE',  ( 7.140971181236829501, 122.4194348751405101, 0.03314210641492772169 ) ) ;
#23818=CARTESIAN_POINT ( 'NONE',  ( -12.69811389000567026, 152.1353413313561305, -1.627698677231679270 ) ) ;
#23819=DIRECTION ( 'NONE',  ( -4.017660918040594346E-17, 1.000000000000000000, 2.376309959284834438E-19 ) ) ;
#23822=CARTESIAN_POINT ( 'NONE',  ( 8.438003980598413278, 119.5616927475980305, -1.071839762751809033 ) ) ;
#23823=CARTESIAN_POINT ( 'NONE',  ( -8.948733625370710598, 124.0488388276255591, -0.04532362284662430629 ) ) ;
#23824=CARTESIAN_POINT ( 'NONE',  ( -3.682264917456324671, 97.37546620154573418, -0.07358041635423968885 ) ) ;
#23825=CARTESIAN_POINT ( 'NONE',  ( -0.005915287708770879636, 116.9295063353193882, 0.2960251855814710065 ) ) ;
#23827=CARTESIAN_POINT ( 'NONE',  ( 3.320832222217961593, -15.07605257934231702, 3.106094183260712516 ) ) ;
#23828=AXIS2_PLACEMENT_3D ( 'NONE', #4131, #6470, #36078 ) ;
#23829=CARTESIAN_POINT ( 'NONE',  ( -1.009415275228709108, 157.6350123088122359, 1.589207162029932174 ) ) ;
#23830=CARTESIAN_POINT ( 'NONE',  ( -0.1719059670432218079, -9.367746741450257986, 0.9581547781327369728 ) ) ;
#23831=CARTESIAN_POINT ( 'NONE',  ( -10.62864291685186480, 157.9324367681937815, -0.7848347606367999107 ) ) ;
#23832=CARTESIAN_POINT ( 'NONE',  ( -0.9568942166608355171, -5.529307923341535869, 0.1941686039811585662 ) ) ;
#23833=ORIENTED_EDGE ( 'NONE', *, *, #1224, .F. ) ;
#23835=CARTESIAN_POINT ( 'NONE',  ( 7.669310211018360413, 124.7206709383052043, 0.1531702926821041921 ) ) ;
#23837=CARTESIAN_POINT ( 'NONE',  ( -6.495086324198092065, 121.6155390319085683, 0.2579311815284318077 ) ) ;
#23838=CARTESIAN_POINT ( 'NONE',  ( 4.589616127059429118, -13.46842606041413681, 3.597705605327369494 ) ) ;
#23839=CARTESIAN_POINT ( 'NONE',  ( 9.755129750886695206, 122.6450757329969434, -0.9482731561257333741 ) ) ;
#23841=CARTESIAN_POINT ( 'NONE',  ( -8.582646176848058417, 120.3810071108087243, -1.481269161951472402 ) ) ;
#23842=CARTESIAN_POINT ( 'NONE',  ( 3.907822414802752942, 115.7034623327353700, 1.591805045670572571 ) ) ;
#23843=ADVANCED_FACE ( 'NONE', ( #14140 ), #7149, .T. ) ;
#23844=AXIS2_PLACEMENT_3D ( 'NONE', #33571, #36762, #4188 ) ;
#23845=CARTESIAN_POINT ( 'NONE',  ( 2.461817612451524084, -15.00653475910608492, 4.866425834902347702 ) ) ;
#23846=CARTESIAN_POINT ( 'NONE',  ( -4.768865426206803093, 117.4736200371610124, -1.192916987142205398 ) ) ;
#23847=CARTESIAN_POINT ( 'NONE',  ( 2.914310908016687129, 156.0868537499222839, -0.09385809996612891337 ) ) ;
#23848=EDGE_CURVE ( 'NONE', #26111, #30817, #28168, .T. ) ;
#23850=CARTESIAN_POINT ( 'NONE',  ( -3.945671927095251164, 109.6290767857811517, 3.598460797816132928 ) ) ;
#23851=CARTESIAN_POINT ( 'NONE',  ( 2.754021448042122344, 107.6241103294158421, 4.560424122646145051 ) ) ;
#23852=CARTESIAN_POINT ( 'NONE',  ( -14.91134437184023653, 120.3281135999119158, -0.2979641475767019765 ) ) ;
#23855=CARTESIAN_POINT ( 'NONE',  ( 23.35661798279346613, 142.7586093370927074, 0.2368412396931510178 ) ) ;
#23858=CARTESIAN_POINT ( 'NONE',  ( 1.650148621069484456, -15.47745783346181270, 5.677412139331382335 ) ) ;
#23860=CARTESIAN_POINT ( 'NONE',  ( 2.711364258112227255, 37.31625399494021877, -1.095520810760639119 ) ) ;
#23861=CARTESIAN_POINT ( 'NONE',  ( 18.06424110348773837, 131.7244750738095149, 2.230326231357608879 ) ) ;
#23863=CARTESIAN_POINT ( 'NONE',  ( -8.304712878168881929, 22.30428017260781459, 1.495267265505846765 ) ) ;
#23864=CARTESIAN_POINT ( 'NONE',  ( -5.525388478442741835, 117.9263796157108999, -1.079542212685845382 ) ) ;
#23865=CARTESIAN_POINT ( 'NONE',  ( -2.282361306983861748, 118.7862729053988318, -0.7764855222020031755 ) ) ;
#23867=CARTESIAN_POINT ( 'NONE',  ( -4.224169503853285157, 111.8944061756419899, -2.913215179389268439 ) ) ;
#23869=CARTESIAN_POINT ( 'NONE',  ( -0.8823465807374654135, 5.041073445128725794, 4.537322665494407659 ) ) ;
#23872=CARTESIAN_POINT ( 'NONE',  ( 3.011490660845400402, -14.57542554230247056, 4.052385860498629810 ) ) ;
#23873=CARTESIAN_POINT ( 'NONE',  ( 4.584908976607962927, 124.7699485019152945, 0.08702032153807698345 ) ) ;
#23874=CARTESIAN_POINT ( 'NONE',  ( -22.84463062875821038, 149.4631731099488832, 0.5130293307460866981 ) ) ;
#23875=CARTESIAN_POINT ( 'NONE',  ( 1.551849484730043249, 37.27687219050756084, 1.848690871642290734 ) ) ;
#23877=EDGE_LOOP ( 'NONE', ( #16722, #7810 ) ) ;
#23879=CARTESIAN_POINT ( 'NONE',  ( 4.790902082350968705, -15.53225359860559074, 1.708430371912022849 ) ) ;
#23880=CARTESIAN_POINT ( 'NONE',  ( -0.4701463269445154691, 118.5593716040226724, 0.5956656855050136423 ) ) ;
#23882=CARTESIAN_POINT ( 'NONE',  ( 0.6634555152105963138, 29.00466287695533296, -0.7151348822165174424 ) ) ;
#23883=B_SPLINE_CURVE_WITH_KNOTS ( 'NONE', 3,
 ( #10053, #7293, #3472, #23233, #279, #910, #16434, #23445 ),
 .UNSPECIFIED., .F., .F.,
 ( 4, 2, 2, 4 ),
 ( 0.000000000000000000, 0.2500000000000000000, 0.5000000000000000000, 1.000000000000000000 ),
 .UNSPECIFIED. ) ;
#23886=CARTESIAN_POINT ( 'NONE',  ( 0.2286055872008740109, 108.3383513567250986, 4.353007566726655675 ) ) ;
#23888=CARTESIAN_POINT ( 'NONE',  ( -8.809140270325823252, 122.1986804192922875, 0.8245386672919369220 ) ) ;
#23890=CARTESIAN_POINT ( 'NONE',  ( 18.60513690094807160, 148.0519089404264150, -1.698284372519642149 ) ) ;
#23891=AXIS2_PLACEMENT_3D ( 'NONE', #14002, #20589, #30401 ) ;
#23892=CARTESIAN_POINT ( 'NONE',  ( -11.41340492329623402, 156.2473422840488979, -2.091747920666957139 ) ) ;
#23894=CARTESIAN_POINT ( 'NONE',  ( 4.160584620051752225, 118.2392938275661862, -0.2307419219016439149 ) ) ;
#23895=CARTESIAN_POINT ( 'NONE',  ( 0.003756957834416090915, 120.7746249494737896, -0.1880135328902412806 ) ) ;
#23897=CARTESIAN_POINT ( 'NONE',  ( 3.178195937486941958, -14.44740043277138675, 1.484392166672811930 ) ) ;
#23901=CARTESIAN_POINT ( 'NONE',  ( -3.984361711520921556, 7.699456178644025428, -2.362637291489932068 ) ) ;
#23902=CARTESIAN_POINT ( 'NONE',  ( 10.36176036692635627, 123.5464890276372785, 1.327270239784479333 ) ) ;
#23903=CARTESIAN_POINT ( 'NONE',  ( -0.6138949730159162232, 32.89880662442777748, 0.9453277557968443601 ) ) ;
#23904=CARTESIAN_POINT ( 'NONE',  ( -0.8068095026012097604, 106.0274289318137306, 5.250488437364327687 ) ) ;
#23906=CIRCLE ( 'NONE', #16424, 0.5080000000000002292 ) ;
#23907=CARTESIAN_POINT ( 'NONE',  ( -0.6244342276652131707, 19.93415720681881353, -4.586363120317934694 ) ) ;
#23908=CARTESIAN_POINT ( 'NONE',  ( 15.64343260727701868, 147.2205073051419504, 0.4407941163815357610 ) ) ;
#23909=CARTESIAN_POINT ( 'NONE',  ( 8.798071512540863282, 117.6842349196870572, 0.1758064070670784795 ) ) ;
#23911=CARTESIAN_POINT ( 'NONE',  ( 8.797820204909040598, 117.6963758506564659, 0.06379098981978209570 ) ) ;
#23914=CARTESIAN_POINT ( 'NONE',  ( 2.081416901521091933, -15.50639809317535089, 5.943648939154567934 ) ) ;
#23916=CARTESIAN_POINT ( 'NONE',  ( -7.781828003681788175, 2.241565531857627303, -3.240848859074576094 ) ) ;
#23921=CARTESIAN_POINT ( 'NONE',  ( -18.56067064112295739, 154.1690995007799927, 0.05235235476399380250 ) ) ;
#23924=CARTESIAN_POINT ( 'NONE',  ( 6.995241510662618900, 121.9554695571096516, 0.1163068145497427736 ) ) ;
#23928=CARTESIAN_POINT ( 'NONE',  ( -8.770618086121094947, 123.6813396614493712, -0.1752578222716850986 ) ) ;
#23929=CARTESIAN_POINT ( 'NONE',  ( 2.079616623477898329, -15.54617723206731839, 5.925385729176050553 ) ) ;
#23930=CARTESIAN_POINT ( 'NONE',  ( -20.71566368020606319, 149.2407879669073054, 1.563226885547172929 ) ) ;
#23931=CARTESIAN_POINT ( 'NONE',  ( 2.832181158176134250, 116.7549172960530939, 0.3515502119895596023 ) ) ;
#23933=CARTESIAN_POINT ( 'NONE',  ( -4.559029627765868398, 31.49133049583988253, -0.6947656260628575220 ) ) ;
#23934=CARTESIAN_POINT ( 'NONE',  ( -21.47487836045326048, 132.5742979909900328, -0.7254175812904735121 ) ) ;
#23936=CARTESIAN_POINT ( 'NONE',  ( 4.812022206586005879, 117.4092931151362933, 1.196645100868244604 ) ) ;
#23937=CARTESIAN_POINT ( 'NONE',  ( -2.199325300168501585, 116.2221077253555137, 0.01996347552337981307 ) ) ;
#23938=CARTESIAN_POINT ( 'NONE',  ( -12.06094766868699431, 124.3217332413628640, 1.226997676231849077 ) ) ;
#23940=CARTESIAN_POINT ( 'NONE',  ( 19.50591060256576270, 149.0830822498907082, -1.724197071773047485 ) ) ;
#23941=CARTESIAN_POINT ( 'NONE',  ( 0.3740510792576948185, -8.494654975422754717, 0.8997923438783246297 ) ) ;
#23942=CARTESIAN_POINT ( 'NONE',  ( -20.18025034597674860, 150.8812763393641490, -2.199297964380012349 ) ) ;
#23945=CARTESIAN_POINT ( 'NONE',  ( 4.307098852976651848, 104.6144662015478701, 3.166141611896306607 ) ) ;
#23946=CARTESIAN_POINT ( 'NONE',  ( 10.15138120625587348, 123.9924233945428682, -0.7101534938561538945 ) ) ;
#23949=CARTESIAN_POINT ( 'NONE',  ( -11.39530606461031326, 123.1738952066917534, -1.661446624139454542 ) ) ;
#23950=CARTESIAN_POINT ( 'NONE',  ( 4.496247062743834455, -15.66418688627994804, 3.575535799018406014 ) ) ;
#23952=CARTESIAN_POINT ( 'NONE',  ( -4.434103822380226489, 118.1614506541414897, -0.6149899926561507302 ) ) ;
#23955=CARTESIAN_POINT ( 'NONE',  ( 17.78478073489614886, 148.4245508482893854, 2.330447787059698239 ) ) ;
#23958=CARTESIAN_POINT ( 'NONE',  ( 8.216926545874459364, 117.5004104479096583, 0.1641937475849289951 ) ) ;
#23959=CARTESIAN_POINT ( 'NONE',  ( 7.433834689873759061, 17.99627214424885580, -4.034796628604029323 ) ) ;
#23960=CARTESIAN_POINT ( 'NONE',  ( 8.161245858290078203, 122.8283871457973362, 0.4521822771171598032 ) ) ;
#23961=CARTESIAN_POINT ( 'NONE',  ( 14.88832262945823537, 121.0052616771249347, -0.5340607732653416262 ) ) ;
#23962=DIRECTION ( 'NONE',  ( 4.017660918040594346E-17, -1.000000000000000000, -2.376309959284834438E-19 ) ) ;
#23966=CARTESIAN_POINT ( 'NONE',  ( -23.38383716176070948, 142.7868430859564626, -0.3143897558744216947 ) ) ;
#23967=ORIENTED_EDGE ( 'NONE', *, *, #36211, .F. ) ;
#23969=CARTESIAN_POINT ( 'NONE',  ( -6.868495830644764766, 121.6811238109402211, -0.6472389319075357861 ) ) ;
#23970=CARTESIAN_POINT ( 'NONE',  ( -8.618292403345975572, 118.6571538964700352, 0.8118115907003122800 ) ) ;
#23972=CARTESIAN_POINT ( 'NONE',  ( 1.614075274083550671, 118.7629491485467952, -1.182329714217916106 ) ) ;
#23973=CARTESIAN_POINT ( 'NONE',  ( -15.64569453857185977, 147.5723176251010784, -0.9037163853702844252 ) ) ;
#23974=CARTESIAN_POINT ( 'NONE',  ( 4.939475803799734166, -12.60685243851100701, 2.184682653711520040 ) ) ;
#23975=CARTESIAN_POINT ( 'NONE',  ( -22.39365319421761313, 148.6363688457942942, 0.9991490326925100973 ) ) ;
#23977=CARTESIAN_POINT ( 'NONE',  ( 3.714261611334540358, 116.6275173757784813, 0.1151834636560012531 ) ) ;
#23979=CARTESIAN_POINT ( 'NONE',  ( 2.862861873098513588, -10.07698056833738320, -3.640125809621840069 ) ) ;
#23980=CARTESIAN_POINT ( 'NONE',  ( -20.69909148798433662, 152.5508394022679113, -0.4136171090298727537 ) ) ;
#23981=FACE_OUTER_BOUND ( 'NONE', #34029, .T. ) ;
#23985=CARTESIAN_POINT ( 'NONE',  ( 8.089976846435130042, 121.0247124080762120, 1.331332829722204680 ) ) ;
#23986=CARTESIAN_POINT ( 'NONE',  ( -4.360315236241580017, -1.596229544307166348, -1.535301415559372940 ) ) ;
#23987=CARTESIAN_POINT ( 'NONE',  ( 2.036215858770189513, 117.3535355059730705, 0.5825239229278259545 ) ) ;
#23989=CARTESIAN_POINT ( 'NONE',  ( 13.44120003175020628, 122.0388263298542739, -1.206224284286116610 ) ) ;
#23990=CARTESIAN_POINT ( 'NONE',  ( -4.434453077421578904, -10.21728329253013179, 1.368390957472948921 ) ) ;
#23991=CARTESIAN_POINT ( 'NONE',  ( -14.92386488306811465, 121.2513550155162960, -1.224273950129214583 ) ) ;
#23993=ORIENTED_EDGE ( 'NONE', *, *, #31869, .F. ) ;
#23994=CARTESIAN_POINT ( 'NONE',  ( -3.725873884401474267, 121.0563512343167645, 0.03194638937107886073 ) ) ;
#23995=CARTESIAN_POINT ( 'NONE',  ( 4.537411113424957065, -14.92057169651182846, 4.687841795668383327 ) ) ;
#23998=CARTESIAN_POINT ( 'NONE',  ( -0.3344305141284643068, 117.9496053196974259, -1.408475212110079200 ) ) ;
#23999=EDGE_CURVE ( 'NONE', #38197, #9800, #16613, .T. ) ;
#24000=EDGE_LOOP ( 'NONE', ( #15614, #9050, #8236, #34472 ) ) ;
#24001=CARTESIAN_POINT ( 'NONE',  ( 12.39214084994775966, 122.8403290575659526, 1.822206477283890624 ) ) ;
#24002=CARTESIAN_POINT ( 'NONE',  ( 4.877618761170128714, 117.7099338327117550, 0.9252109555340380931 ) ) ;
#24003=CARTESIAN_POINT ( 'NONE',  ( 4.756814333351318425, 117.4032681585794791, 1.206529664789174339 ) ) ;
#24005=CARTESIAN_POINT ( 'NONE',  ( -21.96051921721475964, 150.3855106993079005, 0.8576051660729392401 ) ) ;
#24006=CARTESIAN_POINT ( 'NONE',  ( 8.423846519715326053, 3.801276092563157682, 0.04266398729441032295 ) ) ;
#24007=CARTESIAN_POINT ( 'NONE',  ( 16.00153516066838932, 147.3640369757652877, 1.286050259728349632 ) ) ;
#24010=CARTESIAN_POINT ( 'NONE',  ( 23.01821387067764846, 149.5377445326608665, -0.2676165590851171672 ) ) ;
#24013=( LENGTH_UNIT ( ) NAMED_UNIT ( * ) SI_UNIT ( .MILLI., .METRE. ) );
#24016=ADVANCED_FACE ( 'NONE', ( #19400 ), #35613, .T. ) ;
#24017=CARTESIAN_POINT ( 'NONE',  ( -4.493334425098775675, 118.1300705548361378, 0.5259396578861340599 ) ) ;
#24021=EDGE_CURVE ( 'NONE', #1232, #11667, #448, .T. ) ;
#24022=CARTESIAN_POINT ( 'NONE',  ( -3.979033859436909459, 119.1284811785372426, -0.9228774962003568616 ) ) ;
#24023=CARTESIAN_POINT ( 'NONE',  ( -5.947819151547508731, 118.9610140496397719, -0.5876226394569609157 ) ) ;
#24025=CARTESIAN_POINT ( 'NONE',  ( 4.157985138387068069, 118.2393596361145427, 0.3861799695154242706 ) ) ;
#24026=CARTESIAN_POINT ( 'NONE',  ( -14.76847666019565253, 139.2804412874323248, -1.275673245633013320 ) ) ;
#24027=CARTESIAN_POINT ( 'NONE',  ( -0.5849308179726303569, 115.7029860318907737, -1.760411360667945013 ) ) ;
#24028=EDGE_CURVE ( 'NONE', #21265, #37727, #33628, .T. ) ;
#24029=CARTESIAN_POINT ( 'NONE',  ( 1.042872747090432206, 117.9496053355046996, -1.352030660431440268 ) ) ;
#24030=ORIENTED_EDGE ( 'NONE', *, *, #27647, .F. ) ;
#24031=CARTESIAN_POINT ( 'NONE',  ( 6.742182786528933214, 121.2177056076135528, -0.07361405433131842924 ) ) ;
#24032=CARTESIAN_POINT ( 'NONE',  ( -1.805426509874352048, 156.5029897098349636, -1.055579731365336116 ) ) ;
#24033=CARTESIAN_POINT ( 'NONE',  ( -5.329450492226126990, 104.6144662015457243, -0.2809636609891541514 ) ) ;
#24037=CARTESIAN_POINT ( 'NONE',  ( 6.079889191864811693, 121.4459138098642086, 0.1214906558318714913 ) ) ;
#24039=CARTESIAN_POINT ( 'NONE',  ( 15.29070941918896409, 121.1074504348956964, 0.9956366180447248082 ) ) ;
#24041=CARTESIAN_POINT ( 'NONE',  ( 3.231433726605559276, -14.53588044659766254, 1.883291753459793716 ) ) ;
#24042=CARTESIAN_POINT ( 'NONE',  ( -18.09865239071517351, 149.0664087073519681, 1.700023788287825521 ) ) ;
#24043=CARTESIAN_POINT ( 'NONE',  ( 0.5763570944828283471, -5.266575483494631449, -0.7860673829877594665 ) ) ;
#24044=CARTESIAN_POINT ( 'NONE',  ( -22.11976774214192432, 136.9573810088325843, -1.270382039940954000 ) ) ;
#24046=CARTESIAN_POINT ( 'NONE',  ( 0.9581548452940278349, 12.22225311242794099, 0.1719060106794997322 ) ) ;
#24047=ORIENTED_EDGE ( 'NONE', *, *, #27736, .T. ) ;
#24050=CARTESIAN_POINT ( 'NONE',  ( -16.03056103447438829, 147.0154580547469152, 0.5309802628845388117 ) ) ;
#24051=CARTESIAN_POINT ( 'NONE',  ( 2.039565395400614989, -15.13835760176744571, 5.886961163765535687 ) ) ;
#24052=CARTESIAN_POINT ( 'NONE',  ( 16.13547353508407411, 149.3012944676311804, -1.369731486774125040 ) ) ;
#24054=CARTESIAN_POINT ( 'NONE',  ( 4.799643950526473191, 115.7029491485453292, 1.472414092453835588 ) ) ;
#24055=CARTESIAN_POINT ( 'NONE',  ( 3.317891647977158076, -14.03051783662405327, 3.455980060616059113 ) ) ;
#24056=CARTESIAN_POINT ( 'NONE',  ( -4.958175139285456723, 117.4049635120808972, -1.028653955280601773 ) ) ;
#24057=CARTESIAN_POINT ( 'NONE',  ( 11.11302231477177394, 128.0707465396788507, 0.1214933242792291812 ) ) ;
#24059=CARTESIAN_POINT ( 'NONE',  ( 20.37866581877382544, 147.6366098820875266, 2.483541293540720840 ) ) ;
#24060=CARTESIAN_POINT ( 'NONE',  ( 3.009822844306053735, 107.7309519196189882, 4.394584667970089065 ) ) ;
#24061=CIRCLE ( 'NONE', #35634, 3.175000000000001155 ) ;
#24062=CARTESIAN_POINT ( 'NONE',  ( -3.932819197772146946, 27.98301002373794333, 0.4898618918306564263 ) ) ;
#24063=LINE ( 'NONE', #1926, #15675 ) ;
#24066=CARTESIAN_POINT ( 'NONE',  ( 8.212232005054447725, 117.5299140688306352, -0.02651185805045432747 ) ) ;
#24070=CARTESIAN_POINT ( 'NONE',  ( 1.929093603856297579, -15.52458459146700775, 5.992193855007914571 ) ) ;
#24072=CARTESIAN_POINT ( 'NONE',  ( -4.973366403791914081, 117.3993836135847459, -0.9761750303810099449 ) ) ;
#24073=CARTESIAN_POINT ( 'NONE',  ( 20.59518377851916426, 148.5655811199389689, 2.440016074255365819 ) ) ;
#24075=CARTESIAN_POINT ( 'NONE',  ( -8.412017540776835389, 12.59877214424737524, 0.8828606482577823211 ) ) ;
#24076=CARTESIAN_POINT ( 'NONE',  ( -2.262502884342421527, 117.0718098024412086, -0.6252834037462153827 ) ) ;
#24077=CARTESIAN_POINT ( 'NONE',  ( -3.352959238113231155, 119.3320731715853782, -0.6187547705018832112 ) ) ;
#24079=DIRECTION ( 'NONE',  ( 0.9998004120163609398, 0.000000000000000000, 0.01997839162482749689 ) ) ;
#24081=CARTESIAN_POINT ( 'NONE',  ( -0.0002200197270972112785, 124.8375573595198063, 0.01101068683960106966 ) ) ;
#24082=CARTESIAN_POINT ( 'NONE',  ( 2.267534764145236803, 6.115564135048844108, 4.037922524061999141 ) ) ;
#24083=ADVANCED_FACE ( 'NONE', ( #19195 ), #26596, .F. ) ;
#24085=CARTESIAN_POINT ( 'NONE',  ( -5.176291933393869726, 115.6909491485453003, 1.072167014217356051 ) ) ;
#24086=CARTESIAN_POINT ( 'NONE',  ( 3.202083396006969895, -13.65749169606385394, 1.964591208077046902 ) ) ;
#24087=CARTESIAN_POINT ( 'NONE',  ( 4.418733742721376423, 119.2572634999566930, -0.4175613206465202398 ) ) ;
#24088=CARTESIAN_POINT ( 'NONE',  ( 2.445139878417788015, 38.86123358755037316, 1.352914556568929116 ) ) ;
#24090=ORIENTED_EDGE ( 'NONE', *, *, #8464, .T. ) ;
#24091=CARTESIAN_POINT ( 'NONE',  ( -3.265249574949038891, 104.6144662015457243, -3.566735880799804637 ) ) ;
#24093=CARTESIAN_POINT ( 'NONE',  ( 3.468122426543017500, -15.77657449013483770, 4.627414140463686820 ) ) ;
#24094=CARTESIAN_POINT ( 'NONE',  ( -12.91500497980672968, 122.5866728308148055, 1.316509475493082393 ) ) ;
#24096=CARTESIAN_POINT ( 'NONE',  ( 0.3213417908193094141, 16.26526798020547204, 0.9222100932699727194 ) ) ;
#24100=CARTESIAN_POINT ( 'NONE',  ( 2.327304502367511851, 119.2037781873646622, 0.6856724729282703823 ) ) ;
#24101=CARTESIAN_POINT ( 'NONE',  ( -16.74402619291562289, 146.1290494286844819, 1.112937342747913894 ) ) ;
#24103=CARTESIAN_POINT ( 'NONE',  ( 0.03066982525775350035, 157.3074135339440147, -1.534843470138540500 ) ) ;
#24104=CARTESIAN_POINT ( 'NONE',  ( -11.75177080394836615, 120.8928578745602209, -1.619740935434792251 ) ) ;
#24107=CARTESIAN_POINT ( 'NONE',  ( 4.157314486619299920, 118.2390909874852269, -0.2343065005310382420 ) ) ;
#24108=CARTESIAN_POINT ( 'NONE',  ( 9.006799368204273293, 123.6974368934138226, -0.1328627719367737048 ) ) ;
#24110=CARTESIAN_POINT ( 'NONE',  ( 3.131015516031846690, -14.62848841321586946, 3.524024012273756501 ) ) ;
#24113=CARTESIAN_POINT ( 'NONE',  ( 1.173990663012069113, -13.46572784750561880, -4.469126434461346165 ) ) ;
#24114=CARTESIAN_POINT ( 'NONE',  ( 16.97388159461585388, 146.7604995623492243, 1.927701477367710803 ) ) ;
#24115=CARTESIAN_POINT ( 'NONE',  ( -0.8695339520022613566, 32.00309925763205854, 2.544523118616357937 ) ) ;
#24116=CARTESIAN_POINT ( 'NONE',  ( -4.798759560708047545, 116.6039038697339549, 0.9352253033319917197 ) ) ;
#24117=CARTESIAN_POINT ( 'NONE',  ( 3.465721614298269415, 18.43485028915299750, -3.064284189100199729 ) ) ;
#24118=CARTESIAN_POINT ( 'NONE',  ( 0.6448247514296147065, 156.3042436901572216, 0.08557349692115868989 ) ) ;
#24119=CARTESIAN_POINT ( 'NONE',  ( 4.760771785401275658, 118.7629491485453030, 0.9361126076443277988 ) ) ;
#24121=CARTESIAN_POINT ( 'NONE',  ( 8.793698859918160693, 117.7268288381244901, -0.04247273347103042163 ) ) ;
#24126=CARTESIAN_POINT ( 'NONE',  ( -7.580879709009198386, 3.543476842659112780, 3.722543307504006194 ) ) ;
#24127=EDGE_CURVE ( 'NONE', #35799, #12743, #11583, .T. ) ;
#24128=CARTESIAN_POINT ( 'NONE',  ( 5.326632231018254338, 115.7029491485453150, 0.4166893323572425367 ) ) ;
#24129=DIRECTION ( 'NONE',  ( -4.017660918040594346E-17, 1.000000000000000000, 2.376309959284834438E-19 ) ) ;
#24131=CARTESIAN_POINT ( 'NONE',  ( 0.009645608629770095407, 120.9711055683165597, -0.4827056984856004096 ) ) ;
#24132=CARTESIAN_POINT ( 'NONE',  ( -23.27509581586244636, 146.7258352529021863, 0.1368228026537803843 ) ) ;
#24136=ORIENTED_EDGE ( 'NONE', *, *, #8389, .T. ) ;
#24138=CARTESIAN_POINT ( 'NONE',  ( -15.21351360038804579, 143.4186079242267340, -0.3040022078858841126 ) ) ;
#24139=CARTESIAN_POINT ( 'NONE',  ( 4.031817627494778122, -15.29123897636591778, 5.054998095871475527 ) ) ;
#24140=CARTESIAN_POINT ( 'NONE',  ( -0.4301208033650349982, 117.9789173577105572, 0.5453690669796715795 ) ) ;
#24141=CARTESIAN_POINT ( 'NONE',  ( 2.968319594835611142, 117.2422168882539211, -0.4889809032577732140 ) ) ;
#24143=CARTESIAN_POINT ( 'NONE',  ( -18.58235751530899549, 154.1615476314759974, -0.6802042707109061670 ) ) ;
#24146=CARTESIAN_POINT ( 'NONE',  ( -2.184363492873007573, 116.1951706087090628, -0.02372223639846659723 ) ) ;
#24147=CARTESIAN_POINT ( 'NONE',  ( -12.17146470397786473, 153.5325627063460843, 1.540419412064476301 ) ) ;
#24149=CARTESIAN_POINT ( 'NONE',  ( 13.20509474233022473, 123.8872625266795211, -1.378179767694161173 ) ) ;
#24150=CARTESIAN_POINT ( 'NONE',  ( 0.1022289226565744474, -8.938468249466058779, 0.9708619238636220228 ) ) ;
#24151=CARTESIAN_POINT ( 'NONE',  ( -14.06037840947783657, 121.6707806233237363, -1.579157835890536710 ) ) ;
#24153=CARTESIAN_POINT ( 'NONE',  ( 12.52894620082560806, 152.0704867801853766, -0.9584603128924421567 ) ) ;
#24156=EDGE_LOOP ( 'NONE', ( #22859, #8033, #7054, #23069, #25205 ) ) ;
#24157=CARTESIAN_POINT ( 'NONE',  ( -15.09997037988956592, 131.2890697635526465, -2.122864649987122654 ) ) ;
#24158=CARTESIAN_POINT ( 'NONE',  ( 4.790902082350968705, -15.53225359860559074, 1.708430371912022849 ) ) ;
#24160=CARTESIAN_POINT ( 'NONE',  ( -4.280007282747122055, 118.2143720721413302, -0.5181209095560703748 ) ) ;
#24162=CARTESIAN_POINT ( 'NONE',  ( 4.112716839357073439, 118.2429491485453354, 0.3453384130802144014 ) ) ;
#24163=CARTESIAN_POINT ( 'NONE',  ( 3.383623802199790642, 119.6896249646678569, 0.8128912582704553857 ) ) ;
#24164=DIRECTION ( 'NONE',  ( 0.9998004120163609398, 4.016384292689130894E-17, 0.01997839162482749689 ) ) ;
#24165=CARTESIAN_POINT ( 'NONE',  ( 20.69909148798420517, 152.5508394022679113, 0.4136171090298729758 ) ) ;
#24166=CARTESIAN_POINT ( 'NONE',  ( 2.985612812371020386, 19.08565862607713370, -7.890306666671915714 ) ) ;
#24167=CARTESIAN_POINT ( 'NONE',  ( 15.83762317627076044, 145.9541952667573810, 0.7712195890315687308 ) ) ;
#24170=DIRECTION ( 'NONE',  ( -4.017660918040594346E-17, 1.000000000000000000, 2.376309959284834438E-19 ) ) ;
#24173=CARTESIAN_POINT ( 'NONE',  ( -0.3004615168032563344, 116.4565202671238069, 0.06108086412306423102 ) ) ;
#24174=CIRCLE ( 'NONE', #37804, 0.5079999999999997851 ) ;
#24177=CARTESIAN_POINT ( 'NONE',  ( -6.859007239851394822, 121.6278763642771139, -0.6877149167539079455 ) ) ;
#24178=CARTESIAN_POINT ( 'NONE',  ( -8.799660282941871969, 117.6859426315424599, -0.07877357120237717114 ) ) ;
#24179=EDGE_LOOP ( 'NONE', ( #8660, #3736, #21053, #5013 ) ) ;
#24180=CARTESIAN_POINT ( 'NONE',  ( 0.5329804096432148031, 115.7033785807872448, -1.742916349601860704 ) ) ;
#24181=CARTESIAN_POINT ( 'NONE',  ( -9.099523502024201349, 123.9936668703698075, -0.3412791990392151642 ) ) ;
#24182=CARTESIAN_POINT ( 'NONE',  ( 3.112015045868556928, -14.86597822091932564, 5.561823117377171499 ) ) ;
#24183=CARTESIAN_POINT ( 'NONE',  ( -21.68796372492899849, 149.3076860495818323, 1.274097349589627726 ) ) ;
#24185=CARTESIAN_POINT ( 'NONE',  ( 10.80923569951294461, 157.9177219752764358, 0.3353067243844873313 ) ) ;
#24186=CARTESIAN_POINT ( 'NONE',  ( 14.67500508075654508, 148.8517222230099719, 0.2932415260845993576 ) ) ;
#24188=CARTESIAN_POINT ( 'NONE',  ( -0.9756124605737610533, 22.95965383878278843, 0.006055453616918176837 ) ) ;
#24189=CARTESIAN_POINT ( 'NONE',  ( -1.797937260761374167, 116.4670535197835051, -0.04904229828524075269 ) ) ;
#24192=CARTESIAN_POINT ( 'NONE',  ( 4.799643950525145364, 115.7029491485460824, 1.472414092458888879 ) ) ;
#24193=VERTEX_POINT ( 'NONE', #15319 ) ;
#24194=CARTESIAN_POINT ( 'NONE',  ( 6.714516028680165505, 120.2572718181749849, 1.207797431051931492 ) ) ;
#24195=CARTESIAN_POINT ( 'NONE',  ( -4.120466288800530563, -1.808681497221679590, -2.133573495687988597 ) ) ;
#24196=CARTESIAN_POINT ( 'NONE',  ( 0.3765078121167834135, 117.5049145548240972, 0.4786851384288723366 ) ) ;
#24198=CARTESIAN_POINT ( 'NONE',  ( 1.193991991012501419, 158.7113841514841681, -1.470390664574136030 ) ) ;
#24199=CARTESIAN_POINT ( 'NONE',  ( 4.168288449772385995, -6.568960759998498489, 2.029292378399509378 ) ) ;
#24200=CARTESIAN_POINT ( 'NONE',  ( -1.027358375535146306, 117.1967307433898640, -0.4586652788708820982 ) ) ;
#24201=CARTESIAN_POINT ( 'NONE',  ( 4.805135882730054320, 117.7655461501371974, -0.8577152909912308942 ) ) ;
#24203=CARTESIAN_POINT ( 'NONE',  ( -15.75440288366326413, 145.7063497038720925, -0.08391657230255379629 ) ) ;
#24204=CARTESIAN_POINT ( 'NONE',  ( 4.209311184370442049, -15.24947937046475310, 4.910682269069504891 ) ) ;
#24205=CARTESIAN_POINT ( 'NONE',  ( 5.218844378615158597, 115.6909491485453145, 1.134975959208344598 ) ) ;
#24207=CIRCLE ( 'NONE', #1802, 5.588000000000006295 ) ;
#24209=CARTESIAN_POINT ( 'NONE',  ( 18.85642017384686753, 148.8558894138562039, 2.490767737705128493 ) ) ;
#24213=CARTESIAN_POINT ( 'NONE',  ( -7.640054841935688401, 158.5456267226934131, 0.8603666243017554782 ) ) ;
#24214=CARTESIAN_POINT ( 'NONE',  ( 3.645047284007026267, 5.522537913078280347, -7.602695550683356451 ) ) ;
#24215=CARTESIAN_POINT ( 'NONE',  ( -0.005430166084396237554, 120.5648899400503069, 0.2717477157510629904 ) ) ;
#24217=CARTESIAN_POINT ( 'NONE',  ( 18.19405586666655594, 125.1529741258727597, -0.3179404471852274594 ) ) ;
#24225=CARTESIAN_POINT ( 'NONE',  ( -4.162552958233026956, 118.2393839662436932, 0.2285457502593932766 ) ) ;
#24226=CARTESIAN_POINT ( 'NONE',  ( 2.469092600939023274, 107.0260912999244880, -4.723304494335009984 ) ) ;
#24227=VERTEX_POINT ( 'NONE', #14897 ) ;
#24229=CARTESIAN_POINT ( 'NONE',  ( 6.189399099425992645, 119.6256119081757134, -1.002760702448228125 ) ) ;
#24230=CARTESIAN_POINT ( 'NONE',  ( -5.227511188233297190, 116.2365830367532595, -1.175287748399642451 ) ) ;
#24231=CARTESIAN_POINT ( 'NONE',  ( 4.439117808263670639, 118.1598832799868291, 0.6092663547203902574 ) ) ;
#24232=CARTESIAN_POINT ( 'NONE',  ( -15.64597882779404259, 147.9168465093495399, -1.159024332450872663 ) ) ;
#24235=ORIENTED_EDGE ( 'NONE', *, *, #10202, .T. ) ;
#24236=CARTESIAN_POINT ( 'NONE',  ( 5.335400302754617741, 116.6867539651165373, -0.8102459553323388963 ) ) ;
#24237=CARTESIAN_POINT ( 'NONE',  ( -0.7656893570839061747, 156.6562795458349910, -1.120391489380295313 ) ) ;
#24238=EDGE_CURVE ( 'NONE', #38830, #28106, #21913, .T. ) ;
#24243=CARTESIAN_POINT ( 'NONE',  ( -15.19897562098254618, 143.3954161896175492, -0.1009949650227405238 ) ) ;
#24244=DIRECTION ( 'NONE',  ( -0.9998004120163609398, 0.000000000000000000, -0.01997839162482749689 ) ) ;
#24245=CARTESIAN_POINT ( 'NONE',  ( 22.44014329066001423, 150.2745577238280816, 1.412889903812419856 ) ) ;
#24247=CARTESIAN_POINT ( 'NONE',  ( 2.671714809844681238, -14.97371442308345380, 4.574436322856921144 ) ) ;
#24248=CARTESIAN_POINT ( 'NONE',  ( 21.49647223597088797, 141.8478887571778273, -1.286173174470951253 ) ) ;
#24249=CARTESIAN_POINT ( 'NONE',  ( -8.477251816686477426, 120.7201681212196291, 1.097727670418841672 ) ) ;
#24250=CARTESIAN_POINT ( 'NONE',  ( -0.8109939492151988505, -12.39128985057688936, -0.5387275711561630986 ) ) ;
#24251=CARTESIAN_POINT ( 'NONE',  ( -20.97948398557578642, 132.3427885975763161, -1.200284224572990555 ) ) ;
#24252=CARTESIAN_POINT ( 'NONE',  ( 0.6214172073067296687, 11.15065110656550118, 0.7500636867869169278 ) ) ;
#24255=CARTESIAN_POINT ( 'NONE',  ( -8.835859712557510903, 123.2701452714374568, 0.3110363621490747077 ) ) ;
#24256=CARTESIAN_POINT ( 'NONE',  ( 2.546550616605329775, -14.95902107118821078, 5.737972450990987738 ) ) ;
#24257=CARTESIAN_POINT ( 'NONE',  ( 8.008548550999964988, 121.6949282028273132, -0.7800530928440455591 ) ) ;
#24260=CARTESIAN_POINT ( 'NONE',  ( 0.5918605387268460749, 115.7030220337677378, 1.760228907466973913 ) ) ;
#24261=CARTESIAN_POINT ( 'NONE',  ( 2.905753382753808900, -13.11311505661566557, 0.7091545436608904796 ) ) ;
#24264=CARTESIAN_POINT ( 'NONE',  ( 5.933842156842870530, 121.5392726388429168, 0.04747900449317096760 ) ) ;
#24266=CARTESIAN_POINT ( 'NONE',  ( 4.065609891792011155, 118.4217611105734846, 0.9713962693593600761 ) ) ;
#24267=CARTESIAN_POINT ( 'NONE',  ( 1.903258124143570429, 106.6620211890854080, 4.980168853958236497 ) ) ;
#24268=TOROIDAL_SURFACE ( 'NONE', #41992, 5.080000000000005400, 0.5080000000000000071 ) ;
#24271=CARTESIAN_POINT ( 'NONE',  ( 0.003550357975880899172, 159.5989787797044812, -0.1776744311461874171 ) ) ;
#24273=CARTESIAN_POINT ( 'NONE',  ( 23.34154082800037244, 148.8574307740229585, 0.2355990431193898949 ) ) ;
#24275=CARTESIAN_POINT ( 'NONE',  ( 1.954897501163971985, -15.70563665752769467, 5.595021366335008572 ) ) ;
#24277=CARTESIAN_POINT ( 'NONE',  ( -3.151918684035726947, 30.94949030248789157, -0.3028545185056354394 ) ) ;
#24278=CARTESIAN_POINT ( 'NONE',  ( -4.725845587753020993, 117.9582415538433651, 0.6732661676528396422 ) ) ;
#24280=FACE_OUTER_BOUND ( 'NONE', #38867, .T. ) ;
#24281=CARTESIAN_POINT ( 'NONE',  ( -5.844880326603659526, 118.9651452168471621, -1.254347009492448262 ) ) ;
#24282=CARTESIAN_POINT ( 'NONE',  ( -3.169910341315210989, 118.2446163226072713, -0.8422023655252530716 ) ) ;
#24283=CARTESIAN_POINT ( 'NONE',  ( 4.764740839480360535, 117.6706990335958665, 1.115804577579641022 ) ) ;
#24284=DIRECTION ( 'NONE',  ( -0.9998004120163610509, -4.016384292689131511E-17, -0.01997839162482749689 ) ) ;
#24285=CARTESIAN_POINT ( 'NONE',  ( -0.02135216056130928922, 118.1497763966934258, 1.068549427312640132 ) ) ;
#24286=CIRCLE ( 'NONE', #3210, 3.175000000000001155 ) ;
#24287=CARTESIAN_POINT ( 'NONE',  ( -2.707926769430928804, 11.08828375386998033, -3.745406074561137721 ) ) ;
#24289=CARTESIAN_POINT ( 'NONE',  ( -4.826036362034073157, 118.5264896598256854, 0.7768203749786585233 ) ) ;
#24290=CARTESIAN_POINT ( 'NONE',  ( 3.884801864383396808, -13.20605796264157128, 2.953397552313849150 ) ) ;
#24291=CARTESIAN_POINT ( 'NONE',  ( 3.075034626192812759, 115.9530684888725460, -1.465612804093755273 ) ) ;
#24292=ADVANCED_FACE ( 'NONE', ( #41544, #24280 ), #34313, .F. ) ;
#24293=CARTESIAN_POINT ( 'NONE',  ( -3.422508068727017960, 30.97603876469775130, 4.291008727245660737 ) ) ;
#24294=CARTESIAN_POINT ( 'NONE',  ( -0.03519895178523997636, 115.7029491485446613, 1.761499482104069703 ) ) ;
#24297=CARTESIAN_POINT ( 'NONE',  ( 4.206901174280650579, -15.33509931759592604, 0.05204670666830889247 ) ) ;
#24298=CARTESIAN_POINT ( 'NONE',  ( -4.147108463826234548, 118.7489093234570561, 0.8374340306925344146 ) ) ;
#24299=CARTESIAN_POINT ( 'NONE',  ( 0.9593126492114073534, 18.43563504644844642, -0.1793159252426369810 ) ) ;
#24304=CARTESIAN_POINT ( 'NONE',  ( 3.291481622401924767, 124.4927030837263118, 0.08807361928342488655 ) ) ;
#24306=CARTESIAN_POINT ( 'NONE',  ( -16.77072586670524501, 146.3384789841921361, 1.111521918641044548 ) ) ;
#24307=EDGE_CURVE ( 'NONE', #12906, #6137, #37537, .T. ) ;
#24308=CYLINDRICAL_SURFACE ( 'NONE', #97, 3.175000000000001155 ) ;
#24309=CARTESIAN_POINT ( 'NONE',  ( 4.537180947476667114, 118.0682806366738049, -0.6375711883657442236 ) ) ;
#24310=CARTESIAN_POINT ( 'NONE',  ( 2.469877670440021600, 119.5064228623769225, -0.6390414609872483442 ) ) ;
#24311=CARTESIAN_POINT ( 'NONE',  ( -1.175363150376436350, 118.2527139659984101, -0.6673024542226160261 ) ) ;
#24313=CARTESIAN_POINT ( 'NONE',  ( 4.172632738300149136, 118.2392034709942976, -0.2169253999247517106 ) ) ;
#24314=CARTESIAN_POINT ( 'NONE',  ( 15.78585801821209422, 147.2673792861271522, -0.2768292828507332715 ) ) ;
#24316=CARTESIAN_POINT ( 'NONE',  ( 3.187143392547471255, -14.52651900126690876, 3.212499789951002604 ) ) ;
#24318=CARTESIAN_POINT ( 'NONE',  ( -4.901356651777482476, 117.4105916379840266, 0.9668049386046483340 ) ) ;
#24322=CARTESIAN_POINT ( 'NONE',  ( -4.540528814728789442, -1.371322978654152092, -0.8806307088788817294 ) ) ;
#24323=CARTESIAN_POINT ( 'NONE',  ( 10.02184412846586525, 123.2077283916686525, 1.294377628214502751 ) ) ;
#24324=CARTESIAN_POINT ( 'NONE',  ( -2.682217617217326211, 29.83982398439445305, 2.785746292651649192 ) ) ;
#24325=CARTESIAN_POINT ( 'NONE',  ( -1.225173952871761118, 106.6134986179334589, 4.982835752217485314 ) ) ;
#24326=CARTESIAN_POINT ( 'NONE',  ( 4.574821423538755205, -2.080616851812391310, 0.6590154617212384824 ) ) ;
#24327=CARTESIAN_POINT ( 'NONE',  ( 14.67688973683548781, 148.8424012017631242, 0.4203365054377474763 ) ) ;
#24330=CARTESIAN_POINT ( 'NONE',  ( -8.734361280028741348, 117.9425031322647612, -0.7137436082343942001 ) ) ;
#24331=APPLICATION_CONTEXT ( 'automotive_design' ) ;
#24332=CARTESIAN_POINT ( 'NONE',  ( 0.001862839608744629605, 124.0591982226671490, -0.09322411149286709275 ) ) ;
#24334=CARTESIAN_POINT ( 'NONE',  ( -1.156216728506892499, 106.1802426532317725, 5.165773742336502217 ) ) ;
#24335=CARTESIAN_POINT ( 'NONE',  ( -2.958531772299361595, 50.13146620154573441, -1.329372033065077119 ) ) ;
#24336=CARTESIAN_POINT ( 'NONE',  ( -0.3997009428961929567, 0.5197794802236572753, -8.431077252154732804 ) ) ;
#24338=CARTESIAN_POINT ( 'NONE',  ( 0.01009854879914063273, 117.2429491485453070, -0.5053730761605219612 ) ) ;
#24340=CARTESIAN_POINT ( 'NONE',  ( 0.03040743766744064339, 116.4813942609868178, -1.521712522323421579 ) ) ;
#24341=CARTESIAN_POINT ( 'NONE',  ( -18.50641704078269711, 154.1703991122031994, 0.1853567545699120467 ) ) ;
#24346=CARTESIAN_POINT ( 'NONE',  ( -9.163388821854908883, 124.2347608867413413, -0.1831063163140473349 ) ) ;
#24347=CARTESIAN_POINT ( 'NONE',  ( 4.537411113424957065, -14.92057169651182846, 4.687841795668383327 ) ) ;
#24348=CARTESIAN_POINT ( 'NONE',  ( -1.211137314531200770, 158.8088198215516229, 1.425359051240900454 ) ) ;
#24350=CARTESIAN_POINT ( 'NONE',  ( 14.55782549726406927, 156.0472725025049954, -0.8788902920476676650 ) ) ;
#24351=CARTESIAN_POINT ( 'NONE',  ( -4.151662239014343392, 13.23730288530712862, 2.070234887608822572 ) ) ;
#24352=CARTESIAN_POINT ( 'NONE',  ( -3.269635511691731722, 159.4655167044000166, -0.2664280249078421758 ) ) ;
#24357=CARTESIAN_POINT ( 'NONE',  ( -7.333780486663274090, 155.8804291298944236, 1.515250586328038995 ) ) ;
#24359=CARTESIAN_POINT ( 'NONE',  ( 4.252934711844570614, 157.4559852174668322, -1.675102021473321656 ) ) ;
#24360=CARTESIAN_POINT ( 'NONE',  ( -3.034986042679861828, 117.6993298527280984, -0.7527370910433333062 ) ) ;
#24362=CARTESIAN_POINT ( 'NONE',  ( 16.26403174311770883, 147.1082353761072454, -0.7878939306839420897 ) ) ;
#24363=VERTEX_POINT ( 'NONE', #38965 ) ;
#24364=CARTESIAN_POINT ( 'NONE',  ( -8.349261126152672574, 120.8878392079396065, -1.399984990019641495 ) ) ;
#24365=CARTESIAN_POINT ( 'NONE',  ( 3.591698533489739553, -15.62560650602327961, 3.738647084555763112 ) ) ;
#24366=CARTESIAN_POINT ( 'NONE',  ( -4.506702721058643668, 118.1222639539786456, -0.6633736078232330691 ) ) ;
#24370=CARTESIAN_POINT ( 'NONE',  ( 9.190671247345989059, 121.6705353891887995, 1.423780222299954268 ) ) ;
#24372=CARTESIAN_POINT ( 'NONE',  ( 16.14921358636486559, 121.2501203052637493, 0.2714571880805008441 ) ) ;
#24373=CARTESIAN_POINT ( 'NONE',  ( 4.034796628256747120, -3.593727855734754950, 7.433834689985365785 ) ) ;
#24374=CARTESIAN_POINT ( 'NONE',  ( 15.32629999177634872, 148.0267799683202554, 0.7554886701871541543 ) ) ;
#24377=DIRECTION ( 'NONE',  ( 4.017660918040594346E-17, -1.000000000000000000, -2.376309959284834438E-19 ) ) ;
#24378=CARTESIAN_POINT ( 'NONE',  ( -3.343419727707106492, 118.1588900059306440, 0.6560610098329158202 ) ) ;
#24382=CARTESIAN_POINT ( 'NONE',  ( -11.70725067560583099, 118.7242475115495495, -0.1376448473428154018 ) ) ;
#24383=B_SPLINE_CURVE_WITH_KNOTS ( 'NONE', 3,
 ( #36569, #24178, #13970, #26974, #37187, #26552, #8009, #29954, #14175, #39775, #23548, #40193, #23970, #21385, #24387, #31200, #38245, #40600, #24813, #1631, #18628, #18411, #11609, #27591, #41230, #28438, #34210, #8633, #15008, #24593, #8426, #18199, #21182, #11400, #34411, #5038, #28007, #17995, #2043, #14797, #15435, #30993, #21811, #35056, #37600, #21596, #41016, #28224, #9062, #27800, #11824, #14586, #34624, #5451, #22027, #37392 ),
 .UNSPECIFIED., .F., .F.,
 ( 4, 2, 2, 2, 2, 1, 2, 2, 2, 2, 2, 2, 1, 2, 2, 2, 2, 2, 1, 1, 2, 2, 2, 2, 1, 1, 2, 2, 2, 2, 4 ),
 ( 0.000000000000000000, 0.06249999999998684386, 0.1249999999999736877, 0.1874999999999605316, 0.2187499999999565903, 0.2343749999999545919, 0.2421874999999535372, 0.2499999999999524825, 0.3749999999999020783, 0.4374999999998734901, 0.4687499999998556155, 0.4843749999998465117, 0.4921874999998457345, 0.4960937499998452904, 0.4999999999998448463, 0.6249999999998867573, 0.6874999999999077405, 0.7187499999999182876, 0.7343749999999272804, 0.7421874999999317213, 0.7460937499999302780, 0.7499999999999289457, 0.8124999999998901989, 0.8437499999998708811, 0.8593749999998642197, 0.8671874999998637756, 0.8710937499998634426, 0.8749999999998632205, 0.9374999999999336087, 0.9687499999999668043, 1.000000000000000000 ),
 .UNSPECIFIED. ) ;
#24384=ORIENTED_EDGE ( 'NONE', *, *, #5071, .F. ) ;
#24386=CARTESIAN_POINT ( 'NONE',  ( -7.905494947253956184, 121.9601156449555219, -0.9643286209291552780 ) ) ;
#24387=CARTESIAN_POINT ( 'NONE',  ( -8.561575482294372819, 118.9452303826418529, 0.9294693558781963461 ) ) ;
#24389=CARTESIAN_POINT ( 'NONE',  ( 0.5401341148544321902, 115.6909491485452719, -1.744863588967870527 ) ) ;
#24390=CARTESIAN_POINT ( 'NONE',  ( -15.29340151118749525, 148.0176312819745874, -0.6334265850898868067 ) ) ;
#24391=CARTESIAN_POINT ( 'NONE',  ( 3.361239686659836856, -14.56070858809799162, 5.257229516148527182 ) ) ;
#24392=CARTESIAN_POINT ( 'NONE',  ( -1.297493386698629125, 159.2526592949493534, 1.079139715401668420 ) ) ;
#24393=CYLINDRICAL_SURFACE ( 'NONE', #23351, 5.588000000000006295 ) ;
#24394=CARTESIAN_POINT ( 'NONE',  ( 13.41573142586483591, 156.9389434127184018, 0.3962193537810602684 ) ) ;
#24395=CARTESIAN_POINT ( 'NONE',  ( 11.79002894202885265, 130.2874576319956361, 0.2924100448099202776 ) ) ;
#24396=CARTESIAN_POINT ( 'NONE',  ( -5.028626460200799286, 117.3993840973718932, 0.6246689785710292098 ) ) ;
#24397=CARTESIAN_POINT ( 'NONE',  ( -0.6395729929254629909, 24.25746453972198680, 0.7366970655621520869 ) ) ;
#24398=CARTESIAN_POINT ( 'NONE',  ( -16.86029543505362227, 155.2078297922403465, -0.3599557924993777580 ) ) ;
#24401=VERTEX_POINT ( 'NONE', #25747 ) ;
#24402=CARTESIAN_POINT ( 'NONE',  ( 8.314316052578815786, 119.9194173129146748, 1.447167333058394512 ) ) ;
#24403=CARTESIAN_POINT ( 'NONE',  ( 3.417104117279694098, -14.34023910220586906, -3.129441506049576383 ) ) ;
#24404=CARTESIAN_POINT ( 'NONE',  ( 22.03343284943298030, 146.2042277794223537, 2.039575571141828192 ) ) ;
#24406=CARTESIAN_POINT ( 'NONE',  ( 20.46656357041385377, 147.8414448467482600, -1.666390110339677655 ) ) ;
#24407=CARTESIAN_POINT ( 'NONE',  ( 6.480130183504051011, 21.94006803110874415, 5.378050974841823262 ) ) ;
#24408=CARTESIAN_POINT ( 'NONE',  ( -21.46783008853691754, 136.6907720476960435, -1.692068800591147060 ) ) ;
#24409=CARTESIAN_POINT ( 'NONE',  ( 4.948841739784780813, 117.6230884628553497, -0.7513042659447916050 ) ) ;
#24411=CARTESIAN_POINT ( 'NONE',  ( -12.04197430995787954, 130.4833683797432684, 0.05493623226408311799 ) ) ;
#24413=CARTESIAN_POINT ( 'NONE',  ( 6.479796796485603139, -13.80134569450770776, 0.08439370571411514144 ) ) ;
#24415=CARTESIAN_POINT ( 'NONE',  ( -3.743775977915335229, 109.0594729580190005, -3.805242568780236478 ) ) ;
#24417=CARTESIAN_POINT ( 'NONE',  ( 5.836180790127331264, 119.4106843418347950, 1.193569107438471333 ) ) ;
#24419=DIRECTION ( 'NONE',  ( 0.01997839162482749689, 1.040247600000945640E-18, -0.9998004120163610509 ) ) ;
#24420=CARTESIAN_POINT ( 'NONE',  ( -0.3199181899540057272, 107.4969721965504021, 4.676354563382915330 ) ) ;
#24421=CARTESIAN_POINT ( 'NONE',  ( 1.285294229880325600, 5.975470260049262627, -8.359553334813638159 ) ) ;
#24422=CARTESIAN_POINT ( 'NONE',  ( 6.483461908857734102, 121.4942169270607053, 0.6390524964423263121 ) ) ;
#24424=CARTESIAN_POINT ( 'NONE',  ( 16.66487874612757736, 155.2617138006751532, -0.3247879035468687614 ) ) ;
#24427=LINE ( 'NONE', #37432, #11910 ) ;
#24429=DIRECTION ( 'NONE',  ( 0.01997839162482749689, 1.040247600000945640E-18, -0.9998004120163610509 ) ) ;
#24430=CARTESIAN_POINT ( 'NONE',  ( -4.115839894752868489, 118.2429491485453354, 0.1890361656430152582 ) ) ;
#24431=CARTESIAN_POINT ( 'NONE',  ( 3.156006274272449286, 108.3452893864970150, -4.146484234041631467 ) ) ;
#24435=CARTESIAN_POINT ( 'NONE',  ( -8.276141957500152913, 120.1053043740212445, -1.449957327947475338 ) ) ;
#24438=CARTESIAN_POINT ( 'NONE',  ( 4.407114152208388980, 118.1655186915589297, 0.6432706596802734156 ) ) ;
#24439=CARTESIAN_POINT ( 'NONE',  ( -3.646880827531788327, 120.8687762150871379, -0.3676761613455564182 ) ) ;
#24440=CARTESIAN_POINT ( 'NONE',  ( 5.009498726350964937, 117.5220155938639977, -0.6178361814830906074 ) ) ;
#24442=EDGE_LOOP ( 'NONE', ( #13394, #28394, #12175, #37597 ) ) ;
#24443=CARTESIAN_POINT ( 'NONE',  ( -4.420329592304260480, 21.65838872207745425, -1.398650104627336743 ) ) ;
#24444=CARTESIAN_POINT ( 'NONE',  ( -8.539651237459656485, 154.7538831414287870, -1.439145765679522571 ) ) ;
#24448=CARTESIAN_POINT ( 'NONE',  ( -6.065173057319897865, 121.4418940636094391, -0.09687486233282362191 ) ) ;
#24449=CARTESIAN_POINT ( 'NONE',  ( 4.915103509140258176, 117.7039392452923323, -0.7324920538677794912 ) ) ;
#24450=CARTESIAN_POINT ( 'NONE',  ( 22.37507221999716478, 149.9331680011685251, 1.622875787667645842 ) ) ;
#24452=CARTESIAN_POINT ( 'NONE',  ( 2.985050690391415795, -14.25097394772453718, 0.5935303709388186633 ) ) ;
#24453=CARTESIAN_POINT ( 'NONE',  ( 0.02615207601215380553, 159.0391464308674756, -1.308756824028193266 ) ) ;
#24454=CARTESIAN_POINT ( 'NONE',  ( -4.149433946629451420, 157.3082466949932723, 1.660590259719063599 ) ) ;
#24455=CARTESIAN_POINT ( 'NONE',  ( -4.295268622494708310, 18.69437521248495671, 1.722957355393906598 ) ) ;
#24456=CARTESIAN_POINT ( 'NONE',  ( -23.06261834269087174, 146.6371693212631158, -1.324134011023372581 ) ) ;
#24457=CARTESIAN_POINT ( 'NONE',  ( 0.9708619386763404080, 12.65153173543952470, -0.1022289352641109206 ) ) ;
#24458=EDGE_LOOP ( 'NONE', ( #10860, #29019, #18363, #26187 ) ) ;
#24460=CARTESIAN_POINT ( 'NONE',  ( -10.06005632938197714, 124.8772485319846055, 0.3443025955426560758 ) ) ;
#24461=CARTESIAN_POINT ( 'NONE',  ( 5.306636623844629419, -13.66766582561489152, 3.280230747366464694 ) ) ;
#24462=CARTESIAN_POINT ( 'NONE',  ( 11.73912714423988390, 153.3684197651487580, -1.370860710263249960 ) ) ;
#24464=CARTESIAN_POINT ( 'NONE',  ( 1.784244551060144124, 115.7029491485453292, 1.723397082296914684 ) ) ;
#24466=CARTESIAN_POINT ( 'NONE',  ( 3.011490660845400402, -14.57542554230247056, 4.052385860498629810 ) ) ;
#24467=CARTESIAN_POINT ( 'NONE',  ( -4.873043952982492044, 117.7164335358027216, -0.9339496037525177874 ) ) ;
#24469=CARTESIAN_POINT ( 'NONE',  ( 15.23158847265882621, 143.4365109762209158, 0.1756275167766376266 ) ) ;
#24471=EDGE_LOOP ( 'NONE', ( #29949, #34702, #7925, #39474 ) ) ;
#24472=CARTESIAN_POINT ( 'NONE',  ( -0.03153870137021896197, 158.4432089348667319, 1.578325583784928154 ) ) ;
#24473=FACE_OUTER_BOUND ( 'NONE', #30971, .T. ) ;
#24474=CARTESIAN_POINT ( 'NONE',  ( 0.009747742627749139341, 156.3581291470199233, -0.4878169013068171522 ) ) ;
#24475=CARTESIAN_POINT ( 'NONE',  ( 23.27479113596625382, 149.3390083238215595, 0.2346540593346971015 ) ) ;
#24477=CARTESIAN_POINT ( 'NONE',  ( 1.774274676131157191, -15.12224598438900713, 5.803401512178314015 ) ) ;
#24480=CARTESIAN_POINT ( 'NONE',  ( -4.839665964887291949, 117.8306912978229377, 0.7068891268956964957 ) ) ;
#24481=B_SPLINE_SURFACE_WITH_KNOTS ( 'NONE', 1, 3, ( 
 ( #18440, #28252, #12065, #25052, #30608, #14408, #27415, #24205, #22057, #12279, #41684, #3336 ),
 ( #15667, #29090, #35084, #5905, #2501, #15880, #16305, #150, #29306, #9712, #22678, #2713 ) ),
 .UNSPECIFIED., .F., .F., .F.,
 ( 2, 2 ),
 ( 4, 3, 2, 3, 4 ),
 ( 0.000000000000000000, 1.000000000000000000 ),
 ( -0.01867714150337349693, 0.000000000000000000, 0.5000000000000000000, 1.000000000000000000, 1.010000000000000009 ),
 .UNSPECIFIED. ) ;
#24484=CARTESIAN_POINT ( 'NONE',  ( -4.855364188028922001, 117.4053679690828602, 1.004246593774441365 ) ) ;
#24485=CARTESIAN_POINT ( 'NONE',  ( -2.609399678953878698, 117.6784490614926426, -0.7904977363455250039 ) ) ;
#24486=CARTESIAN_POINT ( 'NONE',  ( -4.584725329088070289, 124.7699485019152945, -0.09621079440654284332 ) ) ;
#24487=CARTESIAN_POINT ( 'NONE',  ( 4.872669516377786003, 117.7163985243862783, 0.9341506115307878222 ) ) ;
#24488=CARTESIAN_POINT ( 'NONE',  ( -4.707492808873059431, 117.7228541735984066, -1.103909285615471081 ) ) ;
#24489=CARTESIAN_POINT ( 'NONE',  ( -0.2858543223548531964, 109.4728569552520554, 3.914881836256077552 ) ) ;
#24490=CARTESIAN_POINT ( 'NONE',  ( -4.637963820743935983, -6.603494994175692412, 0.1710436084038768345 ) ) ;
#24491=CARTESIAN_POINT ( 'NONE',  ( 4.828127062081292387, 117.4060377263907213, -1.008211717711906541 ) ) ;
#24492=CARTESIAN_POINT ( 'NONE',  ( -4.808499656004150857, 118.5264896598256854, 0.8103638877405311414 ) ) ;
#24493=CARTESIAN_POINT ( 'NONE',  ( 3.497624268394256219, -13.57517324819364291, 2.900746184505403669 ) ) ;
#24495=CARTESIAN_POINT ( 'NONE',  ( 5.936300781872302146, 120.8604418758245487, -0.1421746502253221078 ) ) ;
#24496=CARTESIAN_POINT ( 'NONE',  ( -4.734860929486131909, 29.02688818834038642, 2.807733122327669140 ) ) ;
#24497=CARTESIAN_POINT ( 'NONE',  ( -6.519774838065697039E-14, 78.83346620154574680, 1.207165459601591275E-19 ) ) ;
#24498=CARTESIAN_POINT ( 'NONE',  ( -0.01876340930523686876, 19.73428105357427853, -4.634220987317214657 ) ) ;
#24500=CARTESIAN_POINT ( 'NONE',  ( 2.199016089875075686, -15.62526216655714428, 5.252760144517266916 ) ) ;
#24501=CARTESIAN_POINT ( 'NONE',  ( -4.169621149806146398, 118.9132445967212419, 0.8414384147219283738 ) ) ;
#24502=CARTESIAN_POINT ( 'NONE',  ( 0.5584349385955980072, -2.506542431320444742, 0.8015440831694167212 ) ) ;
#24503=CARTESIAN_POINT ( 'NONE',  ( 0.9733856798199480576, 17.99895565637743999, 0.09873697238165508872 ) ) ;
#24505=EDGE_LOOP ( 'NONE', ( #5892, #33403, #4068, #3025 ) ) ;
#24507=CARTESIAN_POINT ( 'NONE',  ( 3.662133038521572903, 120.6652674781340551, 0.4257566204602385995 ) ) ;
#24508=CARTESIAN_POINT ( 'NONE',  ( -16.34996387626505765, 143.9496486471311698, 1.129508837753296691 ) ) ;
#24509=CARTESIAN_POINT ( 'NONE',  ( -3.682264917456324671, 97.88346620154572975, -0.07358041635423967497 ) ) ;
#24510=CARTESIAN_POINT ( 'NONE',  ( 4.605456961276924943, 118.0199559457295067, -0.6871734479863592648 ) ) ;
#24511=CARTESIAN_POINT ( 'NONE',  ( 4.278356142283907815, 119.7015364213435333, -0.7555980432150395387 ) ) ;
#24512=CARTESIAN_POINT ( 'NONE',  ( -12.76651978940624410, 122.1393999080170971, -1.787974849574114122 ) ) ;
#24514=AXIS2_PLACEMENT_3D ( 'NONE', #7926, #30697, #17910 ) ;
#24515=ADVANCED_FACE ( 'NONE', ( #6588 ), #9563, .F. ) ;
#24516=CARTESIAN_POINT ( 'NONE',  ( -0.02537255736359545280, 39.20946620154573026, 1.269746523260778304 ) ) ;
#24517=CARTESIAN_POINT ( 'NONE',  ( 9.945677869404924820, 124.8826105625126530, -0.2455395418728890944 ) ) ;
#24519=CARTESIAN_POINT ( 'NONE',  ( 2.985050690391415795, -14.25097394772453718, 0.5935303709388186633 ) ) ;
#24521=CARTESIAN_POINT ( 'NONE',  ( 4.841613500239096979, 117.7629961082686805, 0.9521891642859552363 ) ) ;
#24524=CARTESIAN_POINT ( 'NONE',  ( -2.488979065607898722, -9.142725400274830605, 3.900846118434742493 ) ) ;
#24525=CARTESIAN_POINT ( 'NONE',  ( 16.29178962149223864, 143.9496486471311698, 1.781768755694405071 ) ) ;
#24526=CARTESIAN_POINT ( 'NONE',  ( 2.383384332998917721, 36.54265742952285478, 1.181390620739962483 ) ) ;
#24527=CARTESIAN_POINT ( 'NONE',  ( -2.376338430377652688, 108.4767889311100362, 4.155189222081930644 ) ) ;
#24528=CARTESIAN_POINT ( 'NONE',  ( 4.634220987317881679, -1.855718946426311078, -0.01876340930339078644 ) ) ;
#24529=CARTESIAN_POINT ( 'NONE',  ( 15.78746250177961663, 146.2429432508320417, 0.4439881280938307029 ) ) ;
#24530=CARTESIAN_POINT ( 'NONE',  ( 8.404578209848946102, -5.696077331678487177, -0.5057995593162113446 ) ) ;
#24532=CARTESIAN_POINT ( 'NONE',  ( 2.156385823092337617, 116.5621172156812264, -0.3272761531281138669 ) ) ;
#24533=CARTESIAN_POINT ( 'NONE',  ( 0.01111760956569015496, 120.5507043431653784, -0.5563706444132521245 ) ) ;
#24534=CARTESIAN_POINT ( 'NONE',  ( -3.174366308152013705, 104.6144662015457243, -0.06343139340882732180 ) ) ;
#24536=CARTESIAN_POINT ( 'NONE',  ( -0.02244247360070318262, 39.09286639261657115, 1.286999615499952787 ) ) ;
#24537=AXIS2_PLACEMENT_3D ( 'NONE', #39046, #2649, #9239 ) ;
#24538=CARTESIAN_POINT ( 'NONE',  ( -8.332721659230562850, 3.087680552427906733, 1.359589815967415127 ) ) ;
#24539=CARTESIAN_POINT ( 'NONE',  ( 4.367111786564722209, 117.9394488565217785, 1.183296878226660853 ) ) ;
#24540=DIRECTION ( 'NONE',  ( 5.206863593109713045E-17, -1.000000000000000000, 1.077750396879097359E-30 ) ) ;
#24543=CARTESIAN_POINT ( 'NONE',  ( 0.01635612297673702184, 119.2343925067225427, -0.8185272769044250607 ) ) ;
#24544=CARTESIAN_POINT ( 'NONE',  ( -11.52575769572330344, 118.8226552325407397, 0.2321966025152970570 ) ) ;
#24547=EDGE_CURVE ( 'NONE', #11330, #21134, #38526, .T. ) ;
#24551=CARTESIAN_POINT ( 'NONE',  ( -15.76285804746354380, 145.9067145067653541, -0.3149794173055767699 ) ) ;
#24552=CARTESIAN_POINT ( 'NONE',  ( 2.449088499779481953, -15.60605025760848719, 5.768239595176595458 ) ) ;
#24553=CARTESIAN_POINT ( 'NONE',  ( -13.62782584980156741, 121.9345505566020194, 1.161422094953211470 ) ) ;
#24555=CARTESIAN_POINT ( 'NONE',  ( 17.38882309766589174, 125.1846915036903027, -0.8043053978789252989 ) ) ;
#24556=CARTESIAN_POINT ( 'NONE',  ( 3.465721614298269415, 18.43485028915299750, -3.064284189100199729 ) ) ;
#24557=CARTESIAN_POINT ( 'NONE',  ( -8.196043946343930742, 117.5568930537867800, -0.4237257472399767466 ) ) ;
#24560=CARTESIAN_POINT ( 'NONE',  ( -8.797854266432963755, 117.6962148302091293, -0.06373852044383021553 ) ) ;
#24561=DIRECTION ( 'NONE',  ( -4.017660918040594346E-17, 1.000000000000000000, 2.376309959284834438E-19 ) ) ;
#24562=CARTESIAN_POINT ( 'NONE',  ( -17.79400844405183335, 146.5573550606970628, 1.533700293046251995 ) ) ;
#24563=DIRECTION ( 'NONE',  ( 0.9998004120163608288, 0.000000000000000000, 0.01997839162482760791 ) ) ;
#24564=CARTESIAN_POINT ( 'NONE',  ( 18.05326814683158787, 150.0321773811041339, -1.740468527814021060 ) ) ;
#24565=CARTESIAN_POINT ( 'NONE',  ( -2.141138273642896550, 117.8876587302075194, -0.7126953207602169105 ) ) ;
#24567=CARTESIAN_POINT ( 'NONE',  ( 9.727312926402424509, 123.7664141286412871, -0.5879621312111033005 ) ) ;
#24569=CARTESIAN_POINT ( 'NONE',  ( -18.33584167903968876, 146.8095856830544790, -2.399012226062094300 ) ) ;
#24570=CARTESIAN_POINT ( 'NONE',  ( 4.169050558263453610, -15.30144204372030359, -0.4701337638493395255 ) ) ;
#24571=CARTESIAN_POINT ( 'NONE',  ( -4.467274181827439072, 118.1153900419622431, -0.7451687554449282214 ) ) ;
#24574=CARTESIAN_POINT ( 'NONE',  ( 3.682264917456192777, 82.64346620154573486, 0.07358041635423968885 ) ) ;
#24575=CARTESIAN_POINT ( 'NONE',  ( 11.43271672892777602, 123.4929228318607386, 1.641276387634013290 ) ) ;
#24576=DIRECTION ( 'NONE',  ( 0.9998004120163608288, 0.000000000000000000, 0.01997839162482749342 ) ) ;
#24577=AXIS2_PLACEMENT_3D ( 'NONE', #7422, #4236, #20380 ) ;
#24578=CARTESIAN_POINT ( 'NONE',  ( 5.270772580891830650, -0.5842219557417941411, -6.616342194954959233 ) ) ;
#24579=CARTESIAN_POINT ( 'NONE',  ( 9.304959842724178642, 124.0984330410602183, 0.5077435198050488374 ) ) ;
#24580=CARTESIAN_POINT ( 'NONE',  ( 4.646169936107913401, 117.9325745699973282, -0.7782960047779410306 ) ) ;
#24584=CARTESIAN_POINT ( 'NONE',  ( -1.974101587913926981, 118.1588900521014409, 0.7857444796409881471 ) ) ;
#24586=CARTESIAN_POINT ( 'NONE',  ( -7.844413229920568220, 122.2807544141772524, -0.7395612626406528056 ) ) ;
#24589=CARTESIAN_POINT ( 'NONE',  ( -11.68775717287302740, 118.7263634577040676, -0.08842886322950098410 ) ) ;
#24590=ORIENTED_EDGE ( 'NONE', *, *, #9982, .T. ) ;
#24592=CARTESIAN_POINT ( 'NONE',  ( -7.863154760065894422, 122.1805646130430745, -0.8209280068902528038 ) ) ;
#24593=CARTESIAN_POINT ( 'NONE',  ( -8.131384943450896685, 121.0503350093196815, 0.9968526362124168205 ) ) ;
#24594=ORIENTED_EDGE ( 'NONE', *, *, #17569, .F. ) ;
#24595=CARTESIAN_POINT ( 'NONE',  ( 1.413592544884475721, 118.7629491485454025, -1.196437990151151709 ) ) ;
#24596=CARTESIAN_POINT ( 'NONE',  ( -9.348637138742866171, 124.2740283646700306, -0.4211050520620435722 ) ) ;
#24597=CARTESIAN_POINT ( 'NONE',  ( 2.834973442847717351, -15.21714937722351557, 5.773325752997570781 ) ) ;
#24599=CARTESIAN_POINT ( 'NONE',  ( -20.59913821282573565, 136.3738900553462372, 1.239205967624167792 ) ) ;
#24602=CARTESIAN_POINT ( 'NONE',  ( 1.824897337458711855, 116.5125207362610951, 0.1392185346034943982 ) ) ;
#24604=CARTESIAN_POINT ( 'NONE',  ( 11.83539255247743149, 152.0195595274622349, 0.2364993098673506822 ) ) ;
#24606=CARTESIAN_POINT ( 'NONE',  ( -0.9370761106581132482, 23.39645565634240043, 0.2812775048015344614 ) ) ;
#24607=CARTESIAN_POINT ( 'NONE',  ( -14.83769995734848202, 120.3134675335783754, -0.3991467459773893056 ) ) ;
#24609=ADVANCED_FACE ( 'NONE', ( #30113 ), #13684, .T. ) ;
#24610=VERTEX_POINT ( 'NONE', #10417 ) ;
#24611=CARTESIAN_POINT ( 'NONE',  ( 3.194789458502170110, 117.5549192558606251, 0.8028907591355466389 ) ) ;
#24613=CARTESIAN_POINT ( 'NONE',  ( 17.48314440517386359, 153.9260871938423065, 1.866247694559708403 ) ) ;
#24615=CARTESIAN_POINT ( 'NONE',  ( 8.948346978250095063, 119.7003323559047061, -1.088312767383050605 ) ) ;
#24616=CARTESIAN_POINT ( 'NONE',  ( 7.043328640077428204, 23.89357186360551566, -4.653114003055315528 ) ) ;
#24617=CARTESIAN_POINT ( 'NONE',  ( -1.305078825605850312, 159.4185946040361728, -0.8784184817623136299 ) ) ;
#24618=CARTESIAN_POINT ( 'NONE',  ( 4.775642591496352729, 117.6653311871567382, -0.9390539395389304600 ) ) ;
#24619=CARTESIAN_POINT ( 'NONE',  ( 0.1506203121292604419, 105.8833743670705445, 5.338473058816376238 ) ) ;
#24620=ORIENTED_EDGE ( 'NONE', *, *, #29465, .F. ) ;
#24621=CARTESIAN_POINT ( 'NONE',  ( -11.25890738108754263, 128.1602342495223468, 0.05278459517150006775 ) ) ;
#24622=CARTESIAN_POINT ( 'NONE',  ( -13.39306239354274197, 123.7870877700634509, -1.917211633051635333 ) ) ;
#24624=CARTESIAN_POINT ( 'NONE',  ( 4.954452526664399059, -15.13560178954495505, 4.019779494548574306 ) ) ;
#24626=CARTESIAN_POINT ( 'NONE',  ( -3.960243126016221193, 117.9496055611373748, -1.231645824533994960 ) ) ;
#24628=CARTESIAN_POINT ( 'NONE',  ( 10.36135117696309571, 155.6679353847891321, 2.160796112024522486 ) ) ;
#24630=CARTESIAN_POINT ( 'NONE',  ( -5.319749943626951527, 115.6909491485453003, 0.5104040631377158022 ) ) ;
#24632=CARTESIAN_POINT ( 'NONE',  ( -2.311559032574000749, 118.7862729053988318, 0.6846880608948529012 ) ) ;
#24633=CARTESIAN_POINT ( 'NONE',  ( -4.887076909682236625, -2.444604220856811505, -6.895871986673536291 ) ) ;
#24634=CARTESIAN_POINT ( 'NONE',  ( 4.540840819607053547, 155.9125706774115940, 0.9348598387858672032 ) ) ;
#24636=CARTESIAN_POINT ( 'NONE',  ( 21.54968253652544519, 151.3526640061693342, -0.5241015958777708317 ) ) ;
#24639=CARTESIAN_POINT ( 'NONE',  ( -4.469853575504566301, 31.48943071249222214, -0.6923489671027511783 ) ) ;
#24640=FACE_OUTER_BOUND ( 'NONE', #21562, .T. ) ;
#24641=CARTESIAN_POINT ( 'NONE',  ( -4.303542067741650712, 118.2142174830580359, 0.3397717045260155166 ) ) ;
#24646=ADVANCED_FACE ( 'NONE', ( #29807 ), #39829, .T. ) ;
#24647=CARTESIAN_POINT ( 'NONE',  ( -4.295590839325457821, 119.4259349426024386, -0.9270884132243183418 ) ) ;
#24648=CARTESIAN_POINT ( 'NONE',  ( -5.306918775014303868, 116.0444662015457169, 1.063204892635948307 ) ) ;
#24649=CARTESIAN_POINT ( 'NONE',  ( 4.266316740665818230, 118.2131443819900198, 0.5314761920156354513 ) ) ;
#24650=CARTESIAN_POINT ( 'NONE',  ( -13.85976170726116585, 150.2454140652271803, -1.103110692033625995 ) ) ;
#24651=FACE_OUTER_BOUND ( 'NONE', #18080, .T. ) ;
#24653=ADVANCED_FACE ( 'NONE', ( #40040 ), #29140, .T. ) ;
#24654=ORIENTED_EDGE ( 'NONE', *, *, #2459, .T. ) ;
#24655=CARTESIAN_POINT ( 'NONE',  ( -0.6244342276652131707, 19.93415720681881353, -4.586363120317934694 ) ) ;
#24660=CARTESIAN_POINT ( 'NONE',  ( -6.063368700931957456, 121.4421655836107163, -0.07279211641118281395 ) ) ;
#24661=CARTESIAN_POINT ( 'NONE',  ( -4.596079559025361583, 18.26954911218466648, 0.4757704999388879807 ) ) ;
#24662=CARTESIAN_POINT ( 'NONE',  ( 4.831157780893915010, 117.2114307359545649, 0.6331281246675558583 ) ) ;
#24663=DIRECTION ( 'NONE',  ( -4.017660918040594346E-17, 1.000000000000000000, 2.376309959284834438E-19 ) ) ;
#24664=CARTESIAN_POINT ( 'NONE',  ( 2.931439949929583122, -14.82325452411255640, 4.117531814738872420 ) ) ;
#24665=CARTESIAN_POINT ( 'NONE',  ( 0.4156903444692294225, 117.7785671674745771, -0.5149838300002415048 ) ) ;
#24666=CARTESIAN_POINT ( 'NONE',  ( -14.54156464587795661, 128.5519869857110393, 1.481139062272948337 ) ) ;
#24667=CARTESIAN_POINT ( 'NONE',  ( 2.233585966345281282, 24.54162662436292308, -4.064490141941544898 ) ) ;
#24668=CARTESIAN_POINT ( 'NONE',  ( -20.39753840605640178, 152.5480347002736607, -1.233721349276552637 ) ) ;
#24669=AXIS2_PLACEMENT_3D ( 'NONE', #38764, #20348, #4204 ) ;
#24670=CARTESIAN_POINT ( 'NONE',  ( 0.6786060095046909657, 20.86726683125115756, 0.6988831909418605770 ) ) ;
#24673=CARTESIAN_POINT ( 'NONE',  ( -15.60301224545410825, 143.6313904367523833, 0.5515178422673751024 ) ) ;
#24674=CARTESIAN_POINT ( 'NONE',  ( 2.652408316642993480, -15.27006336626107696, 5.836003982494253783 ) ) ;
#24675=CARTESIAN_POINT ( 'NONE',  ( 17.21539028065161148, 147.4900653055648547, -1.363477025422524802 ) ) ;
#24677=CARTESIAN_POINT ( 'NONE',  ( 0.8957990821136506687, 115.7029491485453150, 1.751259771659311237 ) ) ;
#24680=CARTESIAN_POINT ( 'NONE',  ( 3.301452709780442252, -13.00349394711965090, 1.536261971075179478 ) ) ;
#24681=CARTESIAN_POINT ( 'NONE',  ( -4.734399331529842492, 117.8958854344520262, -0.9305720750720559709 ) ) ;
#24682=CARTESIAN_POINT ( 'NONE',  ( 11.85733017202526440, 130.3381101163291760, 0.1934038552275229028 ) ) ;
#24685=CARTESIAN_POINT ( 'NONE',  ( 12.98660267081546138, 122.0079276396459704, 1.762897954238471954 ) ) ;
#24688=CARTESIAN_POINT ( 'NONE',  ( 0.02969037535068572500, 158.7301711276701894, -1.485827791648137053 ) ) ;
#24689=CARTESIAN_POINT ( 'NONE',  ( 23.39020171064277065, 146.7932648766621639, 0.1331748977937668443 ) ) ;
#24693=CARTESIAN_POINT ( 'NONE',  ( 1.924448629921342357, -15.15080081298969539, 5.916077864091418448 ) ) ;
#24694=DIRECTION ( 'NONE',  ( 0.9998004120163609398, 4.016384292689130894E-17, 0.01997839162482749689 ) ) ;
#24696=CARTESIAN_POINT ( 'NONE',  ( -4.811373471701494431, 117.8747111989650875, 0.6665432265399071632 ) ) ;
#24700=CARTESIAN_POINT ( 'NONE',  ( 5.810495312042946559, 118.7618932863102401, -1.004714121124453241 ) ) ;
#24701=CARTESIAN_POINT ( 'NONE',  ( -3.839037681459759987, 115.3331674797404247, -1.733041430519539183 ) ) ;
#24702=CARTESIAN_POINT ( 'NONE',  ( 4.916126448754050138, 117.5420021306158418, 1.049297650600119258 ) ) ;
#24704=CARTESIAN_POINT ( 'NONE',  ( -1.052442600544543749, 124.5996987749017109, 0.008430925479885411494 ) ) ;
#24705=AXIS2_PLACEMENT_3D ( 'NONE', #38847, #39270, #22416 ) ;
#24706=CARTESIAN_POINT ( 'NONE',  ( -0.2095918955067871126, -8.989892990265463624, -4.636818132431064221 ) ) ;
#24709=CARTESIAN_POINT ( 'NONE',  ( 2.175557056806384448, -14.94057515128023539, 5.440454282391695706 ) ) ;
#24710=CARTESIAN_POINT ( 'NONE',  ( 4.883585300477370161, 117.2937442104795593, -0.7242188414070881430 ) ) ;
#24714=CARTESIAN_POINT ( 'NONE',  ( -1.749991611943370051, 115.7029018373826545, 1.658182375568262312 ) ) ;
#24715=CARTESIAN_POINT ( 'NONE',  ( 2.267534764145236803, 6.115564135048844108, 4.037922524061999141 ) ) ;
#24716=CARTESIAN_POINT ( 'NONE',  ( 22.69296959717475559, 150.3666470947781022, 1.044501570340798713 ) ) ;
#24718=CARTESIAN_POINT ( 'NONE',  ( -0.1040029800483648487, 104.6144662015455964, -4.835167297233627259 ) ) ;
#24719=CARTESIAN_POINT ( 'NONE',  ( 2.909835405328949687, -15.65209430229147536, 4.668939894544173796 ) ) ;
#24720=CARTESIAN_POINT ( 'NONE',  ( -8.613587046216272469, 156.7723266660784986, 1.729508645372233255 ) ) ;
#24721=CARTESIAN_POINT ( 'NONE',  ( -0.4796499176084361160, 15.67505972103439049, -0.8497018901732851237 ) ) ;
#24722=CARTESIAN_POINT ( 'NONE',  ( -0.4212773433310383342, 21.23346528477927819, -0.8800754956890687319 ) ) ;
#24727=CARTESIAN_POINT ( 'NONE',  ( 1.549819036667637873, 118.0223913815010377, 1.039293717761402558 ) ) ;
#24729=CARTESIAN_POINT ( 'NONE',  ( -2.625396581831559661, 120.2926465633240127, 0.4415429531236471083 ) ) ;
#24731=CARTESIAN_POINT ( 'NONE',  ( 1.889397806843069905, -15.09730794468430659, 5.542604807410119072 ) ) ;
#24732=CARTESIAN_POINT ( 'NONE',  ( 16.17691485933963946, 135.1141785778430346, -1.596016904437364659 ) ) ;
#24734=CARTESIAN_POINT ( 'NONE',  ( -20.36154792711273842, 148.1475078817917961, -2.480623434655589765 ) ) ;
#24736=CARTESIAN_POINT ( 'NONE',  ( -1.386537629721184883, 36.36735770096321829, 2.585368322340787284 ) ) ;
#24737=CARTESIAN_POINT ( 'NONE',  ( 8.684730043605602745, 123.3259068333282755, -0.1300027459630655191 ) ) ;
#24738=ORIENTED_EDGE ( 'NONE', *, *, #24238, .F. ) ;
#24739=CARTESIAN_POINT ( 'NONE',  ( 2.971193505762239617, -14.05637172046637851, 0.8995351626913862253 ) ) ;
#24740=CARTESIAN_POINT ( 'NONE',  ( -3.958300029084214522, 28.23836431654049761, 1.224951011016432556 ) ) ;
#24743=CARTESIAN_POINT ( 'NONE',  ( -3.029891238501105644, -9.367638731076009861, 3.490193963561483148 ) ) ;
#24744=CARTESIAN_POINT ( 'NONE',  ( 6.507413728077992232, 121.1369950346570192, 0.8796459533030992484 ) ) ;
#24745=CARTESIAN_POINT ( 'NONE',  ( -2.854324211611072304, 29.11572452856798776, 0.7926346486988061768 ) ) ;
#24746=CARTESIAN_POINT ( 'NONE',  ( -6.089625701343511111, 119.5347744825833871, 0.2725575997743532874 ) ) ;
#24749=CARTESIAN_POINT ( 'NONE',  ( -4.399545650080316506, 2.442302885307133131, -1.471791394725967095 ) ) ;
#24750=CARTESIAN_POINT ( 'NONE',  ( 11.03183784343224616, 128.0124916018596650, 0.2204423744267036411 ) ) ;
#24752=CARTESIAN_POINT ( 'NONE',  ( 6.742867120194277142, -6.769607736128188336, 5.057590804256700601 ) ) ;
#24754=CARTESIAN_POINT ( 'NONE',  ( -2.144839993658618216, 116.4227009531578858, -0.3427478915012472371 ) ) ;
#24755=CARTESIAN_POINT ( 'NONE',  ( 0.06282972276528790700, 111.5577547982949227, -3.144256248693278355 ) ) ;
#24757=CARTESIAN_POINT ( 'NONE',  ( -2.958531772299362039, 50.42904571186020490, -1.329372033065077341 ) ) ;
#24758=CARTESIAN_POINT ( 'NONE',  ( -7.483757832938788823, -7.479835662595867518, -3.861840502031824940 ) ) ;
#24759=CARTESIAN_POINT ( 'NONE',  ( 0.3864482072712463467, 117.9394481662412062, 1.409681420816396580 ) ) ;
#24763=CARTESIAN_POINT ( 'NONE',  ( 0.9884870862448961182, 123.5966405200008325, -0.1018174175105950180 ) ) ;
#24764=CARTESIAN_POINT ( 'NONE',  ( -2.843964318557778981, 116.7549172960530939, 0.2381273168889447012 ) ) ;
#24769=CARTESIAN_POINT ( 'NONE',  ( -15.64207015331068185, 147.2204672151589193, -0.3125657877211906466 ) ) ;
#24770=CARTESIAN_POINT ( 'NONE',  ( 6.422280156622033331, -13.89829431882434818, 0.3667318345078443564 ) ) ;
#24771=CARTESIAN_POINT ( 'NONE',  ( -14.84487292597024499, 154.6636077862465015, 1.582666667450879805 ) ) ;
#24772=CARTESIAN_POINT ( 'NONE',  ( 16.02745508617892867, 155.1095016151506911, -1.019363059911538638 ) ) ;
#24773=CARTESIAN_POINT ( 'NONE',  ( -4.598301960400187127, 22.30806413504685537, 0.5496829067130363233 ) ) ;
#24774=CARTESIAN_POINT ( 'NONE',  ( -16.76609992697674301, 155.2615993841311877, -0.7433399007605485664 ) ) ;
#24778=CARTESIAN_POINT ( 'NONE',  ( -2.183037072706512483, 116.1872911837574947, -0.04021945895725198561 ) ) ;
#24779=CYLINDRICAL_SURFACE ( 'NONE', #14790, 3.175000000000001155 ) ;
#24780=CARTESIAN_POINT ( 'NONE',  ( -11.33340168069295650, 123.5700555580090594, 1.145074488444943528 ) ) ;
#24782=CARTESIAN_POINT ( 'NONE',  ( 19.06441997122210452, 145.0145856610025987, -1.755053680361626345 ) ) ;
#24783=CARTESIAN_POINT ( 'NONE',  ( -14.96081243412116990, 123.1914926142276130, -1.724312424550131562 ) ) ;
#24785=CARTESIAN_POINT ( 'NONE',  ( 16.31827467517370422, 146.7930872653447523, -0.7884962901916309219 ) ) ;
#24786=EDGE_CURVE ( 'NONE', #3481, #18999, #39060, .T. ) ;
#24787=EDGE_LOOP ( 'NONE', ( #25421, #27210, #34696, #32747 ) ) ;
#24788=CARTESIAN_POINT ( 'NONE',  ( -5.440231158483335605, 156.5946142756450570, -1.801097700867929419 ) ) ;
#24789=CARTESIAN_POINT ( 'NONE',  ( 3.946041497568072653, -15.66665589675640646, 3.498282510246776500 ) ) ;
#24790=CARTESIAN_POINT ( 'NONE',  ( -4.105086577347437427, 118.2429491485453070, -0.3532857226942683893 ) ) ;
#24791=ADVANCED_FACE ( 'NONE', ( #27029 ), #10832, .T. ) ;
#24795=CARTESIAN_POINT ( 'NONE',  ( 7.267393677827311826, 155.8804291298944236, 1.807016794997827747 ) ) ;
#24797=( BOUNDED_CURVE ( )  B_SPLINE_CURVE ( 3, ( #11871, #40852, #21642, #24639 ),
 .UNSPECIFIED., .F., .T. ) 
 B_SPLINE_CURVE_WITH_KNOTS ( ( 4, 4 ),
 ( 0.0002600131435865652915, 0.01144530851284875084 ),
 .UNSPECIFIED. ) 
 CURVE ( )  GEOMETRIC_REPRESENTATION_ITEM ( )  RATIONAL_B_SPLINE_CURVE ( ( 0.9989604882768124972, 0.9840622721794859418, 0.9694976849687608755, 0.9552667266446374095 ) ) 
 REPRESENTATION_ITEM ( '' )  );
#24799=CARTESIAN_POINT ( 'NONE',  ( 0.6763034141103227981, -4.228338640871131204, 8.424193199533098309 ) ) ;
#24800=CARTESIAN_POINT ( 'NONE',  ( 9.106360905785095383, 123.9337093609977529, 0.4112724569044294842 ) ) ;
#24801=CARTESIAN_POINT ( 'NONE',  ( 4.801298557440690118, 117.4006788788929896, -1.015947269269607656 ) ) ;
#24802=B_SPLINE_CURVE_WITH_KNOTS ( 'NONE', 3,
 ( #1674, #1044, #37228, #36610, #7638, #10606 ),
 .UNSPECIFIED., .F., .F.,
 ( 4, 2, 4 ),
 ( 0.000000000000000000, 0.0001552906547695077498, 0.0003105813095390154996 ),
 .UNSPECIFIED. ) ;
#24806=CARTESIAN_POINT ( 'NONE',  ( -7.805875142760556606, 122.5029850928241615, -0.4967190073759077951 ) ) ;
#24809=CARTESIAN_POINT ( 'NONE',  ( -10.80084657379841495, 157.9251727141802633, -0.03745751586626412666 ) ) ;
#24812=CARTESIAN_POINT ( 'NONE',  ( -6.854099372262661305, 121.6001605170599618, -0.7074379530687137096 ) ) ;
#24813=CARTESIAN_POINT ( 'NONE',  ( -8.378245210821358313, 119.8566484287661353, 1.107698278211572740 ) ) ;
#24814=VERTEX_POINT ( 'NONE', #31470 ) ;
#24815=CARTESIAN_POINT ( 'NONE',  ( 0.4316031730808821409, 115.7034384546826686, -1.748259241455569546 ) ) ;
#24816=CARTESIAN_POINT ( 'NONE',  ( -1.593749994916005885, 120.9451058151398399, -0.1271097986196581264 ) ) ;
#24817=CARTESIAN_POINT ( 'NONE',  ( 4.653081906828674619, -14.28787889440780212, 4.403751634497075074 ) ) ;
#24818=CARTESIAN_POINT ( 'NONE',  ( -9.329873057606407727, 118.8811571165754941, 0.8296725728930307575 ) ) ;
#24820=CARTESIAN_POINT ( 'NONE',  ( -0.001640166039863760056, 159.6041700698465036, 0.08208061555506501739 ) ) ;
#24821=CARTESIAN_POINT ( 'NONE',  ( 15.72247783716871083, 145.6852940966224708, 0.3814333285848034438 ) ) ;
#24823=CARTESIAN_POINT ( 'NONE',  ( 0.9754839647580387796, 27.70931421350951496, 0.02445524045744520980 ) ) ;
#24824=CARTESIAN_POINT ( 'NONE',  ( -21.64466742782801845, 132.7051459832101443, -0.4972030839502442068 ) ) ;
#24825=CARTESIAN_POINT ( 'NONE',  ( -6.426369768295692736E-14, 159.6054662015457382, 1.032716915552223178E-16 ) ) ;
#24829=CARTESIAN_POINT ( 'NONE',  ( -5.745771690987640845, 118.0751039679726659, 0.8607859349433016893 ) ) ;
#24830=CARTESIAN_POINT ( 'NONE',  ( 4.543739712435177047, -15.19060223592207137, -0.8445694877862246486 ) ) ;
#24831=CARTESIAN_POINT ( 'NONE',  ( 5.844042411599751574, 117.9059190437751141, 0.9510131463654533102 ) ) ;
#24833=CARTESIAN_POINT ( 'NONE',  ( 13.21705611421139359, 122.1656469061080514, -1.250183119358982742 ) ) ;
#24834=CARTESIAN_POINT ( 'NONE',  ( 2.538140519494355374, 21.06397054095828381, 8.048466014368985455 ) ) ;
#24835=CARTESIAN_POINT ( 'NONE',  ( -15.93415399606969096, 122.8751182158008959, -1.397711951582541801 ) ) ;
#24836=CARTESIAN_POINT ( 'NONE',  ( 4.783731562129573511, 117.6342719419094323, -0.9515537801535082219 ) ) ;
#24837=CARTESIAN_POINT ( 'NONE',  ( 5.263686092533300886, 116.7134249176580028, 1.019678336081760506 ) ) ;
#24840=CARTESIAN_POINT ( 'NONE',  ( -9.614588335866276481, 124.8310256250372277, -0.1039111448415539068 ) ) ;
#24841=CARTESIAN_POINT ( 'NONE',  ( -12.24350972434462115, 123.0735437985678971, -1.806721486477698368 ) ) ;
#24842=CARTESIAN_POINT ( 'NONE',  ( 4.975685353906630581, -15.32372399918348371, 3.685287151418908724 ) ) ;
#24845=CARTESIAN_POINT ( 'NONE',  ( -1.067625512720145942, 118.1651004991311851, -0.8760196487506567431 ) ) ;
#24846=ORIENTED_EDGE ( 'NONE', *, *, #19130, .T. ) ;
#24847=B_SPLINE_SURFACE_WITH_KNOTS ( 'NONE', 5, 5, ( 
 ( #17229, #1064, #14031, #24037, #27036, #37052 ),
 ( #28496, #34900, #24448, #11457, #34686, #9124 ),
 ( #5515, #8908, #24660, #21874, #27655, #37452 ),
 ( #38093, #22085, #18056, #18473, #5105, #2323 ),
 ( #24879, #5732, #37669, #18261, #18685, #37876 ),
 ( #27864, #31478, #38303, #31060, #31694, #40666 ),
 ( #21661, #1898, #41295, #35112, #40872, #11890 ),
 ( #15498, #2537, #14860, #8276, #8698, #41506 ),
 ( #12312, #25300, #5938, #21246, #34276, #15283 ),
 ( #30851, #28287, #1695, #8492, #14651, #11673 ),
 ( #21449, #34478, #12098, #5311, #31265, #25086 ),
 ( #2107, #15071, #28071, #41082, #9947, #36165 ),
 ( #23128, #41925, #35951, #32752, #10157, #18898 ),
 ( #42137, #28705, #6551, #25715, #29337, #16116 ),
 ( #15910, #35739, #22499, #15700, #9742, #22710 ),
 ( #19318, #2744, #178, #29119, #9328, #19526 ),
 ( #12933, #3586, #35527, #9530, #31907, #32533 ),
 ( #6348, #32323, #41714, #12520, #26348, #13358 ),
 ( #6763, #32115, #3152, #6143, #38511, #3364 ),
 ( #19108, #39142, #13148, #2946, #28910, #25511 ),
 ( #22290, #22920, #391, #19731, #16331, #35315 ),
 ( #25923, #12726, #26141, #38721, #38931, #16547 ),
 ( #29557, #39354, #23771, #27404, #39788, #29966 ),
 ( #29764, #40414, #33600, #33809, #601, #13574 ),
 ( #17391, #26563, #10583, #40208, #24194, #23985 ),
 ( #806, #37004, #20785, #11210, #6982, #20574 ),
 ( #16757, #36794, #13782, #30381, #4219, #1233 ),
 ( #7612, #23561, #3796, #40000, #10791, #36583 ),
 ( #32971, #14190, #17180, #39570, #4433, #19953 ),
 ( #4637, #7399, #20362, #10375, #27194, #17594 ),
 ( #33385, #23344, #36383, #14396, #1435, #26778 ),
 ( #7199, #20157, #33181, #4009, #11006, #16966 ),
 ( #30179, #1020, #13984, #26989, #7823, #30597 ),
 ( #20996, #40617, #34226, #25040, #37618, #8651 ),
 ( #41245, #15240, #8442, #21825, #21400, #2276 ),
 ( #40825, #11416, #31434, #21612, #11624, #24402 ),
 ( #5055, #34854, #38043, #34428, #5686, #18644 ),
 ( #37408, #5467, #15452, #18011, #18214, #28454 ),
 ( #8863, #8227, #30799, #31215, #31650, #2490 ),
 ( #41460, #12050, #21200, #5261, #31008, #14603 ),
 ( #27608, #1850, #28241, #12267, #14814, #27816 ),
 ( #17802, #2059, #34021, #24611, #15023, #37204 ),
 ( #34639, #28023, #8025, #4846, #41033, #1648 ),
 ( #11842, #24829, #37824, #18426, #19482, #38885 ),
 ( #28660, #6099, #22248, #22873, #13100, #25674 ),
 ( #35911, #2698, #29290, #35480, #16286, #26091 ),
 ( #35274, #19061, #9487, #19688, #41672, #6720 ),
 ( #9078, #32068, #39098, #2904, #25256, #12890 ),
 ( #12684, #19275, #38681, #22663, #32491, #42095 ),
 ( #15867, #28873, #25474, #3319, #25878, #15656 ),
 ( #35696, #9901, #22452, #38470, #29076, #133 ),
 ( #6303, #32705, #32283, #9288, #3112, #6507 ),
 ( #3539, #41886, #9696, #35072, #16072, #16500 ),
 ( #29507, #346, #38261, #22043, #5893, #18854 ),
 ( #12480, #31859, #19905, #20110, #23723, #16709 ),
 ( #7563, #13313, #29712, #39523, #33132, #23297 ),
 ( #10949, #10742, #39948, #26937, #972, #36741 ),
 ( #7775, #23507, #7353, #13737, #20523, #33553 ),
 ( #33763, #3962, #36334, #13529, #4385, #13939 ),
 ( #20738, #17343, #14142, #26731, #26516, #17131 ),
 ( #16923, #10327, #761, #40157, #20312, #7150 ),
 ( #4588, #17547, #30332, #36534, #23086, #1179 ),
 ( #27145, #10538, #23937, #29923, #30133, #39739 ),
 ( #4169, #36954, #33339, #30548, #39308, #26299 ),
 ( #10115, #36120, #6934, #554, #32920, #3751 ),
 ( #14764, #41195, #40985, #27975, #14974, #31170 ),
 ( #11161, #37992, #11574, #15187, #27353, #8816 ),
 ( #40366, #34591, #1387, #27766, #40777, #5003 ),
 ( #24560, #21775, #24146, #8391, #37155, #4798 ),
 ( #31384, #1803, #11787, #37564, #5420, #21563 ),
 ( #28190, #21353, #8600, #18375, #17962, #17749 ),
 ( #2226, #34379, #5213, #40572, #18167, #34801 ),
 ( #11999, #7977, #24778, #2011, #30749, #37775 ),
 ( #11369, #24992, #5635, #18593, #14343, #1599 ) ),
 .UNSPECIFIED., .F., .F., .F.,
 ( 6, 4, 4, 4, 4, 4, 4, 4, 4, 4, 4, 4, 4, 4, 4, 4, 4, 4, 6 ),
 ( 6, 6 ),
 ( 0.000000000000000000, 0.01562500000000000000, 0.03125000000000000000, 0.06250000000000000000, 0.1250000000000000000, 0.2500000000000000000, 0.3750000000000000000, 0.4375000000000000000, 0.5000000000000000000, 0.5625000000000000000, 0.6250000000000000000, 0.7500000000000000000, 0.8125000000000000000, 0.8750000000000000000, 0.9062500000000000000, 0.9375000000000000000, 0.9687500000000000000, 0.9843750000000000000, 1.000000000000000000 ),
 ( 0.000000000000000000, 1.000000000000000000 ),
 .UNSPECIFIED. ) ;
#24848=CARTESIAN_POINT ( 'NONE',  ( 18.91839881582108518, 147.5601278813269914, 2.482394308196493871 ) ) ;
#24850=EDGE_CURVE ( 'NONE', #929, #10361, #34013, .T. ) ;
#24851=CARTESIAN_POINT ( 'NONE',  ( -1.914222150921244481, 118.1238929887923632, -0.9376219136777126373 ) ) ;
#24852=CARTESIAN_POINT ( 'NONE',  ( -0.6988325576871788902, 114.3327162918516962, 2.155465965906840253 ) ) ;
#24853=EDGE_CURVE ( 'NONE', #9260, #18326, #12090, .T. ) ;
#24854=CARTESIAN_POINT ( 'NONE',  ( -5.887876509958990923, -9.367530720701759961, 6.022233148990229878 ) ) ;
#24855=CARTESIAN_POINT ( 'NONE',  ( 3.128511139047426060, 156.1781389015385457, 0.8559903927114133060 ) ) ;
#24858=CARTESIAN_POINT ( 'NONE',  ( 13.10540794497621597, 156.9444350391594014, -0.5617278846626184707 ) ) ;
#24863=CARTESIAN_POINT ( 'NONE',  ( -4.269227857241942203, 118.2238376706496439, 0.2888421812383961118 ) ) ;
#24864=CARTESIAN_POINT ( 'NONE',  ( 4.797736281515663670, 114.9758604107369138, -1.576599161239440772 ) ) ;
#24867=CARTESIAN_POINT ( 'NONE',  ( 6.307464644398110387, 119.8761965894848771, -0.9734222780920257501 ) ) ;
#24868=CARTESIAN_POINT ( 'NONE',  ( -0.1561264326628848120, 116.0444662015457027, 6.158975241439932802 ) ) ;
#24869=CARTESIAN_POINT ( 'NONE',  ( 4.246284764148858137, 118.2248568323353481, 0.4675053700615026120 ) ) ;
#24870=CARTESIAN_POINT ( 'NONE',  ( -8.892178686620095363, 123.2307073318660855, -0.7481024605839378117 ) ) ;
#24872=CARTESIAN_POINT ( 'NONE',  ( 0.2348404565736222915, 117.9496055676323749, -1.400524049365383439 ) ) ;
#24874=CARTESIAN_POINT ( 'NONE',  ( 1.790774717077139089, 25.13178105314743860, 4.274281468382033822 ) ) ;
#24879=CARTESIAN_POINT ( 'NONE',  ( -7.788904331612559240, 122.6147083454303726, -0.08148215068823494445 ) ) ;
#24880=CARTESIAN_POINT ( 'NONE',  ( 1.653223041919489544, 21.06826514481450729, 4.324967054831568625 ) ) ;
#24881=CARTESIAN_POINT ( 'NONE',  ( 7.741078003750540226, 158.6130819278358501, 0.9685178112996220001 ) ) ;
#24882=CARTESIAN_POINT ( 'NONE',  ( -3.260048740554739588, 104.6144662015456674, -3.571460647889730389 ) ) ;
#24883=CARTESIAN_POINT ( 'NONE',  ( 2.755019269514601632, -14.09852029293599784, -0.1464032776252038315 ) ) ;
#24884=CARTESIAN_POINT ( 'NONE',  ( 9.191685830660368595, 119.1751624949753534, -0.9473905404949717335 ) ) ;
#24885=CARTESIAN_POINT ( 'NONE',  ( -18.09605103972953799, 148.5173242358814321, 1.660853775707743507 ) ) ;
#24886=CARTESIAN_POINT ( 'NONE',  ( 3.707542801486926276, 23.89195667223011910, -2.776928957275885068 ) ) ;
#24887=CARTESIAN_POINT ( 'NONE',  ( -14.96245403159076837, 120.9606250904355704, -1.059951836595168118 ) ) ;
#24888=CARTESIAN_POINT ( 'NONE',  ( -0.08600706866453224075, 15.02498995931601122, -0.9728917428382349852 ) ) ;
#24891=CARTESIAN_POINT ( 'NONE',  ( -9.339416610757488968, 123.9819092696984910, 0.2335442159362874082 ) ) ;
#24892=CARTESIAN_POINT ( 'NONE',  ( 4.653081906828674619, -14.28787889440780212, 4.403751634497075074 ) ) ;
#24893=CARTESIAN_POINT ( 'NONE',  ( 15.52878352361680214, 139.6011575924185877, -1.142358493343923920 ) ) ;
#24895=CARTESIAN_POINT ( 'NONE',  ( 0.6068092274946489395, 115.7030931646781511, 1.759830564766369232 ) ) ;
#24896=ORIENTED_EDGE ( 'NONE', *, *, #42049, .T. ) ;
#24897=CARTESIAN_POINT ( 'NONE',  ( -4.811659653300878858, 117.7644762915747378, -1.004442067184477594 ) ) ;
#24898=CARTESIAN_POINT ( 'NONE',  ( 6.500720044509773921, 121.7799842514348541, 0.1008652220075046541 ) ) ;
#24900=CARTESIAN_POINT ( 'NONE',  ( 12.64856329662753076, 122.0451665396574725, 1.778165442619766834 ) ) ;
#24902=PLANE ( 'NONE',  #28634 ) ;
#24904=CARTESIAN_POINT ( 'NONE',  ( 0.01887972822138463125, 159.3676309965788960, -0.9448188026860500077 ) ) ;
#24905=CARTESIAN_POINT ( 'NONE',  ( 6.916478980584438219, 117.2343425291504104, -0.1085122952249094053 ) ) ;
#24907=CARTESIAN_POINT ( 'NONE',  ( 1.668644623944747662, -15.26291410520330771, 5.716625384245738850 ) ) ;
#24910=AXIS2_PLACEMENT_3D ( 'NONE', #21448, #8697, #41081 ) ;
#24911=CARTESIAN_POINT ( 'NONE',  ( -4.732672620930323149, 117.8972391386454319, 0.7793045165695084986 ) ) ;
#24913=ORIENTED_EDGE ( 'NONE', *, *, #41725, .F. ) ;
#24917=CARTESIAN_POINT ( 'NONE',  ( 8.556114498411417912, 118.9718870934816692, -0.9297341161968202261 ) ) ;
#24918=CARTESIAN_POINT ( 'NONE',  ( -3.975629016402025151, 111.5999093057820772, -3.028662833142258037 ) ) ;
#24919=CARTESIAN_POINT ( 'NONE',  ( 4.956589549431869912, 117.4692179202435938, 0.9991419478834157042 ) ) ;
#24920=CARTESIAN_POINT ( 'NONE',  ( 6.475684456959278634, -13.49251406434824574, 0.1304084665236045215 ) ) ;
#24921=CARTESIAN_POINT ( 'NONE',  ( -0.9126123168629748372, 122.5862318000603182, 0.2067773319678724020 ) ) ;
#24922=CARTESIAN_POINT ( 'NONE',  ( -1.825063964020108065, -4.879331645356781877, 4.256838567046823840 ) ) ;
#24923=CARTESIAN_POINT ( 'NONE',  ( -4.855072294470597072, 115.7029491485453718, 1.279409886141102071 ) ) ;
#24924=LINE ( 'NONE', #5562, #32157 ) ;
#24925=CARTESIAN_POINT ( 'NONE',  ( 2.715028358135622266, -14.64271907847003362, 5.065740987199049528 ) ) ;
#24926=CARTESIAN_POINT ( 'NONE',  ( 6.983131083342589029, 124.7321584522365896, 0.1385298619991069402 ) ) ;
#24927=CARTESIAN_POINT ( 'NONE',  ( -17.31991401741520775, 147.8988302317391117, -2.155506138210265821 ) ) ;
#24928=CARTESIAN_POINT ( 'NONE',  ( 5.155022408837186987, 116.8361691014224277, 0.02608676839127775648 ) ) ;
#24930=CARTESIAN_POINT ( 'NONE',  ( -1.835695816207170594, 115.7029480714724627, 1.651914411509646241 ) ) ;
#24931=CARTESIAN_POINT ( 'NONE',  ( 3.263621351691376571, 8.939281053574255509, -3.290156819607050753 ) ) ;
#24932=CARTESIAN_POINT ( 'NONE',  ( 15.04006788896544222, 156.1474796653986630, 0.8176042244810640680 ) ) ;
#24934=CARTESIAN_POINT ( 'NONE',  ( -1.150111429288084519, 105.1233927192594564, -5.219387141699733057 ) ) ;
#24935=CARTESIAN_POINT ( 'NONE',  ( 4.184971198371238543, -15.30562903706386635, -0.2021278847381603183 ) ) ;
#24936=CARTESIAN_POINT ( 'NONE',  ( -16.79779972313721359, 131.5287050380659082, 1.642352026799754672 ) ) ;
#24937=CARTESIAN_POINT ( 'NONE',  ( 0.8610934044332675397, -11.37225059697985863, 0.4573394443077089533 ) ) ;
#24938=CARTESIAN_POINT ( 'NONE',  ( 0.05241920358452190065, 15.83596528477922405, 0.9742995972537078497 ) ) ;
#24939=ORIENTED_EDGE ( 'NONE', *, *, #39977, .T. ) ;
#24942=CARTESIAN_POINT ( 'NONE',  ( 1.569662112149277977, 118.6366899268033279, 0.8670489899392762601 ) ) ;
#24943=CARTESIAN_POINT ( 'NONE',  ( -14.29925251870378489, 150.3563008155378213, 0.9573768768026652554 ) ) ;
#24944=DIRECTION ( 'NONE',  ( -5.206863593109713661E-17, 1.000000000000000000, -1.077750396879097183E-30 ) ) ;
#24945=CARTESIAN_POINT ( 'NONE',  ( 3.456814872816273088, -13.76118077623555891, 3.223863823609153023 ) ) ;
#24946=CARTESIAN_POINT ( 'NONE',  ( 0.02969003158472209580, 157.1787724364823760, -1.485810588193620330 ) ) ;
#24948=CARTESIAN_POINT ( 'NONE',  ( -1.195985117830571820, 118.4063602595805946, -0.6806364119286731906 ) ) ;
#24949=CARTESIAN_POINT ( 'NONE',  ( 4.646169936107913401, 117.9325745699973282, -0.7782960047779410306 ) ) ;
#24951=CARTESIAN_POINT ( 'NONE',  ( -5.922169694189452827, 31.30785624307803872, 2.619824438689082768 ) ) ;
#24952=CARTESIAN_POINT ( 'NONE',  ( 15.86984883002227242, 146.9522167609303267, -0.2762592943789937694 ) ) ;
#24955=CARTESIAN_POINT ( 'NONE',  ( 2.755344442395651683, -14.11966664619605716, -0.1083093155031689958 ) ) ;
#24956=DIRECTION ( 'NONE',  ( -0.9998004120163608288, -4.016384292689131511E-17, -0.01997839162482749342 ) ) ;
#24959=CARTESIAN_POINT ( 'NONE',  ( -1.404924415901314561, -12.60368214249519703, -4.422195601339041993 ) ) ;
#24960=CARTESIAN_POINT ( 'NONE',  ( 16.68619938060333396, 146.1290494286844819, 1.780952809221992394 ) ) ;
#24961=DIRECTION ( 'NONE',  ( -0.9998004120163608288, 0.000000000000000000, -0.01997839162482749342 ) ) ;
#24962=CARTESIAN_POINT ( 'NONE',  ( -5.597156320496795345, 117.9391977826196296, 0.5238424959023465499 ) ) ;
#24964=CARTESIAN_POINT ( 'NONE',  ( 3.345514242732226418, 6.565394131763864216, 3.211428121085859733 ) ) ;
#24965=CARTESIAN_POINT ( 'NONE',  ( 15.72550100231850223, 145.6881679641610674, 0.3142329346387552902 ) ) ;
#24966=CARTESIAN_POINT ( 'NONE',  ( -6.970347610136101046, -0.07026165769430378627, 4.770677917868129114 ) ) ;
#24968=CARTESIAN_POINT ( 'NONE',  ( -2.143470464290757604, 116.4405123390714891, -0.3531553464187269786 ) ) ;
#24969=AXIS2_PLACEMENT_3D ( 'NONE', #26114, #16520, #6118 ) ;
#24970=CARTESIAN_POINT ( 'NONE',  ( 0.02887436318418984751, 106.7790779034713324, -4.972892908546473478 ) ) ;
#24972=CARTESIAN_POINT ( 'NONE',  ( -0.02537255736359465483, 39.20946620154573736, 1.269746523260778082 ) ) ;
#24973=CARTESIAN_POINT ( 'NONE',  ( 8.141433899912401628, -11.15112405914982219, -2.164028758433363286 ) ) ;
#24974=CARTESIAN_POINT ( 'NONE',  ( 4.378691870267736874, 117.3993836135368980, 1.268072117453972636 ) ) ;
#24976=DIRECTION ( 'NONE',  ( 0.9998004120163609398, 0.000000000000000000, 0.01997839162482749689 ) ) ;
#24977=CARTESIAN_POINT ( 'NONE',  ( 0.8881552493050030028, 122.2453746293775652, -0.2465857446897831984 ) ) ;
#24978=CARTESIAN_POINT ( 'NONE',  ( -23.13757068712599718, 148.9583646262859133, 0.2674444443938936988 ) ) ;
#24980=VERTEX_POINT ( 'NONE', #31685 ) ;
#24984=CARTESIAN_POINT ( 'NONE',  ( -6.513455546617618275, 121.7797256742974383, -0.05434986243196536504 ) ) ;
#24985=CARTESIAN_POINT ( 'NONE',  ( 6.296695397805594396, -14.23921929796089003, 0.5540845800015932188 ) ) ;
#24986=CARTESIAN_POINT ( 'NONE',  ( -3.150705211532708994, 118.1710492231644736, 0.7255832847742740288 ) ) ;
#24987=CARTESIAN_POINT ( 'NONE',  ( 22.39365319421748168, 148.6363688457942942, -0.9991490326925096532 ) ) ;
#24988=CARTESIAN_POINT ( 'NONE',  ( -0.01876340930523686876, 19.73428105357427853, -4.634220987317214657 ) ) ;
#24989=CARTESIAN_POINT ( 'NONE',  ( -22.90211176506270974, 150.1344166263168347, -0.9094179090926686193 ) ) ;
#24992=CARTESIAN_POINT ( 'NONE',  ( -5.562407735369756523, 116.6996333467660634, -0.1111501472963731668 ) ) ;
#24994=CARTESIAN_POINT ( 'NONE',  ( -10.78650420462579618, 154.3566586077636487, 1.536168652981084515 ) ) ;
#24996=CARTESIAN_POINT ( 'NONE',  ( 15.49426794143295893, 128.5596447653542498, -1.561415741013213898 ) ) ;
#24997=CARTESIAN_POINT ( 'NONE',  ( -5.844153588741496819, 118.3130479344264501, -1.074361049658993705 ) ) ;
#25000=CARTESIAN_POINT ( 'NONE',  ( 11.19133892028634136, 126.1638007343821641, -0.6664143115430058995 ) ) ;
#25002=CARTESIAN_POINT ( 'NONE',  ( -17.92612601409339490, 146.8415343102147972, -2.296925525151568337 ) ) ;
#25003=CARTESIAN_POINT ( 'NONE',  ( 4.100156219318407125, -15.52122063102406813, 2.251114749721512709 ) ) ;
#25004=CARTESIAN_POINT ( 'NONE',  ( -4.145496126637243428, 118.2391368896328459, -0.3994797739803510606 ) ) ;
#25009=CARTESIAN_POINT ( 'NONE',  ( 10.86423259349699677, 154.4230204216147513, 2.019759596344636865 ) ) ;
#25011=CARTESIAN_POINT ( 'NONE',  ( 5.007560425261973869, -3.380029175189206203, 6.774419414089246416 ) ) ;
#25012=CARTESIAN_POINT ( 'NONE',  ( 2.801574634701638367, 120.9854572005495044, 0.1568784928360138498 ) ) ;
#25020=CARTESIAN_POINT ( 'NONE',  ( -22.65966732694894503, 150.6414900647796173, -0.2998287813802532065 ) ) ;
#25023=CARTESIAN_POINT ( 'NONE',  ( 5.987228303333891333, 121.4272104811933275, -0.001111587135667825967 ) ) ;
#25025=ORIENTED_EDGE ( 'NONE', *, *, #33097, .T. ) ;
#25026=CARTESIAN_POINT ( 'NONE',  ( 3.398732499897371362, 115.7029691176617234, -1.510499792607192582 ) ) ;
#25027=CARTESIAN_POINT ( 'NONE',  ( -5.911602206139031424, 121.5031286879076902, -0.2921876764073586541 ) ) ;
#25028=CARTESIAN_POINT ( 'NONE',  ( 5.341062828015524566, -12.45213391371734168, 1.712110018432928982 ) ) ;
#25029=CARTESIAN_POINT ( 'NONE',  ( -14.13727225732684012, 121.3807765770047666, 0.9276936697596736003 ) ) ;
#25031=CARTESIAN_POINT ( 'NONE',  ( 15.88955207386058532, 121.0219768425927214, 0.4226783167178085332 ) ) ;
#25032=CARTESIAN_POINT ( 'NONE',  ( 15.20596983381132183, 143.4108790439744610, 0.3714088703294859406 ) ) ;
#25034=CARTESIAN_POINT ( 'NONE',  ( 0.8991110484329473129, 28.35728145135693268, -0.3789830077994447155 ) ) ;
#25036=CARTESIAN_POINT ( 'NONE',  ( -20.69515314362144665, 152.5608647341385335, -0.4887519660486649431 ) ) ;
#25040=CARTESIAN_POINT ( 'NONE',  ( 4.178911134271665162, 118.4233117688550152, 1.013387016679737851 ) ) ;
#25042=CARTESIAN_POINT ( 'NONE',  ( 15.75167367066965340, 155.0373533369262589, 1.797107981590890580 ) ) ;
#25043=CARTESIAN_POINT ( 'NONE',  ( 20.31268976784551228, 148.7458375694471044, -1.664162616495830083 ) ) ;
#25044=CARTESIAN_POINT ( 'NONE',  ( 2.357476308904321360, 24.96372521773390929, -8.086248583043326832 ) ) ;
#25045=CARTESIAN_POINT ( 'NONE',  ( -4.872874520552260336, 117.5843641943970681, -0.8145397704027564911 ) ) ;
#25046=CARTESIAN_POINT ( 'NONE',  ( 4.929911170358315609, 117.6593520789608363, -0.7659856277397926183 ) ) ;
#25047=CARTESIAN_POINT ( 'NONE',  ( 7.613751273744796322, 124.2930771091975117, 0.1610855651276039968 ) ) ;
#25048=CARTESIAN_POINT ( 'NONE',  ( -15.77879114986273734, 146.5725700477668170, -0.1868612039608985864 ) ) ;
#25049=CARTESIAN_POINT ( 'NONE',  ( -4.177977944338337579, 119.2415290214368042, -0.9917981586689073037 ) ) ;
#25050=CARTESIAN_POINT ( 'NONE',  ( 4.813411144541747788, -15.18245576741394842, 4.205718551895911261 ) ) ;
#25051=( BOUNDED_SURFACE ( )  B_SPLINE_SURFACE ( 3, 1, ( 
 ( #10419, #40254 ),
 ( #7449, #23390 ),
 ( #11048, #648 ),
 ( #23607, #1483 ),
 ( #7240, #17638 ),
 ( #33853, #36839 ),
 ( #39614, #3842 ),
 ( #30640, #16807 ),
 ( #4681, #36422 ),
 ( #20200, #26395 ),
 ( #23173, #17431 ),
 ( #10203, #7867 ),
 ( #17014, #7659 ),
 ( #20406, #14233 ),
 ( #24033, #33227 ),
 ( #13826, #7029 ) ),
 .UNSPECIFIED., .T., .F., .T. ) 
 B_SPLINE_SURFACE_WITH_KNOTS ( ( 4, 1, 1, 1, 1, 1, 2, 1, 1, 1, 1, 1, 4 ),
 ( 2, 2 ),
 ( 0.000000000000000000, 0.02374999999999993783, 0.1365624999999999478, 0.2493749999999999578, 0.3621874999999999956, 0.4749999999999999778, 0.5000000000000000000, 0.5250000000000000222, 0.6378125000000000044, 0.7506249999999999867, 0.8634374999999999689, 0.9762499999999999512, 1.000000000000000000 ),
 ( 0.000000000000000000, 1.000000000000000000 ),
 .UNSPECIFIED. ) 
 GEOMETRIC_REPRESENTATION_ITEM ( )  RATIONAL_B_SPLINE_SURFACE ( (
 ( 1.000000000000000000, 1.000000000000000000),
 ( 1.000000000000000222, 1.000000000000000000),
 ( 0.8208939328743548591, 1.000000000000000000),
 ( 0.5876145654044752087, 1.000000000000000000),
 ( 0.4813067448364888867, 1.000000000000000000),
 ( 0.5852845309810671415, 1.000000000000000000),
 ( 0.8180077452667815496, 1.000000000000000000),
 ( 0.9982788296041308351, 1.000000000000000000),
 ( 0.9982788296041308351, 1.000000000000000000),
 ( 0.8180077452667815496, 1.000000000000000000),
 ( 0.5852845309810672525, 1.000000000000000000),
 ( 0.4813067448364889422, 1.000000000000000000),
 ( 0.5876145654044749866, 1.000000000000000000),
 ( 0.8208939328743545261, 1.000000000000000000),
 ( 1.000000000000000000, 1.000000000000000000),
 ( 1.000000000000000000, 1.000000000000000000) ) ) 
 REPRESENTATION_ITEM ( '' )  SURFACE ( )  );
#25052=CARTESIAN_POINT ( 'NONE',  ( 4.799946221452094264, 115.6909491485453145, 1.474290515423493764 ) ) ;
#25054=CARTESIAN_POINT ( 'NONE',  ( -0.6792886333135017551, 118.1651005710540687, -0.8882677707207756734 ) ) ;
#25055=ORIENTED_EDGE ( 'NONE', *, *, #15894, .T. ) ;
#25056=CARTESIAN_POINT ( 'NONE',  ( 13.63191106101874617, 125.8243951943327517, 1.964466803988918153 ) ) ;
#25057=CARTESIAN_POINT ( 'NONE',  ( -3.174366308152012373, 82.64346620154573486, -0.06343139340882730792 ) ) ;
#25058=VECTOR ( 'NONE', #13501, 1000.000000000000000 ) ;
#25059=DIRECTION ( 'NONE',  ( -0.9998004120163608288, 0.000000000000000000, -0.01997839162482747608 ) ) ;
#25060=CARTESIAN_POINT ( 'NONE',  ( -1.613589725761693794, 119.1892773189224783, 0.6629358561546617734 ) ) ;
#25061=CARTESIAN_POINT ( 'NONE',  ( -6.277010209292351206, 0.1250379130781943404, 5.629075605414042727 ) ) ;
#25062=CARTESIAN_POINT ( 'NONE',  ( 0.6075365842365665348, 120.7136710450757988, 0.2388278564565363415 ) ) ;
#25064=ADVANCED_FACE ( 'NONE', ( #24651 ), #9748, .F. ) ;
#25065=CARTESIAN_POINT ( 'NONE',  ( 0.9832365512848652012, 116.8374933757159795, -0.2893350595372072842 ) ) ;
#25069=CARTESIAN_POINT ( 'NONE',  ( -8.797017425024156623, 117.6856564229855024, -0.2139691015837985044 ) ) ;
#25072=CARTESIAN_POINT ( 'NONE',  ( -5.772319165918015749, 116.9338547871927858, -0.1153446742911716644 ) ) ;
#25073=ORIENTED_EDGE ( 'NONE', *, *, #39751, .T. ) ;
#25075=CARTESIAN_POINT ( 'NONE',  ( -6.333746706779065150, 120.0360757590860743, -1.205236591762536280 ) ) ;
#25076=DIRECTION ( 'NONE',  ( 0.9998004120163610509, 5.205824365704083805E-17, 0.01997839162482749689 ) ) ;
#25077=CARTESIAN_POINT ( 'NONE',  ( -7.089475284344026740, 121.8675249661327626, -0.6210822171188465912 ) ) ;
#25078=CARTESIAN_POINT ( 'NONE',  ( 5.008579095262371439, 117.3966161975143052, -0.7759206765000108419 ) ) ;
#25081=CARTESIAN_POINT ( 'NONE',  ( 0.6590154617207463206, 19.50938314818779062, -4.574821423538240950 ) ) ;
#25086=CARTESIAN_POINT ( 'NONE',  ( 7.796227911047320269, 122.5475566638853877, 0.4040998892956136346 ) ) ;
#25088=CIRCLE ( 'NONE', #16232, 0.5080000000000002292 ) ;
#25089=CARTESIAN_POINT ( 'NONE',  ( 4.353980591602404360, 23.44215234368072487, -1.583070106892425111 ) ) ;
#25090=CARTESIAN_POINT ( 'NONE',  ( 20.52999062792637019, 132.2049894596293313, 1.489094535601873215 ) ) ;
#25091=CARTESIAN_POINT ( 'NONE',  ( 4.211467216454458651, 104.6144662015457527, -2.363859967688341168 ) ) ;
#25092=CARTESIAN_POINT ( 'NONE',  ( 2.232013814210268343, -15.18320146713449148, 5.067049754691558050 ) ) ;
#25093=CARTESIAN_POINT ( 'NONE',  ( 12.17409717887508513, 120.5818589831333441, -1.028275848330292730 ) ) ;
#25094=CARTESIAN_POINT ( 'NONE',  ( -17.94049195465775881, 148.7876888829155746, 1.661648619591604481 ) ) ;
#25096=CARTESIAN_POINT ( 'NONE',  ( -3.199182136055901626, 19.34408232073488065, 3.339653329369344004 ) ) ;
#25097=CARTESIAN_POINT ( 'NONE',  ( -15.61264994714022869, 121.4606353739761744, -1.010464550865948441 ) ) ;
#25099=CARTESIAN_POINT ( 'NONE',  ( -0.9160044981361634697, -1.370538221358817310, 0.3309596765904046500 ) ) ;
#25102=CARTESIAN_POINT ( 'NONE',  ( -9.286476516978044771, 123.9149913687586064, 0.2326040378870057601 ) ) ;
#25103=CARTESIAN_POINT ( 'NONE',  ( 4.204793715662772158, -14.23101105591234550, 4.663061278791505337 ) ) ;
#25104=CARTESIAN_POINT ( 'NONE',  ( 6.537359847799108614, 121.1369950346570192, -0.6189803324213466462 ) ) ;
#25106=CARTESIAN_POINT ( 'NONE',  ( 2.812738770403601318, 115.7033313022755436, 1.680254796076790180 ) ) ;
#25108=CARTESIAN_POINT ( 'NONE',  ( -4.674760407624344971, 117.8378351759783556, -1.036698452010090810 ) ) ;
#25109=CARTESIAN_POINT ( 'NONE',  ( 13.59242215834131962, 150.2357272821285221, 0.2218801189746054114 ) ) ;
#25110=EDGE_CURVE ( 'NONE', #17903, #39565, #6024, .T. ) ;
#25112=CARTESIAN_POINT ( 'NONE',  ( 15.71367270535921712, 153.2725199748809928, 2.344280857665636209 ) ) ;
#25115=CARTESIAN_POINT ( 'NONE',  ( 0.003550340867665223877, 156.3099534201614631, -0.1776735749810080256 ) ) ;
#25116=CARTESIAN_POINT ( 'NONE',  ( 16.81673201796756700, 155.2524275687165982, 0.03818847721825018027 ) ) ;
#25122=CARTESIAN_POINT ( 'NONE',  ( 1.836962934898605404, -15.06515874082747786, 5.710661141901725024 ) ) ;
#25125=CARTESIAN_POINT ( 'NONE',  ( -4.696693711212855504, 117.9632058761038564, 0.7093352692556416095 ) ) ;
#25127=ORIENTED_EDGE ( 'NONE', *, *, #26050, .T. ) ;
#25130=CARTESIAN_POINT ( 'NONE',  ( -3.087959230053988868, 118.2558998309379064, -0.8917549213772042460 ) ) ;
#25131=CARTESIAN_POINT ( 'NONE',  ( -5.925882289753597654, 120.8604418758245487, -0.3792092984231498209 ) ) ;
#25132=CARTESIAN_POINT ( 'NONE',  ( 4.796130219922325466, 117.5429647511544431, 1.162721217937990659 ) ) ;
#25134=CARTESIAN_POINT ( 'NONE',  ( -0.3885115210726761137, 119.2343925067223722, 0.8110907263698887704 ) ) ;
#25135=CARTESIAN_POINT ( 'NONE',  ( 4.611808778022512989, -11.57686662695173929, 0.3579861242195471194 ) ) ;
#25137=DIRECTION ( 'NONE',  ( -0.9998004120163608288, 0.000000000000000000, -0.01997839162482749342 ) ) ;
#25138=CARTESIAN_POINT ( 'NONE',  ( 2.584330390446285985, -14.72226154538576459, 5.166463236119047231 ) ) ;
#25139=CARTESIAN_POINT ( 'NONE',  ( 5.380575101947356664, 117.2069880336854197, -0.6820287515226022279 ) ) ;
#25140=CARTESIAN_POINT ( 'NONE',  ( -10.21894633145453035, 123.0849000269954701, -1.386333990434162722 ) ) ;
#25142=CARTESIAN_POINT ( 'NONE',  ( -0.2616981356411249848, 38.12352966651759090, 1.602708108658221553 ) ) ;
#25143=CARTESIAN_POINT ( 'NONE',  ( -0.6753594273997497455, 115.7031289524320243, 1.734270338090476260 ) ) ;
#25144=CARTESIAN_POINT ( 'NONE',  ( 0.3994026957563919789, 5.465888722076803319, 4.619092260001838923 ) ) ;
#25145=CARTESIAN_POINT ( 'NONE',  ( 21.25299977426486464, 132.4531229209162575, 0.9669248719381913215 ) ) ;
#25147=CARTESIAN_POINT ( 'NONE',  ( 1.273769851498584904, 105.1233871752103113, -5.190496487146082139 ) ) ;
#25148=CARTESIAN_POINT ( 'NONE',  ( 3.048550003781630213, -15.65190959513015834, 4.520219006486421165 ) ) ;
#25149=B_SPLINE_CURVE_WITH_KNOTS ( 'NONE', 3,
 ( #21803, #38238, #41009, #28000, #24806, #37386, #15214, #8625, #21587, #24586, #34617, #28216, #41223, #9054, #37591, #38019, #12242, #5030, #8840, #22019, #34830, #35048, #2465, #18620, #31626, #1624, #14580, #6909, #16260, #16049, #25650, #38657, #29263, #22429, #36094, #9465, #16475, #29052, #35458, #3514, #15633, #19038, #9264, #22637, #29479, #13073, #23062, #26064, #32044, #2881, #41649, #9876, #39283, #32467, #35673 ),
 .UNSPECIFIED., .F., .F.,
 ( 4, 2, 2, 2, 2, 1, 2, 2, 2, 2, 2, 1, 2, 2, 2, 2, 2, 1, 1, 2, 2, 2, 2, 2, 1, 2, 2, 2, 2, 4 ),
 ( 0.000000000000000000, 0.03125000000001328104, 0.06250000000002656209, 0.09375000000003984313, 0.1093750000000492661, 0.1171875000000572181, 0.1210937500000612149, 0.1250000000000652256, 0.1875000000000549283, 0.2187500000000527078, 0.2343750000000545952, 0.2421875000000584532, 0.2460937500000603129, 0.2500000000000621725, 0.3749999999999173994, 0.4374999999998416267, 0.4687499999998037126, 0.4843749999997847278, 0.4921874999997781774, 0.4960937499997777889, 0.4999999999997774003, 0.6249999999998002709, 0.6874999999998119282, 0.7187499999998145928, 0.7343749999998159250, 0.7421874999998194777, 0.7499999999998230304, 0.8749999999999115152, 0.9374999999999558131, 1.000000000000000000 ),
 .UNSPECIFIED. ) ;
#25150=CARTESIAN_POINT ( 'NONE',  ( -12.53898343483658273, 122.9501582372872406, 1.331292802868025538 ) ) ;
#25151=CARTESIAN_POINT ( 'NONE',  ( 0.4517697234110209514, 20.42248995698831493, 0.8659212905253524939 ) ) ;
#25153=CARTESIAN_POINT ( 'NONE',  ( 0.7153056356866435150, 7.414959551268969662, 0.6636563042211964802 ) ) ;
#25155=EDGE_CURVE ( 'NONE', #5382, #24401, #31506, .T. ) ;
#25158=CARTESIAN_POINT ( 'NONE',  ( 1.155851712377341745, 107.4826764677166864, 4.671650131992445054 ) ) ;
#25160=CARTESIAN_POINT ( 'NONE',  ( -16.53085885483085704, 146.5532241433796230, 0.9478179252731555593 ) ) ;
#25163=CARTESIAN_POINT ( 'NONE',  ( 3.853068500771395399, -13.31557002055877525, 3.124774401994960815 ) ) ;
#25164=CARTESIAN_POINT ( 'NONE',  ( 11.41761608106091685, 123.3954635094115702, -1.178011644471332220 ) ) ;
#25166=CARTESIAN_POINT ( 'NONE',  ( -20.31017440411242347, 148.4497675966422889, -2.477828910454907163 ) ) ;
#25168=CARTESIAN_POINT ( 'NONE',  ( 8.795780368329440435, 117.6859443280086026, 0.2729219573496977080 ) ) ;
#25169=CARTESIAN_POINT ( 'NONE',  ( -6.446885413170102552, 29.42808026494702389, 0.2842954123359195950 ) ) ;
#25170=CARTESIAN_POINT ( 'NONE',  ( 2.954508604761920676, 156.0884104482065595, -0.2429312420959231777 ) ) ;
#25172=CARTESIAN_POINT ( 'NONE',  ( -1.809052985942710023, 106.7492432543851777, -4.947880635703119090 ) ) ;
#25176=CARTESIAN_POINT ( 'NONE',  ( 4.581790953832888924, -15.30257397518579232, -0.5115867857466148694 ) ) ;
#25177=CARTESIAN_POINT ( 'NONE',  ( 15.56955422694807112, 149.1167355181319181, 1.737459915651670350 ) ) ;
#25178=PLANE ( 'NONE',  #41680 ) ;
#25179=CARTESIAN_POINT ( 'NONE',  ( 22.75657594704711784, 137.3797884758947703, 0.4311216471409409778 ) ) ;
#25180=CARTESIAN_POINT ( 'NONE',  ( -5.249845242698206960, 116.4925209815607730, 0.8804580864248583438 ) ) ;
#25181=CARTESIAN_POINT ( 'NONE',  ( -0.2084201458593382406, 5.265951782950084592, 4.622859108429906883 ) ) ;
#25182=CARTESIAN_POINT ( 'NONE',  ( 9.104209967887914701, 153.9432936505793066, 0.1819237819739444872 ) ) ;
#25183=AXIS2_PLACEMENT_3D ( 'NONE', #36871, #7687, #20646 ) ;
#25184=CARTESIAN_POINT ( 'NONE',  ( 8.407117359195193984, -5.923529430292941989, 0.7350785369227282873 ) ) ;
#25185=CARTESIAN_POINT ( 'NONE',  ( -8.773404058708813125, 117.7735243877689726, -0.4939657326346613697 ) ) ;
#25186=CARTESIAN_POINT ( 'NONE',  ( -0.8061429914042389511, 121.2007779179981384, -0.4207382890248004825 ) ) ;
#25188=CARTESIAN_POINT ( 'NONE',  ( 4.496586626007489151, 27.28078351817337222, -1.068494511273165193 ) ) ;
#25189=CARTESIAN_POINT ( 'NONE',  ( 2.751661733825109923, 117.9394479625293997, 1.329244536658263698 ) ) ;
#25190=FACE_OUTER_BOUND ( 'NONE', #18625, .T. ) ;
#25191=CARTESIAN_POINT ( 'NONE',  ( 0.7705677718991392755, 119.3684187487962305, -0.7342037314787065450 ) ) ;
#25192=CARTESIAN_POINT ( 'NONE',  ( -18.31971715989132221, 125.1624627582897915, 0.2149060778942797345 ) ) ;
#25193=ORIENTED_EDGE ( 'NONE', *, *, #29820, .F. ) ;
#25195=ORIENTED_EDGE ( 'NONE', *, *, #34773, .T. ) ;
#25197=CARTESIAN_POINT ( 'NONE',  ( -9.463739348024544640, 124.7787758165406444, -0.09662325335671638482 ) ) ;
#25198=CARTESIAN_POINT ( 'NONE',  ( 5.457633994894312224, -14.92472868577397804, 3.194711634204877804 ) ) ;
#25199=CARTESIAN_POINT ( 'NONE',  ( -20.48420673234498679, 149.1468970683199586, 1.615293151967227780 ) ) ;
#25201=CARTESIAN_POINT ( 'NONE',  ( 19.78757913416905723, 132.0165317526581816, -1.053352019815566365 ) ) ;
#25202=CARTESIAN_POINT ( 'NONE',  ( -4.420329592304260480, 21.65838872207745425, -1.398650104627336743 ) ) ;
#25203=CARTESIAN_POINT ( 'NONE',  ( -4.764559463232044934, 116.8420656028321218, -0.3170442335454676797 ) ) ;
#25205=ORIENTED_EDGE ( 'NONE', *, *, #32717, .F. ) ;
#25207=B_SPLINE_SURFACE_WITH_KNOTS ( 'NONE', 3, 3, ( 
 ( #3361, #13145, #16328, #32319, #388, #3148, #29334, #32969, #6978, #175, #26137, #22495, #32749, #19314, #3582, #13571, #35522, #25711, #10154, #10371, #16111, #13355, #26560, #36162, #26344, #23342, #36380, #38717, #9527, #5050, #23766, #17796, #13778, #40204, #34220, #30377, #23980, #10580, #30592, #7608, #11205, #11001, #37199, #39995, #17589, #4429, #39785 ),
 ( #17387, #1227, #26775, #24189, #37000, #33380, #1432, #18006, #7819, #27603, #14186, #33596, #23558, #33805, #14597, #27189, #20781, #803, #36579, #8221, #37402, #20569, #30793, #13980, #4633, #30175, #20357, #14391, #4215, #1016, #20991, #8020, #26985, #10786, #7395, #36791, #17176, #34014, #24398, #1644, #40612, #27399, #40409, #4842, #11411, #21194, #18210 ),
 ( #38257, #22039, #34635, #34424, #25252, #2485, #5462, #5256, #11837, #28019, #28656, #18850, #31430, #2272, #37819, #9074, #38466, #41241, #35067, #31855, #2054, #41029, #24824, #15236, #25470, #31211, #41668, #8438, #14809, #8647, #2694, #21607, #31002, #18640, #15019, #18422, #25036, #28235, #28450, #5889, #5682, #9284, #12046, #38038, #8858, #21822, #15652 ),
 ( #22244, #41456, #12476, #34850, #31645, #15447, #35270, #12260, #6094, #1845, #27811, #40819, #11620, #24607, #37612, #21396, #32487, #3108, #19685, #28869, #32278, #13308, #16069, #32701, #16704, #10111, #22659, #3537, #26513, #10324, #38677, #42091, #25670, #25874, #29502, #22447, #29072, #26295, #19057, #35476, #12886, #38880, #9692, #3315, #29709, #16496, #342 ),
 ( #39303, #41881, #13525, #29286, #32916, #2901, #39519, #23293, #15863, #23082, #32063, #16281, #130, #35692, #9483, #13095, #36331, #12680, #26087, #6300, #36116, #19271, #6501, #6930, #19901, #19479, #3746, #551, #39094, #9896, #22869, #35907, #6716, #10737, #10534, #1382, #20734, #23719, #23503, #30129, #4165, #4795, #37151, #7560, #20520, #13937, #14340 ),
 ( #40363, #7973, #20309, #17128, #968, #33550, #1596, #36530, #17746, #26727, #33128, #26933, #20942, #39945, #7147, #36951, #7350, #36737, #1175, #4381, #4584, #27350, #23934, #27561, #17543, #17339, #11158, #30329, #7771, #14138, #3958, #40153, #10945, #27140, #33758, #16919, #30544, #24143, #39735, #33967, #40568, #30746, #14553, #11366, #24352, #20104, #29919 ),
 ( #758, #13733, #33335, #3209, #32379, #14970, #25203, #8387, #37772, #24557, #14762, #11995, #27763, #37561, #15396, #31598, #21351, #34376, #5001, #18164, #34173, #28401, #19373, #12213, #38207, #5209, #18372, #8177, #31379, #29175, #31167, #24989, #11571, #8813, #34588, #2223, #41406, #2008, #24774, #9024, #15183, #41191, #27972, #37989, #16170, #40982, #21987 ),
 ( #21, #5417, #35020, #5841, #11784, #8597, #21560, #28187, #12987, #21772, #37358, #40773, #21144, #34798, #17959, #5631, #30959, #18589, #2435, #1799, #20007, #26405, #23401, #20210, #658, #4273, #16603, #6818, #26192, #4065, #13626, #3421, #33446, #36432, #26834, #39410, #39196, #29819, #30023, #3638, #10004, #13416, #10638, #33024, #22976, #863, #17236 ),
 ( #36006, #26617, #35797, #19788, #22764, #16817, #39624, #29611, #10213, #9798, #7251, #36218, #16388, #10430, #30232, #7039, #23617, #446, #23183, #38988, #33237, #39841, #3853, #17025, #1071, #6610, #25980, #20418, #13836, #36638, #32807, #7460, #13210, #29393, #19580, #233, #32588, #34284, #8285, #14243, #1285, #23831, #37059, #10845, #5113, #37677, #31068 ),
 ( #37259, #27043, #8078, #5319, #27250, #1704, #30439, #27663, #11265, #21051, #18065, #20840, #1495, #1906, #34077, #17858, #11059, #30859, #21457, #40266, #14870, #7669, #24251, #24044, #7877, #24456, #34487, #33864, #4904, #18271, #40881, #27872, #4694, #20627, #14659, #11682, #24668, #8500, #31273, #14039, #33657, #36851, #40674, #40052, #4482, #11467, #17442 ),
 ( #17649, #30651, #37460, #21254, #14451, #27461, #40474, #28917, #37884, #8707, #35324, #12528, #21671, #5740, #6150, #19326, #19117, #6355, #25097, #32123, #15079, #41514, #35536, #31703, #25308, #11898, #31917, #8916, #25519, #12321, #38519, #41303, #18906, #18693, #9336, #2954, #2545, #5524, #22299, #15709, #15506, #18481, #38101, #12107, #41932, #15917, #28507 ),
 ( #31486, #21882, #12733, #22507, #34908, #38312, #2116, #25722, #38730, #2331, #34694, #9132, #9537, #28079, #41090, #24887, #15291, #28296, #22093, #5947, #35120, #2753, #28713, #41723, #26148, #10383, #29126, #25931, #29563, #39578, #12940, #10590, #16765, #16974, #38938, #9750, #23353, #608, #22718, #35958, #36390, #7408, #7206, #36590, #13156, #20164, #3159 ),
 ( #13366, #42146, #19960, #39150, #13582, #399, #26570, #29345, #6990, #6772, #35746, #23134, #36173, #19738, #32760, #16123, #33189, #26355, #6558, #32978, #23568, #39361, #29973, #3593, #22927, #19533, #3803, #4017, #16555, #10166, #32330, #32540, #39796, #26786, #9954, #814, #3373, #29772, #16339, #186, #13789, #10798, #7620, #40624, #14609, #20580, #33607 ),
 ( #17187, #11422, #1857, #37414, #8233, #30389, #1442, #33392, #14402, #11630, #4439, #8031, #36801, #34027, #4643, #17600, #23991, #26996, #33816, #40831, #1027, #27410, #4227, #24408, #30186, #23780, #21206, #4852, #20791, #34232, #5062, #30604, #18017, #40421, #27614, #31014, #37011, #17397, #14820, #17808, #7829, #1240, #14196, #27201, #27822, #24617, #11216 ),
 ( #37625, #20370, #24200, #13991, #40007, #40214, #11012, #37211, #21002, #30805, #1655, #6105, #28029, #34434, #15245, #38475, #18431, #8449, #38266, #24835, #38048, #2495, #8868, #5899, #2704, #25261, #28880, #41250, #31439, #8657, #28665, #9083, #41039, #15873, #18860, #9293, #21830, #21617, #12272, #12485, #28246, #34644, #34859, #35280, #15458, #5472, #31656 ),
 ( #41677, #2281, #22049, #18220, #12056, #15661, #25045, #35077, #19068, #25480, #5691, #31864, #41892, #12690, #11849, #18649, #15029, #28459, #22255, #37830, #41465, #32074, #21406, #2910, #25680, #5268, #31221, #2065, #36342, #36127, #23093, #10122, #26306, #6942, #6309, #33138, #6728, #10335, #22458, #3968, #16929, #35487, #29719, #38687, #767, #19281, #29929 ),
 ( #26524, #9703, #39105, #25884, #16078, #13320, #29082, #38891, #16716, #32928, #22670, #35703, #32289, #19489, #3118, #561, #20116, #13536, #39530, #6514, #19695, #9493, #32712, #13744, #32498, #39315, #12896, #19912, #35918, #3547, #23304, #3327, #26099, #7157, #16507, #353, #16293, #3758, #42102, #29297, #141, #13107, #29514, #9908, #22880, #37160, #5008 ),
 ( #23729, #10955, #21152, #980, #24360, #4175, #10544, #33559, #14561, #36748, #26737, #14348, #13945, #14147, #20743, #27150, #24151, #20950, #1392, #17969, #17349, #7569, #26943, #4802, #27359, #17137, #34182, #7981, #27567, #40162, #39954, #30553, #30753, #4393, #10748, #23942, #11373, #33768, #20530, #7782, #33974, #30337, #17753, #1184, #40371, #36540, #36959 ),
 ( #11167, #37365, #1604, #4593, #40576, #30967, #1808, #30139, #17552, #33345, #8184, #39746, #23513, #7359, #20318, #14769, #31175, #40989, #34596, #24783, #28195, #12434, #12221, #41415, #35029, #8606, #5849, #11580, #8396, #12005, #21997, #37569, #35229, #25212, #41627, #21358, #34384, #18804, #38216, #5218, #18381, #31815, #32022, #2653, #19016, #37781, #15611 ),
 ( #27771, #28409, #37997, #24565, #2444, #21568, #9032, #24997, #28616, #11792, #31606, #31389, #18172, #5640, #18598, #2232, #15192, #40782, #25427, #8821, #2016, #15405, #6056, #21781, #38428, #41201, #5425, #14980, #9242, #22200, #34807, #27981, #7101, #28828, #10277, #39472, #22614, #32868, #16027, #3273, #32237, #22407, #19640, #35433, #3069, #23038, #39260 ),
 ( #12638, #25828, #41842, #36069, #26469, #19854, #3700, #12843, #26039, #15820, #39048, #36281, #29027, #32654, #19227, #16448, #82, #9854, #6885, #9647, #32442, #16660, #22824, #6674, #42046, #3490, #23247, #38838, #29667, #38635, #13048, #35648, #6462, #13266, #20062, #19436, #35861, #2860, #508, #13481, #16234, #9440, #29454, #25625, #6257, #29238, #293 ),
 ( #26250, #10066, #27097, #33504, #30498, #36694, #39688, #4334, #11322, #13689, #40108, #16876, #24104, #29877, #23459, #37112, #4539, #17298, #7932, #11116, #30288, #17705, #1129, #40323, #20901, #7516, #36486, #27309, #17500, #20478, #7307, #13896, #30084, #30705, #33922, #14098, #10901, #39897, #4753, #40530, #23892, #1554, #14510, #4123, #923, #26888, #36909 ),
 ( #7726, #27523, #24311, #37316, #8133, #33083, #26680, #10489, #20693, #3914, #715, #33717, #20266, #10694, #33295, #17084, #23674, #1341, #14297, #1760, #41577, #5590, #5798, #14720, #27722, #12169, #31549, #40731, #24734, #25166, #38378, #38165, #25373, #1967, #8979, #34976, #12386, #21106, #34755, #2181, #30922, #8773, #27931, #2394, #18333, #15353, #18125 ),
 ( #17917, #11956, #24948, #37736, #21520, #4957, #28359, #31336, #11531, #21733, #34131, #15139, #18754, #8560, #11746, #24512, #37948, #31764, #34553, #5378, #37520, #8344, #28569, #15565, #40939, #21946, #34342, #28143, #21313, #5171, #18545, #31130, #14931, #41366, #41150, #2606, #3221, #12996, #6209, #25990, #16614, #38581, #13221, #2811, #19385, #25576, #32186 ),
 ( #19180, #32389, #29621, #36015, #39207, #9392, #15772, #16182, #10016, #6829, #32818, #19798, #26203, #28777, #31974, #38999, #456, #22988, #9809, #29403, #3020, #243, #6005, #41789, #6414, #16397, #12587, #13429, #35807, #3648, #22355, #35380, #26416, #19589, #15976, #12789, #9191, #22147, #35179, #18967, #28973, #41993, #25779, #38787, #9597, #22776, #29185 ),
 ( #22567, #32599, #32, #3432, #35596, #6622, #873, #36227, #30241, #1081, #13845, #39851, #23193, #7679, #7469, #29828, #27054, #31226, #20429, #24622, #26843, #30032, #10224, #14050, #11637, #10647, #23628, #2070, #7049, #5275, #34440, #17034, #27827, #10439, #36647, #26626, #16826, #40061, #667, #39634, #17451, #33668, #23411, #36441, #20016, #20219, #33034 ),
 ( #14824, #40835, #7259, #33456, #3862, #4284, #15035, #33245, #10854, #13635, #23841, #17248, #36863, #30450, #4074, #20638, #4492, #1862, #37630, #8455, #21413, #18225, #39420, #41255, #41682, #25686, #19073, #31660, #12489, #35493, #19287, #5477, #8872, #34649, #34864, #38479, #31443, #38053, #22260, #28035, #2286, #12062, #5695, #21835, #41469, #38691, #25484 ),
 ( #11854, #6314, #22464, #18655, #15877, #25049, #28464, #15249, #18437, #2709, #28250, #2499, #6110, #35284, #15463, #12277, #37836, #25267, #24841, #32079, #9498, #2916, #28884, #38271, #9087, #41044, #22053, #32293, #35082, #15665, #5903, #9298, #18865, #31870, #41896, #28671, #12694, #3122, #8663, #21623, #13115, #32934, #23520, #3333, #20122, #9710, #26314 ),
 ( #26531, #36548, #26106, #39322, #7367, #773, #3975, #16302, #22675, #10128, #16936, #13750, #39755, #26745, #33147, #35710, #38898, #19919, #20325, #29935, #3764, #36349, #9916, #7163, #12901, #6519, #13326, #23313, #19494, #33352, #568, #10552, #32505, #29304, #16082, #39536, #148, #19702, #29087, #42107, #25890, #39111, #22886, #35924, #6734, #32721, #3555 ),
 ( #23100, #16514, #36133, #29520, #360, #16723, #6951, #29726, #13542, #10342, #24364, #10962, #33774, #34188, #40377, #7987, #1193, #20957, #11586, #33566, #8188, #39962, #14354, #20536, #27156, #14566, #24569, #14153, #27366, #37575, #30972, #5014, #4399, #10754, #11172, #17973, #1812, #27775, #14775, #21157, #23736, #26950, #33979, #8402, #40786, #4808, #37370 ),
 ( #986, #36756, #1398, #11377, #7575, #21362, #30759, #4181, #17356, #30344, #17145, #27572, #40170, #7788, #30147, #13952, #23949, #36967, #20750, #4601, #17558, #30559, #24157, #17759, #37166, #1609, #40580, #41207, #2657, #31610, #28620, #31393, #9037, #38003, #31179, #25217, #38220, #8825, #34811, #18177, #15615, #2449, #24788, #22002, #25631, #15409, #19020 ),
 ( #35034, #6060, #21785, #5646, #38641, #2020, #41847, #28834, #12009, #22204, #5429, #18604, #21574, #11798, #5854, #37785, #34600, #12439, #41631, #18385, #2238, #14984, #15197, #27986, #25432, #8610, #28200, #25002, #32027, #35235, #28414, #41419, #12226, #38432, #12644, #18810, #9248, #2865, #31819, #15826, #9446, #34389, #5223, #40994, #29673, #29033, #35439 ),
 ( #35655, #22412, #300, #38844, #26045, #19646, #39055, #10072, #36075, #29461, #23254, #29244, #32448, #22621, #6892, #13272, #12849, #36288, #39266, #16666, #9860, #6468, #16455, #32876, #16241, #19443, #22831, #515, #32661, #3280, #6680, #23044, #89, #3707, #13054, #26257, #3075, #35867, #19860, #3496, #13488, #26475, #39479, #10283, #6263, #19234, #32244 ),
 ( #9653, #16034, #42054, #25835, #28337, #12566, #18311, #34734, #2372, #38144, #41346, #31741, #15956, #15748, #2791, #31952, #5983, #28753, #28120, #12769, #28547, #32162, #2157, #25759, #38766, #15117, #9371, #31313, #2585, #15545, #21924, #24927, #41555, #9577, #41129, #25351, #11935, #22335, #37925, #8748, #35358, #41766, #18731, #6188, #38558, #12363, #2996 ),
 ( #19157, #34954, #21710, #25553, #28952, #5777, #5565, #41970, #22546, #18522, #31528, #15330, #12148, #25140, #35575, #8957, #38354, #9171, #22127, #35157, #18946, #434, #39830, #35784, #36206, #22752, #19995, #3627, #13404, #26606, #13196, #35993, #36421, #26394, #10201, #3408, #23172, #13825, #6598, #10418, #9, #16592, #19567, #29381, #16806, #26823, #16376 ),
 ( #33226, #7239, #32576, #12975, #29600, #20199, #4052, #30012, #17013, #23389, #25968, #29163, #7028, #10625, #851, #33013, #39613, #221, #23606, #3196, #38976, #39399, #13616, #9784, #6393, #3841, #19363, #26180, #39183, #32368, #29808, #9992, #22964, #16159, #6807, #19776, #32796, #647, #11453, #8272, #27860, #40868, #8064, #17637, #4262, #24237, #1274 ),
 ( #34272, #27650, #40253, #21039, #1894, #11669, #14026, #17430, #1061, #14231, #4891, #40041, #4472, #30845, #36627, #10834, #20615, #27239, #30428, #7865, #5100, #34064, #17846, #1692, #37247, #14647, #17225, #31055, #4680, #21242, #20405, #14856, #7448, #33435, #40661, #30221, #27032, #23818, #36838, #11047, #24444, #7658, #37048, #33645, #24032, #11253, #20827 ),
 ( #37448, #33852, #30639, #1482, #14438, #27447, #18052, #40463, #32156, #22960, #35569, #6593, #6387, #39180, #13190, #19357, #19772, #32363, #215, #26175, #38761, #38553, #29376, #19561, #9572, #9366, #15951, #2989, #32792, #35989, #3191, #16153, #41965, #9987, #429, #29158, #6803, #3622, #6183, #28948, #12764, #4, #29596, #22330, #16587, #12561, #18941 ),
 ( #25754, #35152, #22747, #35354, #22542, #12970, #25963, #32571, #13400, #9780, #26388, #38970, #35778, #19152, #39395, #3403, #25550, #10197, #16371, #5977, #31948, #2786, #15743, #28747, #41760, #36417, #10620, #7860, #30217, #7235, #4258, #4468, #13820, #14227, #20195, #23812, #33009, #33220, #17425, #4048, #36834, #20821, #27234, #26818, #7653, #30633, #14433 ),
 ( #29803, #30008, #33641, #26603, #17008, #30423, #23168, #39609, #847, #39826, #23602, #36623, #33847, #20610, #1270, #40249, #7443, #17221, #1477, #4675, #11042, #23384, #16801, #1057, #24026, #17633, #27442, #40457, #37042, #643, #3837, #27028, #36202, #7023, #40036, #19991, #20401, #13612, #10413, #33430, #14021, #10831, #34057, #31684, #37865, #38083, #4887 ),
 ( #21651, #17841, #14850, #2313, #28488, #28278, #15489, #34267, #41284, #25077, #2527, #11247, #24870, #34469, #21035, #41072, #18048, #34676, #8484, #5505, #8266, #28061, #27855, #8060, #2097, #15062, #40862, #11664, #37242, #18464, #21440, #1688, #11881, #24232, #5302, #8897, #24650, #1888, #30840, #8689, #21865, #37660, #18250, #14642, #27643, #18677, #5722 ),
 ( #31256, #40656, #11449, #31469, #24439, #37442, #15273, #12089, #21237, #5095, #31049, #34891, #38294, #32524, #22909, #169, #29109, #9114, #35306, #12301, #35516, #32742, #28696, #42127, #15689, #12923, #38711, #6337, #19516, #6134, #28901, #29325, #19308, #3142, #38502, #16105, #6754, #41704, #3355, #35103, #9521, #12512, #22280, #9732, #19723, #22076, #25502 ),
 ( #25914, #39132, #16322, #2937, #38922, #3575, #16536, #18889, #19097, #5927, #32106, #22700, #2734, #9318, #35730, #41496, #15900, #41916, #12716, #25706, #22488, #9938, #6541, #13139, #26131, #35942, #25290, #31897, #32312, #39778, #1219, #13347, #23973, #7812, #26337, #20560, #29547, #13771, #26768, #33170, #36154, #795, #20774, #10148, #36572, #39343, #32961 ),
 ( #29955, #1009, #10572, #33589, #7598, #23551, #14178, #7388, #36782, #4422, #3998, #3787, #23759, #13973, #16956, #16747, #10364, #26553, #27182, #17380, #20349, #33373, #36372, #30370, #36991, #4205, #40196, #10991, #591, #39559, #23335, #17169, #33798, #29752, #4626, #6971, #23118, #7188, #381, #20147, #19942, #30168, #13563, #26977, #39987, #10778, #15011 ),
 ( #38030, #8212, #40603, #17786, #37811, #5247, #37190, #25027, #28010, #18414, #30995, #30785, #21388, #21599, #37395, #1635, #5042, #2263, #24596, #14589, #40811, #41019, #21184, #8636, #27594, #18202, #17997, #4834, #8012, #34414, #20983, #11403, #34627, #11828, #24390, #34213, #27390, #1836, #14381, #5454, #41233, #31421, #31203, #40401, #14800, #30585, #11612 ),
 ( #2046, #34004, #24816, #27803, #37603, #15226, #8430, #28227, #12036, #8850, #21814, #34840, #17581, #1424, #11195, #24181, #41447, #15854, #22030, #28648, #16061, #26078, #2686, #28860, #39086, #32478, #35684, #5880, #12252, #41873, #6493, #3307, #29277, #16273, #9684, #25245, #28441, #9475, #9888, #22650, #22439, #25866, #41659, #38872, #2477, #38248, #2892 ),
 ( #9065, #13086, #3100, #19471, #19049, #18842, #35468, #122, #25461, #31846, #35262, #22861, #12672, #15643, #25661, #29063, #38458, #5674, #12467, #6291, #15438, #9276, #42083, #22234, #19262, #18631, #31636, #6086, #32270, #35059, #32054, #38668, #12877, #334, #542, #4157, #39295, #3738, #30120, #35898, #10102, #19892, #13516, #16696, #7139, #33540, #33327 ),
 ( #23495, #7341, #3527, #30323, #3949, #7552, #14131, #32693, #26924, #6709, #20096, #33120, #39510, #13300, #16910, #27133, #16487, #750, #19677, #23074, #32907, #23710, #36321, #20300, #29911, #39937, #13929, #13724, #20512, #26718, #960, #10729, #10315, #36108, #36729, #17119, #23284, #6922, #29701, #26505, #4372, #17332, #39726, #10525, #36522, #1167, #40146 ),
 ( #10939, #29493, #26287, #20936, #8171, #18367, #40356, #21555, #1376, #7764, #30741, #11779, #33961, #23928, #11566, #11151, #11361, #17953, #24346, #21345, #18159, #40768, #2218, #14547, #4790, #24138, #2003, #24551, #14334, #31374, #34371, #24769, #37353, #37146, #27757, #27967, #1590, #7968, #21139, #8591, #30954, #17741, #4995, #5204, #27556, #14965, #40563 ),
 ( #34168, #31162, #1794, #37556, #34583, #40976, #14757, #8381, #15177, #28181, #27344, #37767, #30537, #5412, #41186, #36943, #20728, #33752, #4578, #17536, #38202, #31802, #21982, #25972, #10206, #9996, #39188, #26184, #225, #22968, #21766, #7032, #22756, #26398, #37983, #19999, #35998, #9788, #6811, #9019, #29385, #15599, #8808, #3412, #16380, #29166, #12979 ),
 ( #35789, #2429, #13200, #3846, #6601, #39403, #13, #2639, #24984, #19780, #23176, #38980, #19572, #16810, #34793, #33017, #29811, #32580, #439, #25197, #32800, #41401, #31592, #3631, #15390, #12208, #16595, #29604, #35015, #5835, #5626, #18789, #18584, #13408, #36210, #11989, #28396, #10422, #36631, #13619, #36842, #34068, #30016, #30432, #17017, #14236, #40045 ),
 ( #30225, #30643, #7662, #4476, #39834, #17434, #8068, #856, #4684, #36425, #10838, #13829, #23610, #11051, #21043, #10630, #23823, #4895, #27452, #1486, #26827, #7244, #20620, #14443, #40467, #24243, #11257, #17641, #20203, #23393, #1278, #17850, #37251, #27242, #20832, #7453, #33856, #39617, #33230, #33650, #7870, #4057, #651, #40258, #26610, #20409, #33439 ) ),
 .UNSPECIFIED., .F., .F., .F.,
 ( 4, 1, 1, 1, 1, 1, 1, 1, 1, 1, 1, 1, 1, 1, 1, 1, 1, 1, 1, 1, 1, 1, 1, 1, 1, 1, 1, 1, 1, 1, 1, 1, 1, 1, 1, 1, 1, 1, 1, 1, 1, 1, 1, 1, 1, 1, 3, 4 ),
 ( 4, 1, 1, 1, 1, 1, 1, 1, 1, 1, 1, 1, 2, 1, 1, 1, 2, 1, 1, 1, 1, 1, 2, 1, 1, 1, 1, 1, 1, 1, 2, 1, 1, 1, 1, 1, 1, 1, 1, 1, 4 ),
 ( 0.000000000000000000, 0.007812500000000000000, 0.01562500000000000000, 0.02343750000000000000, 0.03125000000000000000, 0.04687500000000000000, 0.06250000000000000000, 0.07812500000000000000, 0.09375000000000000000, 0.1093750000000000000, 0.1250000000000000000, 0.1406250000000000000, 0.1562500000000000000, 0.1875000000000000000, 0.2187500000000000000, 0.2500000000000000000, 0.2812500000000000000, 0.3125000000000000000, 0.3281250000000000000, 0.3437500000000000000, 0.3750000000000000000, 0.4062500000000000000, 0.4375000000000000000, 0.4687500000000000000, 0.5000000000000000000, 0.5312500000000000000, 0.5625000000000000000, 0.5937500000000000000, 0.6250000000000000000, 0.6562500000000000000, 0.6718750000000000000, 0.6875000000000000000, 0.7187500000000000000, 0.7500000000000000000, 0.7812500000000000000, 0.8125000000000000000, 0.8437500000000000000, 0.8750000000000000000, 0.8906250000000000000, 0.9062500000000000000, 0.9218750000000000000, 0.9375000000000000000, 0.9531250000000000000, 0.9687500000000000000, 0.9765625000000000000, 0.9843750000000000000, 1.000000000000000000, 1.020397104956431988 ),
 ( 0.000000000000000000, 0.01539374999999999945, 0.03078749999999999890, 0.04618125000000002089, 0.06157499999999999779, 0.07696875000000003020, 0.09236250000000004179, 0.1077562499999999979, 0.1231499999999999956, 0.1431375000000000008, 0.1631250000000000200, 0.1831125000000000114, 0.2031000000000000028, 0.2063375000000000070, 0.2095750000000000113, 0.2128125000000000155, 0.2160500000000000198, 0.2667375000000000163, 0.3174250000000000682, 0.3681125000000000647, 0.4188000000000000611, 0.5201750000000000540, 0.6215500000000000469, 0.6266374999999999584, 0.6317250000000000920, 0.6368124999999997815, 0.6418999999999999151, 0.6469874999999999376, 0.6520749999999999602, 0.6571624999999999828, 0.6622500000000000053, 0.7044687500000000879, 0.7466875000000001705, 0.7889062500000000311, 0.8010555555555555207, 0.8311249999999998916, 0.8733437499999998632, 0.9155625000000000568, 0.9403166666666666895, 0.9577812500000000284, 1.000000000000000000 ),
 .UNSPECIFIED. ) ;
#25208=CARTESIAN_POINT ( 'NONE',  ( -17.11529127082752666, 148.4623951536435698, 1.463161431351220676 ) ) ;
#25210=CARTESIAN_POINT ( 'NONE',  ( 1.009415275228580322, 157.6350123088122359, -1.589207162029931952 ) ) ;
#25212=CARTESIAN_POINT ( 'NONE',  ( -20.70190595857163274, 149.9184980045912425, -2.291194810033231111 ) ) ;
#25215=CARTESIAN_POINT ( 'NONE',  ( 10.01767202841737792, 124.1433363813624311, -0.6017494237236774568 ) ) ;
#25216=ORIENTED_EDGE ( 'NONE', *, *, #27204, .T. ) ;
#25217=CARTESIAN_POINT ( 'NONE',  ( -16.91058881216885368, 149.6223975874448229, -2.301385465272872910 ) ) ;
#25218=CARTESIAN_POINT ( 'NONE',  ( 1.842426711869078471, -15.45708672024491470, 5.391926158250404555 ) ) ;
#25219=CARTESIAN_POINT ( 'NONE',  ( -4.159407845105936197, 118.2392947828752199, -0.3847720730525907018 ) ) ;
#25221=CARTESIAN_POINT ( 'NONE',  ( -4.747830334022490106, 117.7228629901014614, 0.9149653662667899257 ) ) ;
#25222=CARTESIAN_POINT ( 'NONE',  ( 10.89299388415055070, 123.1276765127550021, 1.556224048961160955 ) ) ;
#25225=CARTESIAN_POINT ( 'NONE',  ( -6.572471397769512613, 1.803772144246908127, -5.323917895317753946 ) ) ;
#25226=CARTESIAN_POINT ( 'NONE',  ( 9.301463764468513418, 124.2035065715909496, 0.4191708393134264687 ) ) ;
#25234=CARTESIAN_POINT ( 'NONE',  ( 1.364512232122848889, 118.7629491485454025, 1.251959052674563866 ) ) ;
#25237=B_SPLINE_CURVE_WITH_KNOTS ( 'NONE', 3,
 ( #20475, #19852, #10899, #29874, #27095, #32866 ),
 .UNSPECIFIED., .F., .F.,
 ( 4, 2, 4 ),
 ( 0.000000000000000000, 0.5000000000000000000, 1.000000000000000000 ),
 .UNSPECIFIED. ) ;
#25238=CARTESIAN_POINT ( 'NONE',  ( -23.32536756748188012, 149.0517038676186417, -0.2354165988066208859 ) ) ;
#25241=CARTESIAN_POINT ( 'NONE',  ( -6.958142857130818371, 121.9433530685592046, -0.2545489040402749703 ) ) ;
#25242=CARTESIAN_POINT ( 'NONE',  ( 4.801338745653756845, 117.3993836138989906, -1.016148446936214977 ) ) ;
#25244=CARTESIAN_POINT ( 'NONE',  ( 2.432624640667874427, 115.7029433324280916, -1.605953286633470700 ) ) ;
#25245=CARTESIAN_POINT ( 'NONE',  ( -14.68908181661163148, 148.8396455022467535, -0.5202010721049650233 ) ) ;
#25246=CARTESIAN_POINT ( 'NONE',  ( 3.566861488287894844, -14.88765406650577283, 5.398167181214303945 ) ) ;
#25247=CARTESIAN_POINT ( 'NONE',  ( -21.30706188252199595, 149.4807732621110006, 1.383641861344255153 ) ) ;
#25249=CARTESIAN_POINT ( 'NONE',  ( 10.79372094067536736, 157.9251727141802633, 0.3940533352873709094 ) ) ;
#25250=CARTESIAN_POINT ( 'NONE',  ( 8.708480741344933662, 123.6715853908191605, 0.2610670616659550025 ) ) ;
#25251=CARTESIAN_POINT ( 'NONE',  ( -0.8615061033338488050, 12.60145565637890286, -0.4637196408544374537 ) ) ;
#25252=CARTESIAN_POINT ( 'NONE',  ( -2.743358099589880972, 116.5337465564440578, -0.09497135926289690389 ) ) ;
#25254=CARTESIAN_POINT ( 'NONE',  ( -6.657354853833413522, 117.1094500233132152, -0.1330297985976032216 ) ) ;
#25256=CARTESIAN_POINT ( 'NONE',  ( 5.574731289855488825, 117.5669237741502542, 0.9295890844387997287 ) ) ;
#25257=CARTESIAN_POINT ( 'NONE',  ( -2.587970193024280441, -12.16632112844677494, -3.833404006186521773 ) ) ;
#25258=CARTESIAN_POINT ( 'NONE',  ( 21.23477820244536218, 149.4807732621110006, 2.233729070194449662 ) ) ;
#25259=CARTESIAN_POINT ( 'NONE',  ( 1.172281656590494325, 158.5855360310326319, -1.517099175104413611 ) ) ;
#25260=CARTESIAN_POINT ( 'NONE',  ( 3.683590692373001296, 21.29142263786511080, 7.571256661570916258 ) ) ;
#25261=CARTESIAN_POINT ( 'NONE',  ( -22.31562366552510213, 146.3189071340513294, -1.902122558187540058 ) ) ;
#25262=CARTESIAN_POINT ( 'NONE',  ( 4.819985158455081020, 117.7659792149047888, -0.8434561934874992284 ) ) ;
#25264=B_SPLINE_CURVE_WITH_KNOTS ( 'NONE', 3,
 ( #4056, #1277, #16594, #26826, #17433, #39402, #14030, #26397, #14235, #39833, #6810, #33438, #27241, #19998, #33229, #13828, #23822, #10421, #4265, #3630, #30015, #35997, #20202, #855, #10629, #23609, #36630, #10205, #23392, #17228, #438, #7661, #13407, #33016, #36209, #3845, #36424, #1063, #27035, #16809, #19779, #40044, #36841, #20619, #7243, #29810, #13618, #26609, #33649, #9995, #4475, #22967, #32799, #11256, #18260, #34685 ),
 .UNSPECIFIED., .F., .F.,
 ( 4, 2, 2, 2, 2, 1, 2, 2, 2, 2, 2, 2, 1, 2, 2, 2, 2, 2, 1, 1, 2, 2, 2, 2, 1, 1, 2, 2, 2, 2, 4 ),
 ( 0.000000000000000000, 0.06250000000003663736, 0.1250000000000732747, 0.1875000000001099121, 0.2187500000001282863, 0.2343750000001399991, 0.2421875000001458555, 0.2500000000001517120, 0.3750000000002494671, 0.4375000000002982614, 0.4687500000003190226, 0.4843750000003258505, 0.4921875000003256284, 0.4960937500003254064, 0.5000000000003251843, 0.6250000000001366685, 0.6875000000000456302, 0.7187500000000000000, 0.7343749999999770184, 0.7421874999999621414, 0.7460937499999581446, 0.7499999999999542588, 0.8124999999999031886, 0.8437499999998805400, 0.8593749999998692157, 0.8671874999998636646, 0.8710937499998608891, 0.8749999999998582245, 0.9374999999999291678, 0.9687499999999645839, 1.000000000000000000 ),
 .UNSPECIFIED. ) ;
#25265=CARTESIAN_POINT ( 'NONE',  ( 6.114402651314309267, 119.5149100643186983, 0.5171552335003601897 ) ) ;
#25266=CARTESIAN_POINT ( 'NONE',  ( -15.77201034003361890, 145.9134097338176730, -0.1865891569459577071 ) ) ;
#25267=CARTESIAN_POINT ( 'NONE',  ( -12.16261443152851562, 122.9664497093790629, -1.797897170200384753 ) ) ;
#25268=CARTESIAN_POINT ( 'NONE',  ( 2.285161673027230389, -15.58026522864758334, 5.856586201423784388 ) ) ;
#25270=CARTESIAN_POINT ( 'NONE',  ( -2.756659151272291552, 117.3993815979357578, -1.414639205003844991 ) ) ;
#25272=CARTESIAN_POINT ( 'NONE',  ( 17.07725563869803054, 135.3907879583883869, 2.389267674572352895 ) ) ;
#25273=AXIS2_PLACEMENT_3D ( 'NONE', #30526, #30732, #20502 ) ;
#25274=CARTESIAN_POINT ( 'NONE',  ( 0.01793833495430298061, 118.1627382089642566, -0.8977079103094813828 ) ) ;
#25275=CARTESIAN_POINT ( 'NONE',  ( -0.1450076288961997528, 106.1446358501009826, 5.226538226828138178 ) ) ;
#25276=CARTESIAN_POINT ( 'NONE',  ( -6.970347610136101046, -0.07026165769430378627, 4.770677917868129114 ) ) ;
#25277=CARTESIAN_POINT ( 'NONE',  ( 6.480921187770015912, 121.5572409441427482, 0.5803991303062127072 ) ) ;
#25278=CARTESIAN_POINT ( 'NONE',  ( 0.005431400947610381079, 116.8580640273661118, -0.2718095133625907933 ) ) ;
#25282=DIRECTION ( 'NONE',  ( -0.9998004120163609398, 0.000000000000000000, -0.01997839162482749689 ) ) ;
#25283=AXIS2_PLACEMENT_3D ( 'NONE', #22849, #35889, #6912 ) ;
#25284=AXIS2_PLACEMENT_3D ( 'NONE', #395, #38725, #19112 ) ;
#25286=CARTESIAN_POINT ( 'NONE',  ( -23.11127252101368867, 149.9001116002701224, -0.4618182267416073850 ) ) ;
#25288=CARTESIAN_POINT ( 'NONE',  ( 8.270623378294651218, 120.3814744154732068, -1.107964214892792398 ) ) ;
#25290=CARTESIAN_POINT ( 'NONE',  ( -15.86281397719570307, 145.7686330500600036, -0.9137093302325696165 ) ) ;
#25292=CARTESIAN_POINT ( 'NONE',  ( 22.83504831576691529, 150.4065277667444036, 0.4818782557684029300 ) ) ;
#25293=EDGE_CURVE ( 'NONE', #39680, #32786, #26836, .T. ) ;
#25295=CARTESIAN_POINT ( 'NONE',  ( -3.453265078539333288, 21.00871511114837276, -3.102408547967784092 ) ) ;
#25297=CARTESIAN_POINT ( 'NONE',  ( -7.784012322544769269, 122.6313477034873074, -0.1555430911242075831 ) ) ;
#25299=CARTESIAN_POINT ( 'NONE',  ( -3.682264917456323339, 78.32546620154573702, -0.07358041635423968885 ) ) ;
#25300=CARTESIAN_POINT ( 'NONE',  ( -6.992289727212193107, 121.9234231950531040, 0.03108638981060581064 ) ) ;
#25301=CARTESIAN_POINT ( 'NONE',  ( -1.512449008193210931, 25.81601926892489018, -4.382106060783010903 ) ) ;
#25302=CARTESIAN_POINT ( 'NONE',  ( -0.01289612358334866170, 159.5048567107479585, 0.6453747585945883714 ) ) ;
#25303=CARTESIAN_POINT ( 'NONE',  ( 4.546605812636178356, 104.6144662015457101, -1.650915952755167782 ) ) ;
#25305=CARTESIAN_POINT ( 'NONE',  ( 19.98084523315760208, 136.1824594150436383, -1.423751267309647517 ) ) ;
#25306=CARTESIAN_POINT ( 'NONE',  ( -11.23500844718025782, 122.9575399027323073, 1.191779604289733507 ) ) ;
#25307=CARTESIAN_POINT ( 'NONE',  ( 0.1402366131884419942, -14.11417690215759713, -0.9622292808001302600 ) ) ;
#25308=CARTESIAN_POINT ( 'NONE',  ( -22.78320035282278866, 142.4248215231809240, -1.435786487410106282 ) ) ;
#25309=CARTESIAN_POINT ( 'NONE',  ( -0.8250140797137134330, 8.550980984719981137, 0.5181985368706800710 ) ) ;
#25313=CARTESIAN_POINT ( 'NONE',  ( -10.62256650593141138, 126.1357510980948575, 0.2607537273017401791 ) ) ;
#25314=CARTESIAN_POINT ( 'NONE',  ( 5.906500239725072987, -12.19293670846725774, 0.5532178544325924152 ) ) ;
#25315=CARTESIAN_POINT ( 'NONE',  ( 14.77909737591000905, 150.5114039713088516, -1.257293140667800957 ) ) ;
#25316=CARTESIAN_POINT ( 'NONE',  ( 0.3620310593072569860, 115.7033445315342561, 1.764050944526450726 ) ) ;
#25318=CARTESIAN_POINT ( 'NONE',  ( -4.845260018671773139, 117.7536946542396521, -0.9519537261478631107 ) ) ;
#25319=CARTESIAN_POINT ( 'NONE',  ( 14.17939111974011546, 138.8817910697950140, 0.2325274008182655339 ) ) ;
#25321=EDGE_CURVE ( 'NONE', #21896, #3203, #251, .T. ) ;
#25322=CARTESIAN_POINT ( 'NONE',  ( 20.08651816730950657, 147.5185649274072830, 2.508444087122727595 ) ) ;
#25323=CARTESIAN_POINT ( 'NONE',  ( 11.83539255247743149, 152.0195595274622349, 0.2364993098673506822 ) ) ;
#25324=CARTESIAN_POINT ( 'NONE',  ( -6.096105168583893358E-14, 97.88346620154572975, 1.046006720343116589E-16 ) ) ;
#25326=CARTESIAN_POINT ( 'NONE',  ( -3.682264917456324671, 104.6144662015457243, -0.07358041635423968885 ) ) ;
#25327=TOROIDAL_SURFACE ( 'NONE', #34884, 3.683000000000000718, 0.5080000000000000071 ) ;
#25328=CARTESIAN_POINT ( 'NONE',  ( 20.63094779205695417, 152.5829384802601396, -0.02634999427677312683 ) ) ;
#25330=DIRECTION ( 'NONE',  ( 4.017660918040594346E-17, -1.000000000000000000, -2.376309959284832031E-19 ) ) ;
#25334=CARTESIAN_POINT ( 'NONE',  ( 1.665918867370522083, -15.28033259084871176, 5.729025533920835578 ) ) ;
#25336=DIRECTION ( 'NONE',  ( 0.9998004120163609398, 4.016384292689130894E-17, 0.01997839162482749689 ) ) ;
#25337=B_SPLINE_CURVE_WITH_KNOTS ( 'NONE', 3,
 ( #6107, #144, #23095, #19070, #22882, #32077, #38689 ),
 .UNSPECIFIED., .F., .F.,
 ( 4, 1, 1, 1, 4 ),
 ( 0.6462721360804335458, 0.7047636632187934680, 0.8031757754791957193, 0.9015878877395978597, 1.000000000000000000 ),
 .UNSPECIFIED. ) ;
#25338=CARTESIAN_POINT ( 'NONE',  ( -4.577798419110891359, 118.0358839641028084, 0.6746410181898425673 ) ) ;
#25341=CARTESIAN_POINT ( 'NONE',  ( 5.892261121993457529, 118.9652010781061620, -1.019900290652594688 ) ) ;
#25342=CARTESIAN_POINT ( 'NONE',  ( -4.672526732406542926, 120.2198808273567892, -0.4623614190293560688 ) ) ;
#25343=CARTESIAN_POINT ( 'NONE',  ( 4.624176940134817393, 117.9598222893437054, 0.9309007159876104831 ) ) ;
#25344=DIRECTION ( 'NONE',  ( -5.206863593109713661E-17, 1.000000000000000000, -1.077750396879097183E-30 ) ) ;
#25345=CARTESIAN_POINT ( 'NONE',  ( -0.3809694336149819782, 120.1716774721349168, 0.6201936767135832751 ) ) ;
#25347=CARTESIAN_POINT ( 'NONE',  ( -4.476207883417873568, -7.053342675672244155, -1.178223045331058705 ) ) ;
#25350=CARTESIAN_POINT ( 'NONE',  ( 0.1065646865914872399, 105.8844662015456777, -5.332932678536313809 ) ) ;
#25351=CARTESIAN_POINT ( 'NONE',  ( -16.32868586224187624, 149.3997711511537148, -2.122341471705226912 ) ) ;
#25352=CARTESIAN_POINT ( 'NONE',  ( -6.068057099051500813, 121.4371919376452524, -0.1208108290503153576 ) ) ;
#25353=CARTESIAN_POINT ( 'NONE',  ( -5.712646857600669037, 30.64406086319245404, 3.136461800983552983 ) ) ;
#25355=CARTESIAN_POINT ( 'NONE',  ( 4.573446973487649281, 17.56025517495590904, -0.6989348988664985107 ) ) ;
#25356=CARTESIAN_POINT ( 'NONE',  ( 1.385657586283472797, 159.5796833544862352, 0.3718886678235075460 ) ) ;
#25357=ORIENTED_EDGE ( 'NONE', *, *, #38817, .T. ) ;
#25358=CARTESIAN_POINT ( 'NONE',  ( 2.260647411234051773, 105.1243225396854797, -4.832372919530040001 ) ) ;
#25359=CARTESIAN_POINT ( 'NONE',  ( 3.525547644170144324, -15.07001638954266731, 1.996499786560847367 ) ) ;
#25360=CARTESIAN_POINT ( 'NONE',  ( -1.064682733364023193, 157.9544661020348997, 1.608744340525368077 ) ) ;
#25361=CARTESIAN_POINT ( 'NONE',  ( -0.7860673829865619799, 16.32342451650498916, -0.5763570944834206511 ) ) ;
#25363=CARTESIAN_POINT ( 'NONE',  ( -0.9756160567605162148, 3.744600508531710226, -0.009113680661486545098 ) ) ;
#25366=FACE_OUTER_BOUND ( 'NONE', #29370, .T. ) ;
#25367=CARTESIAN_POINT ( 'NONE',  ( 6.804471202056719292, 123.7298400107579255, 0.1732695889264301847 ) ) ;
#25369=CARTESIAN_POINT ( 'NONE',  ( -9.105332701317941257, 123.1184971541203055, 0.5608273726695749417 ) ) ;
#25370=CARTESIAN_POINT ( 'NONE',  ( -15.70103477329412911, 145.5797129992483292, -0.3137440411564564879 ) ) ;
#25371=CARTESIAN_POINT ( 'NONE',  ( 3.292060170515798578, -12.34027101600769427, 0.7492661515550719242 ) ) ;
#25372=CARTESIAN_POINT ( 'NONE',  ( 17.40456409200965382, 148.7932787949812905, -1.578286399122462713 ) ) ;
#25373=CARTESIAN_POINT ( 'NONE',  ( -19.98568676637960095, 149.3093937917295762, -2.465107550769984446 ) ) ;
#25375=CARTESIAN_POINT ( 'NONE',  ( 8.547710372622628228, 118.8041091126597593, 1.212475388694229217 ) ) ;
#25377=CARTESIAN_POINT ( 'NONE',  ( 12.13843755257572354, 130.5412724693565849, -0.1686832038582289639 ) ) ;
#25379=EDGE_LOOP ( 'NONE', ( #26860, #3692 ) ) ;
#25380=CARTESIAN_POINT ( 'NONE',  ( 0.1066493941971741466, 105.7853621660184871, -5.332931186019222558 ) ) ;
#25382=EDGE_CURVE ( 'NONE', #38342, #2334, #37999, .T. ) ;
#25384=CARTESIAN_POINT ( 'NONE',  ( 4.986734588179421834, 117.3993830463062835, 0.9017165445866112128 ) ) ;
#25387=CARTESIAN_POINT ( 'NONE',  ( 7.043328640077428204, 23.89357186360551566, -4.653114003055315528 ) ) ;
#25388=CARTESIAN_POINT ( 'NONE',  ( 7.189601074672208547, 121.4526873951801633, 0.9441605179235380563 ) ) ;
#25389=DIRECTION ( 'NONE',  ( 0.9998004120163609398, 5.205824365704083189E-17, 0.01997839162482749689 ) ) ;
#25390=CARTESIAN_POINT ( 'NONE',  ( 22.66420477949313650, 150.6410255081855212, 0.3761569768119879531 ) ) ;
#25392=CARTESIAN_POINT ( 'NONE',  ( -5.282628607152124012, 116.7267603939287426, 0.8077565746219078635 ) ) ;
#25394=EDGE_CURVE ( 'NONE', #41701, #26282, #15204, .T. ) ;
#25395=CARTESIAN_POINT ( 'NONE',  ( 2.294499597581835193, -9.852027417895397932, -4.012603411698490774 ) ) ;
#25396=CARTESIAN_POINT ( 'NONE',  ( 7.044606587285096033, 122.0729346620515088, 0.1407680048458705979 ) ) ;
#25397=CARTESIAN_POINT ( 'NONE',  ( 13.99112315924537420, 122.1591959312462592, 1.692395687056787557 ) ) ;
#25398=CARTESIAN_POINT ( 'NONE',  ( -8.048466033148526932, -0.5260294302935444311, 2.538140512261041426 ) ) ;
#25399=CARTESIAN_POINT ( 'NONE',  ( 8.727022611403114638, 118.0966510066766375, -0.5008853566498474574 ) ) ;
#25400=CARTESIAN_POINT ( 'NONE',  ( -0.3568539549766963637, 120.5507043431651510, -0.5637235919965007946 ) ) ;
#25401=CARTESIAN_POINT ( 'NONE',  ( -5.586884702347496123, 100.6774662015457409, -0.1116392523995361624 ) ) ;
#25404=CARTESIAN_POINT ( 'NONE',  ( -5.875566536072981627, -5.528788512802195854, 6.048791003748659634 ) ) ;
#25405=CARTESIAN_POINT ( 'NONE',  ( 2.553797193193295012, 117.3993834737731845, 1.425018694576543510 ) ) ;
#25407=CARTESIAN_POINT ( 'NONE',  ( 3.150244473240279675, -14.07033042043420146, 1.813758411523331393 ) ) ;
#25408=CARTESIAN_POINT ( 'NONE',  ( 0.7355314204967891012, 116.0160817474902331, -1.626749668116675096 ) ) ;
#25409=CARTESIAN_POINT ( 'NONE',  ( -6.917230302149087962, 117.3903047926647787, 0.3126493885886561519 ) ) ;
#25410=ORIENTED_EDGE ( 'NONE', *, *, #22899, .T. ) ;
#25415=CARTESIAN_POINT ( 'NONE',  ( 2.845652327410156612, -15.51977306057959716, 5.689769116265302351 ) ) ;
#25416=CARTESIAN_POINT ( 'NONE',  ( -20.75082247216797171, 147.7542213611591535, 1.617965925928342097 ) ) ;
#25417=CARTESIAN_POINT ( 'NONE',  ( 5.352805660278670885, 158.9031408473208273, -0.9771030980504659125 ) ) ;
#25418=CARTESIAN_POINT ( 'NONE',  ( -0.2480930319908794535, 10.21371511114847053, -4.635561276548324727 ) ) ;
#25421=ORIENTED_EDGE ( 'NONE', *, *, #13992, .F. ) ;
#25422=CARTESIAN_POINT ( 'NONE',  ( -0.0006472084743731488631, 124.6436471961814476, 0.03238895860161147139 ) ) ;
#25424=CARTESIAN_POINT ( 'NONE',  ( -11.42483690514971251, 124.5424752485109963, 1.054873134768184118 ) ) ;
#25426=CARTESIAN_POINT ( 'NONE',  ( 13.18164045127527473, 153.9517556018257096, -1.734949727869875780 ) ) ;
#25427=CARTESIAN_POINT ( 'NONE',  ( -13.99112315924550387, 122.1591959312462592, -1.692395687056787557 ) ) ;
#25430=CARTESIAN_POINT ( 'NONE',  ( 15.65625195688299520, 148.1291547725267037, -0.6483782694814674841 ) ) ;
#25432=CARTESIAN_POINT ( 'NONE',  ( -16.90821003499447528, 140.1729163700083518, -2.280195664865559468 ) ) ;
#25433=CARTESIAN_POINT ( 'NONE',  ( 3.506097670019660217, -15.11506922876175452, 2.387495833752258267 ) ) ;
#25435=CARTESIAN_POINT ( 'NONE',  ( -4.226413698654440054, 118.2242417877410077, -0.4878142890945914023 ) ) ;
#25437=CARTESIAN_POINT ( 'NONE',  ( -4.794585119801084261, 117.6364790366381214, 0.9472855824390624679 ) ) ;
#25438=CARTESIAN_POINT ( 'NONE',  ( 10.97746297113248204, 123.2082810311540300, 1.564610664257709116 ) ) ;
#25440=VECTOR ( 'NONE', #15441, 1000.000000000000114 ) ;
#25441=EDGE_CURVE ( 'NONE', #38260, #29270, #34911, .T. ) ;
#25442=CARTESIAN_POINT ( 'NONE',  ( 4.537321141924904211, 26.63107350737006840, 0.8823464973398146283 ) ) ;
#25443=CARTESIAN_POINT ( 'NONE',  ( 0.6320571215039689772, 120.9405031987692212, 0.1040377489725132221 ) ) ;
#25444=CARTESIAN_POINT ( 'NONE',  ( 3.682264917456193221, 71.97546620154574271, 0.07358041635424013294 ) ) ;
#25445=EDGE_CURVE ( 'NONE', #4283, #29150, #24061, .T. ) ;
#25447=CARTESIAN_POINT ( 'NONE',  ( -0.3675782062531062766, 118.1588899765148000, 0.8952817763280002117 ) ) ;
#25454=CARTESIAN_POINT ( 'NONE',  ( -22.59814275696104957, 137.2245694613254443, -0.1355511068837782773 ) ) ;
#25457=CARTESIAN_POINT ( 'NONE',  ( 6.923717762196975656, 121.8542084741468727, -0.1949843968422386720 ) ) ;
#25458=CARTESIAN_POINT ( 'NONE',  ( 4.976602257458158540, 117.4065341493209331, -0.8843054372351270009 ) ) ;
#25460=CARTESIAN_POINT ( 'NONE',  ( 1.821088186378801099, 115.7029441851158680, -1.652984706171152673 ) ) ;
#25461=CARTESIAN_POINT ( 'NONE',  ( -6.494557633019148568, 121.7745328324513139, -0.2023806202038006818 ) ) ;
#25463=CARTESIAN_POINT ( 'NONE',  ( 4.383797612528895549, -14.46967269938057044, 4.720428574551663203 ) ) ;
#25464=CARTESIAN_POINT ( 'NONE',  ( -18.02024205669876622, 128.5942011134444272, 1.207605415130186710 ) ) ;
#25466=CARTESIAN_POINT ( 'NONE',  ( 22.49140923449501273, 150.7830971219523519, 0.7772193431698347643 ) ) ;
#25467=CARTESIAN_POINT ( 'NONE',  ( 1.628970766729582964, 120.9961522207271969, 0.09962698007392074839 ) ) ;
#25469=CARTESIAN_POINT ( 'NONE',  ( 0.9752960398044887569, 8.493769703755262412, 0.04006526980912952091 ) ) ;
#25470=CARTESIAN_POINT ( 'NONE',  ( -23.40402153822892828, 142.8142681763856388, -0.5431523703306524453 ) ) ;
#25474=CARTESIAN_POINT ( 'NONE',  ( -2.409930537596374212, 116.5911498892034786, 0.3318507686391455880 ) ) ;
#25476=CARTESIAN_POINT ( 'NONE',  ( 13.69970117413521393, 155.7522398296385404, 1.951476099255863739 ) ) ;
#25477=CARTESIAN_POINT ( 'NONE',  ( 1.222221009663079672, 118.4063602595805946, -0.6323148984906140635 ) ) ;
#25479=CARTESIAN_POINT ( 'NONE',  ( 8.395564333921381461, 13.51935342844394583, -0.6424836208785561498 ) ) ;
#25480=CARTESIAN_POINT ( 'NONE',  ( -7.998778050759740132, 118.2752802814886053, -1.041156008592528437 ) ) ;
#25481=CARTESIAN_POINT ( 'NONE',  ( 4.711505574849351063, 117.9616044365023271, -0.6920222299632273755 ) ) ;
#25482=CARTESIAN_POINT ( 'NONE',  ( -0.1065646865916381608, 105.8844662015456777, 5.332932678536313809 ) ) ;
#25483=CARTESIAN_POINT ( 'NONE',  ( -4.580760836099313948, 121.1907927009877000, -0.02326454623414934281 ) ) ;
#25484=CARTESIAN_POINT ( 'NONE',  ( 0.03245814172805025488, 157.7902383798253538, -1.624338139048501439 ) ) ;
#25485=CARTESIAN_POINT ( 'NONE',  ( 5.890162669548780094, -14.87046963210582362, 1.285284309844398898 ) ) ;
#25487=CARTESIAN_POINT ( 'NONE',  ( -0.7769838098421247841, 118.1651004966810774, -0.8853101393953053400 ) ) ;
#25489=CARTESIAN_POINT ( 'NONE',  ( 15.10275521329001336, 128.5586215118215705, 2.151272397954999249 ) ) ;
#25491=CARTESIAN_POINT ( 'NONE',  ( 5.217040494953375962, 115.7029491485453008, 1.134277920141861129 ) ) ;
#25492=CARTESIAN_POINT ( 'NONE',  ( -4.368052411777271438, 123.4689364668338385, -0.008193521294099921984 ) ) ;
#25493=CARTESIAN_POINT ( 'NONE',  ( 5.670988759832523485, -4.508684804710943794, -6.293633234193930726 ) ) ;
#25494=CARTESIAN_POINT ( 'NONE',  ( 16.04872481256637684, 146.6973543426590254, 1.173426683271129090 ) ) ;
#25495=CARTESIAN_POINT ( 'NONE',  ( 23.00823290520135345, 149.2143936249396461, -0.3942700086401350057 ) ) ;
#25496=CARTESIAN_POINT ( 'NONE',  ( 4.662336540953832653, 117.9271336397564909, 0.9606932247104178479 ) ) ;
#25498=CARTESIAN_POINT ( 'NONE',  ( -18.63504953328976299, 154.1157618415863624, -0.3723726386282264489 ) ) ;
#25500=CARTESIAN_POINT ( 'NONE',  ( 6.335329328642134605, 119.9360031486299789, -0.9656527664637336583 ) ) ;
#25502=CARTESIAN_POINT ( 'NONE',  ( 0.008148072696521003327, 156.3406798448389168, -0.4077628766201953359 ) ) ;
#25504=CARTESIAN_POINT ( 'NONE',  ( 15.95982161465177285, 121.0385544001969436, 0.3359599701671937000 ) ) ;
#25506=CARTESIAN_POINT ( 'NONE',  ( 1.111903444298625754, 15.29877551736591812, 4.515507465039587665 ) ) ;
#25508=CARTESIAN_POINT ( 'NONE',  ( -20.69909148798450360, 152.5508394022677692, -0.4136171090298760844 ) ) ;
#25511=CARTESIAN_POINT ( 'NONE',  ( 7.924296910773485081, 121.8627509869352679, 1.022570594433494851 ) ) ;
#25512=CARTESIAN_POINT ( 'NONE',  ( 0.02375515148176195884, 10.92298121479113426, 4.626086752085273979 ) ) ;
#25513=CARTESIAN_POINT ( 'NONE',  ( 9.505306604063411768, 118.4542681464805298, 0.9615324788044604665 ) ) ;
#25516=CARTESIAN_POINT ( 'NONE',  ( 9.140851504705331365, 119.2843051134756536, -0.9831809102843881432 ) ) ;
#25517=CARTESIAN_POINT ( 'NONE',  ( -16.46509630982090400, 135.1966315799913900, 1.639354953089778633 ) ) ;
#25518=CARTESIAN_POINT ( 'NONE',  ( 0.7325351754718939512, 15.47086736126800766, -4.571311019245588803 ) ) ;
#25519=CARTESIAN_POINT ( 'NONE',  ( -22.87667167544120517, 149.1739538623130272, -1.428090254611251275 ) ) ;
#25521=CARTESIAN_POINT ( 'NONE',  ( -15.93731397951220252, 146.3070982487133165, 0.2768821801232404511 ) ) ;
#25523=CARTESIAN_POINT ( 'NONE',  ( 5.669917404453804544, -14.04548127125972101, 2.990483579271598469 ) ) ;
#25525=CARTESIAN_POINT ( 'NONE',  ( -4.564150745914989038, 118.0173319454175669, -0.8780539647668005321 ) ) ;
#25526=CARTESIAN_POINT ( 'NONE',  ( 15.52759540040485753, 147.5317938866932366, 0.2591190040802687222 ) ) ;
#25529=CARTESIAN_POINT ( 'NONE',  ( 16.05419991788299328, 128.5601350900737998, 2.191829208737125612 ) ) ;
#25531=CARTESIAN_POINT ( 'NONE',  ( 5.078986093043054595, 75.27746620154573520, 0.1014902294541237815 ) ) ;
#25532=CARTESIAN_POINT ( 'NONE',  ( -1.008409768533949036, 116.9791385580615781, 0.3449706568517266758 ) ) ;
#25534=CARTESIAN_POINT ( 'NONE',  ( 4.924011148325399212, 117.4782075418523135, -0.9295710142836602907 ) ) ;
#25535=CARTESIAN_POINT ( 'NONE',  ( 23.30518390908419946, 149.0397177335360652, 0.1341373440727925415 ) ) ;
#25536=DIRECTION ( 'NONE',  ( -0.01997839162482737546, -1.040247600000940825E-18, 0.9998004120163610509 ) ) ;
#25537=CARTESIAN_POINT ( 'NONE',  ( 5.341067892174450549, 115.6909491485453145, -0.2000027940544922000 ) ) ;
#25539=CARTESIAN_POINT ( 'NONE',  ( -4.974001918027356695, 117.3966124608058266, -0.9751453930575103568 ) ) ;
#25542=CARTESIAN_POINT ( 'NONE',  ( -4.590661430219167727, 118.0729565861886812, 0.5857098603017855121 ) ) ;
#25545=CARTESIAN_POINT ( 'NONE',  ( -0.6576497334167915598, 118.7629491485454025, -1.273914634100742127 ) ) ;
#25546=CARTESIAN_POINT ( 'NONE',  ( 5.935441270543534209, 119.0670427498981212, -1.024523171172543767 ) ) ;
#25547=CARTESIAN_POINT ( 'NONE',  ( -4.970930975556761666, 121.2162878128435892, -0.3527489803516244971 ) ) ;
#25548=CARTESIAN_POINT ( 'NONE',  ( 4.604483500233246929, 118.0232679518424135, 0.8447168980634072177 ) ) ;
#25550=CARTESIAN_POINT ( 'NONE',  ( -9.846098633339826378, 123.9483309312939099, -0.9889573185143103462 ) ) ;
#25552=CARTESIAN_POINT ( 'NONE',  ( 0.3628555246834703207, 105.8844662015457629, -5.327769491516690437 ) ) ;
#25553=CARTESIAN_POINT ( 'NONE',  ( -2.540463897194821463, 119.9929590031203901, -0.6352340916430189166 ) ) ;
#25554=DIRECTION ( 'NONE',  ( -0.5064479475276348897, 0.8622111466057285067, -0.01012003527073128926 ) ) ;
#25556=TOROIDAL_SURFACE ( 'NONE', #26220, 3.683000000000000718, 0.5080000000000000071 ) ;
#25557=CARTESIAN_POINT ( 'NONE',  ( -2.442087156279620253, 115.7029470234981687, 1.605172157923005383 ) ) ;
#25558=CARTESIAN_POINT ( 'NONE',  ( -1.756104463947763428, 14.33678105357426702, 4.288642365192034234 ) ) ;
#25559=CARTESIAN_POINT ( 'NONE',  ( 13.21954506825620612, 156.9672759736256467, 0.8747755986887107982 ) ) ;
#25561=CARTESIAN_POINT ( 'NONE',  ( -2.150341965413615331, 104.6144662015345972, -4.893691083646714901 ) ) ;
#25562=CARTESIAN_POINT ( 'NONE',  ( 3.758269890760038034, -15.41186319813359162, 2.599103203065302292 ) ) ;
#25563=CARTESIAN_POINT ( 'NONE',  ( -0.4903093677402899919, 118.8635629087341954, 0.5952627799645435758 ) ) ;
#25564=CARTESIAN_POINT ( 'NONE',  ( -0.8770832347484921465, 27.56386522087566249, 0.4220112102557041500 ) ) ;
#25565=CARTESIAN_POINT ( 'NONE',  ( 0.9769954323678800012, -0.8923827921977626199, -0.09387087892739469364 ) ) ;
#25568=VERTEX_POINT ( 'NONE', #7602 ) ;
#25569=CARTESIAN_POINT ( 'NONE',  ( -6.631541954483209765E-14, 98.39146620154573952, -1.863789202389766375E-18 ) ) ;
#25570=CARTESIAN_POINT ( 'NONE',  ( 6.647360066587990168, 123.1390089711370166, 0.2039998645198906335 ) ) ;
#25572=CARTESIAN_POINT ( 'NONE',  ( -0.5989337510913105289, 120.4790399057546182, 0.3068722873270141038 ) ) ;
#25574=CARTESIAN_POINT ( 'NONE',  ( 3.463597221183738917, -14.01103841792809845, 4.185469790819682068 ) ) ;
#25575=CARTESIAN_POINT ( 'NONE',  ( 9.157854976475270803, 121.7740273863187923, -1.020316602444926612 ) ) ;
#25576=CARTESIAN_POINT ( 'NONE',  ( -1.054772537320801673, 158.2739225783580537, -1.630455200628576851 ) ) ;
#25577=DIRECTION ( 'NONE',  ( -0.9998004120163609398, -4.016384292689130894E-17, -0.01997839162482749689 ) ) ;
#25578=CARTESIAN_POINT ( 'NONE',  ( 8.362803050136434990, 119.6845577230325688, 1.431069710389275995 ) ) ;
#25579=CARTESIAN_POINT ( 'NONE',  ( -6.449616047178365896, 30.29533487405314318, -0.03228945779065251626 ) ) ;
#25580=CARTESIAN_POINT ( 'NONE',  ( 13.63867282259125879, 150.2122286517991085, -0.04772847129159314000 ) ) ;
#25581=EDGE_LOOP ( 'NONE', ( #21092, #38002, #19886, #540 ) ) ;
#25583=CARTESIAN_POINT ( 'NONE',  ( 2.866728174840395216, 37.98889525090484653, 1.397978221435859147 ) ) ;
#25585=TOROIDAL_SURFACE ( 'NONE', #26255, 5.080000000000005400, 0.5080000000000000071 ) ;
#25586=CARTESIAN_POINT ( 'NONE',  ( -5.002256584969458686, 16.77047026005132224, -6.819937116506380903 ) ) ;
#25587=CARTESIAN_POINT ( 'NONE',  ( 9.932629385191864557, 123.7598584631124794, 1.097969866555963625 ) ) ;
#25589=CARTESIAN_POINT ( 'NONE',  ( 3.301441731159253656, 159.4676453237595410, 0.05120667577156024636 ) ) ;
#25590=CARTESIAN_POINT ( 'NONE',  ( -5.069034061154344073, 114.3796182124986984, 1.753882200456532647 ) ) ;
#25592=CARTESIAN_POINT ( 'NONE',  ( 14.67500508075654508, 148.8517222230099719, 0.2932415260845993576 ) ) ;
#25594=CARTESIAN_POINT ( 'NONE',  ( 20.38236371569457361, 141.4490678312372722, 2.395676066357400824 ) ) ;
#25595=CARTESIAN_POINT ( 'NONE',  ( 8.391225363336687337, -15.30560670943152957, -0.4339906691978474562 ) ) ;
#25596=CARTESIAN_POINT ( 'NONE',  ( 8.745956712206110595, 117.9959567041441630, -0.4150867728463960016 ) ) ;
#25597=CARTESIAN_POINT ( 'NONE',  ( -0.9302644990745694287, 122.9246775559910390, -0.2070653534288169895 ) ) ;
#25600=CARTESIAN_POINT ( 'NONE',  ( 0.1094753925894137725, 104.6144662015478701, 5.344208972995505569 ) ) ;
#25601=CARTESIAN_POINT ( 'NONE',  ( -3.685501180670149424, 30.72893705507438611, -2.802369389919810772 ) ) ;
#25604=CARTESIAN_POINT ( 'NONE',  ( 1.979733141779612016, -15.19599036556555660, 5.309005240801834447 ) ) ;
#25605=CARTESIAN_POINT ( 'NONE',  ( 2.294838902200146080, 118.2243428780609662, -0.8383363118275910519 ) ) ;
#25606=CARTESIAN_POINT ( 'NONE',  ( -4.829765040637250095, 117.0737178285515654, 0.3500672345979856659 ) ) ;
#25612=CARTESIAN_POINT ( 'NONE',  ( 4.157678856868515460, -15.71065181052187754, 4.128466586810772831 ) ) ;
#25613=CARTESIAN_POINT ( 'NONE',  ( -8.948346978250222961, 119.7003323559047061, 1.088312767383050828 ) ) ;
#25614=CARTESIAN_POINT ( 'NONE',  ( 10.16518949684062534, 157.7687470436769388, -1.006875576665116734 ) ) ;
#25615=CARTESIAN_POINT ( 'NONE',  ( 1.961646697876492373, -0.1315482170498871728, -4.191205975169975950 ) ) ;
#25617=EDGE_LOOP ( 'NONE', ( #31540, #16431, #42151, #30072 ) ) ;
#25619=TOROIDAL_SURFACE ( 'NONE', #13371, 3.683000000000000718, 0.5080000000000000071 ) ;
#25620=CARTESIAN_POINT ( 'NONE',  ( -0.006734421714333356339, 121.9236798544229003, 0.3370180007450782056 ) ) ;
#25621=CARTESIAN_POINT ( 'NONE',  ( -5.874057931648946962, 120.5744318282211651, 0.7168624585904721513 ) ) ;
#25624=CARTESIAN_POINT ( 'NONE',  ( 11.47069961394310411, 122.2847249198043471, -1.269327653809199763 ) ) ;
#25625=CARTESIAN_POINT ( 'NONE',  ( -4.785842063580277639, 158.3075559295907055, -1.719165798332182860 ) ) ;
#25628=EDGE_LOOP ( 'NONE', ( #19764, #28453, #34983, #20009 ) ) ;
#25629=CARTESIAN_POINT ( 'NONE',  ( 5.892782515047439773, 121.3091694753028520, -0.3064017138515002237 ) ) ;
#25630=ORIENTED_EDGE ( 'NONE', *, *, #21163, .T. ) ;
#25631=CARTESIAN_POINT ( 'NONE',  ( -2.103759425340729461, 157.1282018749678002, -1.585319646506186508 ) ) ;
#25632=CARTESIAN_POINT ( 'NONE',  ( 3.394867371861720606, -15.19666007832035071, 3.108802900814295000 ) ) ;
#25633=DIRECTION ( 'NONE',  ( 4.017660918040594346E-17, -1.000000000000000000, -2.376309959284834438E-19 ) ) ;
#25637=CARTESIAN_POINT ( 'NONE',  ( -4.900629823555088471, 117.6430597497268451, 0.8581014524456938020 ) ) ;
#25638=CARTESIAN_POINT ( 'NONE',  ( 17.26689864452585965, 148.5513402141484391, 2.222558794446809927 ) ) ;
#25640=CIRCLE ( 'NONE', #20856, 5.080000000000006288 ) ;
#25641=CARTESIAN_POINT ( 'NONE',  ( -3.957843245660688680, 22.95775517496322848, 2.395914033147342970 ) ) ;
#25642=CARTESIAN_POINT ( 'NONE',  ( 12.03016689884984736, 130.4833683797432684, 0.5359549021282031811 ) ) ;
#25644=TOROIDAL_SURFACE ( 'NONE', #13393, 3.683000000000000718, 0.5080000000000000071 ) ;
#25647=CARTESIAN_POINT ( 'NONE',  ( -0.5679911634757053296, 118.1588899970992372, 0.8844275911688039837 ) ) ;
#25648=CARTESIAN_POINT ( 'NONE',  ( -6.616924617768071466E-14, 97.37546620154573418, 7.965525879364083286E-30 ) ) ;
#25650=CARTESIAN_POINT ( 'NONE',  ( -8.212032660176594945, 120.4197669723354380, -1.432790658092274683 ) ) ;
#25653=ADVANCED_FACE ( 'NONE', ( #21188 ), #24393, .T. ) ;
#25654=CARTESIAN_POINT ( 'NONE',  ( -8.030623918766140790, 158.6806155330135084, 0.07574440115180955391 ) ) ;
#25655=ORIENTED_EDGE ( 'NONE', *, *, #40501, .F. ) ;
#25657=CARTESIAN_POINT ( 'NONE',  ( 7.824763724456980540, 122.4691624671024499, -0.2194572792259929794 ) ) ;
#25658=CARTESIAN_POINT ( 'NONE',  ( 5.008434261519718156, 117.3975399490705342, -0.7758999597088642730 ) ) ;
#25660=CARTESIAN_POINT ( 'NONE',  ( 2.876251655540356111, 115.7032362331918307, -1.566559221233196686 ) ) ;
#25661=CARTESIAN_POINT ( 'NONE',  ( -8.997762725188083621, 123.9218113011205986, -0.2640260769295984522 ) ) ;
#25662=CARTESIAN_POINT ( 'NONE',  ( 5.593658044048013700, -13.59245692957503060, 2.833247147397068399 ) ) ;
#25663=CARTESIAN_POINT ( 'NONE',  ( -21.51828093163823041, 145.9698620541949765, 1.394984360948490432 ) ) ;
#25665=CARTESIAN_POINT ( 'NONE',  ( 21.88244685892433239, 151.4414241944827495, 0.6640443303913107220 ) ) ;
#25666=VECTOR ( 'NONE', #20521, 1000.000000000000000 ) ;
#25667=CARTESIAN_POINT ( 'NONE',  ( 8.867535967563629384, 123.8953242916030462, 0.2653767370228412026 ) ) ;
#25669=CARTESIAN_POINT ( 'NONE',  ( 0.1867991717342751268, 10.66319190514178139, -0.9583599856553294272 ) ) ;
#25670=CARTESIAN_POINT ( 'NONE',  ( -22.82515744214359898, 150.4067493646842593, -0.6093393687072345966 ) ) ;
#25673=VERTEX_POINT ( 'NONE', #15230 ) ;
#25674=CARTESIAN_POINT ( 'NONE',  ( 8.541884356874501094, 118.8312421787186111, 1.225717238265990883 ) ) ;
#25677=CARTESIAN_POINT ( 'NONE',  ( 13.91935487398206739, 155.8415165211600595, 1.849969996916311921 ) ) ;
#25678=CARTESIAN_POINT ( 'NONE',  ( 20.15738656758741598, 148.0303212619860744, -1.701566911850818986 ) ) ;
#25679=CARTESIAN_POINT ( 'NONE',  ( 7.912908961612729719, 12.87109176889305928, 2.878135455392844655 ) ) ;
#25680=CARTESIAN_POINT ( 'NONE',  ( -21.74891716461465663, 141.9756885651356413, -2.029123422127836029 ) ) ;
#25681=CARTESIAN_POINT ( 'NONE',  ( 4.751009958040408598, 117.9441986225446470, -0.6307358576018021745 ) ) ;
#25683=CARTESIAN_POINT ( 'NONE',  ( 5.947819151547380834, 118.9610140496397719, 0.5876226394569610267 ) ) ;
#25685=CARTESIAN_POINT ( 'NONE',  ( -3.751144962740160960, 121.0949217282140182, -0.04819499160668135052 ) ) ;
#25686=CARTESIAN_POINT ( 'NONE',  ( -18.97908907040220683, 145.0145856610025987, -2.515253529532921473 ) ) ;
#25687=CARTESIAN_POINT ( 'NONE',  ( 5.309364964326869440, -15.28511724905957969, 2.738662543889408774 ) ) ;
#25691=CARTESIAN_POINT ( 'NONE',  ( 7.475014592328083296, 120.3045338523282197, 1.338105361635808732 ) ) ;
#25694=CIRCLE ( 'NONE', #29778, 3.683000000000001162 ) ;
#25695=CARTESIAN_POINT ( 'NONE',  ( -4.469499996960022870, 123.9529229959338608, -0.04273414237147016986 ) ) ;
#25696=CARTESIAN_POINT ( 'NONE',  ( 7.100331465950064036, 27.70181474634058461, -4.559502152892632942 ) ) ;
#25697=CARTESIAN_POINT ( 'NONE',  ( 8.043896744443927105, 154.6119571123129788, 0.8805139685443127417 ) ) ;
#25698=CARTESIAN_POINT ( 'NONE',  ( 13.02773564672682127, 156.9259531928012734, -0.6619068571425152925 ) ) ;
#25700=DIRECTION ( 'NONE',  ( -4.017660918040594346E-17, 1.000000000000000000, 2.376309959284834438E-19 ) ) ;
#25702=CARTESIAN_POINT ( 'NONE',  ( -18.84845417996787020, 125.3331924886369961, -0.3579177782036729871 ) ) ;
#25704=CARTESIAN_POINT ( 'NONE',  ( 4.791256430390820498, 119.8698651693515416, -0.7146009144274133584 ) ) ;
#25705=CARTESIAN_POINT ( 'NONE',  ( 5.379065264290444404, -14.65747380975624381, 3.538013181455927914 ) ) ;
#25706=CARTESIAN_POINT ( 'NONE',  ( -9.927929498514854956, 124.8826105625126530, -0.6426615136408515561 ) ) ;
#25708=CARTESIAN_POINT ( 'NONE',  ( 0.2932902739209606313, 116.4254261620736344, 0.01852769337193122673 ) ) ;
#25709=VERTEX_POINT ( 'NONE', #18000 ) ;
#25710=CARTESIAN_POINT ( 'NONE',  ( -4.627450822138572839, 2.892058097378844117, -0.1328416527703782657 ) ) ;
#25711=CARTESIAN_POINT ( 'NONE',  ( -16.18905205736058051, 121.2598130428683447, -0.3234957879086920451 ) ) ;
#25714=DIRECTION ( 'NONE',  ( -4.017660918040594346E-17, 1.000000000000000000, 2.376309959284834438E-19 ) ) ;
#25715=CARTESIAN_POINT ( 'NONE',  ( 6.098048384433346847, 121.2450635489416015, 0.6169096678833930758 ) ) ;
#25716=CARTESIAN_POINT ( 'NONE',  ( -3.833338661037195561, 9.423677021345861604, 2.587938769098377279 ) ) ;
#25717=CARTESIAN_POINT ( 'NONE',  ( 0.3477286622123275106, 117.0882377308211773, 0.3718801884458514673 ) ) ;
#25718=CARTESIAN_POINT ( 'NONE',  ( -4.556757383386185190, 31.49269130883712720, -0.6906699653381264126 ) ) ;
#25720=CARTESIAN_POINT ( 'NONE',  ( 2.840063763404204522, 158.7847427699215928, -1.391859091975727436 ) ) ;
#25721=CARTESIAN_POINT ( 'NONE',  ( -4.556395268149300293, 8.773967715207941609, 0.7749943352582737699 ) ) ;
#25722=CARTESIAN_POINT ( 'NONE',  ( -5.832486214875789443, 117.3024554866451865, -0.6456718139904970011 ) ) ;
#25725=CARTESIAN_POINT ( 'NONE',  ( -0.008148072696648066618, 156.3406798448389168, 0.4077628766201955579 ) ) ;
#25726=CARTESIAN_POINT ( 'NONE',  ( 3.968318174290614397, -14.81366206205479763, 5.151173006574525814 ) ) ;
#25728=CARTESIAN_POINT ( 'NONE',  ( -4.625471757156744523, 117.9841676167708044, -0.8981547367807174442 ) ) ;
#25729=CARTESIAN_POINT ( 'NONE',  ( 8.981069108608807028, 123.9698733229553937, 0.1794631345465901584 ) ) ;
#25731=CARTESIAN_POINT ( 'NONE',  ( 19.83855703208262966, 148.9191654756151024, 2.494779984669014183 ) ) ;
#25734=CARTESIAN_POINT ( 'NONE',  ( -22.87957784423544894, 146.5373477140321938, 0.6332847025415453412 ) ) ;
#25735=CARTESIAN_POINT ( 'NONE',  ( 4.803906986837436222, 117.5395264250762750, -0.9847398809678364895 ) ) ;
#25736=CARTESIAN_POINT ( 'NONE',  ( 21.78567168733521697, 151.4242408681541008, -0.1492089687398848730 ) ) ;
#25742=DIRECTION ( 'NONE',  ( -5.206863593109713661E-17, 1.000000000000000000, -1.077750396879097183E-30 ) ) ;
#25743=CARTESIAN_POINT ( 'NONE',  ( -4.563054629617739444, 118.0738312922104427, 0.6152185306409869714 ) ) ;
#25745=EDGE_LOOP ( 'NONE', ( #22535, #1915, #3706, #11314 ) ) ;
#25747=CARTESIAN_POINT ( 'NONE',  ( 5.078986093043054595, 75.78546620154573077, 0.1014902294541237815 ) ) ;
#25748=AXIS2_PLACEMENT_3D ( 'NONE', #17125, #19682, #4378 ) ;
#25749=CARTESIAN_POINT ( 'NONE',  ( -5.940513678270559872, 119.1894665386702599, -1.265456493235758373 ) ) ;
#25750=CARTESIAN_POINT ( 'NONE',  ( -5.310592030460785651, 116.9519127983885340, -0.9557578278138695316 ) ) ;
#25751=CARTESIAN_POINT ( 'NONE',  ( 4.688515861213570446, 117.9735081910210255, 0.8265790947846195502 ) ) ;
#25754=CARTESIAN_POINT ( 'NONE',  ( 0.006077178772629055273, 120.4695998130595598, -0.3041268764237431421 ) ) ;
#25758=CARTESIAN_POINT ( 'NONE',  ( 5.480007210012603380, 117.5214873295501405, -0.6081561229113361389 ) ) ;
#25759=CARTESIAN_POINT ( 'NONE',  ( -15.36238541928155676, 134.8939017613128328, -2.058614936883395252 ) ) ;
#25760=CARTESIAN_POINT ( 'NONE',  ( 17.31377588638417819, 122.7721875394316555, 0.3459704467065362055 ) ) ;
#25761=CARTESIAN_POINT ( 'NONE',  ( -0.01133159106151501033, 159.5297144918048673, 0.5670791535570577357 ) ) ;
#25763=CARTESIAN_POINT ( 'NONE',  ( -4.157303687089163979, 2.242350289152962528, -2.029258473605290103 ) ) ;
#25764=CARTESIAN_POINT ( 'NONE',  ( 22.76704383476076643, 150.0845277111093310, 1.179919005961814316 ) ) ;
#25767=CARTESIAN_POINT ( 'NONE',  ( 3.462569250300066681, -15.15729918637651075, 2.757833548007345037 ) ) ;
#25768=CARTESIAN_POINT ( 'NONE',  ( -12.38900849369197488, 122.4057692182592092, 1.312116060471626433 ) ) ;
#25769=CARTESIAN_POINT ( 'NONE',  ( 0.4369565669422456611, 1.205365006982008547, 0.8739355888918843851 ) ) ;
#25770=CARTESIAN_POINT ( 'NONE',  ( 0.8726510978149698561, 7.843753604616166442, 0.4398688123008435147 ) ) ;
#25772=ORIENTED_EDGE ( 'NONE', *, *, #35802, .T. ) ;
#25774=CARTESIAN_POINT ( 'NONE',  ( 3.352959238113102813, 119.3320731715853782, 0.6187547705018834332 ) ) ;
#25776=CARTESIAN_POINT ( 'NONE',  ( -15.97699994813262236, 148.2453349897154737, 0.9478121846735144684 ) ) ;
#25777=CARTESIAN_POINT ( 'NONE',  ( 3.873131646279637241, -11.92617534808754165, 0.9134907789774980857 ) ) ;
#25778=CARTESIAN_POINT ( 'NONE',  ( 12.79346581414803907, 125.9836878220586556, -1.262672879670394099 ) ) ;
#25779=CARTESIAN_POINT ( 'NONE',  ( -6.251746415250131861, 157.3995435888475072, -1.956906209352898385 ) ) ;
#25780=CARTESIAN_POINT ( 'NONE',  ( -6.639407854763120941E-14, 101.6934662015457320, 3.307182826377456566E-30 ) ) ;
#25781=CARTESIAN_POINT ( 'NONE',  ( 7.851011797225573297, 122.2448088404016744, 0.7696373360186058443 ) ) ;
#25782=CARTESIAN_POINT ( 'NONE',  ( -0.03167860221993856057, 39.02239338330883811, 0.4531538051958025060 ) ) ;
#25783=CARTESIAN_POINT ( 'NONE',  ( 8.936721596564167314, 123.7033391712731145, -0.04711667938246239667 ) ) ;
#25790=CARTESIAN_POINT ( 'NONE',  ( -4.582397001690157623, 27.87760190724945630, 0.5120981666136417143 ) ) ;
#25791=CARTESIAN_POINT ( 'NONE',  ( 10.02582114772196320, 123.8737202207250618, 1.106617482833786026 ) ) ;
#25792=CARTESIAN_POINT ( 'NONE',  ( 4.581716828367337513, -15.30239761468843973, -0.5121115983836379559 ) ) ;
#25793=CARTESIAN_POINT ( 'NONE',  ( 6.900242392319256624, 117.1694300671557727, 0.09431812980450680894 ) ) ;
#25794=CARTESIAN_POINT ( 'NONE',  ( -5.120189775498736218, 114.3381464724725447, 1.761508159713760957 ) ) ;
#25797=CARTESIAN_POINT ( 'NONE',  ( -4.432242455686237648, 32.76553509196318004, 1.287969469385144006 ) ) ;
#25798=CARTESIAN_POINT ( 'NONE',  ( 16.06052414861342825, 125.3625853296581312, 1.884096674228965540 ) ) ;
#25799=CARTESIAN_POINT ( 'NONE',  ( 0.7325351754718939512, 15.47086736126800766, -4.571311019245588803 ) ) ;
#25800=CARTESIAN_POINT ( 'NONE',  ( 8.358864306157585133, 27.05150166619590379, -1.223686670289468870 ) ) ;
#25801=CARTESIAN_POINT ( 'NONE',  ( 2.178318100214458042, 116.7197325431357626, -0.3987410329529229025 ) ) ;
#25802=CARTESIAN_POINT ( 'NONE',  ( -1.569003042721709651, 118.7759820277219944, -0.8276293794157988382 ) ) ;
#25803=CARTESIAN_POINT ( 'NONE',  ( 2.461950787117386241, 107.2461522219063852, -4.634887458941427951 ) ) ;
#25804=CARTESIAN_POINT ( 'NONE',  ( 3.603301376113230869, 105.1231864822307074, 3.947254286302657622 ) ) ;
#25805=CARTESIAN_POINT ( 'NONE',  ( -4.603678009535974169, 12.38766144714272066, -0.4343361176327051321 ) ) ;
#25806=CARTESIAN_POINT ( 'NONE',  ( 4.691674582040246122, 118.1588881536613655, 0.6237239105626953828 ) ) ;
#25807=CARTESIAN_POINT ( 'NONE',  ( -18.86374853661781970, 125.3403196291361610, -0.3769425889880998470 ) ) ;
#25808=CARTESIAN_POINT ( 'NONE',  ( 3.074000544403499902, -13.70685301784095600, 1.494313880732895283 ) ) ;
#25809=CARTESIAN_POINT ( 'NONE',  ( 1.209846520933339553, 108.5039085404744981, -4.223631676023018144 ) ) ;
#25810=CARTESIAN_POINT ( 'NONE',  ( -8.172070396906034873, 117.7057695168643932, 0.3161122371724937041 ) ) ;
#25815=ORIENTED_EDGE ( 'NONE', *, *, #18492, .F. ) ;
#25816=CARTESIAN_POINT ( 'NONE',  ( 4.081004676854354862, -15.57459693632588760, 4.681182614216856663 ) ) ;
#25817=CARTESIAN_POINT ( 'NONE',  ( -10.41147150295396528, 120.1444133044471556, 1.103258690517171514 ) ) ;
#25818=CARTESIAN_POINT ( 'NONE',  ( 5.877369116561975915, 117.9059190437751141, -0.7167914486236909299 ) ) ;
#25819=CARTESIAN_POINT ( 'NONE',  ( 3.895047602890354010, -2.730319773039217690, 2.488009491782988469 ) ) ;
#25820=EDGE_CURVE ( 'NONE', #19060, #26194, #29522, .T. ) ;
#25824=CARTESIAN_POINT ( 'NONE',  ( 0.3562792453294140183, 120.3637084677653633, 0.5982640298941754864 ) ) ;
#25825=CARTESIAN_POINT ( 'NONE',  ( -8.085704850285766909, 121.5393406094847819, 0.8545391641419388673 ) ) ;
#25827=CARTESIAN_POINT ( 'NONE',  ( 11.86655615995733903, 122.9427978038690270, -1.277170931065712445 ) ) ;
#25828=CARTESIAN_POINT ( 'NONE',  ( -0.4079906055176309998, 117.9789173577105572, -0.5621165275234436542 ) ) ;
#25831=CARTESIAN_POINT ( 'NONE',  ( 4.456149177844714870, 118.1611006391523802, -0.4359789887486856808 ) ) ;
#25833=CARTESIAN_POINT ( 'NONE',  ( 16.08724493259836308, 146.0544122543811341, -0.5338004346038368597 ) ) ;
#25835=CARTESIAN_POINT ( 'NONE',  ( -2.508893989683191883, 119.8406177399916714, -0.6723988897110714236 ) ) ;
#25836=CARTESIAN_POINT ( 'NONE',  ( 3.518836906362542205, -15.09289160254213868, 2.194652486238897193 ) ) ;
#25837=CARTESIAN_POINT ( 'NONE',  ( -3.292844983492351663, 105.1237654751116679, -4.198017798423213875 ) ) ;
#25839=TOROIDAL_SURFACE ( 'NONE', #31286, 5.080000000000005400, 0.5080000000000000071 ) ;
#25840=CARTESIAN_POINT ( 'NONE',  ( -4.880401117214993256, 117.7311422177337477, 0.7973360288362750792 ) ) ;
#25841=CARTESIAN_POINT ( 'NONE',  ( 0.8355136867051613514, 157.0053619834820324, 1.416332280276763056 ) ) ;
#25843=CARTESIAN_POINT ( 'NONE',  ( -3.290491044589036740, 30.52917213649525507, -3.264312889705288878 ) ) ;
#25844=CARTESIAN_POINT ( 'NONE',  ( 9.171413160121566932, 124.0935018032023436, 0.3437271393031031685 ) ) ;
#25846=EDGE_CURVE ( 'NONE', #21511, #32767, #8410, .T. ) ;
#25847=EDGE_CURVE ( 'NONE', #6137, #4990, #37606, .T. ) ;
#25858=B_SPLINE_CURVE_WITH_KNOTS ( 'NONE', 3,
 ( #22081, #38089, #35108, #5933, #31903, #6760, #16544, #9738, #29554, #20154, #42133, #16754, #6344, #22916, #29115, #35736, #23125, #33177, #22707, #35948, #4006, #39139, #7196, #12930, #19522, #19950, #16963, #19728, #3794, #598, #25920, #6548, #32530, #9944, #29963, #38928 ),
 .UNSPECIFIED., .F., .F.,
 ( 4, 2, 2, 2, 2, 2, 2, 2, 2, 2, 2, 2, 2, 2, 2, 2, 2, 4 ),
 ( 0.0005651914853900366935, 0.001585058938068627417, 0.002604926390747218032, 0.003624793843425808647, 0.004644661296104399262, 0.005664528748782989877, 0.006684396201461581359, 0.007704263654140174576, 0.008724131106818766926, 0.009743998559497358408, 0.01076386601217595336, 0.01178373346485454658, 0.01280360091753313979, 0.01382346837021173648, 0.01484333582289032970, 0.01535326954922962457, 0.01586320327556892118, 0.01688307072824751093 ),
 .UNSPECIFIED. ) ;
#25859=CARTESIAN_POINT ( 'NONE',  ( -8.206428610460363871, 117.5568930537867800, 0.09596530983984032093 ) ) ;
#25862=CARTESIAN_POINT ( 'NONE',  ( 7.815145927280279459, 122.5100161380369883, -0.1573892018284728800 ) ) ;
#25863=EDGE_LOOP ( 'NONE', ( #14285, #9695, #24590, #28812 ) ) ;
#25864=CARTESIAN_POINT ( 'NONE',  ( 2.051540280110341286, 115.7029491863636252, -1.635878083004340233 ) ) ;
#25866=CARTESIAN_POINT ( 'NONE',  ( -5.992274430539111130, 155.3621521873626534, -0.2980204051088302664 ) ) ;
#25867=CARTESIAN_POINT ( 'NONE',  ( 2.663994046441380270, -15.36521416583532051, 5.826768514169494040 ) ) ;
#25868=CARTESIAN_POINT ( 'NONE',  ( -2.121647970409728856, 117.6567184779878232, 0.5798693372496744880 ) ) ;
#25869=CARTESIAN_POINT ( 'NONE',  ( -5.041199056414468416, 117.2682846570353234, -0.6824308366424440830 ) ) ;
#25870=CARTESIAN_POINT ( 'NONE',  ( 9.776364138556694172, 118.0142902678875885, 0.3953848830946986581 ) ) ;
#25871=CARTESIAN_POINT ( 'NONE',  ( 4.628951617348011638, 121.2001895567974117, 0.1993854900221215809 ) ) ;
#25873=CARTESIAN_POINT ( 'NONE',  ( 0.1178611003048646577, 6.342877585758503578, 0.9680126135609015137 ) ) ;
#25874=CARTESIAN_POINT ( 'NONE',  ( -22.65355654554115716, 150.6414900647796173, -0.6056372710714957863 ) ) ;
#25878=CARTESIAN_POINT ( 'NONE',  ( 5.544816079372258955, 117.3577646156732328, 0.8411452473849327927 ) ) ;
#25880=DIRECTION ( 'NONE',  ( -0.01997839162482761832, -1.040247600000950455E-18, 0.9998004120163610509 ) ) ;
#25881=CARTESIAN_POINT ( 'NONE',  ( 2.121516847112188575, 117.7847241295267651, 0.6923378844829271017 ) ) ;
#25882=CARTESIAN_POINT ( 'NONE',  ( 0.4701463269443866833, 118.5593716040226724, -0.5956656855050134203 ) ) ;
#25883=CARTESIAN_POINT ( 'NONE',  ( -6.209159877377784298, 7.473591768893033560, -5.687189600455027971 ) ) ;
#25884=CARTESIAN_POINT ( 'NONE',  ( -2.066728864739012295, 117.5043770775735510, -0.6257643424168403135 ) ) ;
#25885=CARTESIAN_POINT ( 'NONE',  ( 4.629299653413243121, 117.9776611452159614, -0.7348692566910467461 ) ) ;
#25887=CARTESIAN_POINT ( 'NONE',  ( 5.298772840285820962, 116.6867539651165373, 1.022742042655826245 ) ) ;
#25888=CARTESIAN_POINT ( 'NONE',  ( -0.001367086239821354828, 156.3041635968983485, 0.06841458569046227067 ) ) ;
#25890=CARTESIAN_POINT ( 'NONE',  ( -9.942133252021321255, 155.4362223408194836, -2.105659105541914045 ) ) ;
#25891=CARTESIAN_POINT ( 'NONE',  ( 5.680254533628135150, -15.02324869320220735, 2.089386157847644920 ) ) ;
#25895=EDGE_CURVE ( 'NONE', #16499, #17903, #4966, .T. ) ;
#25897=B_SPLINE_SURFACE_WITH_KNOTS ( 'NONE', 3, 3, ( 
 ( #7917, #34324, #30272, #21090, #17283, #4735, #1325, #21296, #20882, #11100, #8326, #20461, #31112, #14909, #33907, #14701, #4320 ),
 ( #17688, #24088, #1114, #30687, #40919, #14082, #1537, #33490, #37500, #27084, #37298, #30482, #40092, #17900, #5152, #10888, #27505 ),
 ( #14283, #27292, #37099, #23875, #36895, #14492, #7713, #40513, #20676, #24293, #33700, #18107, #24496, #8116, #4522, #36680, #40714 ),
 ( #34114, #11509, #1949, #17485, #4941, #30903, #7502, #1742, #41132, #22337, #2159, #8540, #34956, #15547, #5779, #38357, #12365 ),
 ( #12150, #18733, #19159, #2374, #15958, #41972, #15119, #2793, #9172, #41557, #15750, #25353, #28122, #32163, #31744, #28955, #21500 ),
 ( #28755, #15333, #37927, #25142, #9373, #2587, #8750, #28549, #5985, #28339, #41768, #21712, #22129, #34533, #34736, #2998, #5359 ) ),
 .UNSPECIFIED., .F., .F., .F.,
 ( 4, 2, 4 ),
 ( 4, 1, 1, 1, 1, 1, 1, 1, 1, 1, 1, 1, 1, 1, 4 ),
 ( 0.000000000000000000, 0.4999999999999998890, 1.000000000000000000 ),
 ( 0.000000000000000000, 0.08300113939718137268, 0.1732806554784933895, 0.2717672377176819087, 0.3752096606209606167, 0.4787223716043260135, 0.5772295444745598747, 0.6668133826162351285, 0.7470991451079272982, 0.7815930070524458317, 0.8169452614683294644, 0.8547689062991584708, 0.8968063284581728745, 0.9447228702782888288, 1.000000000000000000 ),
 .UNSPECIFIED. ) ;
#25898=CARTESIAN_POINT ( 'NONE',  ( 17.73882382519367695, 148.9562551477873740, 2.372964443305868087 ) ) ;
#25900=CIRCLE ( 'NONE', #12318, 5.080000000000006288 ) ;
#25902=CARTESIAN_POINT ( 'NONE',  ( -5.854942301702540597, 124.9344662015456890, -0.1169956811762814242 ) ) ;
#25903=CARTESIAN_POINT ( 'NONE',  ( -6.616342194955179501, 21.00577804425827111, -5.270772580892629122 ) ) ;
#25904=CARTESIAN_POINT ( 'NONE',  ( 10.66982511085990204, 153.0728289088170300, 0.9866062039827817598 ) ) ;
#25906=CARTESIAN_POINT ( 'NONE',  ( 10.46273137052124547, 157.8855781193960297, -0.6617911890761499771 ) ) ;
#25910=CARTESIAN_POINT ( 'NONE',  ( -23.29167281398218492, 149.3519930085110161, -0.4396919384238293094 ) ) ;
#25912=CARTESIAN_POINT ( 'NONE',  ( 4.447838849061712452, 119.5324918327893755, -0.7507019530623586512 ) ) ;
#25913=CARTESIAN_POINT ( 'NONE',  ( 23.34372044208193131, 149.0681261006343448, 0.4664630893998608641 ) ) ;
#25914=CARTESIAN_POINT ( 'NONE',  ( 0.003756957834429965667, 120.7746249494737896, -0.1880135328902410030 ) ) ;
#25915=CARTESIAN_POINT ( 'NONE',  ( 3.354142537596241702, -14.24820561377959649, 4.738596845331590757 ) ) ;
#25917=CARTESIAN_POINT ( 'NONE',  ( 22.98446660148354681, 150.1594536303649932, 0.4849100737359565150 ) ) ;
#25919=CARTESIAN_POINT ( 'NONE',  ( 0.7007450612751181529, 9.901275517365906609, -4.597291952374415125 ) ) ;
#25920=CARTESIAN_POINT ( 'NONE',  ( 5.039110484533481760, 105.1218593930509826, 1.758957507424023570 ) ) ;
#25921=CARTESIAN_POINT ( 'NONE',  ( -5.757472737270721730, 159.1136035536173097, -0.1150480073142621795 ) ) ;
#25923=CARTESIAN_POINT ( 'NONE',  ( -8.046888644775119559, 121.4502209704282052, 0.8789830068023335441 ) ) ;
#25924=CARTESIAN_POINT ( 'NONE',  ( 4.585212383536918956, 13.09695617864405470, 0.6580430208065696229 ) ) ;
#25925=CARTESIAN_POINT ( 'NONE',  ( 15.23381565553107286, 121.5932973536894934, 1.241876992062232343 ) ) ;
#25927=CARTESIAN_POINT ( 'NONE',  ( 3.056907941849938748, 108.4801157075169158, 4.214599240514290024 ) ) ;
#25928=CARTESIAN_POINT ( 'NONE',  ( 12.96767020122738856, 121.2479969211051127, -1.095090382205327062 ) ) ;
#25929=AXIS2_PLACEMENT_3D ( 'NONE', #22939, #622, #3602 ) ;
#25930=CARTESIAN_POINT ( 'NONE',  ( -2.065029617914060367, 6.824861272777455135, -4.134893973632223663 ) ) ;
#25931=CARTESIAN_POINT ( 'NONE',  ( -22.81419135200717818, 148.8343141121478652, -1.537101565576850515 ) ) ;
#25933=CARTESIAN_POINT ( 'NONE',  ( -2.986828117522290604, 156.0959049650892041, 0.3398701836618411853 ) ) ;
#25934=CARTESIAN_POINT ( 'NONE',  ( 2.467627578834723057, -15.39586678991472546, 5.881674146221526733 ) ) ;
#25935=CARTESIAN_POINT ( 'NONE',  ( 0.3140373394025232079, 115.7030944333331632, 1.764426444009986605 ) ) ;
#25937=CARTESIAN_POINT ( 'NONE',  ( 19.55492868859742472, 148.8045834396381508, 2.507096624874099344 ) ) ;
#25941=AXIS2_PLACEMENT_3D ( 'NONE', #37652, #30831, #38074 ) ;
#25942=CARTESIAN_POINT ( 'NONE',  ( -13.06303874853662528, 119.8917521002241955, 0.5243808535303264851 ) ) ;
#25943=CARTESIAN_POINT ( 'NONE',  ( 3.811114225546782475, 116.8316721669309572, -0.2429903670874779542 ) ) ;
#25946=APPLICATION_CONTEXT ( 'automotive_design' ) ;
#25947=CIRCLE ( 'NONE', #15060, 3.175000000000001155 ) ;
#25950=CARTESIAN_POINT ( 'NONE',  ( -4.862785380276537950, 117.4092208852611918, -1.165888418928414216 ) ) ;
#25954=CARTESIAN_POINT ( 'NONE',  ( -4.668965673006310269, 118.0244993202197605, 0.5693437839270533152 ) ) ;
#25957=ORIENTED_EDGE ( 'NONE', *, *, #36760, .T. ) ;
#25959=CARTESIAN_POINT ( 'NONE',  ( -3.637648525249608245, 118.8078150821789905, -0.9359800040424770540 ) ) ;
#25960=CARTESIAN_POINT ( 'NONE',  ( -7.643874070029948342, 124.9344662015457317, -0.1527427953284560547 ) ) ;
#25961=CARTESIAN_POINT ( 'NONE',  ( 4.807312038368031892, 117.8307531015728529, 0.8998899155070840816 ) ) ;
#25963=CARTESIAN_POINT ( 'NONE',  ( -5.176742542608756104, 120.9449653624321144, -0.6121131393098594442 ) ) ;
#25964=CARTESIAN_POINT ( 'NONE',  ( -1.848033302852856385, 115.7026900523373456, -1.721337056304435675 ) ) ;
#25965=CARTESIAN_POINT ( 'NONE',  ( -0.1701498899198997661, 105.9761672132488570, 5.294459536038139014 ) ) ;
#25967=CARTESIAN_POINT ( 'NONE',  ( 5.205184729905183438, 115.4673366222922368, -1.303740999714490201 ) ) ;
#25968=CARTESIAN_POINT ( 'NONE',  ( -7.970993357304875460, 121.6949282028273132, -1.099362369368161785 ) ) ;
#25969=CARTESIAN_POINT ( 'NONE',  ( 22.76738278397251136, 137.3906169244638136, 0.4549464913834384561 ) ) ;
#25970=CARTESIAN_POINT ( 'NONE',  ( -0.009747742627877935620, 156.3581291470199233, 0.4878169013068173743 ) ) ;
#25971=CARTESIAN_POINT ( 'NONE',  ( -2.676945639826796786, 115.7033391084184899, 1.585126308171322496 ) ) ;
#25972=CARTESIAN_POINT ( 'NONE',  ( -12.83038717616591029, 133.7433341693027842, -0.1947450472242223951 ) ) ;
#25973=CARTESIAN_POINT ( 'NONE',  ( 1.104432469574216480, -9.427232690354344413, -4.492858291722996888 ) ) ;
#25974=CARTESIAN_POINT ( 'NONE',  ( 15.60190333658766981, 121.2802728028965475, 0.9237637308081629861 ) ) ;
#25977=CARTESIAN_POINT ( 'NONE',  ( 2.255636784185061749, -15.37476536804864580, 5.049411959999403621 ) ) ;
#25978=CARTESIAN_POINT ( 'NONE',  ( -11.84733475906203104, 122.5845257805695923, 1.288679497020477127 ) ) ;
#25979=CARTESIAN_POINT ( 'NONE',  ( 0.8080343152487895475, 3.801264818822497560, -0.5430376807499140979 ) ) ;
#25980=CARTESIAN_POINT ( 'NONE',  ( -23.12143742665070434, 148.7607265879045144, -1.192451864686425500 ) ) ;
#25982=CARTESIAN_POINT ( 'NONE',  ( 0.2615529312792121419, 0.9453775857588032627, -0.9394305312888860948 ) ) ;
#25984=ORIENTED_EDGE ( 'NONE', *, *, #4529, .T. ) ;
#25986=CARTESIAN_POINT ( 'NONE',  ( 1.365700293149759492, 106.2535611835979239, 5.166841330979377034 ) ) ;
#25987=CARTESIAN_POINT ( 'NONE',  ( -4.473055752542836494, 120.8671296916768227, 0.3242568198034687654 ) ) ;
#25988=CARTESIAN_POINT ( 'NONE',  ( 1.960603841440088146, -15.05276691075377293, 5.730201639535507319 ) ) ;
#25989=CARTESIAN_POINT ( 'NONE',  ( 6.615874392072679910, 120.4115791468657903, -0.8913422009562909087 ) ) ;
#25990=CARTESIAN_POINT ( 'NONE',  ( -12.56843540011194094, 155.2353133052689032, -2.219430909113760730 ) ) ;
#25992=CARTESIAN_POINT ( 'NONE',  ( 2.769760999665409340, -14.92388480464812872, 4.423285184949336646 ) ) ;
#25993=CARTESIAN_POINT ( 'NONE',  ( 0.008457519121113112742, 39.20946620154573026, -0.4232488410869263418 ) ) ;
#25994=CARTESIAN_POINT ( 'NONE',  ( 10.50161782422432921, 126.1106773019354819, -0.1489875947030158132 ) ) ;
#26001=CARTESIAN_POINT ( 'NONE',  ( 16.23473294303248338, 121.3954344197762083, 0.2182100806314835051 ) ) ;
#26002=CARTESIAN_POINT ( 'NONE',  ( -5.284833012248508766, 116.4655405006298849, 0.8823810258511327609 ) ) ;
#26005=DIRECTION ( 'NONE',  ( 0.9998004120163608288, 0.000000000000000000, 0.01997839162482760791 ) ) ;
#26006=CARTESIAN_POINT ( 'NONE',  ( -3.742012044685256722, 31.40836143976739336, -0.4637063799314742329 ) ) ;
#26008=CARTESIAN_POINT ( 'NONE',  ( 0.4079906055175022139, 117.9789173577105572, 0.5621165275234438763 ) ) ;
#26009=CARTESIAN_POINT ( 'NONE',  ( -4.295268622494708310, 18.69437521248495671, 1.722957355393906598 ) ) ;
#26010=CARTESIAN_POINT ( 'NONE',  ( 8.340720164204880049, -15.19402286670749191, -1.049415519506536665 ) ) ;
#26011=CARTESIAN_POINT ( 'NONE',  ( -5.481623637317887265, 117.2526226941921834, -0.8295243230819944191 ) ) ;
#26012=CARTESIAN_POINT ( 'NONE',  ( -0.1346051971226650268, 106.5118632461160217, -5.080372420286161095 ) ) ;
#26014=CARTESIAN_POINT ( 'NONE',  ( 3.113094358168766451, 108.2626774329659440, -4.181916884918123856 ) ) ;
#26015=CARTESIAN_POINT ( 'NONE',  ( 1.938979755385511261, 104.6144662015456817, 4.428504999821790022 ) ) ;
#26016=CARTESIAN_POINT ( 'NONE',  ( 4.256838582791900194, 16.71066835407712858, 1.825063967593055558 ) ) ;
#26019=CARTESIAN_POINT ( 'NONE',  ( 3.221735024265227398, -14.36526069886394730, 2.718910799868354378 ) ) ;
#26020=CARTESIAN_POINT ( 'NONE',  ( 1.613589725761565008, 119.1892773189224783, -0.6629358561546615514 ) ) ;
#26021=CARTESIAN_POINT ( 'NONE',  ( -1.937878880890249844, 116.8467566806161386, 0.3061478142745881481 ) ) ;
#26026=CARTESIAN_POINT ( 'NONE',  ( -3.046231754824816118, 31.09810386281187533, 0.4001267285823233433 ) ) ;
#26027=CARTESIAN_POINT ( 'NONE',  ( 2.279390105945505507, -15.60765617898064761, 5.834426787525912594 ) ) ;
#26028=CARTESIAN_POINT ( 'NONE',  ( -11.46709954559049649, 121.1873859956591843, 1.221572053168039185 ) ) ;
#26029=CARTESIAN_POINT ( 'NONE',  ( 0.02399864187730012949, 159.1630378086529731, -1.200990174154242363 ) ) ;
#26030=CARTESIAN_POINT ( 'NONE',  ( 3.700881553190929374, 8.714383148187751615, -2.768892949411812854 ) ) ;
#26033=CARTESIAN_POINT ( 'NONE',  ( 5.078986093043053707, 97.88346620154572975, 0.1014902294541244060 ) ) ;
#26034=CARTESIAN_POINT ( 'NONE',  ( 0.4066243552752198398, 124.0591982226670211, 0.1013866577921580941 ) ) ;
#26035=SURFACE_STYLE_FILL_AREA ( #23033 ) ;
#26036=CARTESIAN_POINT ( 'NONE',  ( -15.29320056080895007, 150.6904849259475441, 1.473493523582195319 ) ) ;
#26038=CARTESIAN_POINT ( 'NONE',  ( 18.50101540898958774, 149.0103496150362901, -1.723905467370217215 ) ) ;
#26039=CARTESIAN_POINT ( 'NONE',  ( -6.769736154946738083, 118.6475953829349379, -1.187203428762516166 ) ) ;
#26042=CARTESIAN_POINT ( 'NONE',  ( 4.415775866151314233, 118.1645749254845441, -0.4805746343930200060 ) ) ;
#26043=CARTESIAN_POINT ( 'NONE',  ( 10.78632646169009490, 153.0872561326487187, -0.6669751843662026225 ) ) ;
#26045=CARTESIAN_POINT ( 'NONE',  ( -3.403275764582950114, 119.7942873563901713, -0.7909988017435811702 ) ) ;
#26046=CARTESIAN_POINT ( 'NONE',  ( 3.790367410748021637, -15.17722879538144198, -0.1767333597861489025 ) ) ;
#26048=VECTOR ( 'NONE', #36363, 1000.000000000000227 ) ;
#26050=EDGE_CURVE ( 'NONE', #2334, #11330, #23718, .T. ) ;
#26051=CARTESIAN_POINT ( 'NONE',  ( -4.843782464516869446, 117.6435980591638355, 0.9175585232979758255 ) ) ;
#26052=CARTESIAN_POINT ( 'NONE',  ( 14.38208595515599875, 131.1674235819977241, 1.945708262771123076 ) ) ;
#26055=CARTESIAN_POINT ( 'NONE',  ( -4.349660437102230048, 31.17966527223318707, -1.615541842050199461 ) ) ;
#26056=CARTESIAN_POINT ( 'NONE',  ( 7.044359374033473564, 122.0696255612902519, 0.2151282384624544075 ) ) ;
#26059=CARTESIAN_POINT ( 'NONE',  ( 2.185374947706846704, 116.1939849232089443, -0.02259167694784758318 ) ) ;
#26060=DIRECTION ( 'NONE',  ( 0.9998004120163608288, 0.000000000000000000, 0.01997839162482736852 ) ) ;
#26064=CARTESIAN_POINT ( 'NONE',  ( -8.567664903271650090, 118.7102832696748607, -1.176849739173866594 ) ) ;
#26067=DIRECTION ( 'NONE',  ( -0.01997839162482737546, -1.040247600000940825E-18, 0.9998004120163610509 ) ) ;
#26071=CARTESIAN_POINT ( 'NONE',  ( -14.75425959148295618, 120.3062992333385921, -0.06863422566743775100 ) ) ;
#26072=AXIS2_PLACEMENT_3D ( 'NONE', #29570, #10387, #32984 ) ;
#26075=CARTESIAN_POINT ( 'NONE',  ( 6.060350493389893067, 121.4410810028806509, 0.1068649412279469996 ) ) ;
#26078=CARTESIAN_POINT ( 'NONE',  ( -11.17680165766864775, 128.1157469881088105, -0.4152311708251573696 ) ) ;
#26079=CARTESIAN_POINT ( 'NONE',  ( 5.218988718559132600, -14.41095047787725747, 3.833162268628383718 ) ) ;
#26080=CARTESIAN_POINT ( 'NONE',  ( -9.254844111043031063, 119.0402042963619351, 0.8977872906997166336 ) ) ;
#26081=CARTESIAN_POINT ( 'NONE',  ( -5.078986093043186045, 91.53346620154573543, -0.1014902294541237954 ) ) ;
#26083=CARTESIAN_POINT ( 'NONE',  ( 1.410028229074493433, 159.6020224343070026, 0.1582310832764451114 ) ) ;
#26084=CARTESIAN_POINT ( 'NONE',  ( 15.72120838691553502, 146.8976252958255486, 0.4481387442112281794 ) ) ;
#26085=CARTESIAN_POINT ( 'NONE',  ( 4.829493779578470480, 118.5266822147775940, -0.7638424752985826238 ) ) ;
#26086=CARTESIAN_POINT ( 'NONE',  ( -0.02445332296907207215, 6.119348097484421878, 0.9755048060674135213 ) ) ;
#26087=CARTESIAN_POINT ( 'NONE',  ( -16.18495160125072374, 121.3864332154274877, -0.4845229560194668217 ) ) ;
#26091=CARTESIAN_POINT ( 'NONE',  ( 8.585969666846875015, 118.6243502972331498, 1.142660147408910642 ) ) ;
#26095=CARTESIAN_POINT ( 'NONE',  ( 14.34163035669542197, 121.9874158357064857, 1.600522166921893863 ) ) ;
#26096=CARTESIAN_POINT ( 'NONE',  ( 10.04363327864678190, 120.6268241347409855, -1.191437567882422943 ) ) ;
#26097=CARTESIAN_POINT ( 'NONE',  ( 0.5118484794875378663, 4.451237885527871363, -0.8280682483750020362 ) ) ;
#26098=CARTESIAN_POINT ( 'NONE',  ( -8.372926607701892010, 8.771278641329313785, 0.9163881402227073147 ) ) ;
#26099=CARTESIAN_POINT ( 'NONE',  ( -21.36223069762263194, 149.8571540977637255, -2.130384393597193782 ) ) ;
#26100=CARTESIAN_POINT ( 'NONE',  ( 4.783395520282055280, 117.8481480307013385, -0.7930544963161749727 ) ) ;
#26101=CARTESIAN_POINT ( 'NONE',  ( 5.183518906920014935, 115.4398124677065596, 1.515634836823672060 ) ) ;
#26102=EDGE_CURVE ( 'NONE', #20793, #9715, #35471, .T. ) ;
#26103=CARTESIAN_POINT ( 'NONE',  ( 8.687188811298828028, 122.3401343867201945, -0.7349857017399258341 ) ) ;
#26104=CARTESIAN_POINT ( 'NONE',  ( -15.26332761227469881, 148.0152273645666980, -0.2540164781927347626 ) ) ;
#26106=CARTESIAN_POINT ( 'NONE',  ( -1.300143943178302841, 119.1766673560425858, -0.6697961403939315383 ) ) ;
#26107=CARTESIAN_POINT ( 'NONE',  ( 2.247313541653549240, -15.69307202063721718, 5.732350583303913893 ) ) ;
#26111=VERTEX_POINT ( 'NONE', #26081 ) ;
#26112=CIRCLE ( 'NONE', #7758, 5.588000000000006295 ) ;
#26113=CARTESIAN_POINT ( 'NONE',  ( 5.054692016413384614, 119.8577235299091228, 1.014870397641471911 ) ) ;
#26114=CARTESIAN_POINT ( 'NONE',  ( 3.682264917456192332, 88.99346620154574339, 0.07358041635423968885 ) ) ;
#26117=CARTESIAN_POINT ( 'NONE',  ( -3.201024870708126357, 118.2446163226072713, 0.7148959180058855889 ) ) ;
#26118=CARTESIAN_POINT ( 'NONE',  ( -5.435345482397000438, 30.30303275347894854, -6.432456514813170045 ) ) ;
#26119=CARTESIAN_POINT ( 'NONE',  ( 15.71402047398548874, 147.5983985311728759, 1.037567014598419712 ) ) ;
#26120=CARTESIAN_POINT ( 'NONE',  ( 1.973526102370556146, 116.9869758084673208, -0.3704244399607082849 ) ) ;
#26124=CARTESIAN_POINT ( 'NONE',  ( 15.70103477329399766, 145.5797129992483292, 0.3137440411564567100 ) ) ;
#26126=CARTESIAN_POINT ( 'NONE',  ( -18.63485108555828873, 154.1203422869290023, -0.3484461891417473534 ) ) ;
#26128=CARTESIAN_POINT ( 'NONE',  ( 7.959411891889985213, 121.8595877113556156, -0.7022647005503769302 ) ) ;
#26129=CARTESIAN_POINT ( 'NONE',  ( 2.664264518795053327, -15.44973899589986566, 5.798575810372247119 ) ) ;
#26131=CARTESIAN_POINT ( 'NONE',  ( -14.42924251737987262, 139.0941462050048187, -0.8894241721302191817 ) ) ;
#26132=CARTESIAN_POINT ( 'NONE',  ( 3.866302502687585907, -14.02971062843458228, 4.478402296968817531 ) ) ;
#26134=CARTESIAN_POINT ( 'NONE',  ( 3.302029177305205732, 159.4671159221996959, 0.06598240135525389183 ) ) ;
#26136=CARTESIAN_POINT ( 'NONE',  ( -4.274281473441157608, 3.541781053574249327, 1.790774723582081451 ) ) ;
#26137=CARTESIAN_POINT ( 'NONE',  ( -9.822473411059320370, 117.9943479623217399, -0.1962763949404990327 ) ) ;
#26141=CARTESIAN_POINT ( 'NONE',  ( -5.756513278485710927, 120.0202605514778185, 0.8483401204354447112 ) ) ;
#26142=CARTESIAN_POINT ( 'NONE',  ( 3.900846188197024667, 12.44727460162280863, 2.488979119290085862 ) ) ;
#26143=CARTESIAN_POINT ( 'NONE',  ( 18.04579964447621876, 154.0913862843578670, 1.474566393615006854 ) ) ;
#26144=CARTESIAN_POINT ( 'NONE',  ( -0.09221630143976956850, 107.6766875080336376, 4.614880812453268533 ) ) ;
#26146=CARTESIAN_POINT ( 'NONE',  ( 0.4301208033649062124, 117.9789173577105572, -0.5453690669796713575 ) ) ;
#26147=CARTESIAN_POINT ( 'NONE',  ( 4.309711357183296343, 3.151582320728117725, 1.677628897243969464 ) ) ;
#26148=CARTESIAN_POINT ( 'NONE',  ( -22.64839633469834013, 142.3612397021088611, -1.542087416992683924 ) ) ;
#26149=ORIENTED_EDGE ( 'NONE', *, *, #32316, .T. ) ;
#26150=CARTESIAN_POINT ( 'NONE',  ( -1.578387894090459653, 120.8584627942791627, 0.1358179495115143243 ) ) ;
#26151=EDGE_CURVE ( 'NONE', #24227, #23040, #2973, .T. ) ;
#26152=CARTESIAN_POINT ( 'NONE',  ( 5.858142917232623148, -13.84584594667595603, 2.526540219170608115 ) ) ;
#26153=FACE_OUTER_BOUND ( 'NONE', #24471, .T. ) ;
#26154=EDGE_CURVE ( 'NONE', #32528, #18094, #33400, .T. ) ;
#26155=CARTESIAN_POINT ( 'NONE',  ( -2.611003341877406125, 107.7052943677586967, -4.533873330392383494 ) ) ;
#26156=EDGE_LOOP ( 'NONE', ( #15718, #34942, #21199, #30163 ) ) ;
#26157=CARTESIAN_POINT ( 'NONE',  ( 19.13882315974079873, 148.9694856701144090, 2.502273048283856660 ) ) ;
#26159=FACE_OUTER_BOUND ( 'NONE', #29491, .T. ) ;
#26160=CARTESIAN_POINT ( 'NONE',  ( -5.858194661467491571, 117.3723397083485622, 0.4592760973624645526 ) ) ;
#26161=CARTESIAN_POINT ( 'NONE',  ( 3.265120802789828858, 159.4600617640778353, -0.2122772200314291535 ) ) ;
#26162=CARTESIAN_POINT ( 'NONE',  ( 3.682264917456192332, 91.53346620154573543, 0.07358041635424013294 ) ) ;
#26165=CARTESIAN_POINT ( 'NONE',  ( 2.085304100370665381, -15.07063515923644204, 5.677967908721369916 ) ) ;
#26168=CARTESIAN_POINT ( 'NONE',  ( -4.683796573410287323, 118.0096004882185809, 0.5957989904303049311 ) ) ;
#26171=CARTESIAN_POINT ( 'NONE',  ( -8.371648177948166847, 119.6424059396060215, -1.420761012106893650 ) ) ;
#26172=CARTESIAN_POINT ( 'NONE',  ( -7.588497335288529655, 124.2943531750336490, -0.1606663149101727195 ) ) ;
#26173=CARTESIAN_POINT ( 'NONE',  ( 4.829999151938469737, 117.7605300480266521, 0.9794162057613182704 ) ) ;
#26175=CARTESIAN_POINT ( 'NONE',  ( -10.62861998609546710, 124.7671305375842934, -1.166658412819147728 ) ) ;
#26176=CARTESIAN_POINT ( 'NONE',  ( -3.658446277643336852, 115.7029863456469769, -1.617048514123410108 ) ) ;
#26179=CARTESIAN_POINT ( 'NONE',  ( 5.597156320496667448, 117.9391977826196296, -0.5238424959023464389 ) ) ;
#26180=CARTESIAN_POINT ( 'NONE',  ( -16.96873827569995186, 146.4457527449227143, -1.929048950080525904 ) ) ;
#26183=CARTESIAN_POINT ( 'NONE',  ( -3.653537934457985692, 115.7029491755470900, 1.478493708770651560 ) ) ;
#26184=CARTESIAN_POINT ( 'NONE',  ( -15.76292520415746168, 145.9043202870795994, -0.2477380866161832118 ) ) ;
#26185=CARTESIAN_POINT ( 'NONE',  ( -1.251853189678833411, -4.679435864505671283, 4.458631606201990394 ) ) ;
#26186=CARTESIAN_POINT ( 'NONE',  ( 22.97411545401776323, 149.2143936249396461, 1.313106760764511272 ) ) ;
#26187=ORIENTED_EDGE ( 'NONE', *, *, #41797, .T. ) ;
#26188=DIRECTION ( 'NONE',  ( -0.9998004120163609398, 0.000000000000000000, -0.01997839162482749689 ) ) ;
#26189=CARTESIAN_POINT ( 'NONE',  ( 3.668568818830479028, -15.43917834477946727, 2.972162690469843049 ) ) ;
#26190=CARTESIAN_POINT ( 'NONE',  ( -6.044862153450532460, 157.1185343457808301, 1.711190705598350625 ) ) ;
#26191=CARTESIAN_POINT ( 'NONE',  ( 0.7602462924416659718, 13.52415170902173891, -0.6087277422976011820 ) ) ;
#26192=CARTESIAN_POINT ( 'NONE',  ( -23.13850227319436925, 149.2833505036244048, -1.057685438456114735 ) ) ;
#26193=CARTESIAN_POINT ( 'NONE',  ( 0.9725752971277935588, -10.50039532299128808, -0.08436647605774086345 ) ) ;
#26194=VERTEX_POINT ( 'NONE', #17018 ) ;
#26197=CARTESIAN_POINT ( 'NONE',  ( 4.713882987175320949, 112.7966860322829206, 2.559857038700545928 ) ) ;
#26200=CARTESIAN_POINT ( 'NONE',  ( -12.68314523066112365, 130.7634385742845780, 0.6346334167959437611 ) ) ;
#26201=CARTESIAN_POINT ( 'NONE',  ( 3.088592312018083152, -14.58504802601380490, 5.263618629775349333 ) ) ;
#26202=CARTESIAN_POINT ( 'NONE',  ( 12.17146470397773683, 153.5325627063460843, -1.540419412064476079 ) ) ;
#26203=CARTESIAN_POINT ( 'NONE',  ( -11.23789960528901233, 121.3367100885591015, -1.694033198309415900 ) ) ;
#26206=CARTESIAN_POINT ( 'NONE',  ( 2.681353593581013328, -14.83682625404381028, 4.634604895792218571 ) ) ;
#26207=CARTESIAN_POINT ( 'NONE',  ( -3.326449069927084778, 34.44917962613040885, 2.810111972534369507 ) ) ;
#26208=CARTESIAN_POINT ( 'NONE',  ( 15.28485850284622494, 148.0141687878753203, 0.07717638215565311710 ) ) ;
#26209=EDGE_LOOP ( 'NONE', ( #39776, #31556, #16563, #28942, #1028 ) ) ;
#26210=CARTESIAN_POINT ( 'NONE',  ( -3.441191703046090566, 108.4907222760747487, 4.068004305127732145 ) ) ;
#26211=CARTESIAN_POINT ( 'NONE',  ( 0.1714814745455566780, 105.9763118359762188, 5.301227498240227654 ) ) ;
#26214=CARTESIAN_POINT ( 'NONE',  ( 21.90070483041502669, 151.4392833230981239, 0.2858324510978372257 ) ) ;
#26215=CARTESIAN_POINT ( 'NONE',  ( -3.592701615362679846, 108.6576027043044377, 3.989964801148524476 ) ) ;
#26216=CARTESIAN_POINT ( 'NONE',  ( -0.5401806786426563978, 115.6909491485452435, 1.744860971564218932 ) ) ;
#26217=CARTESIAN_POINT ( 'NONE',  ( 4.560443952884764229, -11.68867000232777542, 0.6947937212093100445 ) ) ;
#26218=CARTESIAN_POINT ( 'NONE',  ( -2.234863377544184626, 32.75332796031084115, 0.9421588083577628892 ) ) ;
#26219=CARTESIAN_POINT ( 'NONE',  ( 20.99120442346846716, 145.7918284779248665, 2.367408383378774239 ) ) ;
#26220=AXIS2_PLACEMENT_3D ( 'NONE', #32750, #30378, #39568 ) ;
#26221=CARTESIAN_POINT ( 'NONE',  ( 1.072590735131739414, 20.86836736082219801, 4.503669761903479341 ) ) ;
#26222=CARTESIAN_POINT ( 'NONE',  ( -4.948315225313974608, -9.142465695005178361, 6.828157318318492486 ) ) ;
#26223=CARTESIAN_POINT ( 'NONE',  ( -8.718980399793466063, 118.0112729258643469, -0.7777409526643788151 ) ) ;
#26224=CARTESIAN_POINT ( 'NONE',  ( -3.231038154352895653, 124.0549386377059307, -0.1153833196696141400 ) ) ;
#26227=CARTESIAN_POINT ( 'NONE',  ( -1.754637834204752389, 104.6144662015456674, 4.496842749848052101 ) ) ;
#26228=CARTESIAN_POINT ( 'NONE',  ( 3.121479725567877228, 16.06095178295013071, 3.416230322513892137 ) ) ;
#26229=CYLINDRICAL_SURFACE ( 'NONE', #10317, 0.5080000000000002292 ) ;
#26231=CARTESIAN_POINT ( 'NONE',  ( 2.904419875024614850, -13.46177902185440090, 0.8499660341922408158 ) ) ;
#26232=CARTESIAN_POINT ( 'NONE',  ( 3.159661387648420305, 123.6198120039584154, -0.01957516827081329930 ) ) ;
#26233=CARTESIAN_POINT ( 'NONE',  ( -22.94521658075157333, 142.4877946823990271, 0.4044642804735134600 ) ) ;
#26236=VERTEX_POINT ( 'NONE', #21044 ) ;
#26238=CARTESIAN_POINT ( 'NONE',  ( 3.432040476525267891, -15.74971700692714904, 4.939269227581224442 ) ) ;
#26239=CARTESIAN_POINT ( 'NONE',  ( -17.80465198604245458, 131.6735282812448986, 1.559227381006987434 ) ) ;
#26240=CARTESIAN_POINT ( 'NONE',  ( 18.33177592110327225, 128.6097515361309149, -1.108544906447614720 ) ) ;
#26241=CARTESIAN_POINT ( 'NONE',  ( 0.7007450612751181529, 9.901275517365906609, -4.597291952374415125 ) ) ;
#26245=CARTESIAN_POINT ( 'NONE',  ( 2.157690779482308585, 123.3349985135950959, 0.1620144005770982609 ) ) ;
#26247=CARTESIAN_POINT ( 'NONE',  ( -8.008548551000092885, 121.6949282028273132, 0.7800530928440457812 ) ) ;
#26249=CARTESIAN_POINT ( 'NONE',  ( 0.9814465556259852619, 157.4778559999684830, -1.561959177316861958 ) ) ;
#26250=CARTESIAN_POINT ( 'NONE',  ( 0.01081828485855210013, 118.1092738308834669, -0.5413912121690738211 ) ) ;
#26253=CARTESIAN_POINT ( 'NONE',  ( 4.547657880063963098, 118.1104688511466918, -0.5057482797829222498 ) ) ;
#26254=CARTESIAN_POINT ( 'NONE',  ( 15.92216882203259232, 147.6644253265642135, -0.6463398217596317830 ) ) ;
#26255=AXIS2_PLACEMENT_3D ( 'NONE', #25569, #21725, #2174 ) ;
#26257=CARTESIAN_POINT ( 'NONE',  ( -16.55051581791506621, 149.4842840675632658, -2.199106316832546870 ) ) ;
#26258=CARTESIAN_POINT ( 'NONE',  ( 3.375754317642519098, -15.02680299829225952, 2.760009546110721246 ) ) ;
#26259=CYLINDRICAL_SURFACE ( 'NONE', #41547, 3.175000000000001155 ) ;
#26261=CARTESIAN_POINT ( 'NONE',  ( 3.679437910380295218, 2.726752568732802917, 2.794697870780981752 ) ) ;
#26262=CARTESIAN_POINT ( 'NONE',  ( 15.22212811258876108, 150.6904849259475441, 2.083262412922771922 ) ) ;
#26263=CARTESIAN_POINT ( 'NONE',  ( 2.026275176938348910, 36.00229031759788256, -0.4369541009056890912 ) ) ;
#26264=CARTESIAN_POINT ( 'NONE',  ( -1.471791394198959102, 24.03230288535706549, 4.399545648925609065 ) ) ;
#26265=CARTESIAN_POINT ( 'NONE',  ( 9.288927291931040386, 124.2653519604415067, 0.3477528771403741170 ) ) ;
#26266=CARTESIAN_POINT ( 'NONE',  ( -1.176016126184881161, 105.9610483257683313, 5.207556883177536733 ) ) ;
#26269=CARTESIAN_POINT ( 'NONE',  ( -5.561639213138736437, 116.7025976473698563, -0.1964723455066371971 ) ) ;
#26270=DIRECTION ( 'NONE',  ( 0.9998004120163608288, 0.000000000000000000, 0.01997839162482760791 ) ) ;
#26280=CARTESIAN_POINT ( 'NONE',  ( -16.00576599164912750, 121.2237126890796191, -0.08595866332889588735 ) ) ;
#26281=TOROIDAL_SURFACE ( 'NONE', #18798, 5.080000000000005400, 0.5080000000000000071 ) ;
#26282=VERTEX_POINT ( 'NONE', #33651 ) ;
#26284=CARTESIAN_POINT ( 'NONE',  ( 7.804305114750069272, 122.5549487891343574, -0.07597547369942431184 ) ) ;
#26287=CARTESIAN_POINT ( 'NONE',  ( -1.617373050801775625, 120.9968702744464366, -0.03231896268895485813 ) ) ;
#26288=CARTESIAN_POINT ( 'NONE',  ( 4.135482704272881449, -14.73569165307708673, 5.015242562682193039 ) ) ;
#26289=CARTESIAN_POINT ( 'NONE',  ( -1.228124343681062047, 158.9035955689636523, 1.375095950729814165 ) ) ;
#26290=CARTESIAN_POINT ( 'NONE',  ( -3.130497002865707756, 23.39511390029671745, 3.426874451367011520 ) ) ;
#26291=CARTESIAN_POINT ( 'NONE',  ( 15.91552649980314627, 121.2232988859741027, 0.6415868299260654162 ) ) ;
#26292=CARTESIAN_POINT ( 'NONE',  ( 2.163718758107066709, -15.46264904772556825, 5.921791837560038907 ) ) ;
#26293=CARTESIAN_POINT ( 'NONE',  ( 5.276310133815047543, 115.6909491485453145, -0.8120701714742106780 ) ) ;
#26294=CARTESIAN_POINT ( 'NONE',  ( 0.4358653558703468045, -2.730035452555519271, 0.8728101606764442355 ) ) ;
#26295=CARTESIAN_POINT ( 'NONE',  ( -18.61947985292905017, 154.1412379532633850, -0.5163013828871974020 ) ) ;
#26296=CARTESIAN_POINT ( 'NONE',  ( -4.743925087698587006, 117.9014421663514725, 0.7646676084295724873 ) ) ;
#26299=CARTESIAN_POINT ( 'NONE',  ( 8.781532007625042269, 117.7401941391528624, 0.4292495202309390967 ) ) ;
#26301=CARTESIAN_POINT ( 'NONE',  ( -14.02613073054681614, 152.5802402909829425, 1.631301951249305215 ) ) ;
#26303=CARTESIAN_POINT ( 'NONE',  ( 6.782271978584973660, 118.5360090424673274, 1.159066879843025255 ) ) ;
#26304=CARTESIAN_POINT ( 'NONE',  ( 0.03212618750947002916, 158.2819368290249713, -1.607725792532325171 ) ) ;
#26305=CARTESIAN_POINT ( 'NONE',  ( 0.1234711523483410095, 5.102374915558315571, -0.9659065422363407594 ) ) ;
#26306=CARTESIAN_POINT ( 'NONE',  ( -21.62407820142113835, 149.9601031839316079, -2.013249247985050339 ) ) ;
#26307=CARTESIAN_POINT ( 'NONE',  ( 4.595251882992044123, 118.0172796872295891, -0.6951473410461010971 ) ) ;
#26310=EDGE_CURVE ( 'NONE', #27898, #35651, #22010, .T. ) ;
#26311=CARTESIAN_POINT ( 'NONE',  ( 10.37991283549660437, 123.8962982355681817, -0.8252603836154487338 ) ) ;
#26312=CARTESIAN_POINT ( 'NONE',  ( -14.17939111974024335, 138.8817910697950140, -0.2325274008182653396 ) ) ;
#26313=EDGE_LOOP ( 'NONE', ( #14998, #36061 ) ) ;
#26314=CARTESIAN_POINT ( 'NONE',  ( 0.03212616895145502249, 157.6269964811067155, -1.607724863813388971 ) ) ;
#26315=CARTESIAN_POINT ( 'NONE',  ( 3.900291174488768053, -15.73247852219369847, 4.461464635514134969 ) ) ;
#26317=DIRECTION ( 'NONE',  ( -5.206863593109713661E-17, 1.000000000000000000, -1.077750396879097183E-30 ) ) ;
#26321=CARTESIAN_POINT ( 'NONE',  ( 13.34752792037768820, 125.8771108566470502, 1.915935069336977659 ) ) ;
#26323=CARTESIAN_POINT ( 'NONE',  ( 4.910479103859797689, 115.7029491485453008, 1.454559715794871089 ) ) ;
#26324=CARTESIAN_POINT ( 'NONE',  ( -0.2179432916433551026, 106.0530876078258586, 5.262233728842789837 ) ) ;
#26325=CARTESIAN_POINT ( 'NONE',  ( -8.190863557275731566, 21.65400946394957060, -2.068261358883292989 ) ) ;
#26326=CARTESIAN_POINT ( 'NONE',  ( 9.364230102553010582, 123.8909350679826815, 0.6996930829695083842 ) ) ;
#26327=CARTESIAN_POINT ( 'NONE',  ( 0.3541790919670912419, 116.9919054422455531, -0.3273860145854423642 ) ) ;
#26328=DIRECTION ( 'NONE',  ( 0.1538365266688606903, -0.9876883405951383255, 0.02839128237474894401 ) ) ;
#26332=CARTESIAN_POINT ( 'NONE',  ( -8.217303172778619214, 117.5015518944296247, -0.1195796404652190448 ) ) ;
#26334=CARTESIAN_POINT ( 'NONE',  ( 6.675603198613333511, 120.7516070878810410, -0.8047696622842539504 ) ) ;
#26335=CARTESIAN_POINT ( 'NONE',  ( 6.242199107252148771, -13.90286925626189252, 1.333809230853582273 ) ) ;
#26337=CARTESIAN_POINT ( 'NONE',  ( -15.38106487260184529, 148.0444422243178337, -0.8962548396073235502 ) ) ;
#26338=CARTESIAN_POINT ( 'NONE',  ( 3.948573903914379457, -12.48127506095717010, 1.805458641749257520 ) ) ;
#26339=CARTESIAN_POINT ( 'NONE',  ( -16.02745508617906012, 155.1095016151506911, 1.019363059911538860 ) ) ;
#26341=CARTESIAN_POINT ( 'NONE',  ( 0.2950350728689354329, 116.4333835968663919, 0.04389667002116236227 ) ) ;
#26342=EDGE_LOOP ( 'NONE', ( #41942, #36284, #10790, #37351, #23627 ) ) ;
#26343=CARTESIAN_POINT ( 'NONE',  ( 4.636249899789679496, -11.37698174978397958, -0.2454043791197063895 ) ) ;
#26344=CARTESIAN_POINT ( 'NONE',  ( -23.42514220146296111, 142.8382549601284097, -0.4680900899253088721 ) ) ;
#26346=CARTESIAN_POINT ( 'NONE',  ( 1.217703060157562689, 106.0679358989203536, 5.195502566823263280 ) ) ;
#26348=CARTESIAN_POINT ( 'NONE',  ( 6.997741591014696283, 121.4429130386087934, 0.8574795444661736932 ) ) ;
#26349=CARTESIAN_POINT ( 'NONE',  ( -2.972019672840211513, 9.848453565018933986, 3.538668892428941781 ) ) ;
#26350=CARTESIAN_POINT ( 'NONE',  ( 19.95201466422899728, 152.4248492066682559, 1.669502467017324854 ) ) ;
#26353=CARTESIAN_POINT ( 'NONE',  ( 12.06131655867242713, 120.6765805525287334, -1.069212010736125817 ) ) ;
#26354=CARTESIAN_POINT ( 'NONE',  ( 3.235533175430977515, 2.501875212487111977, 3.308963532380430284 ) ) ;
#26355=CARTESIAN_POINT ( 'NONE',  ( -15.26873630740966270, 121.3917326167944708, -1.149126527656483043 ) ) ;
#26356=EDGE_CURVE ( 'NONE', #9715, #9538, #13175, .T. ) ;
#26357=ORIENTED_EDGE ( 'NONE', *, *, #20613, .F. ) ;
#26359=CARTESIAN_POINT ( 'NONE',  ( -15.60869185768510903, 147.5518517437054982, 0.1389895172399198409 ) ) ;
#26360=CARTESIAN_POINT ( 'NONE',  ( 5.456921283009238621, -14.23391906346564717, 3.426434758229824240 ) ) ;
#26361=MECHANICAL_DESIGN_GEOMETRIC_PRESENTATION_REPRESENTATION('',(#21570),#39329);
#26362=CARTESIAN_POINT ( 'NONE',  ( -3.278664548829097747, 108.1634672882638029, -4.198944545392978789 ) ) ;
#26365=CARTESIAN_POINT ( 'NONE',  ( 13.83536887852627650, 154.2684476645699760, 2.291766773079779718 ) ) ;
#26368=CARTESIAN_POINT ( 'NONE',  ( -22.55548643167962197, 142.2972183020237367, 0.7396483830486686450 ) ) ;
#26369=CARTESIAN_POINT ( 'NONE',  ( 2.538140519494355374, 21.06397054095828381, 8.048466014368985455 ) ) ;
#26371=CARTESIAN_POINT ( 'NONE',  ( 1.406537315630064677, 159.5914066142653098, -0.2310332007158441836 ) ) ;
#26375=CARTESIAN_POINT ( 'NONE',  ( 1.859021851459260022, -15.10376415035639930, 5.547171369656321183 ) ) ;
#26380=CARTESIAN_POINT ( 'NONE',  ( -4.603251683469835598, 118.0757897185588234, 0.5233029099187971322 ) ) ;
#26385=CARTESIAN_POINT ( 'NONE',  ( -3.841645322271367569, 119.0006533405734928, -0.9283627247572711072 ) ) ;
#26386=CARTESIAN_POINT ( 'NONE',  ( -6.689329653978204782, 121.2318545172250737, -0.3418430003135978779 ) ) ;
#26387=CARTESIAN_POINT ( 'NONE',  ( 4.437541795254049681, 118.1257943510456840, 0.7326559301581485606 ) ) ;
#26388=CARTESIAN_POINT ( 'NONE',  ( -7.769844292200057012, 122.1031240515655298, -0.8163738826679363125 ) ) ;
#26390=CARTESIAN_POINT ( 'NONE',  ( -1.801924311864099293, 115.7029148620384404, -1.722817892843705234 ) ) ;
#26392=CARTESIAN_POINT ( 'NONE',  ( 1.138070077757084686, 117.9496053113818448, -1.345098318217916811 ) ) ;
#26393=CARTESIAN_POINT ( 'NONE',  ( 5.774381877465427415, 118.4424948052634647, -0.4329097047088598660 ) ) ;
#26394=CARTESIAN_POINT ( 'NONE',  ( -16.78017617680123763, 148.3581316477378493, -2.036619618061130677 ) ) ;
#26395=CARTESIAN_POINT ( 'NONE',  ( 5.304438957985845526, 116.0444662015456885, -1.082911341041116637 ) ) ;
#26396=CARTESIAN_POINT ( 'NONE',  ( -0.01443894962468954962, 159.4760848062415732, 0.7225840825867287931 ) ) ;
#26397=CARTESIAN_POINT ( 'NONE',  ( 8.675687895398256799, 118.3610464811750802, -0.6699752535086603844 ) ) ;
#26398=CARTESIAN_POINT ( 'NONE',  ( -15.38177525964082371, 147.8337523264461879, -0.2407145083428142707 ) ) ;
#26399=CARTESIAN_POINT ( 'NONE',  ( -1.861891798414337940, 1.167894131763866250, -4.247245584637167504 ) ) ;
#26400=CARTESIAN_POINT ( 'NONE',  ( 22.68171885890631145, 150.0520759213295889, 1.302983692151378436 ) ) ;
#26402=CARTESIAN_POINT ( 'NONE',  ( 2.102798109511007318, -15.25784609616889753, 5.176374340497880588 ) ) ;
#26403=CARTESIAN_POINT ( 'NONE',  ( -11.96109417309370748, 154.9039014673913073, 1.746238851223627986 ) ) ;
#26404=CARTESIAN_POINT ( 'NONE',  ( -0.4136891606132181431, 9.424461778640809584, 0.8817368238460310259 ) ) ;
#26405=CARTESIAN_POINT ( 'NONE',  ( -20.06391502460639842, 128.8637844977697569, -0.9116527748870052461 ) ) ;
#26407=CARTESIAN_POINT ( 'NONE',  ( -0.8351715869602673870, 27.76506109569598024, 0.5290732382595327854 ) ) ;
#26411=CARTESIAN_POINT ( 'NONE',  ( 7.065765265293006969, 122.4340714744230496, 0.2508917249367682567 ) ) ;
#26413=CARTESIAN_POINT ( 'NONE',  ( -0.01341678693510457362, 156.4123495908283985, 0.6714308817992611367 ) ) ;
#26414=CARTESIAN_POINT ( 'NONE',  ( 2.161572811135036964, -15.02537755669194830, 5.771884496758437066 ) ) ;
#26415=CARTESIAN_POINT ( 'NONE',  ( 16.62515567699070473, 149.4842840675632658, -1.536177446654198198 ) ) ;
#26416=CARTESIAN_POINT ( 'NONE',  ( -19.42145995676313674, 149.0830822498907082, -2.502058577541587336 ) ) ;
#26418=CARTESIAN_POINT ( 'NONE',  ( 2.766857707386623400, -13.29092698609396450, 0.4080254275553683585 ) ) ;
#26419=CARTESIAN_POINT ( 'NONE',  ( -0.5146975708209950984, 37.55987809028739832, 0.05064662351078883656 ) ) ;
#26420=CARTESIAN_POINT ( 'NONE',  ( 1.606403942294383214, 120.9755568995931156, -0.03214495494220263178 ) ) ;
#26422=CARTESIAN_POINT ( 'NONE',  ( -5.278861607444886417, 115.7725975576095720, 0.7828656677038698941 ) ) ;
#26427=ADVANCED_FACE ( 'NONE', ( #20204 ), #14993, .F. ) ;
#26428=CARTESIAN_POINT ( 'NONE',  ( 3.292377373361659920, 159.4686222989141697, -0.02724393823342678017 ) ) ;
#26430=CARTESIAN_POINT ( 'NONE',  ( -3.580579253266132689, 108.6681208952157078, 3.986884027299105071 ) ) ;
#26432=DIRECTION ( 'NONE',  ( 0.9998004120163609398, 0.000000000000000000, 0.01997839162482749689 ) ) ;
#26434=CARTESIAN_POINT ( 'NONE',  ( -3.328555392133318858, 33.88165127674241717, 1.160568618710268618 ) ) ;
#26435=CARTESIAN_POINT ( 'NONE',  ( 13.08065502438826400, 121.7804325175133755, 1.718327614618424315 ) ) ;
#26436=CARTESIAN_POINT ( 'NONE',  ( 4.353980591602404360, 23.44215234368072487, -1.583070106892425111 ) ) ;
#26437=CARTESIAN_POINT ( 'NONE',  ( -6.911983299595774177, -11.51556667111630894, -4.837919318831837678 ) ) ;
#26438=CARTESIAN_POINT ( 'NONE',  ( -5.493189927730356636, 117.6942598834481686, -1.012164059239212710 ) ) ;
#26439=CARTESIAN_POINT ( 'NONE',  ( -1.569662112149406763, 118.6366899268033279, -0.8670489899392761490 ) ) ;
#26442=CARTESIAN_POINT ( 'NONE',  ( 2.143370549553493820, 105.1244188156866954, 4.894740234150261493 ) ) ;
#26443=CARTESIAN_POINT ( 'NONE',  ( -2.755274729907521980, 20.69627551736597226, -3.746277899328600558 ) ) ;
#26444=EDGE_CURVE ( 'NONE', #24193, #32067, #4444, .T. ) ;
#26447=CARTESIAN_POINT ( 'NONE',  ( 2.237742905438162122, -15.06201634873256801, 5.120316289255383069 ) ) ;
#26448=CARTESIAN_POINT ( 'NONE',  ( 1.980194564007054403, 113.2583846565721757, -2.436415359710689010 ) ) ;
#26449=CARTESIAN_POINT ( 'NONE',  ( -22.47867321467015955, 150.2745577238280816, 0.5153050491938901967 ) ) ;
#26452=VERTEX_POINT ( 'NONE', #8070 ) ;
#26455=CARTESIAN_POINT ( 'NONE',  ( -6.065440317703094664, 31.08949202354850172, -0.5906148415105061389 ) ) ;
#26456=CARTESIAN_POINT ( 'NONE',  ( 5.620948709224020234, -15.12563517700941951, 1.754161952847088868 ) ) ;
#26457=CARTESIAN_POINT ( 'NONE',  ( -19.51325853822230272, 141.0981142166620259, 1.725252114789138647 ) ) ;
#26458=CARTESIAN_POINT ( 'NONE',  ( 14.13727225732671222, 121.3807765770047666, -0.9276936697596736003 ) ) ;
#26459=CARTESIAN_POINT ( 'NONE',  ( 0.8332047475417917459, 28.58290516567101491, -0.5069163209656499802 ) ) ;
#26462=CARTESIAN_POINT ( 'NONE',  ( -4.918661145027864556, 117.4102335145295370, -1.102851133234106662 ) ) ;
#26463=CARTESIAN_POINT ( 'NONE',  ( 0.9302644990744406428, 122.9246775559910390, 0.2070653534288171282 ) ) ;
#26464=CARTESIAN_POINT ( 'NONE',  ( -1.452025732293910965, 120.0849730816093910, 0.4508766852696775573 ) ) ;
#26466=CIRCLE ( 'NONE', #12204, 0.5080000000000002292 ) ;
#26467=CARTESIAN_POINT ( 'NONE',  ( 3.371641211477126809, 119.4525916976722897, -0.7211689390744320249 ) ) ;
#26468=CLOSED_SHELL ( 'NONE', ( #31779, #31356, #33394, #18032, #9713, #26896, #8217, #41483, #35482, #41130, #9677, #1171, #35220, #7225, #40741, #203, #20395, #39138, #13159, #9295, #17291, #30443, #36318, #36557, #39305, #27934, #14109, #5649, #29091, #17502, #12537, #28721, #40774, #22283, #27883, #29577, #24791, #11840, #40165, #24016, #25653, #31400, #23843, #638, #41265, #39151, #17733, #164, #18451, #13367, #13029, #21097, #24609, #21175, #20126, #4757, #11479, #13669, #9558, #1165, #7417, #3413, #41854, #29217, #36751, #24292, #13855, #24646, #8760, #5585, #4780, #3524, #31284, #32963, #6343, #21619, #37651, #33468, #5305, #19106, #18806, #6130, #38583, #5346, #12117, #33142, #9912, #29741, #34515, #11817, #17212, #21958, #24653, #15933, #28088, #3579, #31087, #11268, #40459, #9956, #21154, #28981, #25064, #28253, #17453, #19079, #26427, #21955, #39844, #35027, #36026, #6785, #11527, #17966, #10221, #9503, #32551, #5128, #6983, #11486, #28517, #5609, #23002, #30769, #12171, #41817, #13338, #15984, #15710, #9458, #5876, #34713, #403, #30815, #24515, #12629, #19637, #30039, #24083, #35288, #8163, #21705, #17197, #4537, #16573, #20178, #16173, #2699, #23752, #17259, #3444, #4814, #20321, #39627, #2984, #38653, #12859, #12831, #20070, #15804, #4724 ) ) ;
#26469=CARTESIAN_POINT ( 'NONE',  ( -3.096092393557038580, 118.0390668470448929, -0.8277768005040341270 ) ) ;
#26472=CARTESIAN_POINT ( 'NONE',  ( 4.507247720737455943, 118.1170994507041030, -0.5526904508501585545 ) ) ;
#26473=CARTESIAN_POINT ( 'NONE',  ( 9.439557112687584350, 123.9587481073520223, -0.3264598115655270028 ) ) ;
#26475=CARTESIAN_POINT ( 'NONE',  ( -7.267393677827440612, 155.8804291298944236, -1.807016794997827525 ) ) ;
#26476=CARTESIAN_POINT ( 'NONE',  ( 2.678036876842718517, -15.12020262989130437, 4.533791366373512766 ) ) ;
#26477=CARTESIAN_POINT ( 'NONE',  ( 1.165615098987396347, 105.1232203586557290, -5.215136134052268169 ) ) ;
#26479=CARTESIAN_POINT ( 'NONE',  ( -3.586339569854333664, 7.474549112184490696, -2.913498476264247294 ) ) ;
#26480=CARTESIAN_POINT ( 'NONE',  ( 5.103418814394237835, 120.3680889145531552, 0.8767301089910152223 ) ) ;
#26481=CARTESIAN_POINT ( 'NONE',  ( 2.979675570102178650, 39.20946620154573026, 0.2712499303477601820 ) ) ;
#26482=CARTESIAN_POINT ( 'NONE',  ( 4.513502956352341222, 8.064680226961385756, -0.9949261897555528034 ) ) ;
#26483=CARTESIAN_POINT ( 'NONE',  ( -0.001255909994615970462, 120.9722815239556439, 0.06285087176068887560 ) ) ;
#26485=EDGE_CURVE ( 'NONE', #19701, #10361, #36950, .T. ) ;
#26488=CARTESIAN_POINT ( 'NONE',  ( -2.183972911347295209, 116.1856571598952144, -0.06668066542220674187 ) ) ;
#26489=CARTESIAN_POINT ( 'NONE',  ( 18.63504953328963154, 154.1157618415863624, 0.3723726386282266709 ) ) ;
#26494=EDGE_CURVE ( 'NONE', #17488, #17144, #36802, .T. ) ;
#26499=CARTESIAN_POINT ( 'NONE',  ( -3.792432603185484474, 116.7736770086926867, 0.1904249565637312347 ) ) ;
#26502=CARTESIAN_POINT ( 'NONE',  ( -6.044933042564573533, 121.4357306406764252, -0.1374383516041701447 ) ) ;
#26504=CARTESIAN_POINT ( 'NONE',  ( 4.825036788390894671, 62.83146620154573014, 0.09641571798141751470 ) ) ;
#26505=CARTESIAN_POINT ( 'NONE',  ( -9.106973723525666031, 153.9337724597031070, -0.2264262902970467783 ) ) ;
#26506=CARTESIAN_POINT ( 'NONE',  ( 5.414172367154487908, -13.81390647261572546, 3.268633212004894872 ) ) ;
#26507=CARTESIAN_POINT ( 'NONE',  ( -21.26977539036090548, 145.8710773725474610, 1.472442194194814702 ) ) ;
#26508=CARTESIAN_POINT ( 'NONE',  ( 4.619096255015035624, 27.05588869245799089, -0.3994036469054788596 ) ) ;
#26509=CARTESIAN_POINT ( 'NONE',  ( 16.76609992697660800, 155.2615993841311877, 0.7433399007605487885 ) ) ;
#26510=CARTESIAN_POINT ( 'NONE',  ( 2.125773701607508226, -15.49174028809012427, 5.936015161737096868 ) ) ;
#26511=CARTESIAN_POINT ( 'NONE',  ( -4.349660437102230048, 31.17966527223318707, -1.615541842050199461 ) ) ;
#26512=CARTESIAN_POINT ( 'NONE',  ( 0.8097498057273965211, -0.1318080948593848278, -0.5455758836208917106 ) ) ;
#26513=CARTESIAN_POINT ( 'NONE',  ( -23.27880353394132484, 149.3453998935430604, -0.6192278183506784162 ) ) ;
#26515=CARTESIAN_POINT ( 'NONE',  ( 4.936888680085094627, 117.4097579285739954, 1.082126315060445876 ) ) ;
#26516=CARTESIAN_POINT ( 'NONE',  ( 5.537423627294297823, 116.8704610243493107, 0.5072075918636228531 ) ) ;
#26518=CARTESIAN_POINT ( 'NONE',  ( -17.52489820599672399, 148.6234142586927476, 1.577473031907404843 ) ) ;
#26519=B_SPLINE_CURVE_WITH_KNOTS ( 'NONE', 3,
 ( #24054, #13846, #26844, #7887, #23842, #4285, #30242, #1082, #36864, #20849, #33874, #7680, #20639, #33669, #20017, #5749, #38109, #40683, #40482, #18489, #37469, #25106, #28305, #11475, #34085, #21466, #41311, #8925, #12116, #27673, #40889, #8508, #21059, #2125, #18701, #2342, #15087, #31495, #34294, #15299, #37267, #21263, #24464, #8294, #18280, #5122, #18075, #37893, #21890, #11692, #31077, #28089, #34919, #1916, #14878, #27880, #31712, #5327, #24677, #2553, #15514, #11276, #37686, #34497, #8086, #41100, #31281, #8717, #11906, #34703, #24895, #24260, #21679, #4913, #17867, #5532, #30868, #1713, #14668, #25316, #25935, #2759, #22723, #28516, #15715 ),
 .UNSPECIFIED., .F., .F.,
 ( 4, 2, 2, 1, 1, 1, 1, 2, 2, 2, 1, 2, 2, 2, 2, 1, 1, 1, 2, 2, 2, 2, 1, 1, 1, 1, 2, 2, 2, 2, 1, 1, 2, 2, 2, 2, 2, 2, 2, 2, 2, 2, 2, 1, 2, 2, 2, 2, 2, 4 ),
 ( 0.000000000000000000, 0.1250000000000123512, 0.1875000000000185407, 0.2187500000000216216, 0.2343750000000231482, 0.2421875000000239253, 0.2460937500000243139, 0.2480468750000243139, 0.2500000000000243139, 0.3125000000000244804, 0.3437500000000247025, 0.3593750000000248135, 0.3750000000000248690, 0.4375000000000253686, 0.4687500000000257017, 0.4843750000000259792, 0.4921875000000259792, 0.4960937500000259792, 0.4980468750000258682, 0.5000000000000256462, 0.5625000000000250910, 0.5937500000000248690, 0.6093750000000248690, 0.6171875000000250910, 0.6210937500000254241, 0.6230468750000255351, 0.6240234375000253131, 0.6250000000000252021, 0.6875000000000200950, 0.7187500000000175415, 0.7343750000000163203, 0.7421875000000157652, 0.7460937500000154321, 0.7500000000000150990, 0.7812500000000131006, 0.7968750000000121014, 0.8125000000000111022, 0.8281250000000101030, 0.8359375000000096589, 0.8398437500000094369, 0.8437500000000093259, 0.8593750000000084377, 0.8671875000000079936, 0.8710937500000077716, 0.8730468750000076605, 0.8750000000000075495, 0.9062500000000056621, 0.9218750000000046629, 0.9375000000000037748, 1.000000000000000000 ),
 .UNSPECIFIED. ) ;
#26521=CARTESIAN_POINT ( 'NONE',  ( 16.78381336521968237, 153.6818489539412553, 2.151947388239847214 ) ) ;
#26522=CARTESIAN_POINT ( 'NONE',  ( 17.85428843624163520, 135.5811125208551857, -1.719929978336786291 ) ) ;
#26523=CARTESIAN_POINT ( 'NONE',  ( -0.9497947497622778457, -2.244019015280241280, -0.2169513509177584398 ) ) ;
#26524=CARTESIAN_POINT ( 'NONE',  ( 0.008945125900382298184, 117.5133074443058945, -0.4476506782301715726 ) ) ;
#26525=CARTESIAN_POINT ( 'NONE',  ( 4.547353028811151887, 118.0891687680434359, -0.5919780852068863286 ) ) ;
#26528=CARTESIAN_POINT ( 'NONE',  ( 5.181828529332998201, 120.8264575521020987, -0.4749581527667975922 ) ) ;
#26529=CARTESIAN_POINT ( 'NONE',  ( -1.572870384098571162, 156.2570369995211479, 0.04660437260867185405 ) ) ;
#26530=ORIENTED_EDGE ( 'NONE', *, *, #9615, .T. ) ;
#26531=CARTESIAN_POINT ( 'NONE',  ( 0.01111639999512560942, 119.1634951276629550, -0.5563101126475826774 ) ) ;
#26533=CARTESIAN_POINT ( 'NONE',  ( 3.313323393711395948, -15.78004832563367721, 4.785553473879357256 ) ) ;
#26535=CARTESIAN_POINT ( 'NONE',  ( -4.989370312398730078, 31.45840840832646990, -0.6923657333659851698 ) ) ;
#26536=CARTESIAN_POINT ( 'NONE',  ( -4.508402063874162202, 118.0683172002946861, -0.8182161505956602188 ) ) ;
#26538=CARTESIAN_POINT ( 'NONE',  ( 4.149473596290089716, 118.2393519115161382, 0.3953539362545949176 ) ) ;
#26539=CARTESIAN_POINT ( 'NONE',  ( 7.646026353518021068, 156.1362479297160348, 1.963328325631339411 ) ) ;
#26540=DIRECTION ( 'NONE',  ( -0.9998004120163610509, -5.205824365704083805E-17, -0.01997839162482764261 ) ) ;
#26541=CARTESIAN_POINT ( 'NONE',  ( 9.822473411059192472, 117.9943479623217399, 0.1962763949404991992 ) ) ;
#26542=CARTESIAN_POINT ( 'NONE',  ( 8.403146708066456583, 17.13307930518084632, 0.5673920214783956251 ) ) ;
#26543=CARTESIAN_POINT ( 'NONE',  ( 3.002817136647192964, 156.1079525116674631, 0.5547493173044987236 ) ) ;
#26544=CARTESIAN_POINT ( 'NONE',  ( 22.85738479169573978, 148.8343141121478652, -0.6244747819152590695 ) ) ;
#26547=CARTESIAN_POINT ( 'NONE',  ( 0.3649948940937479125, 118.7629491485454025, 1.279691011652545285 ) ) ;
#26549=CARTESIAN_POINT ( 'NONE',  ( -21.67502463668058255, 132.7302833492884417, -0.4113505826877427718 ) ) ;
#26551=CARTESIAN_POINT ( 'NONE',  ( 5.481075915974320978, 120.6674672184742008, -0.5362211561704884888 ) ) ;
#26552=CARTESIAN_POINT ( 'NONE',  ( -8.730044398489210877, 118.0746546384499140, 0.4875147713271164585 ) ) ;
#26553=CARTESIAN_POINT ( 'NONE',  ( -9.378755113003734323, 124.2036136473707018, -0.5113998741172592899 ) ) ;
#26554=CARTESIAN_POINT ( 'NONE',  ( 4.181132250215417123, -13.15738584483822038, 3.071181452022354819 ) ) ;
#26555=CARTESIAN_POINT ( 'NONE',  ( -14.85424080674767211, 121.7713424311148032, 0.8456621969668064454 ) ) ;
#26557=CARTESIAN_POINT ( 'NONE',  ( 13.43562511198101994, 156.9186530619738562, 0.2898375456858041654 ) ) ;
#26559=CARTESIAN_POINT ( 'NONE',  ( -0.2095918955067871126, -8.989892990265463624, -4.636818132431064221 ) ) ;
#26560=CARTESIAN_POINT ( 'NONE',  ( -21.68875320759065062, 132.7412702629105468, -0.4333929054516006962 ) ) ;
#26563=CARTESIAN_POINT ( 'NONE',  ( -6.754070470910083834, 120.2528407669736765, 0.9389083524474073350 ) ) ;
#26564=CARTESIAN_POINT ( 'NONE',  ( 2.990331240142678038, -7.206181497205274233, 3.547999066060627094 ) ) ;
#26565=CARTESIAN_POINT ( 'NONE',  ( 2.946415863238953214, 117.2422168882539211, 0.6071713939981751018 ) ) ;
#26567=CARTESIAN_POINT ( 'NONE',  ( -6.538677740023618411E-14, 75.27746620154573520, -7.356392042280733227E-18 ) ) ;
#26568=CARTESIAN_POINT ( 'NONE',  ( 0.02969037535068312292, 158.7301711276701894, -1.485827791648137275 ) ) ;
#26569=CARTESIAN_POINT ( 'NONE',  ( -4.503669762702418033, -0.7216326387320324276, 1.072590735790061922 ) ) ;
#26570=CARTESIAN_POINT ( 'NONE',  ( -4.831157780894042908, 117.2114307359545649, -0.6331281246675557473 ) ) ;
#26572=CARTESIAN_POINT ( 'NONE',  ( -0.002455802209265526767, 120.8958299794632438, 0.1228983847502215371 ) ) ;
#26573=CARTESIAN_POINT ( 'NONE',  ( 2.850629920820032748, -15.47419331854960056, 5.714803783126763292 ) ) ;
#26576=CARTESIAN_POINT ( 'NONE',  ( -2.278603859588497205, 107.0255785817557665, -4.818371926714549502 ) ) ;
#26578=CARTESIAN_POINT ( 'NONE',  ( 11.81048985551409913, 122.0047285378078357, 1.760929439237068239 ) ) ;
#26581=CARTESIAN_POINT ( 'NONE',  ( -17.95360460524307555, 154.0540368679750998, 0.8775891217286384549 ) ) ;
#26582=CARTESIAN_POINT ( 'NONE',  ( 4.500746820419270655, 24.54286538861932598, -7.153999163526271410 ) ) ;
#26583=CARTESIAN_POINT ( 'NONE',  ( 15.92638198489182066, 148.2453349897154737, 1.585317681524597955 ) ) ;
#26585=CARTESIAN_POINT ( 'NONE',  ( 8.196853576809875364, 117.5993832199734328, -0.1745776481207346187 ) ) ;
#26594=CARTESIAN_POINT ( 'NONE',  ( -4.413217288059840371, 118.1641560473096888, 0.4831912002420357122 ) ) ;
#26596=B_SPLINE_SURFACE_WITH_KNOTS ( 'NONE', 1, 3, ( 
 ( #19604, #23003, #39222, #6640, #32616, #3449, #16626, #32832, #16412, #29418, #258, #36244, #36031, #26216, #7064, #13233, #32202, #6844 ),
 ( #19815, #3035, #3661, #20028, #33046, #16842, #29842, #680, #28326, #2574, #37488, #2360, #18721, #21487, #27899, #5345, #34103, #11924 ) ),
 .UNSPECIFIED., .F., .F., .F.,
 ( 2, 2 ),
 ( 4, 2, 2, 2, 2, 2, 2, 2, 4 ),
 ( 0.000000000000000000, 1.000000000000000000 ),
 ( 0.000000000000000000, 0.2500000000000000000, 0.5000000000000000000, 0.6250000000000000000, 0.7500000000000000000, 0.8125000000000000000, 0.8750000000000000000, 0.9375000000000000000, 1.000000000000000000 ),
 .UNSPECIFIED. ) ;
#26599=CARTESIAN_POINT ( 'NONE',  ( -3.864517893783868008, 119.0220221803404286, -0.9271182341797493676 ) ) ;
#26600=CARTESIAN_POINT ( 'NONE',  ( -1.973215784349786839, 106.6933082031156772, -4.964841027628618342 ) ) ;
#26601=TOROIDAL_SURFACE ( 'NONE', #40878, 4.826000000000000512, 0.5080000000000000071 ) ;
#26602=CARTESIAN_POINT ( 'NONE',  ( 4.585520833345769987, 118.0414727501857897, 0.8249672653002678713 ) ) ;
#26603=CARTESIAN_POINT ( 'NONE',  ( -2.692664463852660450, 120.6505882111413683, -0.3986361418428904235 ) ) ;
#26604=CARTESIAN_POINT ( 'NONE',  ( 4.829164506186364392, 117.3993836135881565, -1.010517262250789194 ) ) ;
#26605=CARTESIAN_POINT ( 'NONE',  ( 2.677032024553319012, 107.2224589468338536, -4.627058715154634960 ) ) ;
#26606=CARTESIAN_POINT ( 'NONE',  ( -17.20807765353001528, 147.1820577694790018, -2.053081559533529887 ) ) ;
#26607=EDGE_CURVE ( 'NONE', #14618, #31748, #17461, .T. ) ;
#26609=CARTESIAN_POINT ( 'NONE',  ( 7.880211965457339041, 122.2234151243416989, -0.4724049390182752939 ) ) ;
#26610=CARTESIAN_POINT ( 'NONE',  ( -1.556981180954984945, 156.2629499403934119, 0.08452657509653109524 ) ) ;
#26611=CARTESIAN_POINT ( 'NONE',  ( -4.288638401707804526, -7.253218809911426312, -1.756103832032595680 ) ) ;
#26612=CARTESIAN_POINT ( 'NONE',  ( 13.11470433356379139, 119.8381915656929380, 0.9809890993017411631 ) ) ;
#26613=CARTESIAN_POINT ( 'NONE',  ( 5.010184479710102501, 117.3993854065330851, 0.7504461923096029663 ) ) ;
#26614=CARTESIAN_POINT ( 'NONE',  ( 3.240743527130751200, -15.12236442990058727, 3.435505395146291274 ) ) ;
#26615=CARTESIAN_POINT ( 'NONE',  ( -9.673022701212307339, 121.1143850344477215, 1.180881524473704980 ) ) ;
#26616=CARTESIAN_POINT ( 'NONE',  ( -0.5387148418522960114, 9.198764818822382949, 0.8109227438555447476 ) ) ;
#26617=CARTESIAN_POINT ( 'NONE',  ( -0.3196863354300110704, 116.7093555017326452, -0.2333483032394376433 ) ) ;
#26618=CARTESIAN_POINT ( 'NONE',  ( 0.9169382621377788478, -11.15192339915171793, 0.3232733857163304081 ) ) ;
#26619=EDGE_LOOP ( 'NONE', ( #7398, #29460 ) ) ;
#26621=CARTESIAN_POINT ( 'NONE',  ( 4.807558371750517701, 117.0601473006971105, 0.9798501506189062349 ) ) ;
#26622=CARTESIAN_POINT ( 'NONE',  ( -0.6059414056334104792, 120.5739061664170606, 0.2722191786371237487 ) ) ;
#26624=CARTESIAN_POINT ( 'NONE',  ( 3.953338583042130150, -12.61280045678425665, 2.014973703158344787 ) ) ;
#26625=CARTESIAN_POINT ( 'NONE',  ( 5.873575024772715203, 120.4133487461328826, -0.7716123655894259192 ) ) ;
#26626=CARTESIAN_POINT ( 'NONE',  ( -18.24829758291891579, 150.1405190176936344, -2.471583571221721343 ) ) ;
#26629=CARTESIAN_POINT ( 'NONE',  ( 2.104008947125556528, -15.14483647969354330, 5.217645225406672971 ) ) ;
#26630=CARTESIAN_POINT ( 'NONE',  ( -4.842996840569961492, 117.4782722638060761, -1.161985943875174065 ) ) ;
#26631=EDGE_CURVE ( 'NONE', #7830, #12023, #11063, .T. ) ;
#26632=CARTESIAN_POINT ( 'NONE',  ( 2.818990841020078797, 121.0122979933374978, -0.009253692138209281687 ) ) ;
#26634=CARTESIAN_POINT ( 'NONE',  ( -4.798386392178022319, 114.9758031406785221, 1.576502096137255782 ) ) ;
#26639=CARTESIAN_POINT ( 'NONE',  ( 23.38383716176057803, 142.7868430859564626, 0.3143897558744219167 ) ) ;
#26640=CARTESIAN_POINT ( 'NONE',  ( -4.060783872423834318, 109.8065891650451249, 3.521960838153598505 ) ) ;
#26641=AXIS2_PLACEMENT_3D ( 'NONE', #6698, #19667, #3727 ) ;
#26642=CARTESIAN_POINT ( 'NONE',  ( -3.107210190573434616, 118.0750721850716474, 0.8420533518679624851 ) ) ;
#26644=CARTESIAN_POINT ( 'NONE',  ( 0.2629046284512602805, 36.79895747838261855, -0.7350018967835904027 ) ) ;
#26645=CARTESIAN_POINT ( 'NONE',  ( 20.66962185543543384, 147.7542213611591535, 2.445644978772825162 ) ) ;
#26646=CARTESIAN_POINT ( 'NONE',  ( 3.707542801486926276, 23.89195667223011910, -2.776928957275885068 ) ) ;
#26647=CARTESIAN_POINT ( 'NONE',  ( -7.328769482851726025, 13.23335216599729947, 4.212906450523355772 ) ) ;
#26648=CARTESIAN_POINT ( 'NONE',  ( -5.518892555433418501, 117.8876361237244907, -1.069160601140542344 ) ) ;
#26649=CARTESIAN_POINT ( 'NONE',  ( -0.7466139261200300803, 119.9044272045951374, -0.6467483038796004724 ) ) ;
#26652=CARTESIAN_POINT ( 'NONE',  ( -3.056332105116442932, 108.4800906826746143, -4.214630652369057096 ) ) ;
#26653=CARTESIAN_POINT ( 'NONE',  ( -4.814395258470165473, 104.6144662015522755, 2.302979290232680221 ) ) ;
#26655=CARTESIAN_POINT ( 'NONE',  ( -0.01876340930523686876, 19.73428105357427853, -4.634220987317214657 ) ) ;
#26658=CARTESIAN_POINT ( 'NONE',  ( 2.604768916882071128, -14.79682312136586297, 4.847387382002324330 ) ) ;
#26659=CARTESIAN_POINT ( 'NONE',  ( 3.306315723242806648, 118.9685052735122355, -0.5531158949559312754 ) ) ;
#26660=CARTESIAN_POINT ( 'NONE',  ( -14.83366055447124943, 120.8492938200443092, 0.4607208393402018043 ) ) ;
#26661=CARTESIAN_POINT ( 'NONE',  ( 4.854437695190745750, 117.4070755028450748, -0.9982814861801205808 ) ) ;
#26665=CARTESIAN_POINT ( 'NONE',  ( 0.1949087904810302418, 33.82644263972942156, 0.4054292462034596034 ) ) ;
#26666=CARTESIAN_POINT ( 'NONE',  ( 4.998192975942944649, -15.53260140147937030, 2.284796345537305928 ) ) ;
#26667=CARTESIAN_POINT ( 'NONE',  ( -13.23674331388984093, 122.5785676075921060, 1.297564987558605498 ) ) ;
#26668=CARTESIAN_POINT ( 'NONE',  ( 18.02024205669863477, 128.5942011134444272, -1.207605415130186710 ) ) ;
#26669=CARTESIAN_POINT ( 'NONE',  ( 0.8991110484329473129, 28.35728145135693268, -0.3789830077994447155 ) ) ;
#26673=CARTESIAN_POINT ( 'NONE',  ( -4.967168320455268571, 117.4023968188195681, -1.002192383175803503 ) ) ;
#26674=CARTESIAN_POINT ( 'NONE',  ( 2.033169340629980226, 122.5452913651401587, 0.2335185838714209372 ) ) ;
#26675=CARTESIAN_POINT ( 'NONE',  ( -10.38102865001225261, 154.1877054190025262, 1.364427777124047392 ) ) ;
#26676=DIRECTION ( 'NONE',  ( -0.01997839162482737546, -1.040247600000939284E-18, 0.9998004120163610509 ) ) ;
#26679=CARTESIAN_POINT ( 'NONE',  ( 18.37664568872238036, 148.6295804641074483, -1.698537578660717751 ) ) ;
#26680=CARTESIAN_POINT ( 'NONE',  ( -4.954158841009661529, 118.5534682650580862, -1.066189120819955205 ) ) ;
#26681=DIRECTION ( 'NONE',  ( -0.9998004120163608288, -4.016384292689131511E-17, -0.01997839162482749342 ) ) ;
#26683=CARTESIAN_POINT ( 'NONE',  ( 4.373555915921281567, 118.1839305412106000, -0.4384691235614320837 ) ) ;
#26684=CARTESIAN_POINT ( 'NONE',  ( 1.677891416185167017, 156.3096136994911092, -0.5101806352362399100 ) ) ;
#26686=CARTESIAN_POINT ( 'NONE',  ( 2.112177293979604187, -15.34403890755049815, 5.167321579062071457 ) ) ;
#26691=B_SPLINE_CURVE_WITH_KNOTS ( 'NONE', 3,
 ( #9591, #18960, #18748, #28351, #41360, #31967 ),
 .UNSPECIFIED., .F., .F.,
 ( 4, 2, 4 ),
 ( 0.7472851912383878803, 0.8736425956191939957, 1.000000000000000000 ),
 .UNSPECIFIED. ) ;
#26693=CARTESIAN_POINT ( 'NONE',  ( 3.490194016315742331, 12.22236127277748174, 3.029891289224248219 ) ) ;
#26694=CARTESIAN_POINT ( 'NONE',  ( 9.008986559116410220, 121.9018297702777858, 1.332107995734232109 ) ) ;
#26695=CARTESIAN_POINT ( 'NONE',  ( -1.007477757134449536, 31.95321293912196836, 2.022349366842921103 ) ) ;
#26697=CARTESIAN_POINT ( 'NONE',  ( -1.576536484031922480, 10.66345178295009788, -4.350723848753511369 ) ) ;
#26698=CARTESIAN_POINT ( 'NONE',  ( 5.289698609639951421, 121.3432423864224177, 0.1753557357117460358 ) ) ;
#26702=CARTESIAN_POINT ( 'NONE',  ( 2.163736596230561027, 116.3505410131987787, -0.2071778447972208170 ) ) ;
#26703=CARTESIAN_POINT ( 'NONE',  ( 15.19604463793433169, 156.0859089222169587, 0.3036531364422415669 ) ) ;
#26705=DIRECTION ( 'NONE',  ( 0.9998004120163609398, 4.016384292689130894E-17, 0.01997839162482749689 ) ) ;
#26706=CARTESIAN_POINT ( 'NONE',  ( 5.314256983240370324, 105.1224655745845382, -0.4585143440169748841 ) ) ;
#26712=CARTESIAN_POINT ( 'NONE',  ( -22.51579307796286145, 137.1624432810789358, -0.01304004454942945049 ) ) ;
#26715=CARTESIAN_POINT ( 'NONE',  ( -6.982215578972839509, 121.9499294214156464, -0.1835727084940861342 ) ) ;
#26717=CARTESIAN_POINT ( 'NONE',  ( 3.794806421782703776, 115.7029491485452724, -1.459834282783267767 ) ) ;
#26718=CARTESIAN_POINT ( 'NONE',  ( -15.77055413937423367, 146.5697412905949477, -0.3665361178749758087 ) ) ;
#26719=CARTESIAN_POINT ( 'NONE',  ( 6.311525104866394287, -14.07095602924590594, 0.9561848504773229340 ) ) ;
#26720=CARTESIAN_POINT ( 'NONE',  ( -1.147165779964402832, 117.8708904510121016, 0.5694250185432009337 ) ) ;
#26721=CARTESIAN_POINT ( 'NONE',  ( 4.622858883031034871, 26.85595184169372018, 0.2084198311932835834 ) ) ;
#26722=AXIS2_PLACEMENT_3D ( 'NONE', #12422, #2217, #5625 ) ;
#26723=CARTESIAN_POINT ( 'NONE',  ( 22.90211176506257829, 150.1344166263168347, 0.9094179090926688414 ) ) ;
#26724=CARTESIAN_POINT ( 'NONE',  ( 14.67165028172560604, 148.8681294118411813, 0.4913509943341035635 ) ) ;
#26725=CARTESIAN_POINT ( 'NONE',  ( 4.037907715354051241, 27.70556447992504445, -2.267523456217593214 ) ) ;
#26726=CARTESIAN_POINT ( 'NONE',  ( 0.1248384507886338285, 1.166626901725996035, -0.9703616065359238485 ) ) ;
#26727=CARTESIAN_POINT ( 'NONE',  ( -8.204617290884389291, 117.5299140688306352, -0.3545595769132391384 ) ) ;
#26729=CARTESIAN_POINT ( 'NONE',  ( 4.862391452034746209, 117.4079971399760609, 1.166187604725966054 ) ) ;
#26731=CARTESIAN_POINT ( 'NONE',  ( 2.218330162228713043, 116.2574865890770184, 0.1610120948260720108 ) ) ;
#26732=CARTESIAN_POINT ( 'NONE',  ( -3.787250209144910507, 156.8112981010400802, 1.501541828261893308 ) ) ;
#26734=CARTESIAN_POINT ( 'NONE',  ( -0.01023305610377599727, 117.8848902025789158, 0.5121039721716187376 ) ) ;
#26735=CARTESIAN_POINT ( 'NONE',  ( 6.722174884993919797, 119.4737997143703012, -1.022258653430867970 ) ) ;
#26736=CARTESIAN_POINT ( 'NONE',  ( 0.6771123631923940955, -5.471153235863896569, -0.7014129483058207937 ) ) ;
#26737=CARTESIAN_POINT ( 'NONE',  ( -9.211590693262630580, 119.0402042963619351, -1.266790605762086575 ) ) ;
#26738=CARTESIAN_POINT ( 'NONE',  ( 4.683543233604185119, 118.0095664619904028, -0.5959560594456849714 ) ) ;
#26742=CARTESIAN_POINT ( 'NONE',  ( 7.857169925943599864, 121.9903164032602518, -0.5981771023335124005 ) ) ;
#26745=CARTESIAN_POINT ( 'NONE',  ( -11.21148455117568687, 122.4230570912197038, -1.693600966768365357 ) ) ;
#26746=CARTESIAN_POINT ( 'NONE',  ( 2.515823494799488191, -15.76102479606726625, 5.403604998519412561 ) ) ;
#26747=CARTESIAN_POINT ( 'NONE',  ( -4.558369097197020992, 31.49133049583777932, -0.6947524270963534310 ) ) ;
#26748=CARTESIAN_POINT ( 'NONE',  ( -4.656319957792719677, 118.0096513897839685, -0.7824823237528982789 ) ) ;
#26751=CARTESIAN_POINT ( 'NONE',  ( 4.065926199369043204, 118.2429491485453354, 0.3080910687088499467 ) ) ;
#26752=CARTESIAN_POINT ( 'NONE',  ( 18.33584167903955731, 146.8095856830544790, 2.399012226062094744 ) ) ;
#26755=CARTESIAN_POINT ( 'NONE',  ( -6.439802422954663176E-14, 159.6054662015457382, 9.942593405483322146E-17 ) ) ;
#26756=CARTESIAN_POINT ( 'NONE',  ( 8.424193198035354158, 17.36166136180145259, -0.6763034115371487909 ) ) ;
#26757=CARTESIAN_POINT ( 'NONE',  ( 9.078381139985610915, 123.6795089456687577, 0.5923855214342147457 ) ) ;
#26758=CARTESIAN_POINT ( 'NONE',  ( 21.72212103179832710, 136.7703657609320658, -0.7093728523935389774 ) ) ;
#26763=CARTESIAN_POINT ( 'NONE',  ( -23.29076518286613862, 149.3500807853454546, -0.3882996703880463585 ) ) ;
#26764=ORIENTED_EDGE ( 'NONE', *, *, #25293, .F. ) ;
#26765=CARTESIAN_POINT ( 'NONE',  ( -5.326936277661974195, 120.5144646293056780, -0.7944123752729133070 ) ) ;
#26768=CARTESIAN_POINT ( 'NONE',  ( -10.53234188159483686, 153.0603347025997323, -0.7465333597200853877 ) ) ;
#26769=CARTESIAN_POINT ( 'NONE',  ( 3.953338583042130150, -12.61280045678425665, 2.014973703158344787 ) ) ;
#26770=CARTESIAN_POINT ( 'NONE',  ( -17.38882309766602319, 125.1846915036903027, 0.8043053978789255209 ) ) ;
#26771=CARTESIAN_POINT ( 'NONE',  ( -4.218275339060285845, 155.8585684991085714, -0.08429118021179402009 ) ) ;
#26772=CARTESIAN_POINT ( 'NONE',  ( 3.300851927471557090, 159.4676453237595410, 0.08072286411353209179 ) ) ;
#26774=CARTESIAN_POINT ( 'NONE',  ( 3.746277899330032302, -0.8937244826341392834, -2.755274729908455900 ) ) ;
#26775=CARTESIAN_POINT ( 'NONE',  ( -0.8860745468267199332, 116.4323782974132513, -0.03055428320029199979 ) ) ;
#26778=CARTESIAN_POINT ( 'NONE',  ( 8.223111631096672980, 120.3648856214035590, 1.439954315622481662 ) ) ;
#26779=CARTESIAN_POINT ( 'NONE',  ( -3.522755225739859775, -9.592572062075928940, 3.019445982675781348 ) ) ;
#26780=CARTESIAN_POINT ( 'NONE',  ( 15.97393847379841070, 155.1095016151506911, 1.658827062323852797 ) ) ;
#26783=CARTESIAN_POINT ( 'NONE',  ( 19.67014042257518724, 150.6586468064772646, -1.570413873854537234 ) ) ;
#26785=CARTESIAN_POINT ( 'NONE',  ( -2.329872802932658082, -2.670747431267189498, -3.990024091085845548 ) ) ;
#26786=CARTESIAN_POINT ( 'NONE',  ( -22.05995121575398343, 150.4421090420883900, -1.612468304426259103 ) ) ;
#26787=VERTEX_POINT ( 'NONE', #14604 ) ;
#26789=CARTESIAN_POINT ( 'NONE',  ( -0.6772589037151361957, 156.3292479207028407, 0.3306685775513075742 ) ) ;
#26790=CARTESIAN_POINT ( 'NONE',  ( 4.840206765044483994, -15.05961300585426166, 4.264492456498921946 ) ) ;
#26792=TOROIDAL_SURFACE ( 'NONE', #4376, 3.683000000000000718, 0.5080000000000000071 ) ;
#26793=CARTESIAN_POINT ( 'NONE',  ( -3.582589445373201009, 109.6950671057752373, -3.736549424469191916 ) ) ;
#26795=CARTESIAN_POINT ( 'NONE',  ( 8.358437701610622383, 156.6436466068687423, 2.074018175080058146 ) ) ;
#26796=CARTESIAN_POINT ( 'NONE',  ( -6.617255152258657249E-14, 94.83546620154572793, -2.708805023911452991E-18 ) ) ;
#26799=CARTESIAN_POINT ( 'NONE',  ( -15.15503192428649371, 121.4505734225448066, 0.6300967139502822167 ) ) ;
#26800=CARTESIAN_POINT ( 'NONE',  ( -4.414756536061148928, 7.050034479431100287, -7.184669936685727620 ) ) ;
#26801=CARTESIAN_POINT ( 'NONE',  ( 15.33786013020720773, 149.0334586719817764, 1.566117276479743303 ) ) ;
#26803=CARTESIAN_POINT ( 'NONE',  ( 14.99898601413110022, 156.1447123740162226, -0.3355057415612999749 ) ) ;
#26805=AXIS2_PLACEMENT_3D ( 'NONE', #42008, #39014, #22788 ) ;
#26808=CARTESIAN_POINT ( 'NONE',  ( -3.212720104892762052, 117.3993812109657711, 1.261607097357493323 ) ) ;
#26811=CARTESIAN_POINT ( 'NONE',  ( -4.407706242951269893, 118.1630026188911415, 0.4884894518719885559 ) ) ;
#26812=CARTESIAN_POINT ( 'NONE',  ( 3.893689849856083462, 109.0594030058512232, -3.652599047905514595 ) ) ;
#26815=CARTESIAN_POINT ( 'NONE',  ( 3.996284611207044257, 119.1072997412182701, -0.7644371380813023142 ) ) ;
#26816=CARTESIAN_POINT ( 'NONE',  ( -7.112984908206943402, 122.4243137415680280, -0.2517356677811183885 ) ) ;
#26817=CARTESIAN_POINT ( 'NONE',  ( 4.508147239578550902, 118.0682817303566310, 0.8183067226364422186 ) ) ;
#26818=CARTESIAN_POINT ( 'NONE',  ( -3.128511139047554401, 156.1781389015385457, -0.8559903927114130839 ) ) ;
#26820=CARTESIAN_POINT ( 'NONE',  ( -1.557005993388528964, 115.7027528728559531, -1.730858768160303596 ) ) ;
#26822=CARTESIAN_POINT ( 'NONE',  ( -6.656543858376176668E-14, 104.6144662015457243, -3.850115147268248130E-19 ) ) ;
#26823=CARTESIAN_POINT ( 'NONE',  ( -0.7897433827105079240, 156.7682548876429109, -1.239156740209750307 ) ) ;
#26824=CARTESIAN_POINT ( 'NONE',  ( -6.583861033951825950E-14, 91.02546620154572565, 1.480257718193877056E-29 ) ) ;
#26826=CARTESIAN_POINT ( 'NONE',  ( 8.778228370994069607, 117.8144977861501701, -0.2251889147252496837 ) ) ;
#26827=CARTESIAN_POINT ( 'NONE',  ( -10.06125758770563117, 125.9185081520631257, -0.05443999739187975473 ) ) ;
#26829=CARTESIAN_POINT ( 'NONE',  ( 22.78320035282265721, 142.4248215231809240, 1.435786487410106727 ) ) ;
#26831=CARTESIAN_POINT ( 'NONE',  ( 1.980066450162843106, -15.31690195035381663, 5.269506609478212589 ) ) ;
#26832=CARTESIAN_POINT ( 'NONE',  ( -18.88959041316451604, 148.1672603684278329, 1.723054188180887847 ) ) ;
#26833=CARTESIAN_POINT ( 'NONE',  ( -0.2078495401522961472, -3.970246887572310257, -0.9510052327550873041 ) ) ;
#26834=CARTESIAN_POINT ( 'NONE',  ( -22.39330865153385020, 150.7562895891929031, -1.036336034128335193 ) ) ;
#26835=CARTESIAN_POINT ( 'NONE',  ( 0.7510871189337386955, -11.68616409646884158, 0.6196617644748384501 ) ) ;
#26836=B_SPLINE_CURVE_WITH_KNOTS ( 'NONE', 5,
 ( #384, #2735, #28902, #39346, #9523, #18890 ),
 .UNSPECIFIED., .F., .F.,
 ( 6, 6 ),
 ( 0.000000000000000000, 1.000000000000000000 ),
 .UNSPECIFIED. ) ;
#26837=ORIENTED_EDGE ( 'NONE', *, *, #7319, .F. ) ;
#26839=CARTESIAN_POINT ( 'NONE',  ( 7.643894675291481811, 124.7210964017841377, 0.1527028184316447379 ) ) ;
#26840=CARTESIAN_POINT ( 'NONE',  ( -5.888833980634905707, 121.2452591720019370, 0.3608419296047723490 ) ) ;
#26841=CARTESIAN_POINT ( 'NONE',  ( 4.908419482240064191, -12.74103600948764381, 2.406175225133469819 ) ) ;
#26842=CARTESIAN_POINT ( 'NONE',  ( 17.57956382101102477, 146.6691408387931688, -1.464727724346841953 ) ) ;
#26843=CARTESIAN_POINT ( 'NONE',  ( -14.48730688186172166, 125.6573275863457866, -2.042335292678053360 ) ) ;
#26844=CARTESIAN_POINT ( 'NONE',  ( 4.299095875381824250, 115.7036751318245678, 1.546138500147263839 ) ) ;
#26845=EDGE_CURVE ( 'NONE', #14389, #909, #9035, .T. ) ;
#26846=CARTESIAN_POINT ( 'NONE',  ( 1.979956398862833922, -15.17398463081316784, 5.317940750273952411 ) ) ;
#26847=CARTESIAN_POINT ( 'NONE',  ( -4.932839847226206054, 117.4753194895807979, -1.061409891849272036 ) ) ;
#26848=CARTESIAN_POINT ( 'NONE',  ( 15.81024248929834641, 146.2514283349100594, 0.08545504004084580885 ) ) ;
#26850=CARTESIAN_POINT ( 'NONE',  ( -2.918314285971537636, 107.9144754008294029, 4.333296045763540327 ) ) ;
#26851=CARTESIAN_POINT ( 'NONE',  ( 1.615233038652823305, 106.5840813593882075, 5.022315509531020794 ) ) ;
#26853=CARTESIAN_POINT ( 'NONE',  ( -4.721633889153055819, 27.87760190724945275, 0.5093158822365639882 ) ) ;
#26854=CARTESIAN_POINT ( 'NONE',  ( 22.97142009758390557, 150.1545470440437953, 0.2295619762022475807 ) ) ;
#26856=CARTESIAN_POINT ( 'NONE',  ( 1.824049531341678021, -15.68876244400656184, 5.768564601460718144 ) ) ;
#26858=DIRECTION ( 'NONE',  ( -0.9998004120163608288, 0.000000000000000000, -0.01997839162482749342 ) ) ;
#26859=CARTESIAN_POINT ( 'NONE',  ( 19.36210883413055583, 150.5708382285403388, 2.397539767985719994 ) ) ;
#26860=ORIENTED_EDGE ( 'NONE', *, *, #38613, .T. ) ;
#26861=CARTESIAN_POINT ( 'NONE',  ( -5.416678580886389760, 20.69493382693234196, -6.515560366292809213 ) ) ;
#26862=CARTESIAN_POINT ( 'NONE',  ( -2.347363924070998475, 117.2563622648257962, -0.6826054999005346513 ) ) ;
#26863=CARTESIAN_POINT ( 'NONE',  ( -1.232226514449051402, 109.2701902778323557, -3.967559291276892885 ) ) ;
#26867=CARTESIAN_POINT ( 'NONE',  ( -3.812863311134618183, 2.017465188139291765, -2.614655560905410958 ) ) ;
#26869=CARTESIAN_POINT ( 'NONE',  ( -5.268467657037344765, 115.6909491485453003, 0.8695824031848999880 ) ) ;
#26870=CARTESIAN_POINT ( 'NONE',  ( 2.107392885931908211, -15.11054218480166433, 5.236909061670549370 ) ) ;
#26872=CARTESIAN_POINT ( 'NONE',  ( 3.904686386324433656, 121.5791280715047122, -0.1678698840778539148 ) ) ;
#26873=CARTESIAN_POINT ( 'NONE',  ( -22.62544200675493400, 150.0155710288180444, 0.5141704484958254939 ) ) ;
#26874=CARTESIAN_POINT ( 'NONE',  ( 8.798071512540863282, 117.6842349196870572, 0.1758064070670784795 ) ) ;
#26877=CARTESIAN_POINT ( 'NONE',  ( -2.762866373388253471, 104.6144662015512097, -4.566024155138136642 ) ) ;
#26878=CARTESIAN_POINT ( 'NONE',  ( 4.176612884749554944, -15.71584146423912820, 3.621469129306375656 ) ) ;
#26879=CARTESIAN_POINT ( 'NONE',  ( -20.20415560162858881, 149.0333503175929479, 1.664251383091793768 ) ) ;
#26880=CARTESIAN_POINT ( 'NONE',  ( 0.5513313392710353922, 29.23057874652566923, -0.8050760855368327418 ) ) ;
#26881=ORIENTED_EDGE ( 'NONE', *, *, #40687, .F. ) ;
#26883=CARTESIAN_POINT ( 'NONE',  ( 1.969999177844855121, 122.1523088006674840, 0.2733757396980690535 ) ) ;
#26885=CARTESIAN_POINT ( 'NONE',  ( -4.935370518415244767, 156.1188696671683260, 1.185051001079852284 ) ) ;
#26886=CARTESIAN_POINT ( 'NONE',  ( 1.912930843383831236, 118.1189424416472207, 0.9466463369225973645 ) ) ;
#26887=CARTESIAN_POINT ( 'NONE',  ( 0.5200570697820592336, 119.3183582894065893, -0.5597423419424873980 ) ) ;
#26888=CARTESIAN_POINT ( 'NONE',  ( -1.110739552455700663, 158.5855360310326319, -1.562719372149667274 ) ) ;
#26889=DIRECTION ( 'NONE',  ( 0.9998004120163608288, 4.016384292689131511E-17, 0.01997839162482749342 ) ) ;
#26890=CARTESIAN_POINT ( 'NONE',  ( 4.161853366895682527, 118.2393569085959371, -0.2292923879269599674 ) ) ;
#26891=CARTESIAN_POINT ( 'NONE',  ( 12.05713894362174798, 151.9703418938154584, -0.4396675171196798848 ) ) ;
#26892=ORIENTED_EDGE ( 'NONE', *, *, #7173, .F. ) ;
#26893=CARTESIAN_POINT ( 'NONE',  ( 2.598075364112794716, -15.28479904474297513, 4.671545106743766773 ) ) ;
#26896=ADVANCED_FACE ( 'NONE', ( #27817 ), #33393, .T. ) ;
#26898=CARTESIAN_POINT ( 'NONE',  ( 3.900846188197024667, 12.44727460162280863, 2.488979119290085862 ) ) ;
#26899=CARTESIAN_POINT ( 'NONE',  ( 6.954653016369009677, 155.6889469082406947, 1.616181084571816307 ) ) ;
#26900=CARTESIAN_POINT ( 'NONE',  ( -2.502258884723083554, 30.19631072378583170, 1.542227018752644119 ) ) ;
#26901=CARTESIAN_POINT ( 'NONE',  ( -2.755274729907521980, 20.69627551736597226, -3.746277899328600558 ) ) ;
#26902=CARTESIAN_POINT ( 'NONE',  ( 15.77366026095708129, 146.5725700477668170, 0.4436318658883101618 ) ) ;
#26904=EDGE_CURVE ( 'NONE', #22816, #9488, #8652, .T. ) ;
#26906=CARTESIAN_POINT ( 'NONE',  ( -5.542008918447461241, 116.7834412270213562, -0.4238622777438119105 ) ) ;
#26907=DIRECTION ( 'NONE',  ( 0.01997839162482749689, 1.040247600000945640E-18, -0.9998004120163610509 ) ) ;
#26911=CARTESIAN_POINT ( 'NONE',  ( 5.579263951540290201, 8.940976842658965751, -6.340258638080404019 ) ) ;
#26915=CARTESIAN_POINT ( 'NONE',  ( 0.006734421711972093244, 121.9236798544229003, -0.3370180007451226700 ) ) ;
#26916=CARTESIAN_POINT ( 'NONE',  ( -0.004910662370487326248, 159.5928157220454295, 0.2457496255665023166 ) ) ;
#26919=CARTESIAN_POINT ( 'NONE',  ( -6.969786809622995349, 121.9471538115466700, -0.2197179574160783577 ) ) ;
#26924=CARTESIAN_POINT ( 'NONE',  ( -6.499560145427196289, 121.7799842514348541, -0.1589113151347878727 ) ) ;
#26925=CARTESIAN_POINT ( 'NONE',  ( 6.166227012738786151, -13.75546675568918609, 1.699147612634045235 ) ) ;
#26926=CARTESIAN_POINT ( 'NONE',  ( -12.06131655867255503, 120.6765805525287334, 1.069212010736126039 ) ) ;
#26927=CARTESIAN_POINT ( 'NONE',  ( -3.957843245660688680, 22.95775517496322848, 2.395914033147342970 ) ) ;
#26928=CARTESIAN_POINT ( 'NONE',  ( 23.23349130944691154, 142.6711341654318801, 0.9216821775544488116 ) ) ;
#26930=CARTESIAN_POINT ( 'NONE',  ( 2.202447430380541249, -15.40435026327015322, 5.902591840625516895 ) ) ;
#26931=CARTESIAN_POINT ( 'NONE',  ( 2.889066315880882030, 25.55657059589919911, 3.609430016826872478 ) ) ;
#26932=CARTESIAN_POINT ( 'NONE',  ( -0.9739946362265716751, -5.975847910206034896, -0.08934465120823924245 ) ) ;
#26933=CARTESIAN_POINT ( 'NONE',  ( -11.65197432296793068, 118.7334002725740874, -0.4428703322330640457 ) ) ;
#26934=DIRECTION ( 'NONE',  ( -0.9998004120163610509, -5.205824365704083805E-17, -0.01997839162482749689 ) ) ;
#26937=CARTESIAN_POINT ( 'NONE',  ( 2.248466038385836807, 116.3129351467598127, 0.2264917513733100685 ) ) ;
#26938=CARTESIAN_POINT ( 'NONE',  ( -5.873949295438763762, 120.1673030736515955, 0.8402073876045392797 ) ) ;
#26940=CARTESIAN_POINT ( 'NONE',  ( -0.02768730785358111679, 158.9256195073445213, 1.385586103196075891 ) ) ;
#26941=CARTESIAN_POINT ( 'NONE',  ( 19.22350799450994430, 148.9694856701144090, -1.735702374547824167 ) ) ;
#26942=CARTESIAN_POINT ( 'NONE',  ( -0.9685753864191435358, -11.31243604255521085, 0.1179740209226832204 ) ) ;
#26943=CARTESIAN_POINT ( 'NONE',  ( -19.06843068773027383, 131.8899703912256314, -2.039348754248471174 ) ) ;
#26945=CARTESIAN_POINT ( 'NONE',  ( 3.897805094127884118, 104.6144662015456674, 2.864625571244531876 ) ) ;
#26946=CARTESIAN_POINT ( 'NONE',  ( 10.66674206690810500, 124.7671305375842934, -0.7411263988551108906 ) ) ;
#26948=CARTESIAN_POINT ( 'NONE',  ( -7.783246152616193569, 154.6561476914895081, -0.1555277812256514736 ) ) ;
#26950=CARTESIAN_POINT ( 'NONE',  ( -7.646026353518148966, 156.1362479297160348, -1.963328325631339411 ) ) ;
#26951=CARTESIAN_POINT ( 'NONE',  ( 4.270102617218862306, -15.70017440876955739, 3.434341872514240723 ) ) ;
#26953=CARTESIAN_POINT ( 'NONE',  ( -4.554733065532879266, 118.0858692952890863, -0.7374014039634101403 ) ) ;
#26955=CARTESIAN_POINT ( 'NONE',  ( 4.065926199369043204, 118.2429491485453354, 0.3080910687088499467 ) ) ;
#26956=B_SPLINE_SURFACE_WITH_KNOTS ( 'NONE', 3, 3, ( 
 ( #1360, #36713, #11550, #1151, #24332, #17520, #14318, #27330, #4775, #7953, #30727, #1576, #37337, #4980, #17937, #30940, #24533, #2832, #16000, #34779, #31787, #9003, #9214, #19201, #37969, #21970, #24755, #15585, #2626, #32209, #34571, #35000, #28800, #38605 ),
 ( #5820, #12408, #28590, #15161, #28382, #18776, #35403, #41598, #35202, #41172, #28167, #8578, #21752, #37754, #31994, #22377, #25400, #38186, #11976, #38402, #22171, #9411, #18569, #40960, #15792, #3042, #6028, #21542, #5398, #6230, #18990, #24970, #8794, #41388 ),
 ( #5613, #11766, #41814, #12193, #18354, #31360, #12610, #25597, #2203, #31576, #2416, #15376, #25186, #3457, #36460, #29209, #3245, #26649, #6434, #12812, #39228, #19822, #10038, #478, #16634, #16204, #16419, #23010, #23431, #6647, #20241, #4096, #19408, #7071 ),
 ( #52, #9620, #7279, #13451, #13659, #20035, #13018, #3669, #32415, #35620, #32624, #33054, #28999, #3884, #33267, #9829, #16849, #687, #42016, #25802, #26439, #36038, #38808, #29641, #35831, #29425, #39021, #266, #39443, #19611, #10461, #26012, #6853, #36250 ),
 ( #22796, #13240, #10246, #26224, #32839, #23217, #22588, #29849, #39657, #36884, #27074, #30472, #14691, #10667, #1527, #39871, #27283, #23865, #1733, #1316, #20663, #30892, #895, #11500, #37491, #14273, #37287, #26863, #27696, #21080, #7702, #30262, #4513, #40704 ),
 ( #34105, #24486, #8314, #21286, #30679, #40297, #23648, #4726, #33689, #17474, #40082, #11090, #17678, #24077, #34315, #33478, #37089, #24282, #17055, #7907, #36670, #27495, #20871, #7491, #14483, #30057, #33895, #13869, #40503, #11298, #20451, #8106, #4308, #4932 ),
 ( #17890, #17271, #1103, #14070, #10877, #18937, #31101, #41757, #25547, #18512, #25342, #14899, #31945, #31518, #8739, #11714, #2362, #38550, #27901, #12139, #1940, #5974, #24701, #5769, #41120, #40909, #28539, #15739, #21490, #38133, #15321, #11926, #37915, #5555 ),
 ( #21700, #34522, #28328, #5348, #41336, #2148, #2783, #35149, #25131, #37707, #9363, #38345, #28744, #8948, #9163, #12558, #18302, #8530, #34724, #22326, #31303, #15107, #5144, #28110, #24918, #21915, #34945, #18723, #31733, #2576, #15537, #41546, #12354, #18098 ),
 ( #22120, #6800, #16150, #3835, #32153, #6384, #15948, #13610, #19768, #19989, #13398, #22539, #9984, #38758, #19354, #29801, #28945, #32360, #35775, #32789, #39607, #33007, #16584, #3400, #10410, #41962, #3188, #1, #3619, #9568, #29154, #29593, #35351, #35566 ),
 ( #25960, #6179, #26172, #7021, #427, #16367, #22957, #26386, #39393, #36200, #39177, #2986, #12966, #6590, #38967, #12761, #25750, #32567, #35985, #10195, #23165, #9777, #22744, #19558, #29373, #212, #16799, #641, #13187, #26600, #19148, #14225, #20607, #21033 ),
 ( #27232, #33639, #30215, #14019, #23810, #26816, #4046, #27026, #39824, #4466, #23600, #36831, #20399, #34055, #11245, #7651, #17006, #1686, #1474, #24230, #17423, #14431, #37240, #36621, #30005, #40034, #30837, #7441, #10618, #4884, #845, #7233, #30421, #40246 ),
 ( #11040, #33427, #10829, #1268, #17839, #1055, #14640, #40654, #13817, #27439, #7858, #24023, #40455, #37040, #4256, #27641, #17218, #20819, #23382, #20193, #33845, #8058, #4673, #17631, #30631, #36415, #33218, #37658, #34675, #34890, #2095, #2525, #8482, #12088 ) ),
 .UNSPECIFIED., .F., .F., .F.,
 ( 4, 1, 1, 1, 1, 1, 3, 4 ),
 ( 4, 1, 1, 1, 1, 1, 1, 1, 1, 1, 1, 1, 1, 1, 1, 1, 1, 1, 1, 2, 1, 1, 1, 1, 1, 1, 1, 1, 1, 1, 4 ),
 ( 0.000000000000000000, 0.1666666666666666574, 0.2500000000000000000, 0.5000000000000000000, 0.5555555555555555802, 0.7500000000000000000, 1.000000000000000000, 1.010000000000000009 ),
 ( 0.000000000000000000, 0.02126250000000000015, 0.04252500000000000030, 0.06378749999999999698, 0.08505000000000000060, 0.1063125000000000042, 0.1275749999999999940, 0.1488374999999999837, 0.1701000000000000012, 0.1913624999999999909, 0.2126250000000000084, 0.2338874999999999704, 0.2551500000000000434, 0.2764124999999999499, 0.2870437499999999864, 0.2976749999999999674, 0.3083062500000000039, 0.3189375000000000404, 0.3295687499999999659, 0.3402000000000000024, 0.4226750000000000229, 0.5051499999999999879, 0.5876249999999998419, 0.6700999999999999179, 0.7525749999999999940, 0.7938125000000000320, 0.8350499999999999590, 0.8762874999999994419, 0.9175249999999994799, 0.9587624999999999620, 1.000000000000000000 ),
 .UNSPECIFIED. ) ;
#26957=CARTESIAN_POINT ( 'NONE',  ( 14.87841870982556358, 131.2528086460777388, 2.073644862699850933 ) ) ;
#26958=DIRECTION ( 'NONE',  ( -0.01997839162482793057, 0.000000000000000000, 0.9998004120163608288 ) ) ;
#26959=CARTESIAN_POINT ( 'NONE',  ( 11.73725613052199535, 118.7267541726749869, 0.2187512536375166017 ) ) ;
#26961=CARTESIAN_POINT ( 'NONE',  ( 5.158690622980511620, 18.63085216599767691, -6.696816702733363158 ) ) ;
#26962=CARTESIAN_POINT ( 'NONE',  ( 9.269771126213358414, 123.9149913687586064, 0.6034020272129928530 ) ) ;
#26964=EDGE_CURVE ( 'NONE', #32861, #4233, #19099, .T. ) ;
#26965=AXIS2_PLACEMENT_3D ( 'NONE', #25444, #35879, #28844 ) ;
#26966=CARTESIAN_POINT ( 'NONE',  ( 15.27126642897840192, 121.5932973536894934, -0.6323128539531662762 ) ) ;
#26967=AXIS2_PLACEMENT_3D ( 'NONE', #11706, #18504, #37083 ) ;
#26968=CARTESIAN_POINT ( 'NONE',  ( -4.808149584360944750, 105.1224662015457483, 0.4147572885131461939 ) ) ;
#26970=CARTESIAN_POINT ( 'NONE',  ( -10.82496502431745000, 157.9086237439880733, -0.1564342443379707071 ) ) ;
#26973=CARTESIAN_POINT ( 'NONE',  ( 8.002845466965794685, 121.6569013250319387, -0.7958636649122211582 ) ) ;
#26974=CARTESIAN_POINT ( 'NONE',  ( -8.778228370994318297, 117.8144977861501701, 0.2251889147251710244 ) ) ;
#26976=CARTESIAN_POINT ( 'NONE',  ( -4.826173324110722973, 117.7976308133446821, -0.9239831869685056764 ) ) ;
#26977=CARTESIAN_POINT ( 'NONE',  ( -2.942445288855481511, 156.0884104482065595, -0.3607664148606968268 ) ) ;
#26978=CARTESIAN_POINT ( 'NONE',  ( 4.564001774108119136, -12.95384785397724059, 2.770574723176509657 ) ) ;
#26979=CARTESIAN_POINT ( 'NONE',  ( -21.63845757858517871, 150.4657531037631486, 1.001545151475624174 ) ) ;
#26981=CARTESIAN_POINT ( 'NONE',  ( 5.786284826928784319, 116.9447284183608389, 0.1988161383433787732 ) ) ;
#26984=CARTESIAN_POINT ( 'NONE',  ( -3.832284926465886254, -5.753926550059754064, 2.584458424559757272 ) ) ;
#26985=CARTESIAN_POINT ( 'NONE',  ( -22.83504831576704674, 150.4065277667444036, -0.4818782557684027079 ) ) ;
#26989=CARTESIAN_POINT ( 'NONE',  ( 4.368446179951305020, 118.5872638624673243, 1.043865840824246716 ) ) ;
#26990=CARTESIAN_POINT ( 'NONE',  ( -2.168033660621066172, 0.5777166996233511487, 4.103230905123370853 ) ) ;
#26991=CARTESIAN_POINT ( 'NONE',  ( 9.442718531279737704, 118.5748184150550060, 1.042386753229705088 ) ) ;
#26993=CARTESIAN_POINT ( 'NONE',  ( -6.616924617768071466E-14, 97.37546620154573418, 7.965525879364083286E-30 ) ) ;
#26994=CARTESIAN_POINT ( 'NONE',  ( 20.91036014055495684, 148.6614476615901594, -1.563091210272363085 ) ) ;
#26995=CARTESIAN_POINT ( 'NONE',  ( 1.294644163514462987, -7.843371450943685375, 4.453423563430108700 ) ) ;
#26996=CARTESIAN_POINT ( 'NONE',  ( -15.11776246977262694, 121.4505734225448066, -1.235019191190165344 ) ) ;
#26997=ORIENTED_EDGE ( 'NONE', *, *, #13171, .T. ) ;
#26999=CARTESIAN_POINT ( 'NONE',  ( -8.581106358026319825, 123.3373102669514765, -0.01935445114830152899 ) ) ;
#27000=CARTESIAN_POINT ( 'NONE',  ( 6.419191409189793696, -13.32337952207179832, 0.5587850172365541601 ) ) ;
#27004=CARTESIAN_POINT ( 'NONE',  ( 10.72551448100089111, 121.7859837122882283, 1.665033671525604442 ) ) ;
#27008=AXIS2_PLACEMENT_3D ( 'NONE', #18641, #22040, #3316 ) ;
#27009=CARTESIAN_POINT ( 'NONE',  ( -3.922549711534387917, 117.3164332630744298, 0.5226386447273276836 ) ) ;
#27010=CARTESIAN_POINT ( 'NONE',  ( -2.144872632962109726, 6.596990873201863614, -8.179991544870226505 ) ) ;
#27011=CARTESIAN_POINT ( 'NONE',  ( 16.44150122627317856, 146.0252812507985141, 1.609049209688531157 ) ) ;
#27013=CARTESIAN_POINT ( 'NONE',  ( 23.09108451844687693, 149.2510847660714148, -0.2673146292145802128 ) ) ;
#27020=CARTESIAN_POINT ( 'NONE',  ( -4.537165138249189766, 118.1142604855938316, 0.5194510162086110050 ) ) ;
#27021=CARTESIAN_POINT ( 'NONE',  ( 0.6790819876102632824, 105.9272292791364265, -5.296718569794414577 ) ) ;
#27025=CARTESIAN_POINT ( 'NONE',  ( 8.350555576214318876, 119.9924706458420758, -1.116089668697638260 ) ) ;
#27026=CARTESIAN_POINT ( 'NONE',  ( -6.711594774621165271, 121.2247800624193133, -0.3423702293131483665 ) ) ;
#27027=CARTESIAN_POINT ( 'NONE',  ( 4.543433710119733071, 118.0881514374072196, 0.7498910874544754135 ) ) ;
#27028=CARTESIAN_POINT ( 'NONE',  ( -16.00153516066852077, 147.3640369757652877, -1.286050259728349410 ) ) ;
#27029=FACE_OUTER_BOUND ( 'NONE', #24179, .T. ) ;
#27030=CARTESIAN_POINT ( 'NONE',  ( 0.7141878136923727194, 118.1651004746852749, -0.8604252410570366605 ) ) ;
#27031=CARTESIAN_POINT ( 'NONE',  ( 7.639359131133803160, 124.2918010433613745, 0.1437932647211237758 ) ) ;
#27032=CARTESIAN_POINT ( 'NONE',  ( -14.47722597845739223, 150.4300676932417389, -1.698653275673423835 ) ) ;
#27035=CARTESIAN_POINT ( 'NONE',  ( 8.019189887688648710, 121.5801876769127006, -0.8265596201061345960 ) ) ;
#27036=CARTESIAN_POINT ( 'NONE',  ( 7.002510706568009446, 121.9568449752713661, 0.1399268290605550913 ) ) ;
#27038=CARTESIAN_POINT ( 'NONE',  ( 14.81745968805112312, 156.1223461918646933, 1.150419650929870752 ) ) ;
#27040=CARTESIAN_POINT ( 'NONE',  ( 2.778183380295619287, -15.08691762314898277, 4.378844564414270835 ) ) ;
#27041=CARTESIAN_POINT ( 'NONE',  ( -18.72287149482797730, 147.1333978507680627, 1.701234099286256463 ) ) ;
#27042=CARTESIAN_POINT ( 'NONE',  ( -0.9497947497622778457, -2.244019015280241280, -0.2169513509177584398 ) ) ;
#27043=CARTESIAN_POINT ( 'NONE',  ( -0.3250403508453759693, 116.7787044104018861, -0.2632219653755002997 ) ) ;
#27044=AXIS2_PLACEMENT_3D ( 'NONE', #41196, #5845, #38424 ) ;
#27045=CARTESIAN_POINT ( 'NONE',  ( -0.9222101193809760789, -5.324732007522724686, 0.3213417913276819249 ) ) ;
#27048=CARTESIAN_POINT ( 'NONE',  ( 4.381926848743999514, 111.2539628214143903, 3.135495374750700837 ) ) ;
#27050=CARTESIAN_POINT ( 'NONE',  ( -16.08724493259849453, 146.0544122543811341, 0.5338004346038370818 ) ) ;
#27051=CARTESIAN_POINT ( 'NONE',  ( 4.778187575955942457, -13.11831155531867310, 3.026993680286476973 ) ) ;
#27052=CARTESIAN_POINT ( 'NONE',  ( 3.455858276899827608, 119.9243055703230851, -0.6230356542855078894 ) ) ;
#27054=CARTESIAN_POINT ( 'NONE',  ( -12.48017577322021232, 122.5542284311838870, -1.820249166172293265 ) ) ;
#27055=CARTESIAN_POINT ( 'NONE',  ( 4.372915526211548887, 104.6144662015457527, 2.049786579368134021 ) ) ;
#27056=CARTESIAN_POINT ( 'NONE',  ( 2.234143439902941175, -15.10063862499563747, 5.099642030148213934 ) ) ;
#27057=CARTESIAN_POINT ( 'NONE',  ( -4.755622421505391273, 117.4716786420896284, -1.195466823065375994 ) ) ;
#27058=CARTESIAN_POINT ( 'NONE',  ( 15.66469409602187746, 147.2250547476223801, 0.08357164438767009096 ) ) ;
#27062=CARTESIAN_POINT ( 'NONE',  ( 3.799804381934697606, 109.6290786634575483, 3.753174195237087840 ) ) ;
#27063=DIRECTION ( 'NONE',  ( 4.017660918040594346E-17, -1.000000000000000000, -2.376309959284834438E-19 ) ) ;
#27064=CARTESIAN_POINT ( 'NONE',  ( -6.540217103314379345E-14, 82.64346620154573486, 2.383338306179204368E-29 ) ) ;
#27065=CARTESIAN_POINT ( 'NONE',  ( 18.64921795038422658, 125.2334963081946313, 0.1144521110716927581 ) ) ;
#27067=CARTESIAN_POINT ( 'NONE',  ( 2.109569702550104786, -15.45397857566253919, 5.961763561042187298 ) ) ;
#27069=CARTESIAN_POINT ( 'NONE',  ( -3.212145564005312259, 31.43389969159332509, 0.5456719981668799457 ) ) ;
#27070=CARTESIAN_POINT ( 'NONE',  ( -0.03067001211942077879, 158.6015251912307633, 1.534852821454057992 ) ) ;
#27071=EDGE_LOOP ( 'NONE', ( #41418, #15883, #2101, #33039 ) ) ;
#27072=CARTESIAN_POINT ( 'NONE',  ( -0.9765287272027848298, 24.25689591457997452, 8.364652468500624494 ) ) ;
#27073=CARTESIAN_POINT ( 'NONE',  ( 8.671363884827380630, 118.3858182005267707, -0.6829674701833058359 ) ) ;
#27074=CARTESIAN_POINT ( 'NONE',  ( -2.642867612521379250, 121.0686911241271702, -0.3905210903889252405 ) ) ;
#27075=CARTESIAN_POINT ( 'NONE',  ( 4.756814328053569518, 117.4032681585788396, 1.206529665642613658 ) ) ;
#27076=CARTESIAN_POINT ( 'NONE',  ( -2.274862078065374771, 107.2457239391372354, -4.729709913239623198 ) ) ;
#27077=CARTESIAN_POINT ( 'NONE',  ( -0.002462548248923642717, 123.7646714092002611, 0.1232359841711014870 ) ) ;
#27078=CARTESIAN_POINT ( 'NONE',  ( -2.948169924849943335, 1.592661447142720732, -3.562413953034572867 ) ) ;
#27080=CARTESIAN_POINT ( 'NONE',  ( -4.831828830118795715, 118.5264896598256854, 0.7503674394378322399 ) ) ;
#27081=CARTESIAN_POINT ( 'NONE',  ( 3.001448597307602828, -14.49079452896849496, 4.301892286087903194 ) ) ;
#27082=CARTESIAN_POINT ( 'NONE',  ( 0.1065646865914871844, 105.8844662015457061, -5.332932678536314697 ) ) ;
#27083=CARTESIAN_POINT ( 'NONE',  ( -22.97084167624232975, 148.6798292920915117, 0.5140709287734972488 ) ) ;
#27084=CARTESIAN_POINT ( 'NONE',  ( -2.993548618139343809, 30.66372051476451688, 4.100031124125591120 ) ) ;
#27088=CARTESIAN_POINT ( 'NONE',  ( 4.902411944313367798, -15.42400938342815309, 0.6670879667284028702 ) ) ;
#27089=CARTESIAN_POINT ( 'NONE',  ( -5.018689047519398372, 118.8869175073591578, 0.8997529482361045217 ) ) ;
#27090=CARTESIAN_POINT ( 'NONE',  ( -3.832284926465886254, -5.753926550059754064, 2.584458424559757272 ) ) ;
#27091=VERTEX_POINT ( 'NONE', #28875 ) ;
#27093=CARTESIAN_POINT ( 'NONE',  ( 0.6699575554300896130, 116.0160817474902331, 1.654834682733560713 ) ) ;
#27094=CARTESIAN_POINT ( 'NONE',  ( -10.60975745311351481, 123.7931190674884050, 0.9249770984159895182 ) ) ;
#27095=CARTESIAN_POINT ( 'NONE',  ( -4.807616723150741400, 117.4049522327240709, -1.198082295914128403 ) ) ;
#27096=CARTESIAN_POINT ( 'NONE',  ( 7.897101653775039587, 156.2605297791399437, -1.696642280025655536 ) ) ;
#27097=CARTESIAN_POINT ( 'NONE',  ( -1.154696340448394309, 118.0995038195805904, -0.6495305470935904824 ) ) ;
#27100=CARTESIAN_POINT ( 'NONE',  ( 4.159944195614486695, 118.2392574709719497, -0.2314631920685276401 ) ) ;
#27101=CARTESIAN_POINT ( 'NONE',  ( 0.008148072696519268604, 156.3406798448389168, -0.4077628766201953359 ) ) ;
#27103=CARTESIAN_POINT ( 'NONE',  ( 3.134532381368876575, -15.16579696257060128, 3.749817985361381112 ) ) ;
#27104=CARTESIAN_POINT ( 'NONE',  ( -5.003023251195230614, 117.4023580318003184, 0.8028984813139020682 ) ) ;
#27105=CARTESIAN_POINT ( 'NONE',  ( -3.682264917456324671, 104.1064662015457287, -0.07358041635423968885 ) ) ;
#27106=CARTESIAN_POINT ( 'NONE',  ( 4.064497669612420871, 2.951628549105334898, 2.233594334442648766 ) ) ;
#27107=CARTESIAN_POINT ( 'NONE',  ( 16.66101725429939506, 148.5304741467402323, 2.032660103712368382 ) ) ;
#27108=CARTESIAN_POINT ( 'NONE',  ( 1.657835265779881828, 35.17127109692723508, 1.237340896742229690 ) ) ;
#27109=CARTESIAN_POINT ( 'NONE',  ( -6.479951895127766370, 122.5560431351108974, -0.01853871597398567064 ) ) ;
#27111=CARTESIAN_POINT ( 'NONE',  ( 1.325333094648095011, 19.28447512809159292, -4.440015753949128730 ) ) ;
#27112=CARTESIAN_POINT ( 'NONE',  ( 4.590565121197709431, 121.2030596905490540, 0.1190299148670779517 ) ) ;
#27113=CARTESIAN_POINT ( 'NONE',  ( 3.682264917456191888, 97.88346620154572975, 0.07358041635424013294 ) ) ;
#27115=CARTESIAN_POINT ( 'NONE',  ( -2.176638237496801409, 116.2240395599583564, -0.1684747500132947051 ) ) ;
#27120=CARTESIAN_POINT ( 'NONE',  ( -8.432237393326710517, 2.893158626077577900, 0.2611430682616783239 ) ) ;
#27122=DIRECTION ( 'NONE',  ( -0.9998004120163608288, -5.205824365704081956E-17, -0.01997839162482748995 ) ) ;
#27125=CARTESIAN_POINT ( 'NONE',  ( 0.05238710761679706701, 113.0327356262574341, -2.621665085262908423 ) ) ;
#27126=CARTESIAN_POINT ( 'NONE',  ( -23.28378132671084089, 148.8247458934765461, -0.01018146431420857180 ) ) ;
#27127=VERTEX_POINT ( 'NONE', #27769 ) ;
#27133=CARTESIAN_POINT ( 'NONE',  ( -9.006184665392849453, 123.9742709865185191, -0.2138692079817591241 ) ) ;
#27134=CARTESIAN_POINT ( 'NONE',  ( 3.844517683078125803, -15.15487594273597161, 5.256808347261554104 ) ) ;
#27135=CARTESIAN_POINT ( 'NONE',  ( -16.12297089460582100, 125.3625853296581312, 1.240993850804037013 ) ) ;
#27136=CARTESIAN_POINT ( 'NONE',  ( 23.02941925350872410, 142.5499849734818838, 1.196609915892170584 ) ) ;
#27137=CARTESIAN_POINT ( 'NONE',  ( 15.19088230065812617, 143.3954212834698865, 0.5062221952166892081 ) ) ;
#27138=CARTESIAN_POINT ( 'NONE',  ( 4.300553167417687561, 27.50566818391071422, -1.719522505244270860 ) ) ;
#27139=CARTESIAN_POINT ( 'NONE',  ( 0.9581433470387596962, -10.92824219907890360, 0.1848338584972420151 ) ) ;
#27140=CARTESIAN_POINT ( 'NONE',  ( -22.62002883431073741, 150.6357905964555925, -0.7802727354960531381 ) ) ;
#27142=EDGE_CURVE ( 'NONE', #32704, #37473, #36136, .T. ) ;
#27143=CARTESIAN_POINT ( 'NONE',  ( 4.862200918029492058, 117.4104105557795634, 1.165822508186273865 ) ) ;
#27144=EDGE_LOOP ( 'NONE', ( #37891, #16953 ) ) ;
#27145=CARTESIAN_POINT ( 'NONE',  ( -8.789204892644862710, 117.7553426919097745, 0.1101893534113697198 ) ) ;
#27146=CARTESIAN_POINT ( 'NONE',  ( -0.5348915910374654192, 119.5442839488369628, 0.5285302399602643808 ) ) ;
#27148=CARTESIAN_POINT ( 'NONE',  ( 19.59580906854006699, 147.4874203640471535, -1.738765900131762576 ) ) ;
#27149=CARTESIAN_POINT ( 'NONE',  ( 0.9235644399502331847, -7.204839741120207641, 0.3177745608231433705 ) ) ;
#27150=CARTESIAN_POINT ( 'NONE',  ( -13.86838617718244393, 121.5005676099359846, -1.565740997395133949 ) ) ;
#27152=FACE_OUTER_BOUND ( 'NONE', #26342, .T. ) ;
#27153=CARTESIAN_POINT ( 'NONE',  ( 12.34427413551888719, 128.4316967252784991, -0.8534409008407578545 ) ) ;
#27154=CARTESIAN_POINT ( 'NONE',  ( -14.67500508075667298, 148.8517222230099719, -0.2932415260845991356 ) ) ;
#27155=EDGE_LOOP ( 'NONE', ( #36793, #2257, #11948, #38157 ) ) ;
#27156=CARTESIAN_POINT ( 'NONE',  ( -17.40616913868966620, 140.3598469681121514, -2.385085200778919834 ) ) ;
#27157=CARTESIAN_POINT ( 'NONE',  ( 4.642828252855901283, -15.60299999947604910, 2.403246459791627210 ) ) ;
#27158=CARTESIAN_POINT ( 'NONE',  ( -6.513165593194060347E-14, 68.92746620154572668, -8.865348866426607246E-18 ) ) ;
#27159=CARTESIAN_POINT ( 'NONE',  ( -4.434135272687235840, 118.1246147528386530, -0.7353779375332715196 ) ) ;
#27162=CARTESIAN_POINT ( 'NONE',  ( 4.756814333351318425, 117.4032681585794791, 1.206529664789174339 ) ) ;
#27163=CARTESIAN_POINT ( 'NONE',  ( 15.09997037988943802, 131.2890697635526465, 2.122864649987123098 ) ) ;
#27165=EDGE_CURVE ( 'NONE', #29654, #36953, #22467, .T. ) ;
#27166=VECTOR ( 'NONE', #16321, 1000.000000000000227 ) ;
#27168=CARTESIAN_POINT ( 'NONE',  ( 4.717508175643458479, 116.7562497393984415, 0.08034061319516429267 ) ) ;
#27170=CARTESIAN_POINT ( 'NONE',  ( 6.435022864794023079, 6.566661361801033436, 5.478585407919045025 ) ) ;
#27171=CARTESIAN_POINT ( 'NONE',  ( 7.919085485410333192, 154.5997988942315260, 0.6546929905378093828 ) ) ;
#27172=CARTESIAN_POINT ( 'NONE',  ( 1.024802081479738280, 117.0751458430253393, -0.3787107017154777155 ) ) ;
#27175=CARTESIAN_POINT ( 'NONE',  ( -16.23473294303261483, 121.3954344197762083, -0.2182100806314834218 ) ) ;
#27178=CARTESIAN_POINT ( 'NONE',  ( 5.954738066914381456, 121.4009902524702369, -0.05856541418628991025 ) ) ;
#27179=DIRECTION ( 'NONE',  ( 4.017660918040594346E-17, -1.000000000000000000, -2.376309959284834438E-19 ) ) ;
#27181=CARTESIAN_POINT ( 'NONE',  ( 0.5071815534827258665, 115.7034655862730830, -1.744310922642317907 ) ) ;
#27182=CARTESIAN_POINT ( 'NONE',  ( -9.426771831325675421, 124.2753396726362780, -0.5138045435804896588 ) ) ;
#27183=CARTESIAN_POINT ( 'NONE',  ( 3.798736437616232919, -14.27876630094554500, 4.860596070177301442 ) ) ;
#27184=CARTESIAN_POINT ( 'NONE',  ( -8.033985789953094425, 118.2752802814886053, 0.7207832311977436790 ) ) ;
#27186=CARTESIAN_POINT ( 'NONE',  ( 0.8970928355477491012, 116.4604358222411236, 0.08699291512134199600 ) ) ;
#27188=CARTESIAN_POINT ( 'NONE',  ( -2.983771112188844832, -5.329111280313512999, 3.548611825089460048 ) ) ;
#27189=CARTESIAN_POINT ( 'NONE',  ( -15.72148175706237971, 120.8394623874526275, -0.3311059221235124195 ) ) ;
#27190=DIRECTION ( 'NONE',  ( 0.01997839162482749689, 1.040247600000945640E-18, -0.9998004120163610509 ) ) ;
#27191=AXIS2_PLACEMENT_3D ( 'NONE', #31344, #20960, #24956 ) ;
#27194=CARTESIAN_POINT ( 'NONE',  ( 6.430476594291733683, 119.6278830040221948, 1.257881746540687740 ) ) ;
#27196=CARTESIAN_POINT ( 'NONE',  ( -3.029891238501105644, -9.367638731076009861, 3.490193963561483148 ) ) ;
#27197=CARTESIAN_POINT ( 'NONE',  ( 22.02091170609368831, 149.7938220333360846, 1.879853634988783551 ) ) ;
#27199=CARTESIAN_POINT ( 'NONE',  ( 13.60271346700648465, 122.2126086331852974, -1.213557020469313574 ) ) ;
#27200=CARTESIAN_POINT ( 'NONE',  ( -2.488979065607898722, -9.142725400274830605, 3.900846118434742493 ) ) ;
#27201=CARTESIAN_POINT ( 'NONE',  ( -5.389281185859767120, 158.9671755112622122, -1.064713296837521694 ) ) ;
#27204=EDGE_CURVE ( 'NONE', #26282, #41701, #37477, .T. ) ;
#27205=CARTESIAN_POINT ( 'NONE',  ( -8.936721596564296988, 123.7033391712731145, 0.04711667938246253545 ) ) ;
#27206=CARTESIAN_POINT ( 'NONE',  ( 6.387155697962850986, -12.89254730397265725, 0.3290856906432634288 ) ) ;
#27209=DIRECTION ( 'NONE',  ( 5.206863593109713661E-17, -1.000000000000000000, 1.077750396879097183E-30 ) ) ;
#27210=ORIENTED_EDGE ( 'NONE', *, *, #10863, .F. ) ;
#27211=CARTESIAN_POINT ( 'NONE',  ( 11.61050889437339784, 122.1450671466348439, 1.749762830748087694 ) ) ;
#27213=CARTESIAN_POINT ( 'NONE',  ( 4.756911902486301358, 117.3993836135862949, 1.207145067066230038 ) ) ;
#27214=CARTESIAN_POINT ( 'NONE',  ( -14.59306090326471050, 120.9595740141730289, 0.6228583445698290255 ) ) ;
#27216=CARTESIAN_POINT ( 'NONE',  ( -3.896388542364412455, 10.26897056970580380, 7.485861278012786002 ) ) ;
#27217=CARTESIAN_POINT ( 'NONE',  ( 7.725927843277549556, 122.1869765257964673, 0.7315739442948010485 ) ) ;
#27218=CARTESIAN_POINT ( 'NONE',  ( -3.682264917456324227, 91.02546620154572565, -0.07358041635423968885 ) ) ;
#27219=CIRCLE ( 'NONE', #40166, 3.175000000000001155 ) ;
#27220=CARTESIAN_POINT ( 'NONE',  ( 21.14621813959886865, 132.3956117394162106, -0.2431941713936562333 ) ) ;
#27222=EDGE_CURVE ( 'NONE', #35734, #38903, #777, .T. ) ;
#27227=CARTESIAN_POINT ( 'NONE',  ( -4.496509515934371315, 118.1299520530536569, 0.5225237042064447834 ) ) ;
#27228=CARTESIAN_POINT ( 'NONE',  ( 2.934006498407145447, 107.6241103294071451, -4.446763787522097999 ) ) ;
#27231=CARTESIAN_POINT ( 'NONE',  ( -8.281850670998682773, 120.0774609856632225, -1.450002526945398218 ) ) ;
#27232=CARTESIAN_POINT ( 'NONE',  ( -7.669269000495163802, 124.9344662015457317, -0.1532502464757266591 ) ) ;
#27233=CARTESIAN_POINT ( 'NONE',  ( 4.481705483751912134, 118.1291794842778273, 0.6917936338195805890 ) ) ;
#27234=CARTESIAN_POINT ( 'NONE',  ( -4.540840819607181444, 155.9125706774115940, -0.9348598387858669811 ) ) ;
#27235=CARTESIAN_POINT ( 'NONE',  ( -1.405640664959715513, 115.7027605823517717, -1.735603269989020703 ) ) ;
#27237=CARTESIAN_POINT ( 'NONE',  ( 4.018990735853727791, 117.3993838140831230, -1.158690488846763955 ) ) ;
#27238=CARTESIAN_POINT ( 'NONE',  ( 5.287753629968712232, 116.2229785614576798, -0.9666386099593877734 ) ) ;
#27239=CARTESIAN_POINT ( 'NONE',  ( -10.33865867007045125, 123.8962982355681817, -1.239266749756491093 ) ) ;
#27241=CARTESIAN_POINT ( 'NONE',  ( 8.618292403345778396, 118.6571538964698931, -0.8118115907002622089 ) ) ;
#27242=CARTESIAN_POINT ( 'NONE',  ( -15.38532232246978282, 147.8388113238944186, -0.1074854512288092867 ) ) ;
#27244=CARTESIAN_POINT ( 'NONE',  ( 9.590549175011847893, 118.2964180356302961, 0.8317573021886300877 ) ) ;
#27246=CARTESIAN_POINT ( 'NONE',  ( 3.113553847179573175, -14.91884098843750195, 3.610284256090800170 ) ) ;
#27248=CARTESIAN_POINT ( 'NONE',  ( -18.37664568872251181, 148.6295804641074483, 1.698537578660717973 ) ) ;
#27249=CARTESIAN_POINT ( 'NONE',  ( -0.7773729966126706747, -2.891840825076433585, -0.5888577047253038543 ) ) ;
#27250=CARTESIAN_POINT ( 'NONE',  ( -2.849674052733137231, 116.8186761214209213, -0.3958730627374473232 ) ) ;
#27251=CARTESIAN_POINT ( 'NONE',  ( 0.8739363859948088287, 22.79536383596403226, -0.4369566804381688208 ) ) ;
#27254=CARTESIAN_POINT ( 'NONE',  ( 5.752478121743081374, 118.4424948052634647, 0.6632437998952304126 ) ) ;
#27256=CARTESIAN_POINT ( 'NONE',  ( -13.50624371993754558, 134.2048320552371763, 0.5584564168634340575 ) ) ;
#27257=CARTESIAN_POINT ( 'NONE',  ( 3.288375567735513094, -14.78372392556953585, 5.458595067156710279 ) ) ;
#27258=CARTESIAN_POINT ( 'NONE',  ( 1.430496892223362293, 119.9358631726476574, -0.4886406555826710019 ) ) ;
#27260=CARTESIAN_POINT ( 'NONE',  ( 3.897805094888262989, 104.6144662015456817, 2.864625572161799916 ) ) ;
#27262=CARTESIAN_POINT ( 'NONE',  ( 3.282182858002726356, -14.11059071864860570, 3.604430013830858037 ) ) ;
#27263=CARTESIAN_POINT ( 'NONE',  ( -4.908372319998136390, 117.6281534842222669, -0.9701036486395447911 ) ) ;
#27264=CARTESIAN_POINT ( 'NONE',  ( 9.188648150231653489, 124.1858035287836231, 0.09819667026458973880 ) ) ;
#27266=CARTESIAN_POINT ( 'NONE',  ( 4.954158841009532743, 118.5534682650580862, 1.066189120819955427 ) ) ;
#27267=CARTESIAN_POINT ( 'NONE',  ( 3.276466505201106827, 108.4907294079988418, 4.202205409544957249 ) ) ;
#27270=AXIS2_PLACEMENT_3D ( 'NONE', #34804, #12839, #16230 ) ;
#27272=CARTESIAN_POINT ( 'NONE',  ( 0.01133159106138491301, 159.5297144918048673, -0.5670791535570575137 ) ) ;
#27273=CARTESIAN_POINT ( 'NONE',  ( 23.41759249777140539, 146.8136392739129974, 0.2357739188755809401 ) ) ;
#27274=CYLINDRICAL_SURFACE ( 'NONE', #11816, 3.175000000000001155 ) ;
#27275=CIRCLE ( 'NONE', #32730, 5.080000000000006288 ) ;
#27276=CARTESIAN_POINT ( 'NONE',  ( 1.921025692115251982, -15.60942222372031729, 5.455320770239441508 ) ) ;
#27278=CARTESIAN_POINT ( 'NONE',  ( -4.969430860872935618, 117.5911946925397871, -0.8218521176953593743 ) ) ;
#27279=CARTESIAN_POINT ( 'NONE',  ( 20.53125589898976244, 145.6130255286810495, 2.451886524809591350 ) ) ;
#27281=CARTESIAN_POINT ( 'NONE',  ( -7.794209556482943668, 13.03656553185805222, 3.210957146378262461 ) ) ;
#27282=CARTESIAN_POINT ( 'NONE',  ( 2.482649978626910059, 117.4442030770385941, -0.6349463395262938681 ) ) ;
#27283=CARTESIAN_POINT ( 'NONE',  ( -2.302803873444659644, 118.9955205646042344, -0.7292456921539737236 ) ) ;
#27286=CARTESIAN_POINT ( 'NONE',  ( -0.01180776361650071223, 120.3637084677655764, 0.5909087754570012674 ) ) ;
#27287=CARTESIAN_POINT ( 'NONE',  ( 4.076717266748975277, 8.489475128091552136, -2.202413229635628689 ) ) ;
#27289=CARTESIAN_POINT ( 'NONE',  ( -4.765964266679635131, 118.5264896598256854, 0.8411723569164160086 ) ) ;
#27290=CARTESIAN_POINT ( 'NONE',  ( 3.260250311156894121, -12.89034478651954174, 1.323980178024680043 ) ) ;
#27291=CARTESIAN_POINT ( 'NONE',  ( 0.9873284109326271318, 106.8474934270474392, -4.901623504225490535 ) ) ;
#27292=CARTESIAN_POINT ( 'NONE',  ( 1.952296795662580298, 38.90900249396371180, 1.348506300408716552 ) ) ;
#27295=CARTESIAN_POINT ( 'NONE',  ( -3.054491883998568191, 105.1240845014440453, -4.374327510956630860 ) ) ;
#27296=CARTESIAN_POINT ( 'NONE',  ( 3.739721301978734314, -15.76301488427489517, 4.305968564470687987 ) ) ;
#27297=CARTESIAN_POINT ( 'NONE',  ( -19.50591060256589415, 149.0830822498907082, 1.724197071773047707 ) ) ;
#27299=CARTESIAN_POINT ( 'NONE',  ( 1.104432469574216480, -9.427232690354344413, -4.492858291722996888 ) ) ;
#27303=CARTESIAN_POINT ( 'NONE',  ( 2.988627099740976512, 122.7580772961051707, 0.2146329844597062719 ) ) ;
#27305=CARTESIAN_POINT ( 'NONE',  ( -14.53352838467451313, 150.4300676932417389, 1.118949361739814519 ) ) ;
#27306=DIRECTION ( 'NONE',  ( -4.017660918040594346E-17, 1.000000000000000000, 2.376309959284834438E-19 ) ) ;
#27307=CARTESIAN_POINT ( 'NONE',  ( 0.5348915910373366334, 119.5442839488369628, -0.5285302399602642698 ) ) ;
#27309=CARTESIAN_POINT ( 'NONE',  ( -20.67294874948574801, 147.9587796579421308, -2.444796510662507139 ) ) ;
#27311=CARTESIAN_POINT ( 'NONE',  ( 4.287347022130586716, 118.2136450426441598, -0.3572067982262181474 ) ) ;
#27312=CARTESIAN_POINT ( 'NONE',  ( 5.231962949222344506, 121.1607713875043117, -0.2380388119251649337 ) ) ;
#27314=CARTESIAN_POINT ( 'NONE',  ( 2.931439949929583122, -14.82325452411255640, 4.117531814738872420 ) ) ;
#27318=EDGE_CURVE ( 'NONE', #10591, #32067, #5994, .T. ) ;
#27319=CARTESIAN_POINT ( 'NONE',  ( 4.135298993362768627, -14.76517611359900961, -2.065434832541708676 ) ) ;
#27320=CARTESIAN_POINT ( 'NONE',  ( 13.16414530391289617, 152.2904283036577908, 1.902647459344306791 ) ) ;
#27321=CARTESIAN_POINT ( 'NONE',  ( 2.928799644063047936, 38.81416391459460158, 1.351591292951386469 ) ) ;
#27322=CARTESIAN_POINT ( 'NONE',  ( -5.936300781872430932, 120.8604418758245487, 0.1421746502253222466 ) ) ;
#27325=CARTESIAN_POINT ( 'NONE',  ( -0.5093740622119584671, 14.76157059199007016, 4.595130897425484306 ) ) ;
#27326=CARTESIAN_POINT ( 'NONE',  ( 15.72560005962091800, 146.8994026175788008, 0.4425663129111797600 ) ) ;
#27329=CARTESIAN_POINT ( 'NONE',  ( 2.179771977182863640, 116.2367762333986718, -0.09915394068943080008 ) ) ;
#27330=CARTESIAN_POINT ( 'NONE',  ( 0.003708075274061980488, 123.1683257372384901, -0.1855672496570262564 ) ) ;
#27334=CARTESIAN_POINT ( 'NONE',  ( -2.337594367139880003, 4.813278044257511823, 8.129740476481943645 ) ) ;
#27338=CARTESIAN_POINT ( 'NONE',  ( 0.005099097579422138225, 122.5569158606516993, -0.2551796940111168976 ) ) ;
#27339=CARTESIAN_POINT ( 'NONE',  ( -5.826550815406482009, 117.0573985505404693, 0.1859578237674348045 ) ) ;
#27344=CARTESIAN_POINT ( 'NONE',  ( -7.546549060383340723, 122.4259254537243464, -0.1108676762560423107 ) ) ;
#27345=CARTESIAN_POINT ( 'NONE',  ( 5.611968257679588845, -14.69514533571547688, 3.041973840610588287 ) ) ;
#27346=CARTESIAN_POINT ( 'NONE',  ( -20.57754816582981405, 149.5144255282053223, 1.563875036196712642 ) ) ;
#27347=CARTESIAN_POINT ( 'NONE',  ( 23.13850227319423780, 149.2833505036244048, 1.057685438456114957 ) ) ;
#27348=CARTESIAN_POINT ( 'NONE',  ( 5.427513099616278147, 158.9671755112622122, -0.8485680044740093741 ) ) ;
#27350=CARTESIAN_POINT ( 'NONE',  ( -20.28976221201026320, 128.9598305440861452, -0.6839793015867964288 ) ) ;
#27353=CARTESIAN_POINT ( 'NONE',  ( 5.556916953519710489, 116.7209935381689974, 0.2595115648362693594 ) ) ;
#27354=CARTESIAN_POINT ( 'NONE',  ( -15.71777585039863645, 134.9797526104055123, 1.508943449597504705 ) ) ;
#27357=CARTESIAN_POINT ( 'NONE',  ( 8.434619947227306014, 156.6436466068687423, -1.738452918000226388 ) ) ;
#27358=CARTESIAN_POINT ( 'NONE',  ( 0.5763570944828283471, -5.266575483494631449, -0.7860673829877594665 ) ) ;
#27359=CARTESIAN_POINT ( 'NONE',  ( -21.10167996235837862, 141.7209635633906259, -2.240609589767335041 ) ) ;
#27363=CARTESIAN_POINT ( 'NONE',  ( 16.60605961459992130, 147.5857818452174115, -1.108006280952564815 ) ) ;
#27366=CARTESIAN_POINT ( 'NONE',  ( -18.34612162485809606, 147.3262642721504960, -2.396769171045068703 ) ) ;
#27367=CARTESIAN_POINT ( 'NONE',  ( 4.856922264871083250, -15.58127974107270575, 2.741789226191331252 ) ) ;
#27369=CARTESIAN_POINT ( 'NONE',  ( -4.303161701476582834, 118.2117301101246341, -0.4941263280093639021 ) ) ;
#27373=CARTESIAN_POINT ( 'NONE',  ( 4.106383402388294357, 118.2429491485453354, 0.3519430347307819229 ) ) ;
#27374=CARTESIAN_POINT ( 'NONE',  ( 18.09674421129283672, 146.7121067869193496, 2.346545542165937803 ) ) ;
#27375=CARTESIAN_POINT ( 'NONE',  ( 23.36121599382897074, 148.8756354988261990, 0.4668126921608657942 ) ) ;
#27376=CARTESIAN_POINT ( 'NONE',  ( -0.9514613986627886710, 10.21077804425927305, -8.405459466743828045 ) ) ;
#27377=CARTESIAN_POINT ( 'NONE',  ( 15.32065199451904647, 143.5038931315047535, 0.7650733020788533789 ) ) ;
#27379=CARTESIAN_POINT ( 'NONE',  ( 10.39199171643957698, 157.8614378686282862, -0.7539791864280579459 ) ) ;
#27380=CARTESIAN_POINT ( 'NONE',  ( 5.332935397695205637, 105.1224662015457199, 0.1065647409268305201 ) ) ;
#27381=CARTESIAN_POINT ( 'NONE',  ( 3.999888396376028332, 115.6909491485452435, 1.587082580931593379 ) ) ;
#27384=CARTESIAN_POINT ( 'NONE',  ( -21.90557141593814094, 151.4352167165723415, -0.3614719721193417334 ) ) ;
#27387=CARTESIAN_POINT ( 'NONE',  ( -5.800372561083844580, 121.2106355307726346, -0.4875482425884115623 ) ) ;
#27389=CARTESIAN_POINT ( 'NONE',  ( 0.4392373074537823663, 115.6909491485452719, -1.750094695205981044 ) ) ;
#27390=CARTESIAN_POINT ( 'NONE',  ( -13.62587875280891581, 150.2122286517991085, -0.5925390977946540794 ) ) ;
#27391=CARTESIAN_POINT ( 'NONE',  ( 4.721845526343314781, -13.23797770169883670, 3.222865150663026590 ) ) ;
#27392=CARTESIAN_POINT ( 'NONE',  ( -14.19262213114356896, 155.9232964860746620, 1.164639009528573022 ) ) ;
#27394=CARTESIAN_POINT ( 'NONE',  ( 23.27880353394119339, 149.3453998935430604, 0.6192278183506786382 ) ) ;
#27395=CARTESIAN_POINT ( 'NONE',  ( 10.39478676155560244, 153.1349730030725595, 0.2678714069608246762 ) ) ;
#27397=CARTESIAN_POINT ( 'NONE',  ( 0.9280917288853990366, 18.63875360461660335, -0.3060232888646727822 ) ) ;
#27399=CARTESIAN_POINT ( 'NONE',  ( -10.82992898448790520, 157.9016520041087688, -0.2364045824791623507 ) ) ;
#27401=CIRCLE ( 'NONE', #30795, 3.683000000000001162 ) ;
#27404=CARTESIAN_POINT ( 'NONE',  ( 5.609552972221978351, 119.8608102258102690, 1.095074600700395306 ) ) ;
#27405=CARTESIAN_POINT ( 'NONE',  ( 4.587442282481145384, -5.694351208059624803, -0.5507456681084095251 ) ) ;
#27406=CARTESIAN_POINT ( 'NONE',  ( 10.97563396989510132, 119.3804150619309468, 1.219877759958876595 ) ) ;
#27408=CARTESIAN_POINT ( 'NONE',  ( 6.797121414357278901, 118.7881172115286148, -0.9472104157431980864 ) ) ;
#27409=CARTESIAN_POINT ( 'NONE',  ( 3.573240411403531436, -4.819783300376494495, -2.961220487682876268 ) ) ;
#27410=CARTESIAN_POINT ( 'NONE',  ( -19.15327062675862280, 128.6826163344482268, -1.506695251711823058 ) ) ;
#27413=CARTESIAN_POINT ( 'NONE',  ( -6.023029630345043905, 155.3544091381320982, 0.1360875627331028515 ) ) ;
#27414=CARTESIAN_POINT ( 'NONE',  ( 2.468517452056580463, -15.43523125850157562, 5.870468177969554446 ) ) ;
#27415=CARTESIAN_POINT ( 'NONE',  ( 5.167420783512489457, 115.6909491485453145, 1.238004321684439191 ) ) ;
#27417=CARTESIAN_POINT ( 'NONE',  ( -0.5456937337276765998, 117.3993834314855462, -1.492633053494221596 ) ) ;
#27419=CARTESIAN_POINT ( 'NONE',  ( 5.003445044761828164, 119.2220797256985350, 1.100019038710256414 ) ) ;
#27423=CARTESIAN_POINT ( 'NONE',  ( -5.863496024706905452, 117.4684171610355747, 0.5179920176435335311 ) ) ;
#27424=CARTESIAN_POINT ( 'NONE',  ( -8.197529660144020625, 8.984976746712527884, 2.078235512056660017 ) ) ;
#27425=CARTESIAN_POINT ( 'NONE',  ( 15.16020740373466325, 148.9716719698033387, 1.401450122450045521 ) ) ;
#27427=EDGE_CURVE ( 'NONE', #32767, #21511, #38851, .T. ) ;
#27428=CARTESIAN_POINT ( 'NONE',  ( 23.06568927493560750, 148.7220611141358404, -0.3950670065760722438 ) ) ;
#27433=CARTESIAN_POINT ( 'NONE',  ( -4.120329755912500502, 118.2429491485453354, 0.1840211939346729775 ) ) ;
#27434=CARTESIAN_POINT ( 'NONE',  ( 3.444129741522558685, 108.1634925278479500, -4.064689422066845026 ) ) ;
#27438=CARTESIAN_POINT ( 'NONE',  ( 6.316787761850397587, 119.8961530332412195, -0.9708787764513430174 ) ) ;
#27439=CARTESIAN_POINT ( 'NONE',  ( -6.329649118423223086, 120.0627515544778134, -0.4542292512502629220 ) ) ;
#27441=CARTESIAN_POINT ( 'NONE',  ( 4.392636428124883530, 118.1805772463083599, 0.5719164910104670430 ) ) ;
#27442=CARTESIAN_POINT ( 'NONE',  ( -16.11589901136889935, 145.8839827664328368, -1.295141180005177528 ) ) ;
#27443=CARTESIAN_POINT ( 'NONE',  ( -0.9954745042087072004, 115.7029401122920973, -1.748196735769753873 ) ) ;
#27444=CARTESIAN_POINT ( 'NONE',  ( 2.732111087507031133, 116.5293111276780849, 0.05459408159141355271 ) ) ;
#27446=CARTESIAN_POINT ( 'NONE',  ( 1.581412096509125842, 106.2431249238853894, -5.111785082781967304 ) ) ;
#27447=CARTESIAN_POINT ( 'NONE',  ( -4.409042980950640178, 120.6578283891288379, -0.6218799582752131405 ) ) ;
#27448=B_SPLINE_CURVE_WITH_KNOTS ( 'NONE', 3,
 ( #30673, #34309, #15101, #1521, #40496, #11291 ),
 .UNSPECIFIED., .F., .F.,
 ( 4, 2, 4 ),
 ( 0.000000000000000000, 0.5000000000000000000, 1.000000000000000000 ),
 .UNSPECIFIED. ) ;
#27452=CARTESIAN_POINT ( 'NONE',  ( -9.059071224495744090, 124.2128079895686170, -0.04632541238150574697 ) ) ;
#27455=CARTESIAN_POINT ( 'NONE',  ( 22.93196816944033856, 148.6798292920915117, 1.431318312106270474 ) ) ;
#27457=CARTESIAN_POINT ( 'NONE',  ( 2.770264620702337588, -13.86593384134129892, 0.2159450460461957433 ) ) ;
#27458=CARTESIAN_POINT ( 'NONE',  ( 21.68796372492886704, 149.3076860495818323, -1.274097349589627282 ) ) ;
#27459=CARTESIAN_POINT ( 'NONE',  ( -0.03212616895158381530, 157.6269964811067155, 1.607724863813389415 ) ) ;
#27460=CARTESIAN_POINT ( 'NONE',  ( 0.9235644399502331847, -7.204839741120207641, 0.3177745608231433705 ) ) ;
#27461=CARTESIAN_POINT ( 'NONE',  ( -3.829241263245407367, 116.9593488885201538, -0.4901781634895738260 ) ) ;
#27462=AXIS2_PLACEMENT_3D ( 'NONE', #27105, #3923, #4346 ) ;
#27464=CARTESIAN_POINT ( 'NONE',  ( -0.7014129483091587902, 16.11884676413550466, -0.6771123631929140130 ) ) ;
#27466=B_SPLINE_CURVE_WITH_KNOTS ( 'NONE', 3,
 ( #2348, #14885, #31289, #41318, #28095, #8930, #28522, #41530, #9146, #25323, #37693, #22104, #35132 ),
 .UNSPECIFIED., .F., .F.,
 ( 4, 1, 1, 1, 1, 1, 1, 1, 1, 1, 4 ),
 ( 0.000000000000000000, 0.1249999999999999167, 0.1767086109055020227, 0.2499999999999998335, 0.3750000000000003886, 0.5000000000000003331, 0.5890287030183404271, 0.6249999999999998890, 0.7499999999999995559, 0.8749999999999997780, 1.000000000000000000 ),
 .UNSPECIFIED. ) ;
#27468=CARTESIAN_POINT ( 'NONE',  ( -8.914966108837955261, 123.2307073318660855, 0.3922733289213622410 ) ) ;
#27469=CARTESIAN_POINT ( 'NONE',  ( 2.370890509137566937, -15.02769382788871155, 5.804473790077508077 ) ) ;
#27470=CARTESIAN_POINT ( 'NONE',  ( 4.378102236263064384, 120.3584862571861436, -0.5730137456143137298 ) ) ;
#27474=CARTESIAN_POINT ( 'NONE',  ( 3.202083396006969895, -13.65749169606385394, 1.964591208077046902 ) ) ;
#27475=CARTESIAN_POINT ( 'NONE',  ( -5.212520885064538589, 31.45212241211192605, -0.4657032193360506334 ) ) ;
#27476=CARTESIAN_POINT ( 'NONE',  ( 8.794423163103090246, 123.6850765633735421, 0.1423839433359068429 ) ) ;
#27478=CARTESIAN_POINT ( 'NONE',  ( 6.734570810858505396, 118.9580315507705706, 1.247721039026444600 ) ) ;
#27479=CARTESIAN_POINT ( 'NONE',  ( 1.187367250949410868, 106.3000011757731187, 5.151998247764457695 ) ) ;
#27483=CARTESIAN_POINT ( 'NONE',  ( 0.002426349801083684584, 116.5266044092193880, -0.1214244658147704270 ) ) ;
#27486=CARTESIAN_POINT ( 'NONE',  ( 1.844779171034190757, -15.45366112431178962, 5.998838294486427358 ) ) ;
#27489=EDGE_CURVE ( 'NONE', #11121, #5326, #25237, .T. ) ;
#27490=CARTESIAN_POINT ( 'NONE',  ( -4.744868711034945896, 117.8975728021022604, 0.7672496759666370680 ) ) ;
#27492=CARTESIAN_POINT ( 'NONE',  ( -6.929632415086860675, 11.50928017261270497, -4.815005168835179816 ) ) ;
#27494=CARTESIAN_POINT ( 'NONE',  ( -8.398419497799205047, 119.5137114544897088, -1.401694671710796314 ) ) ;
#27495=CARTESIAN_POINT ( 'NONE',  ( -3.099458292115011115, 117.0475107411037641, -1.222660999933594450 ) ) ;
#27497=CARTESIAN_POINT ( 'NONE',  ( 4.726358237794381800, 117.7280284874452860, 1.096895477954969556 ) ) ;
#27499=CARTESIAN_POINT ( 'NONE',  ( -0.01635612297686582159, 119.2343925067225427, 0.8185272769044252827 ) ) ;
#27500=CARTESIAN_POINT ( 'NONE',  ( 1.068493265602401987, 5.690783753869971484, 4.496582723949734017 ) ) ;
#27502=CARTESIAN_POINT ( 'NONE',  ( -5.252607328145010079, 115.6909491485453003, 0.9237163795073232153 ) ) ;
#27503=CARTESIAN_POINT ( 'NONE',  ( 3.201139452527619333, -14.28037012539873274, 4.574913560108570643 ) ) ;
#27504=CARTESIAN_POINT ( 'NONE',  ( 4.107119205180127963, 117.8719421043398370, -0.6926522829710090035 ) ) ;
#27505=CARTESIAN_POINT ( 'NONE',  ( -4.456559794634359584, 27.80638087737987973, 0.5384073243751467119 ) ) ;
#27506=CARTESIAN_POINT ( 'NONE',  ( -1.423643091077623879, 115.7027630026304337, 1.681650016434340422 ) ) ;
#27507=ORIENTED_EDGE ( 'NONE', *, *, #7319, .T. ) ;
#27508=CARTESIAN_POINT ( 'NONE',  ( -5.183055225334214811, 105.1221871011891125, -1.273223601473996158 ) ) ;
#27509=AXIS2_PLACEMENT_3D ( 'NONE', #13652, #32408, #26432 ) ;
#27510=CARTESIAN_POINT ( 'NONE',  ( 5.161689517976459030, -15.45231451347503437, 1.550260198497607877 ) ) ;
#27511=CARTESIAN_POINT ( 'NONE',  ( -19.17595810167867398, 140.9752145814059645, 1.751973952106584020 ) ) ;
#27513=CARTESIAN_POINT ( 'NONE',  ( -0.9636992805836054332, 23.18535052081312386, 0.1494942155713751553 ) ) ;
#27516=CARTESIAN_POINT ( 'NONE',  ( -4.230865311087580238, 31.47871655110595768, -0.6839938589234777488 ) ) ;
#27517=CARTESIAN_POINT ( 'NONE',  ( 2.726848673931656197, 121.4869043954268903, 0.3408589522888662571 ) ) ;
#27519=CARTESIAN_POINT ( 'NONE',  ( -3.575420174884087476, 120.5283240077024800, 0.4162329711438423341 ) ) ;
#27521=CARTESIAN_POINT ( 'NONE',  ( 4.519236749211172466, 118.0837734081209192, -0.6171982530284805257 ) ) ;
#27522=CARTESIAN_POINT ( 'NONE',  ( 1.377724515701647334, 119.5584937100158243, -0.5648184346096530861 ) ) ;
#27523=CARTESIAN_POINT ( 'NONE',  ( -0.4261125263670469954, 118.2558431149878402, -0.5943921922486901099 ) ) ;
#27526=CARTESIAN_POINT ( 'NONE',  ( 4.288979916322937846, 118.2138448364286347, -0.3554799478401594048 ) ) ;
#27527=CARTESIAN_POINT ( 'NONE',  ( 5.903620821223727333, 121.4229528491920576, -0.1845582724821505927 ) ) ;
#27528=ORIENTED_EDGE ( 'NONE', *, *, #26904, .F. ) ;
#27529=CARTESIAN_POINT ( 'NONE',  ( 3.076715286590720133, -14.17522324541667444, 1.337940584860995319 ) ) ;
#27532=CARTESIAN_POINT ( 'NONE',  ( -3.538659794179211726, -11.74154716455626257, -2.972011832598964176 ) ) ;
#27533=CARTESIAN_POINT ( 'NONE',  ( 17.14717842969334072, 147.4900653055648547, 2.050122926623737740 ) ) ;
#27534=CARTESIAN_POINT ( 'NONE',  ( 1.733480476724572172, 35.69352191795299944, 2.306000102516378991 ) ) ;
#27535=CARTESIAN_POINT ( 'NONE',  ( -0.3401008104888438854, 105.9117620634264370, 5.317146732969808554 ) ) ;
#27536=CARTESIAN_POINT ( 'NONE',  ( -1.544744425833544099, 4.816215111148435923, 4.377641278133862279 ) ) ;
#27537=CARTESIAN_POINT ( 'NONE',  ( 9.075584820321502377, 124.0722828908287454, 0.2154388746608567884 ) ) ;
#27541=CARTESIAN_POINT ( 'NONE',  ( -5.535853918629470627, 116.8115403336140474, -0.4677966508803286794 ) ) ;
#27544=CARTESIAN_POINT ( 'NONE',  ( -0.3947539175594134142, 105.8842979884933726, 5.327223850753324719 ) ) ;
#27546=CARTESIAN_POINT ( 'NONE',  ( -7.218840658378264052, 2.017470825009220370, -4.342437029863850384 ) ) ;
#27550=CARTESIAN_POINT ( 'NONE',  ( 0.007670926888197925585, 121.5961256765098284, -0.3838845493045227597 ) ) ;
#27551=CARTESIAN_POINT ( 'NONE',  ( -0.004355829920665829462, 116.7171338949676738, 0.2179835409713599403 ) ) ;
#27556=CARTESIAN_POINT ( 'NONE',  ( -1.561582345843753217, 156.2588034088681184, -0.03120413162939504950 ) ) ;
#27557=CARTESIAN_POINT ( 'NONE',  ( 4.692294315076144251, -14.85586321182354119, 4.526698459197877611 ) ) ;
#27558=CARTESIAN_POINT ( 'NONE',  ( -20.41374081727979473, 149.7738053052645171, 1.564883410832889510 ) ) ;
#27559=CARTESIAN_POINT ( 'NONE',  ( 5.868821994818586241, 117.5931221156369730, -0.5844160582045566654 ) ) ;
#27560=CARTESIAN_POINT ( 'NONE',  ( -4.374560056058969693, 13.03735028915297534, 1.504755201125916875 ) ) ;
#27561=CARTESIAN_POINT ( 'NONE',  ( -22.58551839157542318, 137.2245694613254443, -0.7673259740012311481 ) ) ;
#27564=CARTESIAN_POINT ( 'NONE',  ( -12.79346581414816697, 125.9836878220586556, 1.262672879670394321 ) ) ;
#27566=CARTESIAN_POINT ( 'NONE',  ( 11.96109417309357958, 154.9039014673913073, -1.746238851223627764 ) ) ;
#27567=CARTESIAN_POINT ( 'NONE',  ( -21.49578583461358150, 148.6087350971780836, -2.244132633923697107 ) ) ;
#27569=CARTESIAN_POINT ( 'NONE',  ( 12.09414715658290085, 128.3964238929853252, -0.7197952935306336508 ) ) ;
#27571=ORIENTED_EDGE ( 'NONE', *, *, #20655, .F. ) ;
#27572=CARTESIAN_POINT ( 'NONE',  ( -9.271712722858243438, 121.5662863950884400, -1.459403803239323505 ) ) ;
#27573=CARTESIAN_POINT ( 'NONE',  ( 1.925067723532086994, -15.61332249492565438, 5.452854070638914585 ) ) ;
#27574=CARTESIAN_POINT ( 'NONE',  ( -4.495574403056286528, 118.0850938064217246, -0.7939362711117921023 ) ) ;
#27576=CARTESIAN_POINT ( 'NONE',  ( -5.006118277528749161, 117.4009255802263283, 0.7893014723888780448 ) ) ;
#27577=CARTESIAN_POINT ( 'NONE',  ( 18.07470265256048236, 147.5382818419693649, 2.342107984669389964 ) ) ;
#27579=CARTESIAN_POINT ( 'NONE',  ( 22.66443576792679693, 150.6395781703034231, 0.4273611094724397153 ) ) ;
#27580=CARTESIAN_POINT ( 'NONE',  ( -3.946719713907086202, 4.502433826932805694, 7.497755479828382086 ) ) ;
#27581=CARTESIAN_POINT ( 'NONE',  ( 14.42924251737974473, 139.0941462050048187, 0.8894241721302194037 ) ) ;
#27584=CARTESIAN_POINT ( 'NONE',  ( 4.522962677521610964, 110.7917694958216401, -2.894362350303244291 ) ) ;
#27585=CARTESIAN_POINT ( 'NONE',  ( 4.336254965884680068, 118.7629491485453741, 1.056156474602399697 ) ) ;
#27587=CARTESIAN_POINT ( 'NONE',  ( -17.22554230343062542, 122.7389118244895769, -0.2345756144184561187 ) ) ;
#27588=VERTEX_POINT ( 'NONE', #36906 ) ;
#27590=CARTESIAN_POINT ( 'NONE',  ( 6.883184783311018684, 121.6011013064247379, -0.4353592733600721854 ) ) ;
#27591=CARTESIAN_POINT ( 'NONE',  ( -8.330184522151240500, 120.0920323058250858, 1.118340454250549731 ) ) ;
#27593=CARTESIAN_POINT ( 'NONE',  ( 0.2141205576264084698, 115.7030700283022782, -1.756908841275494293 ) ) ;
#27594=CARTESIAN_POINT ( 'NONE',  ( -14.27613791431603119, 138.9852717218771261, -0.6171993629658318881 ) ) ;
#27595=CARTESIAN_POINT ( 'NONE',  ( 4.648743876849892764, -12.57259931633604388, 2.147031799546866182 ) ) ;
#27596=CARTESIAN_POINT ( 'NONE',  ( -9.838452836889556963, 157.5983698538113629, 1.280564089889915769 ) ) ;
#27598=CARTESIAN_POINT ( 'NONE',  ( 15.65298122355231492, 120.8241032224722176, 0.4173319239378796008 ) ) ;
#27599=CARTESIAN_POINT ( 'NONE',  ( 10.13917656308076864, 125.9557277354818012, 0.2514634351610266494 ) ) ;
#27600=ORIENTED_EDGE ( 'NONE', *, *, #31869, .T. ) ;
#27601=CARTESIAN_POINT ( 'NONE',  ( 0.9679928046509989059, 27.93285725408814812, -0.1178628334679577422 ) ) ;
#27602=EDGE_CURVE ( 'NONE', #6891, #26236, #16084, .T. ) ;
#27603=CARTESIAN_POINT ( 'NONE',  ( -8.216553068272286708, 117.5004391570743394, -0.1790601237764437026 ) ) ;
#27608=CARTESIAN_POINT ( 'NONE',  ( -8.455225958726231283, 119.4764566065096005, 1.058818690914600458 ) ) ;
#27609=CARTESIAN_POINT ( 'NONE',  ( -3.074427775304182209, -11.96646105551300465, -3.469969274305642060 ) ) ;
#27610=CARTESIAN_POINT ( 'NONE',  ( 18.58655447097567404, 128.6297099747515347, 1.738804191113343833 ) ) ;
#27612=CARTESIAN_POINT ( 'NONE',  ( 1.201082828432564087, 118.2527139659984101, -0.6198154079389066595 ) ) ;
#27613=CARTESIAN_POINT ( 'NONE',  ( 7.984751813625430295, 22.47881364768745271, 2.830840501157275924 ) ) ;
#27614=CARTESIAN_POINT ( 'NONE',  ( -21.78097984573151535, 150.5404744109896171, -1.730106343981699268 ) ) ;
#27615=CARTESIAN_POINT ( 'NONE',  ( 4.852265073632695547, 117.6441343497408667, -0.9100757317102342592 ) ) ;
#27617=CARTESIAN_POINT ( 'NONE',  ( -0.001786757842276731579, 120.9379535345006076, 0.08941666878750659242 ) ) ;
#27618=CARTESIAN_POINT ( 'NONE',  ( 4.283822907657564016, -15.48171044555848930, 4.591852530049981063 ) ) ;
#27620=CARTESIAN_POINT ( 'NONE',  ( -0.5436877124052815757, 117.9496053982743149, -1.405509504246643004 ) ) ;
#27622=ORIENTED_EDGE ( 'NONE', *, *, #16629, .F. ) ;
#27623=CARTESIAN_POINT ( 'NONE',  ( 17.96932707993145328, 150.0321773811041339, 2.460285709456810466 ) ) ;
#27624=DIRECTION ( 'NONE',  ( -5.206863593109713661E-17, 1.000000000000000000, -1.077750396879097183E-30 ) ) ;
#27625=CARTESIAN_POINT ( 'NONE',  ( 4.752069321396074741, 117.6028811792687350, 1.174454948735748294 ) ) ;
#27626=CARTESIAN_POINT ( 'NONE',  ( -1.272828668259226248, 111.9985432423065959, 2.911558293332169534 ) ) ;
#27627=CARTESIAN_POINT ( 'NONE',  ( 8.241158353334730791, 13.74789577914289929, -1.876134369653635448 ) ) ;
#27629=CARTESIAN_POINT ( 'NONE',  ( 0.7026863962999440050, 156.4221767039705071, 0.7130674712139345450 ) ) ;
#27630=CARTESIAN_POINT ( 'NONE',  ( -5.240514789080909175, 115.6909491485453003, -1.019557571888159098 ) ) ;
#27631=CARTESIAN_POINT ( 'NONE',  ( 5.638719538426313349, 159.1014311945586712, -0.3820744581509933346 ) ) ;
#27636=CARTESIAN_POINT ( 'NONE',  ( -4.252766745286226779, 118.2250244251308828, 0.3074143273816778987 ) ) ;
#27637=CARTESIAN_POINT ( 'NONE',  ( 2.352955416729489713, 107.1115117626462450, -4.697798642113138357 ) ) ;
#27638=ORIENTED_EDGE ( 'NONE', *, *, #26154, .F. ) ;
#27640=CARTESIAN_POINT ( 'NONE',  ( 6.241659769608493669, 119.7361415367193587, -0.9904423240702238118 ) ) ;
#27641=CARTESIAN_POINT ( 'NONE',  ( -5.402623002109140593, 117.1681999988027911, -0.9004238350613810171 ) ) ;
#27642=CARTESIAN_POINT ( 'NONE',  ( 4.274869760779545835, 118.2142274725316753, 0.5231722506238379866 ) ) ;
#27643=CARTESIAN_POINT ( 'NONE',  ( -1.656170893582116443, 156.3096136994911092, -0.5768031348127031777 ) ) ;
#27647=EDGE_CURVE ( 'NONE', #27588, #17493, #10966, .T. ) ;
#27649=CARTESIAN_POINT ( 'NONE',  ( 1.580769961479467911, 28.79261460129497863, -4.363931058323818668 ) ) ;
#27650=CARTESIAN_POINT ( 'NONE',  ( -0.5640265924887369886, 120.2131932824006526, -0.4111470527632632987 ) ) ;
#27655=CARTESIAN_POINT ( 'NONE',  ( 6.997804181779785360, 121.9551933346753714, 0.1784859520612882000 ) ) ;
#27656=DIRECTION ( 'NONE',  ( 0.9998004120163608288, 0.000000000000000000, 0.01997839162482760791 ) ) ;
#27657=CARTESIAN_POINT ( 'NONE',  ( 21.41027608214055888, 151.3201912522522719, 1.490379992046950264 ) ) ;
#27659=CARTESIAN_POINT ( 'NONE',  ( 3.130567944924658175, -14.75736435017342707, 3.480214150758962788 ) ) ;
#27660=CARTESIAN_POINT ( 'NONE',  ( 7.920278096381447419, 118.7344292658239340, -0.9023208588851655554 ) ) ;
#27661=CARTESIAN_POINT ( 'NONE',  ( -18.67487979129062481, 147.7499600834086948, 1.698815563122507921 ) ) ;
#27662=CARTESIAN_POINT ( 'NONE',  ( -3.990024091077861268, 18.91925256873344807, 2.329872802929966902 ) ) ;
#27663=CARTESIAN_POINT ( 'NONE',  ( -5.825324126169852512, 117.1711376449269721, -0.5405197603966793718 ) ) ;
#27664=CARTESIAN_POINT ( 'NONE',  ( -0.4796499176084361160, 15.67505972103439049, -0.8497018901732851237 ) ) ;
#27668=CARTESIAN_POINT ( 'NONE',  ( -9.597885446028771028, 124.1734284925964573, 0.3307417288639282194 ) ) ;
#27669=CARTESIAN_POINT ( 'NONE',  ( 4.828046317437772572, -12.99562652935115636, 2.825559498992329832 ) ) ;
#27670=CARTESIAN_POINT ( 'NONE',  ( 10.26617122093349543, 123.0849000269954701, -0.9769925898671677489 ) ) ;
#27673=CARTESIAN_POINT ( 'NONE',  ( 2.395182152955315225, 115.7029496081253512, 1.700632368870516276 ) ) ;
#27674=CARTESIAN_POINT ( 'NONE',  ( 3.191397606779386109, -14.26579101578730224, 3.890870127686782087 ) ) ;
#27675=CARTESIAN_POINT ( 'NONE',  ( -4.698701480185317969, 117.8441750417280076, -1.023598512841458863 ) ) ;
#27676=CARTESIAN_POINT ( 'NONE',  ( 11.90298433346883300, 130.3805625696445816, 0.1299774887382024458 ) ) ;
#27678=CARTESIAN_POINT ( 'NONE',  ( 0.4261125263669181540, 118.2558431149878402, 0.5943921922486902210 ) ) ;
#27680=AXIS2_PLACEMENT_3D ( 'NONE', #26796, #21421, #15469 ) ;
#27681=CARTESIAN_POINT ( 'NONE',  ( -15.47023807670837314, 120.6682698389898434, -0.3091321738930619678 ) ) ;
#27682=EDGE_CURVE ( 'NONE', #11667, #6467, #34417, .T. ) ;
#27683=CARTESIAN_POINT ( 'NONE',  ( 0.01133107913638299775, 156.3792106723807649, -0.5670535347366656431 ) ) ;
#27684=CIRCLE ( 'NONE', #20860, 0.5080000000000002292 ) ;
#27685=CARTESIAN_POINT ( 'NONE',  ( 20.30088961563504313, 128.9598305440861452, 0.1271185223121274743 ) ) ;
#27689=CARTESIAN_POINT ( 'NONE',  ( 2.055526052377715462, -15.16505444338715769, 5.893956344503145317 ) ) ;
#27691=CARTESIAN_POINT ( 'NONE',  ( -4.858498820925455597, 117.7576908667619620, -0.8801082217429874177 ) ) ;
#27692=CARTESIAN_POINT ( 'NONE',  ( -4.798162323025271903, 117.8843545273942794, 0.6935535454817384204 ) ) ;
#27695=CARTESIAN_POINT ( 'NONE',  ( 2.899848536121923281, 118.0059886663794231, -0.7391867022396521048 ) ) ;
#27696=CARTESIAN_POINT ( 'NONE',  ( -1.040151681621160229, 108.5039085404744981, -4.268591994808179635 ) ) ;
#27697=CARTESIAN_POINT ( 'NONE',  ( 4.931585812799779589, 117.5375468106932431, 1.014273347241211320 ) ) ;
#27699=CARTESIAN_POINT ( 'NONE',  ( -0.3790891741045420149, 120.5507043431651510, 0.5490176968301536675 ) ) ;
#27701=CARTESIAN_POINT ( 'NONE',  ( 1.719524320724281852, 5.915668354077112667, 4.300554535892874064 ) ) ;
#27702=CARTESIAN_POINT ( 'NONE',  ( 4.801216665947148243, 117.4032681888235459, -1.015537427445656782 ) ) ;
#27703=CARTESIAN_POINT ( 'NONE',  ( -0.1690072757122455804, 105.7852416022782478, -5.338485453081204035 ) ) ;
#27704=CARTESIAN_POINT ( 'NONE',  ( 1.858891552337619935, -15.10179129218686178, 5.555419934288654993 ) ) ;
#27705=CARTESIAN_POINT ( 'NONE',  ( 5.239677827970672830, 116.1170857923940787, -1.027392938984838633 ) ) ;
#27706=DIRECTION ( 'NONE',  ( -4.017660918040594346E-17, 1.000000000000000000, 2.376309959284834438E-19 ) ) ;
#27707=CARTESIAN_POINT ( 'NONE',  ( -2.051794397732527475, 115.7029490351849006, 1.635858944951805061 ) ) ;
#27708=CARTESIAN_POINT ( 'NONE',  ( -0.6244342276652131707, 19.93415720681881353, -4.586363120317934694 ) ) ;
#27709=ORIENTED_EDGE ( 'NONE', *, *, #12647, .T. ) ;
#27710=CARTESIAN_POINT ( 'NONE',  ( -4.305676042947723658, 104.6144662015411626, -3.167619746371888034 ) ) ;
#27711=CARTESIAN_POINT ( 'NONE',  ( 4.538337246427208704, -15.41107556132688394, 0.6303774773485874006 ) ) ;
#27712=CARTESIAN_POINT ( 'NONE',  ( -2.330377461923392346, 118.7486697826011977, 0.7097125967482104114 ) ) ;
#27713=CARTESIAN_POINT ( 'NONE',  ( -0.7839530942921373313, 14.33508526448824760, 0.5845576647881698396 ) ) ;
#27717=CARTESIAN_POINT ( 'NONE',  ( 4.014846287426770743, 122.0441497943765370, 0.2789485273175661972 ) ) ;
#27718=CARTESIAN_POINT ( 'NONE',  ( -0.5902664527120891069, 120.3589971203204669, 0.3461335206401335851 ) ) ;
#27720=CARTESIAN_POINT ( 'NONE',  ( 4.638991104174423619, 118.0227226582861420, -0.6551358822890929190 ) ) ;
#27721=CARTESIAN_POINT ( 'NONE',  ( 0.01051219832175660264, 119.4384375980492194, -0.5260733902271049756 ) ) ;
#27722=CARTESIAN_POINT ( 'NONE',  ( -19.76635024033938137, 141.2215177107240436, -2.477633452034130990 ) ) ;
#27724=CARTESIAN_POINT ( 'NONE',  ( 4.282392886588548997, 118.2128385315536860, -0.3623839240741059675 ) ) ;
#27725=CARTESIAN_POINT ( 'NONE',  ( 15.52187087609520688, 147.8629129908177049, -0.2796426011346633822 ) ) ;
#27728=CARTESIAN_POINT ( 'NONE',  ( 2.769760999665409340, -14.92388480464812872, 4.423285184949336646 ) ) ;
#27729=CARTESIAN_POINT ( 'NONE',  ( -4.922306677375791750, 117.4109580117980016, 0.9480543157666212473 ) ) ;
#27732=CARTESIAN_POINT ( 'NONE',  ( -2.329872802932658082, -2.670747431267189498, -3.990024091085845548 ) ) ;
#27733=CARTESIAN_POINT ( 'NONE',  ( 10.24488040547488943, 123.7737839053064022, 1.229789271442949694 ) ) ;
#27734=CARTESIAN_POINT ( 'NONE',  ( -3.732951360862769352, 28.31137488888144915, 1.178986259223461230 ) ) ;
#27735=CARTESIAN_POINT ( 'NONE',  ( -3.706399805698186167, 113.7286232773062125, 2.153009399082070452 ) ) ;
#27736=EDGE_CURVE ( 'NONE', #13530, #39307, #27954, .T. ) ;
#27737=CARTESIAN_POINT ( 'NONE',  ( -2.424025297795170619, -5.104216246930970868, 3.935102955759355758 ) ) ;
#27738=CARTESIAN_POINT ( 'NONE',  ( 15.52804360843196463, 147.5314071815517138, 0.4383331365498630561 ) ) ;
#27740=CARTESIAN_POINT ( 'NONE',  ( 1.329249052905784323, 1.652534479431654546, 8.327223686629459110 ) ) ;
#27742=CARTESIAN_POINT ( 'NONE',  ( -8.759430686813598044, 117.8325680729238343, -0.5873362267662896041 ) ) ;
#27745=CARTESIAN_POINT ( 'NONE',  ( 2.047221892555402434, -15.65848914036231676, 5.808978358897259220 ) ) ;
#27747=CARTESIAN_POINT ( 'NONE',  ( 7.690436415270363923, 8.290658626076512050, -3.468142284020285793 ) ) ;
#27748=FACE_OUTER_BOUND ( 'NONE', #9176, .T. ) ;
#27751=CARTESIAN_POINT ( 'NONE',  ( 0.1065646865914870178, 105.8844662015456919, -5.332932678536313809 ) ) ;
#27752=CARTESIAN_POINT ( 'NONE',  ( -6.918545264603769063, 117.3320596397172721, 0.2494728033470791639 ) ) ;
#27757=CARTESIAN_POINT ( 'NONE',  ( -15.26262975079004569, 148.0175730704188481, -0.3049836654608575892 ) ) ;
#27758=CARTESIAN_POINT ( 'NONE',  ( 5.218378134725943696, -15.03467804911627681, 3.623131781705042354 ) ) ;
#27759=CARTESIAN_POINT ( 'NONE',  ( -1.179722549733782877, 118.0995038195805904, 0.6028833020595597558 ) ) ;
#27761=CARTESIAN_POINT ( 'NONE',  ( 14.41840636618835880, 121.0470547900126519, -0.7241072410554124650 ) ) ;
#27762=CARTESIAN_POINT ( 'NONE',  ( -4.563195415240126174, 21.88328375387019165, -0.7336086519975816289 ) ) ;
#27763=CARTESIAN_POINT ( 'NONE',  ( -13.50792085693146838, 119.6474162840860771, -0.5731308571144441144 ) ) ;
#27766=CARTESIAN_POINT ( 'NONE',  ( 2.183922297081623665, 116.1979336525763671, 0.06695608452006818201 ) ) ;
#27768=CARTESIAN_POINT ( 'NONE',  ( -17.81417655509816456, 146.7645792007554633, 1.532459167469646610 ) ) ;
#27769=CARTESIAN_POINT ( 'NONE',  ( -5.078986093043185157, 69.43546620154572224, -0.1014902294541231847 ) ) ;
#27770=CARTESIAN_POINT ( 'NONE',  ( 0.01147819631899514234, 118.8623374019222894, -0.5744158801423951966 ) ) ;
#27771=CARTESIAN_POINT ( 'NONE',  ( 0.01023305610364720099, 117.8848902025789158, -0.5121039721716186266 ) ) ;
#27773=CARTESIAN_POINT ( 'NONE',  ( 3.602148172789689795, 120.6468399921648711, -0.3585086490597836906 ) ) ;
#27775=CARTESIAN_POINT ( 'NONE',  ( -14.16178827078164026, 152.6618899727951089, -2.241469232429742942 ) ) ;
#27776=CARTESIAN_POINT ( 'NONE',  ( 3.297442402085044133, -15.64565814434701352, 4.209479195861737466 ) ) ;
#27777=CARTESIAN_POINT ( 'NONE',  ( -4.390462178403575777, 118.1641434913643138, -0.6590699376955369004 ) ) ;
#27779=DIRECTION ( 'NONE',  ( -0.9998004120163608288, 0.000000000000000000, -0.01997839162482747608 ) ) ;
#27780=CARTESIAN_POINT ( 'NONE',  ( 11.17842967653866459, 122.9575399027323073, 1.639653439019827408 ) ) ;
#27781=DIRECTION ( 'NONE',  ( 4.017660918040594346E-17, -1.000000000000000000, -2.376309959284834438E-19 ) ) ;
#27783=( BOUNDED_SURFACE ( )  B_SPLINE_SURFACE ( 3, 2, ( 
 ( #30207, #14999, #33210 ),
 ( #835, #11392, #36613 ),
 ( #1047, #7432, #18190 ),
 ( #11814, #29791, #24378 ),
 ( #26808, #39816, #37385 ),
 ( #33415, #21172, #34203 ),
 ( #37590, #5029, #17986 ),
 ( #1825, #11600, #24584 ),
 ( #8417, #21376, #34402 ),
 ( #5236, #31409, #18401 ),
 ( #2671, #34828, #5661 ),
 ( #5866, #31624, #32258 ),
 ( #35045, #15212, #12863 ),
 ( #35454, #15630, #25647 ),
 ( #18618, #41221, #9051 ),
 ( #2462, #8838, #3087 ),
 ( #2250, #28633, #25447 ),
 ( #6073, #22220, #21800 ),
 ( #41646, #29049, #12239 ),
 ( #19035, #15425, #16046 ) ),
 .UNSPECIFIED., .F., .F., .F. ) 
 B_SPLINE_SURFACE_WITH_KNOTS ( ( 4, 2, 2, 2, 2, 2, 2, 2, 2, 4 ),
 ( 3, 3 ),
 ( -2.835792020584096599E-05, 0.001133685587513493529, 0.001714707341373160852, 0.002295729095232827959, 0.003457772602952162606, 0.003748283479881996377, 0.004038794356811830147, 0.004184049795276746815, 0.004329305233741663483, 0.004619816110671496820 ),
 ( 0.000000000000000000, 0.7006144518607101412 ),
 .UNSPECIFIED. ) 
 GEOMETRIC_REPRESENTATION_ITEM ( )  RATIONAL_B_SPLINE_SURFACE ( (
 ( 1.000000000000000000, 0.8321369569203693750, 0.8994884616705510760),
 ( 1.000000000000000000, 0.8321369569203693750, 0.8994884616705510760),
 ( 1.000000000000000000, 0.8321370030818711072, 0.8994884893107240043),
 ( 1.000000000000000000, 0.8321369330536090292, 0.8994884473798248070),
 ( 1.000000000000000000, 0.8321364034739958671, 0.8994881302828594549),
 ( 1.000000000000000000, 0.8321364926397946116, 0.8994881836727623980),
 ( 1.000000000000000000, 0.8321369244513672214, 0.8994884422290512216),
 ( 1.000000000000000000, 0.8321370276008952516, 0.8994885039920070824),
 ( 1.000000000000000000, 0.8321369665538331795, 0.8994884674387908507),
 ( 1.000000000000000000, 0.8321369547486586749, 0.8994884603701935877),
 ( 1.000000000000000000, 0.8321369676810204119, 0.8994884681137178539),
 ( 1.000000000000000000, 0.8321369492625183550, 0.8994884570852512695),
 ( 1.000000000000000000, 0.8321371141846684027, 0.8994885558358678423),
 ( 1.000000000000000000, 0.8321369149363557760, 0.8994884365317372676),
 ( 1.000000000000000000, 0.8321367296521178236, 0.8994883255888910245),
 ( 1.000000000000000000, 0.8321365983280889500, 0.8994882469558581617),
 ( 1.000000000000000000, 0.8321368728221703037, 0.8994884113149801408),
 ( 1.000000000000000000, 0.8321370919515077569, 0.8994885425232939102),
 ( 1.000000000000000000, 0.8321369569197746285, 0.8994884616701950275),
 ( 1.000000000000000000, 0.8321369569197746285, 0.8994884616701950275) ) ) 
 REPRESENTATION_ITEM ( '' )  SURFACE ( )  );
#27785=CARTESIAN_POINT ( 'NONE',  ( -6.690270197923770645, -5.753818539685515709, 5.116497609988504891 ) ) ;
#27786=CARTESIAN_POINT ( 'NONE',  ( 10.53234188159470897, 153.0603347025997323, 0.7465333597200856097 ) ) ;
#27791=CARTESIAN_POINT ( 'NONE',  ( 0.6578851187915285559, 105.8204382098766700, -5.299257009308196764 ) ) ;
#27796=CARTESIAN_POINT ( 'NONE',  ( -18.61428830734555362, 154.1511370093759865, -0.1565858633853991211 ) ) ;
#27799=CARTESIAN_POINT ( 'NONE',  ( -6.890691652417186397, 121.7969240507482169, -0.5388405038592991581 ) ) ;
#27800=CARTESIAN_POINT ( 'NONE',  ( -7.862390625643993936, 122.3040693727414663, 0.4082539156324949126 ) ) ;
#27802=CARTESIAN_POINT ( 'NONE',  ( 2.015163235281668630, 118.7629491485439956, -1.152909370120437149 ) ) ;
#27803=CARTESIAN_POINT ( 'NONE',  ( -2.801574634701766708, 120.9854572005495044, -0.1568784928360136832 ) ) ;
#27804=CARTESIAN_POINT ( 'NONE',  ( 5.545296128261989033, -13.31524510490228508, 2.629257322947794684 ) ) ;
#27805=CARTESIAN_POINT ( 'NONE',  ( -21.51971352461183074, 150.2128557559047692, 1.148904605754655694 ) ) ;
#27806=CARTESIAN_POINT ( 'NONE',  ( 0.02983097946976470335, 117.3993836135854707, -1.492864285907033572 ) ) ;
#27807=CARTESIAN_POINT ( 'NONE',  ( 5.738526254234393775, 159.1207877133979309, 0.2162537097210232850 ) ) ;
#27808=CARTESIAN_POINT ( 'NONE',  ( 2.877599497300482145, 156.0997331449266028, 0.1009948612926021977 ) ) ;
#27810=CARTESIAN_POINT ( 'NONE',  ( 0.9303216910925710126, 27.28174836166085981, 0.2932329443217298603 ) ) ;
#27811=CARTESIAN_POINT ( 'NONE',  ( -9.803363283900923264, 117.9968303279965340, -0.2884128246907767257 ) ) ;
#27813=ORIENTED_EDGE ( 'NONE', *, *, #27222, .T. ) ;
#27816=CARTESIAN_POINT ( 'NONE',  ( 8.405933479366224148, 119.4776037158581801, 1.396206739680378339 ) ) ;
#27817=FACE_OUTER_BOUND ( 'NONE', #40461, .T. ) ;
#27818=CARTESIAN_POINT ( 'NONE',  ( 19.25714749039842388, 152.1947311750261065, 2.059892502987373142 ) ) ;
#27820=CARTESIAN_POINT ( 'NONE',  ( 14.40310572532104594, 154.4775811199918110, -1.681202589455180085 ) ) ;
#27821=CARTESIAN_POINT ( 'NONE',  ( -8.047487967707532164, 27.33737370333709649, -2.486188741727015206 ) ) ;
#27822=CARTESIAN_POINT ( 'NONE',  ( -3.066799924081489159, 159.2904672602661549, -0.9578552656232321993 ) ) ;
#27823=CARTESIAN_POINT ( 'NONE',  ( 4.936507465849099496, 117.6536220454318311, -0.7445373667808669049 ) ) ;
#27826=CARTESIAN_POINT ( 'NONE',  ( -9.295404511957364946, 124.2653519604415067, -0.02360630055292697871 ) ) ;
#27827=CARTESIAN_POINT ( 'NONE',  ( -19.13882315974093018, 148.9694856701144090, -2.502273048283856660 ) ) ;
#27829=CARTESIAN_POINT ( 'NONE',  ( 3.223661160190148145, -15.48894043311785396, 5.519697737696615647 ) ) ;
#27832=CARTESIAN_POINT ( 'NONE',  ( -2.554027823802438313, 117.3993834736394888, -1.425007985248354148 ) ) ;
#27834=CARTESIAN_POINT ( 'NONE',  ( 13.13949684203664781, 123.8872625266795211, 1.904607404193280562 ) ) ;
#27835=CARTESIAN_POINT ( 'NONE',  ( 4.886022116125724679, 117.7561648045584519, -0.7145573245312663024 ) ) ;
#27836=CARTESIAN_POINT ( 'NONE',  ( -6.552964542248172189E-14, 78.83346620154574680, -6.511376220759049693E-18 ) ) ;
#27837=CARTESIAN_POINT ( 'NONE',  ( -2.330098105383639595, 118.9955205646042344, 0.6366692849230545237 ) ) ;
#27838=CARTESIAN_POINT ( 'NONE',  ( -8.048466033148526932, -0.5260294302935444311, 2.538140512261041426 ) ) ;
#27839=CARTESIAN_POINT ( 'NONE',  ( 16.16038979459555236, 146.4165046419237228, 1.293905914731260598 ) ) ;
#27842=CARTESIAN_POINT ( 'NONE',  ( 22.82237111512518979, 142.4248215231809240, -0.5244786342524966338 ) ) ;
#27847=CARTESIAN_POINT ( 'NONE',  ( -4.416343619678607446, 118.1792209726063874, 0.3907444955660914210 ) ) ;
#27848=CARTESIAN_POINT ( 'NONE',  ( -16.18905205736058051, 121.2598130428683447, -0.3234957879086919341 ) ) ;
#27852=CARTESIAN_POINT ( 'NONE',  ( -6.259582159009869251, 119.8770361027300027, -1.223887577771844537 ) ) ;
#27854=CARTESIAN_POINT ( 'NONE',  ( 4.160022638901372360, 118.2392538408114717, 0.3840984172949051811 ) ) ;
#27855=CARTESIAN_POINT ( 'NONE',  ( -12.50622671840202393, 130.7145975665201831, -1.030918987520083485 ) ) ;
#27858=EDGE_LOOP ( 'NONE', ( #18603, #14055 ) ) ;
#27859=CARTESIAN_POINT ( 'NONE',  ( 3.655561289726139140, 27.93047918286777076, -2.829280713513928180 ) ) ;
#27860=CARTESIAN_POINT ( 'NONE',  ( -8.727673846237186339, 154.8283212766472445, -1.585547369736019840 ) ) ;
#27864=CARTESIAN_POINT ( 'NONE',  ( -7.791833174368864690, 122.6039448250109132, -0.04536756530948493626 ) ) ;
#27865=CARTESIAN_POINT ( 'NONE',  ( 4.626035402534343532, 22.79242798913371360, 0.3558936578225105341 ) ) ;
#27866=CARTESIAN_POINT ( 'NONE',  ( 11.27775095430294350, 119.0414093155750379, 0.9684783378491815808 ) ) ;
#27868=CARTESIAN_POINT ( 'NONE',  ( 2.831922340016455042, -13.93067033233365315, 0.4309514144534042912 ) ) ;
#27869=CARTESIAN_POINT ( 'NONE',  ( 20.94193450296696923, 149.6610172957225586, -1.461262285038966047 ) ) ;
#27870=CARTESIAN_POINT ( 'NONE',  ( -12.07275429247933829, 123.1955650103826798, 1.290935347410189449 ) ) ;
#27871=CARTESIAN_POINT ( 'NONE',  ( -2.961220487682185709, 16.77021669962341477, -3.573240411402743621 ) ) ;
#27872=CARTESIAN_POINT ( 'NONE',  ( -22.68171885890644290, 150.0520759213295889, -1.302983692151378214 ) ) ;
#27873=CARTESIAN_POINT ( 'NONE',  ( 0.7602462924416659718, 13.52415170902173891, -0.6087277422976011820 ) ) ;
#27876=CARTESIAN_POINT ( 'NONE',  ( -4.503927054024219778, 120.9948550335633115, 0.2290337153283758254 ) ) ;
#27877=CARTESIAN_POINT ( 'NONE',  ( 2.291753010757021869, -15.38865404460348962, 5.937071240476925027 ) ) ;
#27878=CARTESIAN_POINT ( 'NONE',  ( 10.90507628433457832, 123.7747955097422476, -1.016219593014793920 ) ) ;
#27880=CARTESIAN_POINT ( 'NONE',  ( 0.9953799440056341208, 115.7029401158592492, 1.748199640645290209 ) ) ;
#27881=CARTESIAN_POINT ( 'NONE',  ( 3.243601939617143159, -13.81697766888033385, 2.329280267808830907 ) ) ;
#27882=CARTESIAN_POINT ( 'NONE',  ( -4.764346593062310120, 117.8854850664883998, -0.8882920174160988669 ) ) ;
#27883=ADVANCED_FACE ( 'NONE', ( #14927 ), #24308, .T. ) ;
#27884=CARTESIAN_POINT ( 'NONE',  ( 10.21313493804724715, 125.9885856776569426, 0.1666469060040939310 ) ) ;
#27885=EDGE_LOOP ( 'NONE', ( #6362, #23967, #18617, #22341 ) ) ;
#27886=CARTESIAN_POINT ( 'NONE',  ( 18.81387422072291216, 135.8679125664981484, 2.390408806419126009 ) ) ;
#27887=CARTESIAN_POINT ( 'NONE',  ( -3.174366308152013705, 104.6144662015457243, -0.06343139340882732180 ) ) ;
#27891=CARTESIAN_POINT ( 'NONE',  ( 22.47159541194093180, 150.7739627601066275, -0.0002021107738995970768 ) ) ;
#27893=CARTESIAN_POINT ( 'NONE',  ( 1.912458138725795065, -15.07098942588634749, 5.790420633640319892 ) ) ;
#27895=CARTESIAN_POINT ( 'NONE',  ( 5.332935397695204749, 51.14746620154573264, 0.1065647409268304785 ) ) ;
#27896=EDGE_CURVE ( 'NONE', #17488, #23143, #10293, .T. ) ;
#27897=CARTESIAN_POINT ( 'NONE',  ( -4.685403574366763912, 117.8875460371219788, 0.8142817779486657415 ) ) ;
#27898=VERTEX_POINT ( 'NONE', #24509 ) ;
#27899=CARTESIAN_POINT ( 'NONE',  ( -0.4158538715318880197, 118.7629491485454025, 1.264086991023878115 ) ) ;
#27900=CARTESIAN_POINT ( 'NONE',  ( 2.971243059491443184, 118.0891348236419844, -0.7498842069557943857 ) ) ;
#27901=CARTESIAN_POINT ( 'NONE',  ( -4.012272795662658709, 117.4230540797109938, -0.9751040681224720785 ) ) ;
#27903=CARTESIAN_POINT ( 'NONE',  ( 4.914877656105587356, 117.6230825708500305, 0.9484198851692730026 ) ) ;
#27905=CARTESIAN_POINT ( 'NONE',  ( -0.3981704103450558474, 123.4679809879532542, 0.1459118279324087830 ) ) ;
#27906=CARTESIAN_POINT ( 'NONE',  ( 3.064284189169764971, -3.155149710853871525, 3.465721614369133174 ) ) ;
#27908=DIRECTION ( 'NONE',  ( -0.01997839162482749342, -1.040247600000944484E-18, 0.9998004120163608288 ) ) ;
#27909=CARTESIAN_POINT ( 'NONE',  ( 2.265044067826554652, -14.95788512594138631, 5.210342366881125287 ) ) ;
#27910=CARTESIAN_POINT ( 'NONE',  ( 6.479951895127638473, 122.5560431351108974, 0.01853871597398580595 ) ) ;
#27911=CARTESIAN_POINT ( 'NONE',  ( -6.989407220697516188, 121.9513345406523399, -0.1628094617627758867 ) ) ;
#27912=FACE_OUTER_BOUND ( 'NONE', #8242, .T. ) ;
#27914=CARTESIAN_POINT ( 'NONE',  ( -1.574722418245668942, 115.7027552838863045, 1.670860613881942847 ) ) ;
#27915=CARTESIAN_POINT ( 'NONE',  ( 4.523211737919912601, 7.414965188139293062, 0.9565071382433592007 ) ) ;
#27916=EDGE_LOOP ( 'NONE', ( #39252, #10699, #40970, #41101 ) ) ;
#27917=CARTESIAN_POINT ( 'NONE',  ( 4.429703416477502209, 104.6144662015456817, -1.943618747302600092 ) ) ;
#27918=CARTESIAN_POINT ( 'NONE',  ( 2.004873297308811253, -15.47002699807756265, 5.272742632645636363 ) ) ;
#27919=CARTESIAN_POINT ( 'NONE',  ( -12.07139305262857043, 121.8643784861682065, 1.276542069712922611 ) ) ;
#27920=CARTESIAN_POINT ( 'NONE',  ( -0.9630862182390291792, 27.11985920190685917, 0.1463314843619143713 ) ) ;
#27921=CARTESIAN_POINT ( 'NONE',  ( 0.8728101606606677443, 18.85996454746999618, -0.4358653558870161926 ) ) ;
#27926=CARTESIAN_POINT ( 'NONE',  ( 2.170296427606156708, 116.5145642697238344, 1.453337335755149784 ) ) ;
#27927=CARTESIAN_POINT ( 'NONE',  ( -7.932268303791008890, 121.8456834504061845, 0.6952039612942496616 ) ) ;
#27929=CARTESIAN_POINT ( 'NONE',  ( 3.391857759029038633, -13.93828481737184610, 3.530066096054821134 ) ) ;
#27930=CARTESIAN_POINT ( 'NONE',  ( 5.874384117068456312, 120.0568572605186546, -0.8667843538975028572 ) ) ;
#27931=CARTESIAN_POINT ( 'NONE',  ( -6.532233579562855219, 157.6773268839678508, -1.915660460402585530 ) ) ;
#27932=CARTESIAN_POINT ( 'NONE',  ( 4.741393556337476944, 117.7888895289213878, -0.8991427661700817087 ) ) ;
#27933=VECTOR ( 'NONE', #12051, 1000.000000000000227 ) ;
#27934=ADVANCED_FACE ( 'NONE', ( #30918 ), #39563, .F. ) ;
#27935=CARTESIAN_POINT ( 'NONE',  ( 4.122343337852331757, 118.2429491485453497, -0.1816822259850767451 ) ) ;
#27936=CARTESIAN_POINT ( 'NONE',  ( 5.257554009420233321, 121.2670714900434206, -0.1164621724739933611 ) ) ;
#27937=ORIENTED_EDGE ( 'NONE', *, *, #37873, .F. ) ;
#27938=CARTESIAN_POINT ( 'NONE',  ( 2.856221160286674277, -14.96258862872340600, 4.237710179968991575 ) ) ;
#27940=CARTESIAN_POINT ( 'NONE',  ( -3.932819197772147390, 27.98301002373794333, 0.4898618918306563708 ) ) ;
#27942=CARTESIAN_POINT ( 'NONE',  ( 1.818839793882075728, -13.69063247836898611, -4.255424433905749204 ) ) ;
#27943=CARTESIAN_POINT ( 'NONE',  ( 16.79675997928894304, 147.6865045845431723, 1.918872074639297098 ) ) ;
#27944=CARTESIAN_POINT ( 'NONE',  ( -2.630585380139099705, 29.80773254623414914, 2.003937124266777836 ) ) ;
#27945=CARTESIAN_POINT ( 'NONE',  ( -3.905206024139432408, 115.3331674797404247, 1.578293011005953650 ) ) ;
#27946=CARTESIAN_POINT ( 'NONE',  ( 3.064284189169764971, -3.155149710853871525, 3.465721614369133174 ) ) ;
#27947=CARTESIAN_POINT ( 'NONE',  ( -1.114473875789821378, 36.31367722304657519, -0.2353634988756885538 ) ) ;
#27948=CARTESIAN_POINT ( 'NONE',  ( -4.887076909682236625, -2.444604220856811505, -6.895871986673536291 ) ) ;
#27950=CARTESIAN_POINT ( 'NONE',  ( 5.545678171451279503, 116.8412816117532742, -0.2872682508620105768 ) ) ;
#27953=CARTESIAN_POINT ( 'NONE',  ( -6.346781410994640993, 30.04503731349425166, 1.591420273447384348 ) ) ;
#27954=CIRCLE ( 'NONE', #36158, 3.175000000000001155 ) ;
#27955=CARTESIAN_POINT ( 'NONE',  ( 0.2927481059715184020, -9.205330264445118260, -8.420370646799414160 ) ) ;
#27956=CARTESIAN_POINT ( 'NONE',  ( 0.3872878167242116976, 117.3993820581147389, 1.495215202982832947 ) ) ;
#27958=DIRECTION ( 'NONE',  ( 4.017660918040594346E-17, -1.000000000000000000, -2.376309959284834438E-19 ) ) ;
#27959=CARTESIAN_POINT ( 'NONE',  ( 0.7718547489770499759, 119.9044272045951374, -0.6164056859965564295 ) ) ;
#27960=CARTESIAN_POINT ( 'NONE',  ( -0.006534887713674904404, 159.5822087645323393, 0.3270325034788581497 ) ) ;
#27965=VERTEX_POINT ( 'NONE', #12584 ) ;
#27967=CARTESIAN_POINT ( 'NONE',  ( -14.67500508075667298, 148.8517222230099719, -0.2932415260845991356 ) ) ;
#27968=CARTESIAN_POINT ( 'NONE',  ( 5.598737995799250911, -15.07077801197512201, 2.339151774602123979 ) ) ;
#27969=CARTESIAN_POINT ( 'NONE',  ( -19.85075266274223083, 150.7280352275851101, 1.521773064777484308 ) ) ;
#27970=CARTESIAN_POINT ( 'NONE',  ( 21.20416308100189440, 151.2337125027825095, -0.8636963275675616503 ) ) ;
#27971=CARTESIAN_POINT ( 'NONE',  ( -2.614655561276646889, 23.60746518810343986, 3.812863311767609620 ) ) ;
#27972=CARTESIAN_POINT ( 'NONE',  ( -7.991309159113160199, 158.6817341734954425, -0.4848270063548277276 ) ) ;
#27974=VERTEX_POINT ( 'NONE', #41574 ) ;
#27975=CARTESIAN_POINT ( 'NONE',  ( 2.185361284265998183, 116.2036773648440402, 0.07441525802958044722 ) ) ;
#27977=CARTESIAN_POINT ( 'NONE',  ( -9.055011062052066961, 121.9018297702777858, 0.9711463333382076568 ) ) ;
#27980=CARTESIAN_POINT ( 'NONE',  ( 0.4903093677401612061, 118.8635629087341954, -0.5952627799645435758 ) ) ;
#27981=CARTESIAN_POINT ( 'NONE',  ( -20.82206258336681159, 149.3152741295656369, -2.348048710389011529 ) ) ;
#27984=CARTESIAN_POINT ( 'NONE',  ( 9.105332701317813360, 123.1184971541203055, -0.5608273726695747197 ) ) ;
#27985=ORIENTED_EDGE ( 'NONE', *, *, #26631, .T. ) ;
#27986=CARTESIAN_POINT ( 'NONE',  ( -15.87222905729445266, 135.0473088626721392, -2.190551936964585167 ) ) ;
#27987=CARTESIAN_POINT ( 'NONE',  ( 2.909835405328949687, -15.65209430229147536, 4.668939894544173796 ) ) ;
#27988=CARTESIAN_POINT ( 'NONE',  ( -4.502791693421113628, 118.1162640722260164, -0.7113048364058234263 ) ) ;
#27991=CARTESIAN_POINT ( 'NONE',  ( -4.995814232853128090, 117.4677515080094707, 0.7870683612790911887 ) ) ;
#27992=CARTESIAN_POINT ( 'NONE',  ( 10.71652553037521827, 154.3566586077636487, 1.965850361453045814 ) ) ;
#27994=CARTESIAN_POINT ( 'NONE',  ( -6.252972126910993467, 3.963778981710710969, 5.644239715445565686 ) ) ;
#27995=CARTESIAN_POINT ( 'NONE',  ( 2.970866406646140767, 156.0959049650892041, 0.4589190987796911703 ) ) ;
#27999=CARTESIAN_POINT ( 'NONE',  ( 4.027359296022574142, 109.3894120745859055, -3.506257160670660067 ) ) ;
#28000=CARTESIAN_POINT ( 'NONE',  ( -7.799329138056211974, 122.5403491326864298, -0.4385002940562175433 ) ) ;
#28003=CARTESIAN_POINT ( 'NONE',  ( -15.85175717768499659, 121.0146182718019645, -0.1572851932169302969 ) ) ;
#28004=ORIENTED_EDGE ( 'NONE', *, *, #30849, .T. ) ;
#28006=CARTESIAN_POINT ( 'NONE',  ( 5.812554992953963051, 121.1879478854047392, -0.2779057282218665992 ) ) ;
#28007=CARTESIAN_POINT ( 'NONE',  ( -8.022816897867325991, 121.5631586913658140, 0.8332660241015908964 ) ) ;
#28009=CARTESIAN_POINT ( 'NONE',  ( 0.1384230549150444467, 115.7030668735399246, -1.759162436720742795 ) ) ;
#28010=CARTESIAN_POINT ( 'NONE',  ( -6.485149764178151699, 121.7431354732680973, -0.3115821950655745520 ) ) ;
#28011=CARTESIAN_POINT ( 'NONE',  ( 4.549387865739121573, -13.93190642666217194, 4.188617477609191120 ) ) ;
#28012=CARTESIAN_POINT ( 'NONE',  ( -12.49407882476853082, 156.7420262770442037, 1.161473977901223753 ) ) ;
#28014=AXIS2_PLACEMENT_3D ( 'NONE', #29691, #16262, #19459 ) ;
#28015=CARTESIAN_POINT ( 'NONE',  ( 5.792301705315622939, 116.9567987913546006, 0.2385690759321334731 ) ) ;
#28016=CARTESIAN_POINT ( 'NONE',  ( 15.26262975078991779, 148.0175730704188481, 0.3049836654608578113 ) ) ;
#28018=CARTESIAN_POINT ( 'NONE',  ( 0.3817720443006957232, 19.93710050853265869, -0.8978640518339636722 ) ) ;
#28019=CARTESIAN_POINT ( 'NONE',  ( -8.215520591712516918, 117.5015518944296247, -0.2087872862963602583 ) ) ;
#28020=CARTESIAN_POINT ( 'NONE',  ( 5.008289758173663841, 117.3984635900009295, -0.7758770640922041384 ) ) ;
#28023=CARTESIAN_POINT ( 'NONE',  ( -5.802623703142025136, 118.2257019569944987, 0.8941158778616000724 ) ) ;
#28024=CARTESIAN_POINT ( 'NONE',  ( -5.334232279151433609, 105.1224713109533155, 0.08197798277522774790 ) ) ;
#28025=CARTESIAN_POINT ( 'NONE',  ( 1.070729637574014737, 117.4935207075373569, 0.5386181289574429876 ) ) ;
#28027=CARTESIAN_POINT ( 'NONE',  ( 20.59420924110313678, 148.8605967840894095, -1.615102827552612252 ) ) ;
#28028=CARTESIAN_POINT ( 'NONE',  ( 8.421720897435127640, 23.01747231734997357, -0.09500337383513672573 ) ) ;
#28029=CARTESIAN_POINT ( 'NONE',  ( -12.77893255256123339, 120.0678233105195716, -1.216039656670922176 ) ) ;
#28030=CARTESIAN_POINT ( 'NONE',  ( 4.896450774471631462, 117.7232630146785368, -0.7635348429027170036 ) ) ;
#28031=EDGE_CURVE ( 'NONE', #36618, #41397, #32980, .T. ) ;
#28032=CARTESIAN_POINT ( 'NONE',  ( 6.689329653978076884, 121.2318545172250737, 0.3418430003135980444 ) ) ;
#28034=CARTESIAN_POINT ( 'NONE',  ( -11.11302231477190361, 128.0707465396788507, -0.1214933242792290563 ) ) ;
#28035=CARTESIAN_POINT ( 'NONE',  ( -11.88178580215919133, 154.9039014673913073, -2.222676336029907773 ) ) ;
#28037=CARTESIAN_POINT ( 'NONE',  ( 4.717164877559400615, -15.39354034361711854, 4.072675418279473547 ) ) ;
#28040=ORIENTED_EDGE ( 'NONE', *, *, #30525, .F. ) ;
#28041=CARTESIAN_POINT ( 'NONE',  ( 17.41382892593903620, 149.8167423968465073, 2.401583459992671976 ) ) ;
#28045=CARTESIAN_POINT ( 'NONE',  ( -1.803835135052293870, 120.9773948236336878, 0.3431470217397348255 ) ) ;
#28046=CARTESIAN_POINT ( 'NONE',  ( -1.690137127919513649, -8.491432666745847513, 8.270632449787910900 ) ) ;
#28047=CARTESIAN_POINT ( 'NONE',  ( 1.517991627498671114, 120.5919059741422217, 0.3392643659851173332 ) ) ;
#28049=CARTESIAN_POINT ( 'NONE',  ( 22.39781672572311422, 150.5530013069706285, -0.3987920954333211698 ) ) ;
#28054=CARTESIAN_POINT ( 'NONE',  ( -4.172699785897756364, 118.2392038860674290, 0.2169064230006704508 ) ) ;
#28055=CIRCLE ( 'NONE', #14465, 3.683000000000001162 ) ;
#28058=CARTESIAN_POINT ( 'NONE',  ( 4.053501715161472951, 119.1603328138294984, -0.7634023787871468958 ) ) ;
#28059=CARTESIAN_POINT ( 'NONE',  ( -0.1506890447697080415, 104.6144662015457527, 6.108955356427616223 ) ) ;
#28060=CARTESIAN_POINT ( 'NONE',  ( 4.418034652924236916, 118.1647599079729360, 0.6322107996853220113 ) ) ;
#28061=CARTESIAN_POINT ( 'NONE',  ( -11.72694347678957705, 128.3321206738457647, -0.9702521317530997669 ) ) ;
#28064=CARTESIAN_POINT ( 'NONE',  ( 15.56076557482319700, 120.7233670659379214, 0.3109411287488705877 ) ) ;
#28066=CARTESIAN_POINT ( 'NONE',  ( -4.191205975170537279, 21.45845178295031630, -1.961646697876042511 ) ) ;
#28071=CARTESIAN_POINT ( 'NONE',  ( -6.086536517656333523, 121.3448157377453214, 0.2330812820862587509 ) ) ;
#28072=CARTESIAN_POINT ( 'NONE',  ( -4.384008014420753163, 17.61986127277741332, -1.463615122064717111 ) ) ;
#28073=CARTESIAN_POINT ( 'NONE',  ( 6.882329627759393276, 117.5897289630162987, 0.7523600398187280103 ) ) ;
#28074=CARTESIAN_POINT ( 'NONE',  ( -3.485531464485784880, 104.6144662015454685, -3.352429072091678286 ) ) ;
#28075=CARTESIAN_POINT ( 'NONE',  ( 3.131015516031846690, -14.62848841321586946, 3.524024012273756501 ) ) ;
#28076=CARTESIAN_POINT ( 'NONE',  ( 1.132512924677445243, 117.7697124030934077, -0.5521475598058975809 ) ) ;
#28077=CARTESIAN_POINT ( 'NONE',  ( -17.21863486588935288, 149.7102054596878702, 1.666570748255499224 ) ) ;
#28078=CARTESIAN_POINT ( 'NONE',  ( -4.487480840803009130, 27.34045677879159442, -1.100063755011520872 ) ) ;
#28079=CARTESIAN_POINT ( 'NONE',  ( -14.21090189159867023, 120.4756499382577886, -1.027290292067533306 ) ) ;
#28081=CARTESIAN_POINT ( 'NONE',  ( -0.5888577047260095121, 18.69815917492401880, 0.7773729966010974879 ) ) ;
#28084=CARTESIAN_POINT ( 'NONE',  ( -0.6885929357778710624, 156.3445873232922736, 0.4144571531603685188 ) ) ;
#28085=CARTESIAN_POINT ( 'NONE',  ( 3.754230566796173285, -14.80532124960526374, 5.272564796848507207 ) ) ;
#28086=CARTESIAN_POINT ( 'NONE',  ( 9.865641862003126761, 123.3250567171901082, -0.7964883383408414286 ) ) ;
#28088=ADVANCED_FACE ( 'NONE', ( #15769 ), #38162, .F. ) ;
#28089=CARTESIAN_POINT ( 'NONE',  ( 1.187391129625792630, 115.7029482326351086, 1.742295690021671062 ) ) ;
#28090=AXIS2_PLACEMENT_3D ( 'NONE', #26968, #36981, #23327 ) ;
#28091=CARTESIAN_POINT ( 'NONE',  ( -4.731399709915055318, 117.6315807060625929, -1.144721263631117703 ) ) ;
#28092=CARTESIAN_POINT ( 'NONE',  ( 15.38626016046108447, 147.8278496344100859, 0.1795882337043284427 ) ) ;
#28093=ORIENTED_EDGE ( 'NONE', *, *, #39691, .F. ) ;
#28094=CARTESIAN_POINT ( 'NONE',  ( 13.31282764718921818, 122.3357896625302459, 1.791091420989350480 ) ) ;
#28095=CARTESIAN_POINT ( 'NONE',  ( 4.218275339060157059, 155.8585684991085714, 0.08429118021179421438 ) ) ;
#28097=CARTESIAN_POINT ( 'NONE',  ( 0.01645572339161321951, 159.4324016994384010, -0.8235116888278192215 ) ) ;
#28098=CARTESIAN_POINT ( 'NONE',  ( 1.860994725975919639, 116.5907236856068181, -0.1449800026146564336 ) ) ;
#28101=CARTESIAN_POINT ( 'NONE',  ( 1.755413149268191475, -15.27739615427885234, 5.432748241580562798 ) ) ;
#28102=CARTESIAN_POINT ( 'NONE',  ( -2.872265077263356226, 44.28946620154572855, -5.646510212151727437 ) ) ;
#28105=CARTESIAN_POINT ( 'NONE',  ( -4.725628595103277263, 117.9692962743044120, 0.6259887252853451045 ) ) ;
#28106=VERTEX_POINT ( 'NONE', #15350 ) ;
#28109=CARTESIAN_POINT ( 'NONE',  ( 5.625948711771986410, 118.2002780182136235, -0.9209370785259048953 ) ) ;
#28110=CARTESIAN_POINT ( 'NONE',  ( -4.310423192639097678, 113.1344509532474376, -2.465321907391796241 ) ) ;
#28111=CARTESIAN_POINT ( 'NONE',  ( 4.894219456065178164, 117.5445796760222521, 1.081411616995204161 ) ) ;
#28112=CARTESIAN_POINT ( 'NONE',  ( -4.641629919619552957, 117.8847811183079841, -1.004318260171652266 ) ) ;
#28113=CARTESIAN_POINT ( 'NONE',  ( -0.3848090724908974636, 122.5569158606515003, 0.2475921850528965407 ) ) ;
#28115=CARTESIAN_POINT ( 'NONE',  ( -4.515506726787251068, -6.291224493951820484, 1.111903093310195212 ) ) ;
#28118=CARTESIAN_POINT ( 'NONE',  ( 3.463597221183738917, -14.01103841792809845, 4.185469790819682068 ) ) ;
#28119=CARTESIAN_POINT ( 'NONE',  ( 4.642736441617618226, 114.7252160460498516, -1.690332539979629400 ) ) ;
#28120=CARTESIAN_POINT ( 'NONE',  ( -11.08617792162982063, 123.6647009725989648, -1.535475951868171984 ) ) ;
#28121=CARTESIAN_POINT ( 'NONE',  ( 5.125711319336574867, 116.9834589889111385, -0.2401983985477860184 ) ) ;
#28122=CARTESIAN_POINT ( 'NONE',  ( -6.024379985667599691, 30.10344933946137402, 2.517894167085569457 ) ) ;
#28123=CARTESIAN_POINT ( 'NONE',  ( -1.330810070361397646, 115.7029491485453576, 1.688173640172494272 ) ) ;
#28124=CARTESIAN_POINT ( 'NONE',  ( -4.636761822055341042, 12.60011390031314349, 0.2095705037016724059 ) ) ;
#28125=CARTESIAN_POINT ( 'NONE',  ( 20.06391502460626697, 128.8637844977697569, 0.9116527748870054682 ) ) ;
#28126=ORIENTED_EDGE ( 'NONE', *, *, #22168, .T. ) ;
#28127=CARTESIAN_POINT ( 'NONE',  ( 2.874780220322234126, 104.6144662015304476, -4.506434701495114048 ) ) ;
#28128=CARTESIAN_POINT ( 'NONE',  ( 4.348370292662268710, -15.56902811939260545, 2.317716755344581880 ) ) ;
#28129=CARTESIAN_POINT ( 'NONE',  ( -12.27894764211880485, 122.3148578561100948, 1.306772475271723799 ) ) ;
#28130=CARTESIAN_POINT ( 'NONE',  ( 0.7509867122348852231, -11.68634165275979342, 0.6197512838553165260 ) ) ;
#28131=CARTESIAN_POINT ( 'NONE',  ( 0.1081409728947390902, 20.38375149489202443, -0.9727671068919315767 ) ) ;
#28132=EDGE_CURVE ( 'NONE', #8806, #39680, #38496, .T. ) ;
#28135=VERTEX_POINT ( 'NONE', #15973 ) ;
#28137=CARTESIAN_POINT ( 'NONE',  ( 0.8148005656457013579, 107.7619142660649203, 4.566897024910153924 ) ) ;
#28138=CARTESIAN_POINT ( 'NONE',  ( -11.28744401931967545, 153.2158294759273360, 1.114070445992416003 ) ) ;
#28139=DIRECTION ( 'NONE',  ( -0.9998004120163609398, 0.000000000000000000, -0.01997839162482749689 ) ) ;
#28140=CARTESIAN_POINT ( 'NONE',  ( 2.317735183313462066, -14.86924938851764999, 5.343245562499194357 ) ) ;
#28141=CARTESIAN_POINT ( 'NONE',  ( 3.856066505249522880, 156.9018388488748883, -1.546468145409083839 ) ) ;
#28143=CARTESIAN_POINT ( 'NONE',  ( -20.09316625820300573, 147.7236477000422497, -2.507557202006583719 ) ) ;
#28144=DIRECTION ( 'NONE',  ( 0.9998004120163609398, 0.000000000000000000, 0.01997839162482749689 ) ) ;
#28145=CARTESIAN_POINT ( 'NONE',  ( -4.998096739426165946, 117.4661840451863100, 0.7739782158464477702 ) ) ;
#28146=CARTESIAN_POINT ( 'NONE',  ( 4.119320774684384290, 118.2429491485453354, -0.1851223333593593479 ) ) ;
#28147=CARTESIAN_POINT ( 'NONE',  ( 5.910930898603123929, 121.4708175001875077, -0.1161132702817543050 ) ) ;
#28150=CARTESIAN_POINT ( 'NONE',  ( 3.151249207183300260, -14.28495848352401332, 1.742053583190615207 ) ) ;
#28152=CARTESIAN_POINT ( 'NONE',  ( 4.956296842134184644, 117.5943721824530286, 0.8964810703344230358 ) ) ;
#28155=CARTESIAN_POINT ( 'NONE',  ( -4.227217475240903077, -11.31673468295422147, -1.889206449475258509 ) ) ;
#28156=CARTESIAN_POINT ( 'NONE',  ( 8.650892266477013592, 122.3401343867201945, 1.081441824013609443 ) ) ;
#28157=CARTESIAN_POINT ( 'NONE',  ( -3.635086774663250697, 28.08801940460646307, 0.4607281247925576473 ) ) ;
#28158=CARTESIAN_POINT ( 'NONE',  ( -0.8750585742504035647, 105.9515744484354371, 5.278707647178442208 ) ) ;
#28159=AXIS2_PLACEMENT_3D ( 'NONE', #33314, #10302, #23270 ) ;
#28160=AXIS2_PLACEMENT_3D ( 'NONE', #36228, #17658, #30659 ) ;
#28161=CARTESIAN_POINT ( 'NONE',  ( 3.895047602890354010, -2.730319773039217690, 2.488009491782988469 ) ) ;
#28162=CARTESIAN_POINT ( 'NONE',  ( 1.617373050801646839, 120.9968702744464366, 0.03231896268895497609 ) ) ;
#28164=CARTESIAN_POINT ( 'NONE',  ( -1.148743315670426535, 1.199490873200159013, 8.378133985588048560 ) ) ;
#28166=CARTESIAN_POINT ( 'NONE',  ( 8.767697749502918469, 117.8781695899573094, -0.2943500221663000183 ) ) ;
#28167=CARTESIAN_POINT ( 'NONE',  ( -0.3702369378895170593, 122.2435587914033022, -0.3018087652966766066 ) ) ;
#28168=CIRCLE ( 'NONE', #6413, 0.5080000000000002292 ) ;
#28169=DIRECTION ( 'NONE',  ( 0.03102909223834449809, -0.9876883405951377704, -0.1533262446135272294 ) ) ;
#28171=CARTESIAN_POINT ( 'NONE',  ( 2.951631207686332470, -3.807527625098089175, 7.891363245966695139 ) ) ;
#28172=CARTESIAN_POINT ( 'NONE',  ( 0.9880450978810132456, 117.9394488772434357, 1.394221648772276501 ) ) ;
#28175=CARTESIAN_POINT ( 'NONE',  ( 0.3884485718551349831, 122.8649044353670803, -0.2114733659581321257 ) ) ;
#28176=CARTESIAN_POINT ( 'NONE',  ( -21.71781664064065609, 151.4054434770023363, 0.2817300504337352240 ) ) ;
#28181=CARTESIAN_POINT ( 'NONE',  ( -7.045182791479643214, 122.0730096167837075, -0.1019486566929637128 ) ) ;
#28182=CARTESIAN_POINT ( 'NONE',  ( 6.174787192795118784, -14.39888150296345160, 1.159817306988995211 ) ) ;
#28183=CARTESIAN_POINT ( 'NONE',  ( -20.47035330145914145, 150.0074677946399504, 1.517022030030165114 ) ) ;
#28184=CARTESIAN_POINT ( 'NONE',  ( 21.96051921721462463, 150.3855106993079005, -0.8576051660729390180 ) ) ;
#28185=CARTESIAN_POINT ( 'NONE',  ( 4.585487687326599726, 17.13547844546973309, 0.5842699607688729424 ) ) ;
#28187=CARTESIAN_POINT ( 'NONE',  ( -5.814470848032789796, 117.0573985505404693, -0.4185731406947917899 ) ) ;
#28190=CARTESIAN_POINT ( 'NONE',  ( -8.798546888910362185, 117.6874511587486580, -0.1190107558871881799 ) ) ;
#28192=CARTESIAN_POINT ( 'NONE',  ( -17.62053193735426859, 147.9903219242534078, 1.529691019407825259 ) ) ;
#28194=CARTESIAN_POINT ( 'NONE',  ( 19.30447918735891477, 147.3692480224366079, -1.738561774106543556 ) ) ;
#28195=CARTESIAN_POINT ( 'NONE',  ( -16.25125256408151131, 125.3309463260932830, -1.843050201054562187 ) ) ;
#28198=CARTESIAN_POINT ( 'NONE',  ( 14.11809548624345645, 150.3034377993741657, -0.8008162161465683937 ) ) ;
#28199=VERTEX_POINT ( 'NONE', #34460 ) ;
#28200=CARTESIAN_POINT ( 'NONE',  ( -17.90704175211121552, 146.6345634702618952, -2.297399834898016469 ) ) ;
#28201=CARTESIAN_POINT ( 'NONE',  ( 4.493636945811098293, -15.48460478268967577, 1.406059860741644574 ) ) ;
#28202=CARTESIAN_POINT ( 'NONE',  ( -4.225035204153935631, 118.2240506214291997, -0.4891602333557787952 ) ) ;
#28204=FACE_OUTER_BOUND ( 'NONE', #34614, .T. ) ;
#28205=CARTESIAN_POINT ( 'NONE',  ( 6.563805965709463841, 120.5225452898634728, 1.124017915699712100 ) ) ;
#28208=CARTESIAN_POINT ( 'NONE',  ( -8.092465427151658730, -6.292564624861634037, 2.510960718618908238 ) ) ;
#28209=CARTESIAN_POINT ( 'NONE',  ( -0.002455802209282870532, 120.8958299794632438, 0.1228983847502211901 ) ) ;
#28214=FACE_OUTER_BOUND ( 'NONE', #4463, .T. ) ;
#28216=CARTESIAN_POINT ( 'NONE',  ( -7.849349869104243815, 122.2537424897477365, -0.7623017139119617758 ) ) ;
#28217=EDGE_CURVE ( 'NONE', #37727, #21265, #2835, .T. ) ;
#28220=CARTESIAN_POINT ( 'NONE',  ( -14.80501208800833801, 120.3086691715681695, -0.1403833142216708296 ) ) ;
#28223=CARTESIAN_POINT ( 'NONE',  ( -6.904663929053937999, 121.8518053346438847, -0.4690476237073744614 ) ) ;
#28224=CARTESIAN_POINT ( 'NONE',  ( -7.880211965457519341, 122.2234151243416989, 0.4724049390182800678 ) ) ;
#28226=CARTESIAN_POINT ( 'NONE',  ( 0.8471914301801410918, 115.7028160007855746, -1.722473985426866472 ) ) ;
#28227=CARTESIAN_POINT ( 'NONE',  ( -5.920896852643748431, 121.5237468798633955, -0.2406035128457658101 ) ) ;
#28228=CARTESIAN_POINT ( 'NONE',  ( 4.204793715662772158, -14.23101105591234550, 4.663061278791505337 ) ) ;
#28229=CARTESIAN_POINT ( 'NONE',  ( -21.87558878470086299, 148.2155681941778482, 1.275940291167070306 ) ) ;
#28231=CARTESIAN_POINT ( 'NONE',  ( -0.001838942458919137161, 116.4858755864912183, 0.09202820039585839218 ) ) ;
#28232=CARTESIAN_POINT ( 'NONE',  ( 0.6412933796112577634, 156.3034662015457741, 0.01281456791805622199 ) ) ;
#28234=CARTESIAN_POINT ( 'NONE',  ( -0.6053885369530382921, 31.17761759867932980, -0.7634260365338448873 ) ) ;
#28235=CARTESIAN_POINT ( 'NONE',  ( -18.62929286701957565, 154.1293031355326946, -0.4449488992651825514 ) ) ;
#28236=CARTESIAN_POINT ( 'NONE',  ( -6.654617103318593247E-14, 104.6144662015457243, 1.534725424433578570E-31 ) ) ;
#28238=EDGE_CURVE ( 'NONE', #276, #3703, #8996, .T. ) ;
#28241=CARTESIAN_POINT ( 'NONE',  ( -3.476201915147119959, 117.7824304111185825, 0.7268633819961063391 ) ) ;
#28242=CARTESIAN_POINT ( 'NONE',  ( -5.314278422745059238, 105.1224610256965235, 0.4583187270701644667 ) ) ;
#28243=CARTESIAN_POINT ( 'NONE',  ( 21.70872022418674163, 149.0176745010074342, 2.143008773150906876 ) ) ;
#28244=CARTESIAN_POINT ( 'NONE',  ( 13.46871114105383072, 122.4565580348552913, -1.263039180185647314 ) ) ;
#28245=CARTESIAN_POINT ( 'NONE',  ( 0.5082173563136543892, -13.24086043563247728, -4.610200172643777350 ) ) ;
#28246=CARTESIAN_POINT ( 'NONE',  ( -12.63141193514832494, 156.8164516032445306, -1.520932111850479274 ) ) ;
#28247=CARTESIAN_POINT ( 'NONE',  ( 4.909174002396540004, 117.7132343993233690, -0.7287170198434957946 ) ) ;
#28248=CARTESIAN_POINT ( 'NONE',  ( 5.310592030460657753, 116.9519127983885340, 0.9557578278138696426 ) ) ;
#28249=CARTESIAN_POINT ( 'NONE',  ( -2.914310908016815471, 156.0868537499222839, 0.09385809996612910766 ) ) ;
#28250=CARTESIAN_POINT ( 'NONE',  ( -8.504430935371939171, 120.5511696877957775, -1.462663580662433072 ) ) ;
#28251=CARTESIAN_POINT ( 'NONE',  ( 5.341109902925343711, -14.98078892696824660, 3.412803344283087181 ) ) ;
#28252=CARTESIAN_POINT ( 'NONE',  ( 4.791633145718989795, 115.6909491485453145, 1.475629664436550526 ) ) ;
#28253=ADVANCED_FACE ( 'NONE', ( #24640 ), #40954, .F. ) ;
#28256=ORIENTED_EDGE ( 'NONE', *, *, #12059, .T. ) ;
#28257=CARTESIAN_POINT ( 'NONE',  ( 18.63140056563934266, 147.4429432625130119, 2.446051816127022160 ) ) ;
#28258=CARTESIAN_POINT ( 'NONE',  ( 5.152689472752729039, 116.8412042436348912, 0.1029629964107459106 ) ) ;
#28259=CARTESIAN_POINT ( 'NONE',  ( -4.794753315118858161, 118.7629491485453599, 0.7450739223749697215 ) ) ;
#28260=CARTESIAN_POINT ( 'NONE',  ( -0.1833862045737031932, 106.0860833631645193, 5.249533627824055415 ) ) ;
#28261=CARTESIAN_POINT ( 'NONE',  ( 5.057098040335121780, -7.207523253290371024, 6.778223571298113370 ) ) ;
#28262=CARTESIAN_POINT ( 'NONE',  ( 14.94204527009761385, 148.8997249754567349, 1.137790122619589450 ) ) ;
#28265=CARTESIAN_POINT ( 'NONE',  ( 4.829765040637122198, 117.0737178285515654, -0.3500672345979854994 ) ) ;
#28271=CARTESIAN_POINT ( 'NONE',  ( -4.284176567086307230, 118.2131471502228237, 0.3606148463560187034 ) ) ;
#28272=CARTESIAN_POINT ( 'NONE',  ( 5.278445427832044068, 115.7725906505842062, -0.7833317346122758984 ) ) ;
#28276=CARTESIAN_POINT ( 'NONE',  ( -4.340105779944698483, 119.4684907284004964, -0.9269682760289738033 ) ) ;
#28277=CARTESIAN_POINT ( 'NONE',  ( 0.09004192032669379453, 116.0444662015457169, -6.160295767268807232 ) ) ;
#28278=CARTESIAN_POINT ( 'NONE',  ( -4.473455768776904762, 120.9326014760084007, -0.4576173489010090245 ) ) ;
#28279=DIRECTION ( 'NONE',  ( 4.017660918040594346E-17, -1.000000000000000000, -2.376309959284834438E-19 ) ) ;
#28282=CARTESIAN_POINT ( 'NONE',  ( -2.768688662514669385, 30.30441277318858795, -3.700580903672975541 ) ) ;
#28287=CARTESIAN_POINT ( 'NONE',  ( -6.993568332462578141, 121.9043679937891795, 0.08578656617081802105 ) ) ;
#28288=( BOUNDED_SURFACE ( )  B_SPLINE_SURFACE ( 3, 2, ( 
 ( #39750, #10338, #7571 ),
 ( #4395, #10547, #10750 ),
 ( #4597, #39532, #23516 ),
 ( #36544, #36750, #20118 ),
 ( #33562, #32930, #33141 ),
 ( #7362, #13538, #13948 ),
 ( #20320, #33347, #3760 ),
 ( #3970, #4177, #40164 ),
 ( #30340, #17141, #1188 ),
 ( #30142, #14149, #10957 ),
 ( #982, #23945, #26945 ),
 ( #39958, #23731, #12613 ),
 ( #25804, #16636, #29212 ),
 ( #55, #32842, #6856 ),
 ( #13455, #13022, #36041 ),
 ( #32418, #32212, #23013 ),
 ( #3248, #3045, #9623 ),
 ( #26442, #29644, #26015 ),
 ( #39446, #6233, #3672 ),
 ( #7075, #38810, #9832 ),
 ( #10249, #481, #29002 ),
 ( #19204, #25600, #35623 ),
 ( #22591, #28802, #16423 ),
 ( #16208, #22799, #39024 ),
 ( #19826, #3460, #20038 ),
 ( #6437, #42019, #23221 ),
 ( #16003, #36253, #26227 ),
 ( #35834, #12816, #32627 ),
 ( #19411, #6650, #19614 ),
 ( #29428, #269, #13243 ),
 ( #39231, #33057, #10040 ),
 ( #3887, #41819, #38608 ),
 ( #9414, #22380, #35406 ),
 ( #4099, #36463, #33692 ),
 ( #17058, #37092, #11093 ),
 ( #30061, #26653, #39874 ),
 ( #7910, #40506, #17681 ),
 ( #39660, #10670, #29852 ),
 ( #8109, #898, #4516 ),
 ( #30475, #14073, #10881 ),
 ( #23651, #4311, #4729 ),
 ( #36673, #13873, #14486 ) ),
 .UNSPECIFIED., .F., .F., .T. ) 
 B_SPLINE_SURFACE_WITH_KNOTS ( ( 4, 2, 2, 2, 2, 2, 2, 2, 2, 2, 2, 2, 2, 2, 2, 2, 2, 2, 2, 2, 4 ),
 ( 3, 3 ),
 ( 0.01508659279077888271, 0.01602950484020540523, 0.01697241688963192774, 0.01744387291434518900, 0.01791532893905845025, 0.01885824098848497624, 0.01980115303791150222, 0.02027260906262476348, 0.02074406508733802473, 0.02168697713676454725, 0.02262988918619106976, 0.02357280123561759227, 0.02451571328504411826, 0.02498716930975738298, 0.02545862533447064424, 0.02640153738389716676, 0.02734444943332368927, 0.02828736148275021178, 0.02875881750746347304, 0.02923027353217673430, 0.03017318558160326028 ),
 ( 0.000000000000000000, 1.000000000000000000 ),
 .UNSPECIFIED. ) 
 GEOMETRIC_REPRESENTATION_ITEM ( )  RATIONAL_B_SPLINE_SURFACE ( (
 ( 1.000000000000000000, 0.7071072175333618093, 1.000000000000000000),
 ( 1.000000000000000000, 0.7071125701626851390, 1.000000000000000000),
 ( 1.000000000000000000, 0.7070885819517980231, 1.000000000000000000),
 ( 1.000000000000000000, 0.7071155700417062206, 1.000000000000000000),
 ( 1.000000000000000000, 0.7072884777352917984, 1.000000000000000000),
 ( 1.000000000000000000, 0.7075382887060654991, 1.000000000000000000),
 ( 1.000000000000000000, 0.7076187781276516153, 1.000000000000000000),
 ( 1.000000000000000000, 0.7077331820335120982, 1.000000000000000000),
 ( 1.000000000000000000, 0.7077675007750334757, 1.000000000000000000),
 ( 1.000000000000000000, 0.7077686675487847578, 1.000000000000000000),
 ( 1.000000000000000000, 0.7076263510399570800, 1.000000000000000000),
 ( 1.000000000000000000, 0.7070463795844047494, 1.000000000000000000),
 ( 1.000000000000000000, 0.7066053812610246787, 1.000000000000000000),
 ( 1.000000000000000000, 0.7061250891750091574, 1.000000000000000000),
 ( 1.000000000000000000, 0.7059929351571929690, 1.000000000000000000),
 ( 1.000000000000000000, 0.7058117510952008899, 1.000000000000000000),
 ( 1.000000000000000000, 0.7057630826365799415, 1.000000000000000000),
 ( 1.000000000000000000, 0.7057465095916261033, 1.000000000000000000),
 ( 1.000000000000000000, 0.7059103451324751921, 1.000000000000000000),
 ( 1.000000000000000000, 0.7063930724344579248, 1.000000000000000000),
 ( 1.000000000000000000, 0.7067109810593208419, 1.000000000000000000),
 ( 1.000000000000000000, 0.7071150251610267556, 1.000000000000000000),
 ( 1.000000000000000000, 0.7071578580764347199, 1.000000000000000000),
 ( 1.000000000000000000, 0.7068314760137596187, 1.000000000000000000),
 ( 1.000000000000000000, 0.7065268676894724820, 1.000000000000000000),
 ( 1.000000000000000000, 0.7061479767406342312, 1.000000000000000000),
 ( 1.000000000000000000, 0.7060332234545864116, 1.000000000000000000),
 ( 1.000000000000000000, 0.7058611809846090379, 1.000000000000000000),
 ( 1.000000000000000000, 0.7058040174201852812, 1.000000000000000000),
 ( 1.000000000000000000, 0.7057564474746290673, 1.000000000000000000),
 ( 1.000000000000000000, 0.7058984215012326091, 1.000000000000000000),
 ( 1.000000000000000000, 0.7064705227655466713, 1.000000000000000000),
 ( 1.000000000000000000, 0.7069135182905013082, 1.000000000000000000),
 ( 1.000000000000000000, 0.7075440222900022391, 1.000000000000000000),
 ( 1.000000000000000000, 0.7077280451744416556, 1.000000000000000000),
 ( 1.000000000000000000, 0.7077773545919098241, 1.000000000000000000),
 ( 1.000000000000000000, 0.7077573002275580061, 1.000000000000000000),
 ( 1.000000000000000000, 0.7076645137286782239, 1.000000000000000000),
 ( 1.000000000000000000, 0.7075922911518204295, 1.000000000000000000),
 ( 1.000000000000000000, 0.7073505092953880080, 1.000000000000000000),
 ( 1.000000000000000000, 0.7071543910050398507, 1.000000000000000000),
 ( 1.000000000000000000, 0.7071103834195795468, 1.000000000000000000) ) ) 
 REPRESENTATION_ITEM ( '' )  SURFACE ( )  );
#28290=CARTESIAN_POINT ( 'NONE',  ( 17.76144578550747966, 125.1550653296939970, 1.296339218450673014 ) ) ;
#28291=CARTESIAN_POINT ( 'NONE',  ( 3.865556019884660799, 104.6144662015457243, -2.894260390300009256 ) ) ;
#28292=CARTESIAN_POINT ( 'NONE',  ( 3.187143392547471255, -14.52651900126690876, 3.212499789951002604 ) ) ;
#28293=CARTESIAN_POINT ( 'NONE',  ( 2.888962495634898708, 158.8946464937287999, -1.317949658345221708 ) ) ;
#28294=CARTESIAN_POINT ( 'NONE',  ( -18.13417818756210664, 144.6555253171603397, 1.679261103697791135 ) ) ;
#28295=CARTESIAN_POINT ( 'NONE',  ( 3.287934792154566299, 21.71798121574904172, 3.254339964430349230 ) ) ;
#28296=CARTESIAN_POINT ( 'NONE',  ( -15.38106892591223662, 121.3506620944898060, -1.079669858139658212 ) ) ;
#28297=CARTESIAN_POINT ( 'NONE',  ( 0.8366737682863060188, 2.078006455476229419, 0.4978880095337852585 ) ) ;
#28301=CARTESIAN_POINT ( 'NONE',  ( -15.92039698932596892, 146.6311637152522565, 0.2762755564230132133 ) ) ;
#28302=CARTESIAN_POINT ( 'NONE',  ( 5.392686582494618186, -13.55334589181164695, 3.069518437182660264 ) ) ;
#28303=CARTESIAN_POINT ( 'NONE',  ( 0.8098364334000902609, 156.6562795458349910, -1.088908734543432955 ) ) ;
#28305=CARTESIAN_POINT ( 'NONE',  ( 2.661383351097782679, 115.7033367011135709, 1.688185195617331713 ) ) ;
#28307=CARTESIAN_POINT ( 'NONE',  ( -4.772391204760736194, 117.7363031211461220, -1.071217607564205698 ) ) ;
#28308=CARTESIAN_POINT ( 'NONE',  ( 7.552512487614144732, 122.4261604937442485, 0.1509171734833088807 ) ) ;
#28310=CARTESIAN_POINT ( 'NONE',  ( 6.695514854630599366, 119.3011930948910759, 1.284729283498812658 ) ) ;
#28313=CARTESIAN_POINT ( 'NONE',  ( 4.915642170617802620, 117.4785366793690571, -0.9402594631468037534 ) ) ;
#28314=B_SPLINE_CURVE_WITH_KNOTS ( 'NONE', 3,
 ( #8670, #27625, #2509, #8245 ),
 .UNSPECIFIED., .F., .F.,
 ( 4, 4 ),
 ( 0.000000000000000000, 0.4003840206711454242 ),
 .UNSPECIFIED. ) ;
#28315=CARTESIAN_POINT ( 'NONE',  ( 13.38634958471956438, 156.9592627042916604, -0.007429229355843724146 ) ) ;
#28316=CARTESIAN_POINT ( 'NONE',  ( 0.04257260547685356306, 114.5099076536771321, -2.130507264987491212 ) ) ;
#28317=CARTESIAN_POINT ( 'NONE',  ( 4.842662086898184448, 118.7629491485453030, 0.3780004892236683567 ) ) ;
#28318=CARTESIAN_POINT ( 'NONE',  ( 1.664631964234967842, -15.26880034211669468, 5.559520488082625000 ) ) ;
#28321=AXIS2_PLACEMENT_3D ( 'NONE', #491, #5568, #11511 ) ;
#28322=CARTESIAN_POINT ( 'NONE',  ( -4.764223389954819865, 117.8480438172858840, 0.8126175582787710239 ) ) ;
#28324=ORIENTED_EDGE ( 'NONE', *, *, #8732, .F. ) ;
#28325=VERTEX_POINT ( 'NONE', #40448 ) ;
#28326=CARTESIAN_POINT ( 'NONE',  ( -1.413722513147405824, 118.7629491485454025, 1.196428764754537299 ) ) ;
#28327=CARTESIAN_POINT ( 'NONE',  ( -2.731950974749316252, 117.8398921135531481, -0.8256334691123825564 ) ) ;
#28328=CARTESIAN_POINT ( 'NONE',  ( -6.931894935422283410, 124.3275308867733600, -0.1497658092569640054 ) ) ;
#28329=CARTESIAN_POINT ( 'NONE',  ( 4.853897125124975176, 117.7484357747367198, 0.9336096688446040570 ) ) ;
#28330=CARTESIAN_POINT ( 'NONE',  ( 3.116451998213339625, -14.00698646007624149, 1.619014592372306716 ) ) ;
#28331=CARTESIAN_POINT ( 'NONE',  ( -0.8881552493051317887, 122.2453746293775652, 0.2465857446897833649 ) ) ;
#28332=CARTESIAN_POINT ( 'NONE',  ( -3.594857975007920814, -7.703025367003809798, -2.923569511714296798 ) ) ;
#28333=CARTESIAN_POINT ( 'NONE',  ( 4.921840205057578466, 117.4109437077822946, -0.9481957113721782848 ) ) ;
#28335=CARTESIAN_POINT ( 'NONE',  ( 3.666546702136318725, -13.72720857325485078, 3.759896688191319836 ) ) ;
#28336=CARTESIAN_POINT ( 'NONE',  ( 5.326805317745445301, 116.9650601603920279, -0.7421267338694929050 ) ) ;
#28337=CARTESIAN_POINT ( 'NONE',  ( -3.428210029137864101, 119.9243055703230851, -0.7605957222121785266 ) ) ;
#28338=DIRECTION ( 'NONE',  ( 0.01997839162482749689, 1.040247600000945640E-18, -0.9998004120163610509 ) ) ;
#28339=CARTESIAN_POINT ( 'NONE',  ( -4.873850642958228008, 32.38564726215445688, 3.744354677719523572 ) ) ;
#28340=CARTESIAN_POINT ( 'NONE',  ( -1.895780330261635394, 115.7029491485453434, 1.647506384871404217 ) ) ;
#28341=CARTESIAN_POINT ( 'NONE',  ( -2.359559261509405204, 14.11188314818778444, 3.974389579228013503 ) ) ;
#28342=CARTESIAN_POINT ( 'NONE',  ( 3.233108093638791924, 159.4494809562368971, 0.4325382840285663111 ) ) ;
#28343=ORIENTED_EDGE ( 'NONE', *, *, #42049, .F. ) ;
#28344=CARTESIAN_POINT ( 'NONE',  ( -1.150407940190810052, 104.6144662015545777, -5.220267424023966818 ) ) ;
#28345=CARTESIAN_POINT ( 'NONE',  ( 4.136722333222721204, -15.50381924862055705, 2.038268645697551396 ) ) ;
#28346=CARTESIAN_POINT ( 'NONE',  ( -19.58040708638642613, 147.7952244890416296, 1.737278836974155416 ) ) ;
#28347=CARTESIAN_POINT ( 'NONE',  ( 0.6786060095046909657, 20.86726683125115756, 0.6988831909418605770 ) ) ;
#28348=CARTESIAN_POINT ( 'NONE',  ( -0.9394305312890779414, 22.53537758578342931, -0.2615529312561373776 ) ) ;
#28351=CARTESIAN_POINT ( 'NONE',  ( -4.948517985667383101, 117.5250047935927995, -0.9665297271245709698 ) ) ;
#28352=CARTESIAN_POINT ( 'NONE',  ( 0.4858112859842325659, 106.1608668108878817, 5.224277761219202176 ) ) ;
#28354=CARTESIAN_POINT ( 'NONE',  ( -15.90968206782444128, 148.0001117310855250, 0.7891277450764204726 ) ) ;
#28356=CARTESIAN_POINT ( 'NONE',  ( 3.206936388013850614, -12.21552616865279006, 0.5380348851386724807 ) ) ;
#28357=CARTESIAN_POINT ( 'NONE',  ( 10.76835564757999819, 122.7614441063800399, -1.139041423164458111 ) ) ;
#28359=CARTESIAN_POINT ( 'NONE',  ( -4.966515250750420662, 118.7197616721209670, -1.086191325688556697 ) ) ;
#28361=CARTESIAN_POINT ( 'NONE',  ( 8.438889187357746735, 119.3200643466248465, 1.362719739275324526 ) ) ;
#28362=CARTESIAN_POINT ( 'NONE',  ( 4.074910602682932925, 118.2429491485453354, -0.1454311599470142491 ) ) ;
#28363=CARTESIAN_POINT ( 'NONE',  ( 1.578387894090330645, 120.8584627942791627, -0.1358179495115141855 ) ) ;
#28366=CARTESIAN_POINT ( 'NONE',  ( -0.9489272475186022460, 106.1802426532330514, -5.207839528941200058 ) ) ;
#28368=CARTESIAN_POINT ( 'NONE',  ( -1.879194370357706756, 31.42354579518680424, 3.981814511614890417 ) ) ;
#28370=CARTESIAN_POINT ( 'NONE',  ( 4.581731014592691054, -15.30239759458089388, -0.5121113081912510578 ) ) ;
#28371=CARTESIAN_POINT ( 'NONE',  ( 16.63795227869222515, 147.2809512400332608, 1.774228895505126413 ) ) ;
#28372=CARTESIAN_POINT ( 'NONE',  ( -6.631541954483209765E-14, 98.39146620154573952, -1.863789202389766375E-18 ) ) ;
#28373=CARTESIAN_POINT ( 'NONE',  ( 15.69674027099051195, 120.8333755831694702, 0.2629491152481264193 ) ) ;
#28374=CARTESIAN_POINT ( 'NONE',  ( -7.614108603649571094, 124.2930771091975117, -0.1432033155151095360 ) ) ;
#28376=CARTESIAN_POINT ( 'NONE',  ( 2.829288187452689396, 6.340478445469713620, 3.655570690059357197 ) ) ;
#28377=CARTESIAN_POINT ( 'NONE',  ( 15.64207015331054862, 147.2204672151589193, 0.3125657877211908686 ) ) ;
#28378=CARTESIAN_POINT ( 'NONE',  ( -6.568537450833661140, -2.023721358670699466, -5.272568914532883788 ) ) ;
#28380=CARTESIAN_POINT ( 'NONE',  ( 8.760849894608837118, 117.9156266018594579, -0.3360442439942614157 ) ) ;
#28382=CARTESIAN_POINT ( 'NONE',  ( -0.4066243552753486257, 124.0591982226670211, -0.1013866577921579831 ) ) ;
#28383=CARTESIAN_POINT ( 'NONE',  ( 5.586884702347364673, 79.34146620154574236, 0.1116392523995368424 ) ) ;
#28385=CARTESIAN_POINT ( 'NONE',  ( 2.163044864548389956, 28.58015952483584954, -4.087059112497700042 ) ) ;
#28386=CARTESIAN_POINT ( 'NONE',  ( 2.756409082185796056, 117.3993815990797458, 1.414652500441052396 ) ) ;
#28389=CARTESIAN_POINT ( 'NONE',  ( 0.3351388899280297595, 111.5577547982948801, -3.138814863473581518 ) ) ;
#28390=CARTESIAN_POINT ( 'NONE',  ( -23.09108451844700838, 149.2510847660714148, 0.2673146292145804348 ) ) ;
#28394=ORIENTED_EDGE ( 'NONE', *, *, #870, .T. ) ;
#28396=CARTESIAN_POINT ( 'NONE',  ( -13.59309109316558128, 150.2605162272564030, -0.1417888325812674266 ) ) ;
#28397=CARTESIAN_POINT ( 'NONE',  ( 4.975685353906630581, -15.32372399918348371, 3.685287151418908724 ) ) ;
#28398=CARTESIAN_POINT ( 'NONE',  ( -20.75411281516097262, 147.9587796579421308, 1.616985229673752800 ) ) ;
#28399=CARTESIAN_POINT ( 'NONE',  ( 7.412489149516406250, 158.3992165788449711, -1.135539963648919848 ) ) ;
#28400=CARTESIAN_POINT ( 'NONE',  ( -3.957843245660688680, 22.95775517496322848, 2.395914033147342970 ) ) ;
#28401=CARTESIAN_POINT ( 'NONE',  ( -20.19069946793844039, 128.9119615565081176, -0.7900021088785404988 ) ) ;
#28404=CARTESIAN_POINT ( 'NONE',  ( -0.001261869788360067647, 124.3520329708341876, 0.06314912420803703297 ) ) ;
#28405=CARTESIAN_POINT ( 'NONE',  ( -5.816409885615420272, 28.29835777331257063, 0.3468669796613692569 ) ) ;
#28406=CARTESIAN_POINT ( 'NONE',  ( -7.304865317682213366, 121.1388872696715282, 0.8066302172824781902 ) ) ;
#28408=CARTESIAN_POINT ( 'NONE',  ( 6.663576545388588457, 119.9895581359321994, -0.9799952387295396417 ) ) ;
#28409=CARTESIAN_POINT ( 'NONE',  ( -0.4013927055963539270, 117.8786474493541050, -0.5472391114537519252 ) ) ;
#28411=CIRCLE ( 'NONE', #10030, 0.5079999999999946780 ) ;
#28412=CARTESIAN_POINT ( 'NONE',  ( 5.884536728137893746, 121.1554468101848130, -0.4284271420130266184 ) ) ;
#28413=EDGE_LOOP ( 'NONE', ( #37805, #14428 ) ) ;
#28414=CARTESIAN_POINT ( 'NONE',  ( -17.82368987960366269, 147.7668373613703352, -2.290061161587756633 ) ) ;
#28415=CARTESIAN_POINT ( 'NONE',  ( 3.437591410214265064, -15.71306207096091789, 4.322042152151218453 ) ) ;
#28416=CARTESIAN_POINT ( 'NONE',  ( -4.065972646788793554, 118.2429491485452928, -0.3080848862740693250 ) ) ;
#28418=CARTESIAN_POINT ( 'NONE',  ( -4.816142268852273034, 117.5417147180202022, 0.9796457938337586047 ) ) ;
#28419=CARTESIAN_POINT ( 'NONE',  ( 12.73281086834426290, 125.9836878220586556, 1.772748636948829004 ) ) ;
#28422=CARTESIAN_POINT ( 'NONE',  ( -7.992722778381481596, -7.251515252772184894, -2.728257467986670903 ) ) ;
#28423=CARTESIAN_POINT ( 'NONE',  ( 15.76594527475406338, 145.7191243368997675, 0.6468106390071733935 ) ) ;
#28434=CARTESIAN_POINT ( 'NONE',  ( -5.742584425896393618, 159.1207877133979309, -0.01316620519284343246 ) ) ;
#28437=CARTESIAN_POINT ( 'NONE',  ( 6.965125855778357078, 121.9452357174143913, 0.01188280683295246491 ) ) ;
#28438=CARTESIAN_POINT ( 'NONE',  ( -8.323020013683432694, 120.1269634747937971, 1.118279847563952600 ) ) ;
#28440=CARTESIAN_POINT ( 'NONE',  ( 2.241029890824462356, 115.7026179593451616, -1.621430037521891077 ) ) ;
#28441=CARTESIAN_POINT ( 'NONE',  ( -13.60737276370619675, 150.2179846313823930, -0.4949411041190264759 ) ) ;
#28442=CARTESIAN_POINT ( 'NONE',  ( 4.326150682005948767, -14.13415638199089130, 4.511655897031580764 ) ) ;
#28443=CARTESIAN_POINT ( 'NONE',  ( -0.02399864187742892577, 159.1630378086529731, 1.200990174154242585 ) ) ;
#28444=CARTESIAN_POINT ( 'NONE',  ( 3.222064683888731018, 117.3993833697546449, -1.271138870486020478 ) ) ;
#28446=CARTESIAN_POINT ( 'NONE',  ( 2.778732907383107520, 116.5968896900294709, 0.2040764120049697039 ) ) ;
#28447=CARTESIAN_POINT ( 'NONE',  ( 15.63990901280855716, 147.2221586356311036, 0.4463020126745949057 ) ) ;
#28449=CARTESIAN_POINT ( 'NONE',  ( -0.3507176028818052571, 11.51684809748499028, -0.9106068057588879716 ) ) ;
#28450=CARTESIAN_POINT ( 'NONE',  ( -16.85465591277215225, 155.2173118157008673, -0.4068649486066868715 ) ) ;
#28453=ORIENTED_EDGE ( 'NONE', *, *, #27489, .F. ) ;
#28454=CARTESIAN_POINT ( 'NONE',  ( 8.360143117074091634, 119.6977532042923968, 1.428540289422721488 ) ) ;
#28456=CARTESIAN_POINT ( 'NONE',  ( 1.196040046930053613, 159.0162744061759099, 1.350631977726330701 ) ) ;
#28457=CARTESIAN_POINT ( 'NONE',  ( 2.650128318467419586, 158.3255140430775043, -1.577873239259485638 ) ) ;
#28458=CARTESIAN_POINT ( 'NONE',  ( -8.406874004389072397, 27.76653542065474056, -0.1818807619882521764 ) ) ;
#28459=CARTESIAN_POINT ( 'NONE',  ( -14.69745991766254001, 121.6338672040446767, -1.430666218478179763 ) ) ;
#28460=CARTESIAN_POINT ( 'NONE',  ( 4.797366694452281699, 117.7649354367249401, -0.8643881762267181523 ) ) ;
#28461=CARTESIAN_POINT ( 'NONE',  ( 5.384759902136762477, 117.1811293437636721, 0.8990931802006212337 ) ) ;
#28462=EDGE_CURVE ( 'NONE', #31901, #5241, #23906, .T. ) ;
#28463=CARTESIAN_POINT ( 'NONE',  ( -7.821695933845212778, 154.6216606121152495, 0.03501689623823082270 ) ) ;
#28464=CARTESIAN_POINT ( 'NONE',  ( -5.016192601342632784, 119.3892302351119810, -1.087184205914811352 ) ) ;
#28465=EDGE_CURVE ( 'NONE', #15805, #15736, #40276, .T. ) ;
#28466=CARTESIAN_POINT ( 'NONE',  ( 2.845652327410156612, -15.51977306057959716, 5.689769116265302351 ) ) ;
#28468=EDGE_CURVE ( 'NONE', #39579, #17268, #38224, .T. ) ;
#28471=CARTESIAN_POINT ( 'NONE',  ( 18.57470247777319727, 148.7425187291823363, 2.467219961595396693 ) ) ;
#28476=CARTESIAN_POINT ( 'NONE',  ( -1.859996092182737426, 121.3688471916803451, 0.2894809034927953717 ) ) ;
#28477=CARTESIAN_POINT ( 'NONE',  ( -8.165053131321412749, -1.372107735949496421, -2.092221094348168275 ) ) ;
#28478=CARTESIAN_POINT ( 'NONE',  ( 9.461503173624029372, 123.8597080710187015, 0.7891915900027409725 ) ) ;
#28479=CARTESIAN_POINT ( 'NONE',  ( 22.84463062875807893, 149.4631731099488832, -0.5130293307460864760 ) ) ;
#28483=CARTESIAN_POINT ( 'NONE',  ( 5.586884702347364673, 81.62746620154572952, 0.1116392523995368424 ) ) ;
#28484=LINE ( 'NONE', #18459, #11794 ) ;
#28486=CARTESIAN_POINT ( 'NONE',  ( 8.247687365870664422, 120.4923382035136683, -1.097851349060563475 ) ) ;
#28487=CARTESIAN_POINT ( 'NONE',  ( -5.332935397695335311, 104.6144662015457385, -0.1065647409268299373 ) ) ;
#28488=CARTESIAN_POINT ( 'NONE',  ( -3.627630705028967117, 120.8049117488720015, -0.4115075270184372358 ) ) ;
#28489=CARTESIAN_POINT ( 'NONE',  ( 23.29064488658015719, 149.3519930085110161, 0.4911336289882584638 ) ) ;
#28491=CARTESIAN_POINT ( 'NONE',  ( 4.458631606973747274, 16.91056413504885825, 1.251853190366734259 ) ) ;
#28493=CARTESIAN_POINT ( 'NONE',  ( -8.078287538471746743, 158.6595088495342338, -0.1614234102745197019 ) ) ;
#28494=DIRECTION ( 'NONE',  ( -0.9998004120163609398, 0.000000000000000000, -0.01997839162482749689 ) ) ;
#28496=CARTESIAN_POINT ( 'NONE',  ( -7.785084361432222266, 122.6279490200930837, -0.1367715089808489159 ) ) ;
#28497=AXIS2_PLACEMENT_3D ( 'NONE', #18248, #21864, #14848 ) ;
#28498=CARTESIAN_POINT ( 'NONE',  ( 1.027636191897724816, 24.96647085856908177, -4.506105791511280323 ) ) ;
#28500=CARTESIAN_POINT ( 'NONE',  ( 16.38310316169952330, 155.2191194103077407, 1.312707330359597524 ) ) ;
#28502=CARTESIAN_POINT ( 'NONE',  ( 0.1568724191532814560, 105.9762912437439155, 5.300943958216106644 ) ) ;
#28503=CARTESIAN_POINT ( 'NONE',  ( 9.669117252159342257, 157.4977751962898083, -1.392273965589622353 ) ) ;
#28504=CARTESIAN_POINT ( 'NONE',  ( -16.09548914235268313, 150.9843922791743296, 1.671617783681723646 ) ) ;
#28506=CARTESIAN_POINT ( 'NONE',  ( 2.794707274389933715, 24.31675177525179876, -3.679445548267922916 ) ) ;
#28507=CARTESIAN_POINT ( 'NONE',  ( 0.01133159106138491301, 159.5297144918048673, -0.5670791535570575137 ) ) ;
#28508=CARTESIAN_POINT ( 'NONE',  ( -0.9353260110528880400, 8.126651709021682990, 0.2714574413461035007 ) ) ;
#28511=CARTESIAN_POINT ( 'NONE',  ( -2.758537940429013346, 120.8469057251343060, 0.1732774955029140751 ) ) ;
#28513=CARTESIAN_POINT ( 'NONE',  ( 4.896986379477733742, -14.09362661677580952, 4.057159877996594055 ) ) ;
#28514=CARTESIAN_POINT ( 'NONE',  ( 10.06555281207532815, 123.2077283916686525, -0.8929836319946561352 ) ) ;
#28515=ORIENTED_EDGE ( 'NONE', *, *, #30873, .T. ) ;
#28516=CARTESIAN_POINT ( 'NONE',  ( 0.06879994401897256140, 115.7029491485452581, 1.763577627545462878 ) ) ;
#28517=ADVANCED_FACE ( 'NONE', ( #19666 ), #34815, .T. ) ;
#28518=CARTESIAN_POINT ( 'NONE',  ( -4.707492808873059431, 117.7228541735984066, -1.103909285615471081 ) ) ;
#28519=CARTESIAN_POINT ( 'NONE',  ( 1.563936845556439303, 156.2577446057484281, 0.001723203835320212280 ) ) ;
#28521=CARTESIAN_POINT ( 'NONE',  ( 12.01076045986759233, 121.8643784861682065, 1.757760809232696175 ) ) ;
#28522=CARTESIAN_POINT ( 'NONE',  ( 7.783246152616065672, 154.6561476914895081, 0.1555277812256516956 ) ) ;
#28525=CARTESIAN_POINT ( 'NONE',  ( 4.848342634033197207, 117.5455766057886393, -0.9616795127513765307 ) ) ;
#28526=CARTESIAN_POINT ( 'NONE',  ( 22.77159426375455098, 150.3871190066015799, 0.004147128915567849759 ) ) ;
#28529=CARTESIAN_POINT ( 'NONE',  ( 0.05238710761679706701, 113.0327356262574341, -2.621665085262908423 ) ) ;
#28532=CARTESIAN_POINT ( 'NONE',  ( 1.707630795344756480, -15.17184983623502603, 5.724163072428519072 ) ) ;
#28535=CARTESIAN_POINT ( 'NONE',  ( -4.639261538484346303, 118.0227684624969413, 0.6550054986553982550 ) ) ;
#28538=CARTESIAN_POINT ( 'NONE',  ( 5.953013861836208065, 119.1077922858878679, -1.025847558928856929 ) ) ;
#28539=CARTESIAN_POINT ( 'NONE',  ( -2.588518934356020207, 109.4146836159258669, -3.874296054094246600 ) ) ;
#28540=CARTESIAN_POINT ( 'NONE',  ( 4.596289261446199426, 117.9776677021676221, 0.9191970225659147342 ) ) ;
#28542=CARTESIAN_POINT ( 'NONE',  ( -0.3786798576917292380, 121.5961256765096152, 0.3764709079149205495 ) ) ;
#28543=CARTESIAN_POINT ( 'NONE',  ( -2.424025297795170619, -5.104216246930970868, 3.935102955759355758 ) ) ;
#28546=CARTESIAN_POINT ( 'NONE',  ( 6.650203214911467597, 123.1390089711370166, 0.06171709628626046579 ) ) ;
#28547=CARTESIAN_POINT ( 'NONE',  ( -12.49704818634944381, 126.0212559692275249, -1.705261654849118846 ) ) ;
#28549=CARTESIAN_POINT ( 'NONE',  ( -3.044072069279135651, 34.44269722464345307, 3.574075509920750626 ) ) ;
#28550=CARTESIAN_POINT ( 'NONE',  ( -2.432812730531299650, 115.7029433065083879, 1.605937827969098342 ) ) ;
#28551=CARTESIAN_POINT ( 'NONE',  ( -4.492784857928645792, 12.16275517495587977, -1.104450737933446725 ) ) ;
#28552=CARTESIAN_POINT ( 'NONE',  ( 15.27623507474945086, 120.8527393138689376, 0.8201955439070727216 ) ) ;
#28553=ORIENTED_EDGE ( 'NONE', *, *, #20593, .F. ) ;
#28554=CARTESIAN_POINT ( 'NONE',  ( 1.274087442039063101, 104.6144662015545492, -5.191363564694317034 ) ) ;
#28555=CARTESIAN_POINT ( 'NONE',  ( 3.235674727752381852, -14.79813088844142399, -0.3705354414145333730 ) ) ;
#28556=CARTESIAN_POINT ( 'NONE',  ( -11.87140890173658647, 122.0047285378078357, 1.287708742280476715 ) ) ;
#28557=CARTESIAN_POINT ( 'NONE',  ( -0.8351715869602673870, 27.76506109569598024, 0.5290732382595327854 ) ) ;
#28558=CARTESIAN_POINT ( 'NONE',  ( -0.6518678778066554491, 5.040965284779599820, 0.7259998264446282379 ) ) ;
#28560=AXIS2_PLACEMENT_3D ( 'NONE', #35813, #3440, #38793 ) ;
#28563=CARTESIAN_POINT ( 'NONE',  ( 6.983090746392633719, 124.7321584522365896, 0.1405484879196984560 ) ) ;
#28564=CARTESIAN_POINT ( 'NONE',  ( -10.01767202841750581, 124.1433363813624311, 0.6017494237236775678 ) ) ;
#28566=AXIS2_PLACEMENT_3D ( 'NONE', #21823, #18009, #31432 ) ;
#28567=CARTESIAN_POINT ( 'NONE',  ( 2.131140412894510838, -15.01828590152304344, 5.319755587316977952 ) ) ;
#28568=CARTESIAN_POINT ( 'NONE',  ( 11.17823620286574382, 123.1247571232444784, -1.162497134544157706 ) ) ;
#28569=CARTESIAN_POINT ( 'NONE',  ( -17.39176377602798240, 131.6241255656270255, -2.296140998891703422 ) ) ;
#28571=EDGE_CURVE ( 'NONE', #22816, #27091, #17702, .T. ) ;
#28572=CARTESIAN_POINT ( 'NONE',  ( 8.504347257126880777, 119.0088918578701396, 1.280434527939347866 ) ) ;
#28574=CARTESIAN_POINT ( 'NONE',  ( 3.712124141557857637, 121.0264708767875561, -0.07522066808841043617 ) ) ;
#28575=ORIENTED_EDGE ( 'NONE', *, *, #32552, .T. ) ;
#28576=CARTESIAN_POINT ( 'NONE',  ( 3.220330141560203696, -14.30903721375789317, 2.546581355196453345 ) ) ;
#28581=CARTESIAN_POINT ( 'NONE',  ( -8.287855504117665362, 18.49606730478969752, 1.603550922811438406 ) ) ;
#28582=CARTESIAN_POINT ( 'NONE',  ( 3.381852828898099794, 156.3978305292817481, 1.289121224278522160 ) ) ;
#28584=CARTESIAN_POINT ( 'NONE',  ( 22.98521553460854605, 150.1595482613961110, 0.3823759483556145589 ) ) ;
#28585=CARTESIAN_POINT ( 'NONE',  ( -7.304536785993930970, 123.0387167848234355, -0.07720001398428667783 ) ) ;
#28586=CARTESIAN_POINT ( 'NONE',  ( 3.315635589170360831, -10.27688868798473720, -3.234826238065521053 ) ) ;
#28588=CARTESIAN_POINT ( 'NONE',  ( 2.927854471352651533, -7.645316342317141967, 7.903470162911977681 ) ) ;
#28589=CARTESIAN_POINT ( 'NONE',  ( -5.490732243613680730, 117.1204472715084677, -0.7545457724575556080 ) ) ;
#28590=CARTESIAN_POINT ( 'NONE',  ( -0.4207377039451877243, 124.6436471961814050, -0.04080923199211373281 ) ) ;
#28591=CARTESIAN_POINT ( 'NONE',  ( 6.475684456959278634, -13.49251406434824574, 0.1304084665236045215 ) ) ;
#28593=CARTESIAN_POINT ( 'NONE',  ( 8.369515367582838650, -11.69187915512254783, 0.7729349465547848963 ) ) ;
#28594=CARTESIAN_POINT ( 'NONE',  ( 0.9717804538599504882, 118.1588881589075442, 0.8936527240592224697 ) ) ;
#28596=CARTESIAN_POINT ( 'NONE',  ( 1.860714312465608478, -15.17550571231866741, 5.451645902226371021 ) ) ;
#28597=CARTESIAN_POINT ( 'NONE',  ( 0.8223074630896127779, 121.2007779179981384, -0.3881979734473209320 ) ) ;
#28598=CARTESIAN_POINT ( 'NONE',  ( -10.59335592519058089, 157.9214973357695158, 0.4646299181629828801 ) ) ;
#28602=DIRECTION ( 'NONE',  ( 4.017660918040594346E-17, -1.000000000000000000, -2.376309959284834438E-19 ) ) ;
#28603=CARTESIAN_POINT ( 'NONE',  ( 4.813411144541747788, -15.18245576741394842, 4.205718551895911261 ) ) ;
#28604=CARTESIAN_POINT ( 'NONE',  ( -13.60271346700661255, 122.2126086331852974, 1.213557020469313574 ) ) ;
#28607=CARTESIAN_POINT ( 'NONE',  ( 20.93040400792215650, 136.4823663107028722, -1.114867025985508242 ) ) ;
#28608=CARTESIAN_POINT ( 'NONE',  ( 1.616848224653315569, 9.589005055319924864, -4.350374724214612243 ) ) ;
#28610=ORIENTED_EDGE ( 'NONE', *, *, #33419, .T. ) ;
#28611=CARTESIAN_POINT ( 'NONE',  ( -0.05238710762259597004, 113.0327356262574341, 2.621665085262795625 ) ) ;
#28613=CARTESIAN_POINT ( 'NONE',  ( -10.54966536967472024, 123.3532649940754027, 0.9932924318631480842 ) ) ;
#28615=CARTESIAN_POINT ( 'NONE',  ( 19.01335237852154947, 147.2511928822236769, -1.726116106780063886 ) ) ;
#28616=CARTESIAN_POINT ( 'NONE',  ( -6.782271978585102445, 118.5360090424673274, -1.159066879843025255 ) ) ;
#28618=CARTESIAN_POINT ( 'NONE',  ( 9.756861847786440833, 124.2227999206177032, -0.4199055954619891340 ) ) ;
#28619=EDGE_LOOP ( 'NONE', ( #32967, #17675 ) ) ;
#28620=CARTESIAN_POINT ( 'NONE',  ( -18.00824595900801839, 147.8422069945528108, -2.338981374327669727 ) ) ;
#28621=CARTESIAN_POINT ( 'NONE',  ( 3.879201355988149746, -15.32975156973215292, 1.565980057466964670 ) ) ;
#28622=CARTESIAN_POINT ( 'NONE',  ( -4.065972646788793554, 118.2429491485453070, -0.3080848862740693250 ) ) ;
#28624=CARTESIAN_POINT ( 'NONE',  ( -4.907886530739225428, 117.6707254041722308, 0.8184263495228992769 ) ) ;
#28625=CARTESIAN_POINT ( 'NONE',  ( 17.59644933020960522, 144.4767212251450417, 2.299577266864830438 ) ) ;
#28628=CARTESIAN_POINT ( 'NONE',  ( -3.562413952978887632, 23.18266144714348798, 2.948169924785601470 ) ) ;
#28629=CARTESIAN_POINT ( 'NONE',  ( 7.590630008421936026, 122.4062900713904440, 0.3515417406328249506 ) ) ;
#28633=CARTESIAN_POINT ( 'NONE',  ( -0.3905063200769877674, 117.9394516740210008, 1.395597172505927963 ) ) ;
#28634=AXIS2_PLACEMENT_3D ( 'NONE', #25324, #34302, #11700 ) ;
#28641=CARTESIAN_POINT ( 'NONE',  ( -0.3042766021093734619, 116.4832816433156069, 0.08781055504204338114 ) ) ;
#28644=CARTESIAN_POINT ( 'NONE',  ( -7.800884090505101121, 122.5201264184580339, -0.4525784575430527590 ) ) ;
#28645=CARTESIAN_POINT ( 'NONE',  ( 8.094215573201640979, 117.4700539315208800, 0.1617416903150405150 ) ) ;
#28647=CARTESIAN_POINT ( 'NONE',  ( 2.049820458554627134, 115.7029491482436612, -1.636007937353470387 ) ) ;
#28648=CARTESIAN_POINT ( 'NONE',  ( -9.673174862102012384, 124.8500477395539576, -0.3609973675953364602 ) ) ;
#28649=CARTESIAN_POINT ( 'NONE',  ( 5.820712434538892310, -12.64545009755467575, 1.387492028720230364 ) ) ;
#28650=CARTESIAN_POINT ( 'NONE',  ( -7.920278096381575317, 118.7344292658239340, 0.9023208588851656664 ) ) ;
#28652=CARTESIAN_POINT ( 'NONE',  ( 22.58551839157529173, 137.2245694613254443, 0.7673259740012313701 ) ) ;
#28653=CARTESIAN_POINT ( 'NONE',  ( 5.958951692567330483, 121.5457842488350764, 0.1932771691850621587 ) ) ;
#28655=CARTESIAN_POINT ( 'NONE',  ( -0.8572797930410298584, 14.11360927180527014, 0.4650159543037101773 ) ) ;
#28656=CARTESIAN_POINT ( 'NONE',  ( -9.813487807256334960, 117.9943556427423488, -0.2419611575297472283 ) ) ;
#28657=LINE ( 'NONE', #22245, #10005 ) ;
#28660=CARTESIAN_POINT ( 'NONE',  ( -8.584196973278151788, 118.8304167724923559, 0.8833087002087991468 ) ) ;
#28662=CARTESIAN_POINT ( 'NONE',  ( 3.973247942572128988, 117.7793252414215317, 0.8392447889045230314 ) ) ;
#28663=CARTESIAN_POINT ( 'NONE',  ( 19.62644950592608240, 149.4594839399872512, -1.701416438606881965 ) ) ;
#28664=CARTESIAN_POINT ( 'NONE',  ( 3.644365486686961919, 11.68381519529092216, 7.647779612420950279 ) ) ;
#28665=CARTESIAN_POINT ( 'NONE',  ( -22.13959287704981449, 149.5167998366165989, -1.884152790553834667 ) ) ;
#28666=CARTESIAN_POINT ( 'NONE',  ( 4.692231461927983460, 117.8897540888554261, -0.8101663176662557975 ) ) ;
#28669=CARTESIAN_POINT ( 'NONE',  ( 0.1524052867846317494, 105.8811906981200934, 5.339394923009169958 ) ) ;
#28670=CARTESIAN_POINT ( 'NONE',  ( -8.537819074431743260, 123.3353292868209365, -0.08920952957173433617 ) ) ;
#28671=CARTESIAN_POINT ( 'NONE',  ( -17.69102400252393537, 149.9241642446907292, -2.437100891716216022 ) ) ;
#28672=CARTESIAN_POINT ( 'NONE',  ( 5.114706464973534317, -15.35711304900182128, 3.188446684335360271 ) ) ;
#28673=CIRCLE ( 'NONE', #10973, 0.5080000000000002292 ) ;
#28675=CARTESIAN_POINT ( 'NONE',  ( -3.313229848479803508, 118.1651004895808370, -0.7746738955758309952 ) ) ;
#28677=CARTESIAN_POINT ( 'NONE',  ( 3.311752042447743349, 119.2933411826354728, 0.8767012952321084907 ) ) ;
#28681=CARTESIAN_POINT ( 'NONE',  ( -5.132724724882987921, 121.7269124416356192, 0.09984968675566534280 ) ) ;
#28682=CARTESIAN_POINT ( 'NONE',  ( 8.237246883283409815, -6.118032110028554627, 1.824569540066587114 ) ) ;
#28683=CARTESIAN_POINT ( 'NONE',  ( 1.530927031713785080, 120.6610732671444595, 0.3086461854719845244 ) ) ;
#28684=CARTESIAN_POINT ( 'NONE',  ( 14.33434017258152338, 120.4308286971427862, -0.3827902340739949283 ) ) ;
#28688=TOROIDAL_SURFACE ( 'NONE', #15760, 4.826000000000000512, 0.5080000000000000071 ) ;
#28690=CARTESIAN_POINT ( 'NONE',  ( -4.123530728113747656, 118.2429491485453354, 0.1804270098900454256 ) ) ;
#28691=CARTESIAN_POINT ( 'NONE',  ( -4.713631738767456447, 116.7564862437112794, -0.09418957996065566163 ) ) ;
#28693=CARTESIAN_POINT ( 'NONE',  ( 6.461527244427501593, 120.2130761765557452, -0.9247372324219909068 ) ) ;
#28696=CARTESIAN_POINT ( 'NONE',  ( -12.37067103324092443, 130.6617397222824479, -0.9131297178954277394 ) ) ;
#28698=CARTESIAN_POINT ( 'NONE',  ( 22.66341594453896136, 150.6395781703034231, 0.4783972420343530207 ) ) ;
#28700=CARTESIAN_POINT ( 'NONE',  ( -3.609430071560130848, 3.966570591990036032, 2.889066364458971137 ) ) ;
#28705=CARTESIAN_POINT ( 'NONE',  ( -7.005943499892747894, 121.7887304234075003, 0.2845919825715230167 ) ) ;
#28706=CARTESIAN_POINT ( 'NONE',  ( -3.633452533992190592, 26.69063122243967356, -2.854640957048627747 ) ) ;
#28707=CARTESIAN_POINT ( 'NONE',  ( 1.008854969157035431, 117.0751458430253393, 0.4193480094219991239 ) ) ;
#28710=CARTESIAN_POINT ( 'NONE',  ( 10.59408866556482742, 119.9085704333771787, -1.028430606607102726 ) ) ;
#28711=CARTESIAN_POINT ( 'NONE',  ( -11.64488154209797877, 123.4149316504530702, 1.218180013452823562 ) ) ;
#28712=CARTESIAN_POINT ( 'NONE',  ( 4.233688895176465294, 13.94658232072815807, -1.861163356065342001 ) ) ;
#28713=CARTESIAN_POINT ( 'NONE',  ( -20.68355264112289049, 132.2482564273973935, -1.400420337322433761 ) ) ;
#28716=CARTESIAN_POINT ( 'NONE',  ( -15.88665273169782921, 145.7686330500600036, 0.2792794258575000965 ) ) ;
#28717=CARTESIAN_POINT ( 'NONE',  ( 4.992311776856191763, -13.37494578157311054, 3.269494339340476952 ) ) ;
#28720=CARTESIAN_POINT ( 'NONE',  ( -4.616126210598159751, 118.0369330104597623, -0.7916877136874118648 ) ) ;
#28721=ADVANCED_FACE ( 'NONE', ( #33318 ), #113, .T. ) ;
#28722=CARTESIAN_POINT ( 'NONE',  ( 15.38068278028558922, 147.8292851303062321, 0.2562860988859089195 ) ) ;
#28724=CARTESIAN_POINT ( 'NONE',  ( 12.70548372655388114, 122.4237789811383550, 1.817438969878694577 ) ) ;
#28727=CARTESIAN_POINT ( 'NONE',  ( -7.773589648320968770, 158.6130819278358501, 0.6584978287542905262 ) ) ;
#28728=CARTESIAN_POINT ( 'NONE',  ( 4.887628697012647905, 117.4785758328482217, -0.9709680806009058918 ) ) ;
#28730=CARTESIAN_POINT ( 'NONE',  ( 14.68764241912298729, 120.3119357913517291, -0.01896423869846134910 ) ) ;
#28735=CARTESIAN_POINT ( 'NONE',  ( -4.962531982528343377, 117.4056870407710989, -1.029597432040127991 ) ) ;
#28738=CARTESIAN_POINT ( 'NONE',  ( -4.519476466213967036, 118.0838058619411441, 0.6171013934025890713 ) ) ;
#28741=CARTESIAN_POINT ( 'NONE',  ( -3.160680854049036093, 118.7629491485454309, -1.175202071525837999 ) ) ;
#28743=CARTESIAN_POINT ( 'NONE',  ( -3.526808273775506208, 118.7004473170249668, -0.9357397655257763125 ) ) ;
#28744=CARTESIAN_POINT ( 'NONE',  ( -5.237871118309435303, 118.7524313932052991, -0.6368175916084591881 ) ) ;
#28745=CARTESIAN_POINT ( 'NONE',  ( 4.811267787481693148, 117.7644185172598554, 1.004593082574424256 ) ) ;
#28747=CARTESIAN_POINT ( 'NONE',  ( -13.80305775881212327, 134.3516747369166069, -1.357216474725372546 ) ) ;
#28748=AXIS2_PLACEMENT_3D ( 'NONE', #39294, #10728, #30740 ) ;
#28752=CARTESIAN_POINT ( 'NONE',  ( 0.3637657132512605029, 105.8833743670705445, -5.328194401858565854 ) ) ;
#28753=CARTESIAN_POINT ( 'NONE',  ( -11.01900745353701083, 123.5714170083676748, -1.527874194239944305 ) ) ;
#28754=CARTESIAN_POINT ( 'NONE',  ( 20.51686376604209983, 129.1072961674477710, 0.4099757654675942331 ) ) ;
#28755=CARTESIAN_POINT ( 'NONE',  ( -0.02537255736359531402, 39.20946620154573026, 1.269746523260778304 ) ) ;
#28756=CARTESIAN_POINT ( 'NONE',  ( -3.475550415873033039, 115.7029637594141604, 1.501259963919143070 ) ) ;
#28757=CARTESIAN_POINT ( 'NONE',  ( 3.345514242732226418, 6.565394131763864216, 3.211428121085859733 ) ) ;
#28758=CARTESIAN_POINT ( 'NONE',  ( 14.97360968503852341, 156.1447123740162226, 0.9344295344441085893 ) ) ;
#28760=CARTESIAN_POINT ( 'NONE',  ( -0.1151806861323783349, 105.1224247242857075, -5.344135852030379219 ) ) ;
#28761=CARTESIAN_POINT ( 'NONE',  ( 3.794293369880153310, -15.39696243832143452, 2.404174946430260196 ) ) ;
#28762=CARTESIAN_POINT ( 'NONE',  ( -15.81176147471982674, 128.5598958631237565, 1.562949982248214464 ) ) ;
#28763=CARTESIAN_POINT ( 'NONE',  ( 0.9467939684353117169, 21.72092434492431323, 0.2316696090552467224 ) ) ;
#28765=CARTESIAN_POINT ( 'NONE',  ( 0.2560056206704328097, 6.564126901726701213, 0.9442708342526761056 ) ) ;
#28771=CARTESIAN_POINT ( 'NONE',  ( 5.810938089476312740, 124.3836500214474654, 0.1311214433933295398 ) ) ;
#28773=CARTESIAN_POINT ( 'NONE',  ( -6.511415066510978455, 121.4051597255373025, 0.4520850151541543904 ) ) ;
#28774=CARTESIAN_POINT ( 'NONE',  ( -8.935197197525255319, 123.9063447689825779, -0.1785465045940570761 ) ) ;
#28775=CARTESIAN_POINT ( 'NONE',  ( 2.973740295910565212, -14.46567735677360744, 4.831635400698222504 ) ) ;
#28776=CARTESIAN_POINT ( 'NONE',  ( 0.02874415600660452930, 157.0795416643300939, -1.438475106415293858 ) ) ;
#28777=CARTESIAN_POINT ( 'NONE',  ( -12.01076045986772023, 121.8643784861682065, -1.757760809232695953 ) ) ;
#28779=CARTESIAN_POINT ( 'NONE',  ( 8.016682068476109535, 121.3927152696642366, 1.222808765174667522 ) ) ;
#28780=CARTESIAN_POINT ( 'NONE',  ( 4.074910602682932925, 118.2429491485453354, -0.1454311599470142491 ) ) ;
#28781=CARTESIAN_POINT ( 'NONE',  ( 15.30649785019662801, 148.0176312819745874, -0.02196777213629026379 ) ) ;
#28787=EDGE_CURVE ( 'NONE', #37991, #26194, #32099, .T. ) ;
#28789=CARTESIAN_POINT ( 'NONE',  ( 4.581850893073086795, -15.30275035579069254, -0.5110622633019785699 ) ) ;
#28790=CARTESIAN_POINT ( 'NONE',  ( 14.05504870572961629, 134.4521314832425389, 1.517394082013088674 ) ) ;
#28791=DIRECTION ( 'NONE',  ( -0.01997839162482761832, -1.040247600000950455E-18, 0.9998004120163610509 ) ) ;
#28792=CARTESIAN_POINT ( 'NONE',  ( 23.36108720469560041, 148.8745345081378559, 0.4410421544236570179 ) ) ;
#28793=CARTESIAN_POINT ( 'NONE',  ( -5.578601203221947635, 117.9513286348681476, 0.5234822864975617884 ) ) ;
#28796=CARTESIAN_POINT ( 'NONE',  ( 10.18105065676961729, 125.9743313966586129, 0.2034416216762106322 ) ) ;
#28797=CARTESIAN_POINT ( 'NONE',  ( 21.10297322700568756, 148.1333099715771766, 2.360403108977008557 ) ) ;
#28798=CARTESIAN_POINT ( 'NONE',  ( 2.403447530314441583, 28.79142288871172539, -8.109455235164826803 ) ) ;
#28799=CARTESIAN_POINT ( 'NONE',  ( 8.749828080525578144, 117.9752082124837074, -0.3959020732588000580 ) ) ;
#28800=CARTESIAN_POINT ( 'NONE',  ( 0.1041500444722623514, 106.1822392402443143, -5.212094112990278028 ) ) ;
#28802=CARTESIAN_POINT ( 'NONE',  ( -0.2386826763840395327, 104.6144662015434221, 5.340208467583181573 ) ) ;
#28803=CARTESIAN_POINT ( 'NONE',  ( 3.740357457071568081, -9.854013591530623728, -7.545904704300070875 ) ) ;
#28806=DIRECTION ( 'NONE',  ( 4.017660918040594346E-17, -1.000000000000000000, -2.376309959284834438E-19 ) ) ;
#28807=CARTESIAN_POINT ( 'NONE',  ( 3.177488185987922709, -14.13217061847354472, 2.003775387181677026 ) ) ;
#28808=CARTESIAN_POINT ( 'NONE',  ( 0.3869134157276650776, 116.4813942609866899, -1.514588684444738709 ) ) ;
#28809=CARTESIAN_POINT ( 'NONE',  ( -0.9702981664979649645, 116.7682604261274264, 0.2585377725347693945 ) ) ;
#28812=ORIENTED_EDGE ( 'NONE', *, *, #14420, .F. ) ;
#28814=AXIS2_PLACEMENT_3D ( 'NONE', #41450, #14804, #41022 ) ;
#28815=CARTESIAN_POINT ( 'NONE',  ( 5.396943489592968213, -15.24705710738187570, 2.503009974473451749 ) ) ;
#28816=CARTESIAN_POINT ( 'NONE',  ( -6.797121414357407687, 118.7881172115286148, 0.9472104157431981974 ) ) ;
#28817=CARTESIAN_POINT ( 'NONE',  ( 3.003295232750816002, 159.1263692740743068, -1.093010787580665610 ) ) ;
#28818=CARTESIAN_POINT ( 'NONE',  ( -2.406711483539481389, 4.503775517365914638, 3.979180414515509412 ) ) ;
#28824=CARTESIAN_POINT ( 'NONE',  ( -5.671251014262852941, 28.19322323727007884, 0.3848925825754440644 ) ) ;
#28825=CARTESIAN_POINT ( 'NONE',  ( -17.48603724727291819, 147.5992144370567871, 1.461888717290058315 ) ) ;
#28827=CARTESIAN_POINT ( 'NONE',  ( 11.94919878421452708, 122.6721150436042223, -1.294096368778067996 ) ) ;
#28828=CARTESIAN_POINT ( 'NONE',  ( -20.51891680819880648, 149.8464234248869786, -2.337676305755668871 ) ) ;
#28832=CARTESIAN_POINT ( 'NONE',  ( 8.914966108837827363, 123.2307073318660855, -0.3922733289213620744 ) ) ;
#28834=CARTESIAN_POINT ( 'NONE',  ( -5.835695000730485305, 120.1673030736515955, -1.074193948046630487 ) ) ;
#28835=CARTESIAN_POINT ( 'NONE',  ( 3.866492242221801767, -15.24987600803320831, 0.6064936129020901401 ) ) ;
#28836=CARTESIAN_POINT ( 'NONE',  ( -4.160788897500995454, 118.2392053592570420, -0.3833967187953443712 ) ) ;
#28838=CARTESIAN_POINT ( 'NONE',  ( -4.936883229164080511, 117.6536490159478774, 0.7443082606323431216 ) ) ;
#28839=CARTESIAN_POINT ( 'NONE',  ( 17.90704175211108407, 146.6345634702618952, 2.297399834898016913 ) ) ;
#28842=CARTESIAN_POINT ( 'NONE',  ( 2.739727753987758252, 28.35525327666260864, -3.728201022356329553 ) ) ;
#28843=CARTESIAN_POINT ( 'NONE',  ( 15.82044549406348288, 146.2622375132148989, 0.6472507553222683896 ) ) ;
#28844=DIRECTION ( 'NONE',  ( 0.9998004120163608288, 0.000000000000000000, 0.01997839162482762526 ) ) ;
#28848=DIRECTION ( 'NONE',  ( -0.9998004120163609398, 0.000000000000000000, -0.01997839162482749689 ) ) ;
#28850=CARTESIAN_POINT ( 'NONE',  ( -6.555005513994535572E-14, 79.34146620154574236, -6.390659674827382268E-18 ) ) ;
#28853=CARTESIAN_POINT ( 'NONE',  ( -13.38634958471969405, 156.9592627042916604, 0.007429229355843914098 ) ) ;
#28856=CARTESIAN_POINT ( 'NONE',  ( -5.970780167368420877, 121.4216606831084988, -0.2372359777413814430 ) ) ;
#28859=CARTESIAN_POINT ( 'NONE',  ( 0.7578165627612494237, 115.7030197700005090, -1.728705102643625535 ) ) ;
#28860=CARTESIAN_POINT ( 'NONE',  ( -12.96905644698489013, 133.8854804328748571, -0.4775921230882990698 ) ) ;
#28862=CARTESIAN_POINT ( 'NONE',  ( 6.231544205925810154, -13.28212530995504004, 1.212557631246017564 ) ) ;
#28863=CARTESIAN_POINT ( 'NONE',  ( -20.87437586479492779, 150.1670661137953289, 1.386469220648549383 ) ) ;
#28865=CARTESIAN_POINT ( 'NONE',  ( 5.727173706516636820, 159.1225378944267845, 0.2665985390141683009 ) ) ;
#28866=CARTESIAN_POINT ( 'NONE',  ( 8.943424089997177973, 124.0488429294995711, 0.3121749486774180182 ) ) ;
#28867=CARTESIAN_POINT ( 'NONE',  ( 4.808056391921498474, 118.5266822147775940, -0.8104460292946976674 ) ) ;
#28868=CARTESIAN_POINT ( 'NONE',  ( -0.8667032531718782407, 4.505117207799016477, 0.4606053492026337959 ) ) ;
#28869=CARTESIAN_POINT ( 'NONE',  ( -17.22116264704572686, 122.7389118244895769, -0.4537515290936992574 ) ) ;
#28870=CARTESIAN_POINT ( 'NONE',  ( 5.586884702347363785, 100.6774662015457409, 0.1116392523995368286 ) ) ;
#28873=CARTESIAN_POINT ( 'NONE',  ( -5.574303926328670222, 117.3559425346390839, 0.6178643877552448815 ) ) ;
#28875=CARTESIAN_POINT ( 'NONE',  ( 2.958531772299235918, 50.13146620154573441, 1.329372033065076453 ) ) ;
#28876=CARTESIAN_POINT ( 'NONE',  ( 17.95761459997873999, 128.5942011134444272, 1.926528613670785095 ) ) ;
#28877=CARTESIAN_POINT ( 'NONE',  ( 18.88973499030869618, 150.3568762430427910, -1.706130117709411476 ) ) ;
#28878=AXIS2_PLACEMENT_3D ( 'NONE', #8737, #21697, #5553 ) ;
#28879=CARTESIAN_POINT ( 'NONE',  ( 5.986726992493722754, 14.59627609256335923, -5.926391003037220884 ) ) ;
#28880=CARTESIAN_POINT ( 'NONE',  ( -22.34269864632769043, 148.4347612714453248, -1.893969414928640571 ) ) ;
#28881=CARTESIAN_POINT ( 'NONE',  ( 4.752741535181148613, 117.9428596717473283, -0.6274105461657691896 ) ) ;
#28883=CARTESIAN_POINT ( 'NONE',  ( -15.64855408859538244, 147.2205073051419504, -0.1844942485914528030 ) ) ;
#28884=CARTESIAN_POINT ( 'NONE',  ( -16.04699077284492148, 131.4332636412663931, -2.269269673164716838 ) ) ;
#28885=CARTESIAN_POINT ( 'NONE',  ( 2.040901337265842663, -15.69771917786945359, 5.688463219523050896 ) ) ;
#28889=CARTESIAN_POINT ( 'NONE',  ( 18.01629081398013099, 149.0664087073519681, 2.421686302305671390 ) ) ;
#28891=CARTESIAN_POINT ( 'NONE',  ( -2.922973558833878549, 114.3344743418335128, 2.013556875909916943 ) ) ;
#28892=CARTESIAN_POINT ( 'NONE',  ( 4.580344459542567748, 28.35322510196829171, -7.077419036913218164 ) ) ;
#28893=CARTESIAN_POINT ( 'NONE',  ( 4.473455768776775976, 120.9326014760084007, 0.4576173489010091910 ) ) ;
#28894=CARTESIAN_POINT ( 'NONE',  ( 0.005915287708639699847, 116.9295063353193882, -0.2960251855814708954 ) ) ;
#28895=CARTESIAN_POINT ( 'NONE',  ( 5.237379388564935567, 115.7029491485453150, 1.024072862575109655 ) ) ;
#28897=CARTESIAN_POINT ( 'NONE',  ( -2.744962145539713294, 116.5337465564440578, -0.01469834071105278160 ) ) ;
#28899=CARTESIAN_POINT ( 'NONE',  ( 6.426253893156781416, 120.1342996155803888, -0.9373394870581658322 ) ) ;
#28900=CARTESIAN_POINT ( 'NONE',  ( 3.641052418405362090, -15.28906014138697422, 5.355520729203003150 ) ) ;
#28901=CARTESIAN_POINT ( 'NONE',  ( -15.91553746749639942, 146.9815093338748966, -1.044385907527698443 ) ) ;
#28902=CARTESIAN_POINT ( 'NONE',  ( -6.068413118431933206, 121.4395679076997823, -0.1212613395058407956 ) ) ;
#28903=CARTESIAN_POINT ( 'NONE',  ( 22.66375647020915807, 150.6386093215955100, 0.4528757910175261192 ) ) ;
#28904=EDGE_LOOP ( 'NONE', ( #12989, #10215, #24939, #33338 ) ) ;
#28905=CARTESIAN_POINT ( 'NONE',  ( 4.364008504204949013, 7.202613900313124873, 1.580794030135405537 ) ) ;
#28907=CARTESIAN_POINT ( 'NONE',  ( -22.46755768833301303, 150.8526571111528654, -0.4489552724284875951 ) ) ;
#28910=CARTESIAN_POINT ( 'NONE',  ( 6.972867087885918025, 121.1626460931736347, 0.9873634393825863054 ) ) ;
#28911=CARTESIAN_POINT ( 'NONE',  ( 1.748379858460863856, 5.525481214791113871, -4.283037568778763848 ) ) ;
#28912=CARTESIAN_POINT ( 'NONE',  ( 2.920589480036142049, 117.1197906563906344, 0.5561477985301584992 ) ) ;
#28914=CARTESIAN_POINT ( 'NONE',  ( 1.569777447552894500, 106.5494078766684822, 5.038031550283630366 ) ) ;
#28915=CARTESIAN_POINT ( 'NONE',  ( 13.59286959522813909, 121.6867650304669013, -1.114243377227002396 ) ) ;
#28916=CARTESIAN_POINT ( 'NONE',  ( 1.391598188199559161, 15.24595356501894017, -4.406646451508545503 ) ) ;
#28917=CARTESIAN_POINT ( 'NONE',  ( -5.829268545577303229, 117.2350771734024164, -0.5950018394081720841 ) ) ;
#28918=ORIENTED_EDGE ( 'NONE', *, *, #23848, .F. ) ;
#28919=CARTESIAN_POINT ( 'NONE',  ( -15.66930740726056293, 147.5723176251010784, 0.2779681209298468514 ) ) ;
#28920=CARTESIAN_POINT ( 'NONE',  ( 4.815776949948430641, -14.65450223259012752, 4.385166865640996114 ) ) ;
#28922=CARTESIAN_POINT ( 'NONE',  ( -4.608275094037495911, 117.9807440340913303, -0.9110670956906681273 ) ) ;
#28923=CARTESIAN_POINT ( 'NONE',  ( 11.82813386268891165, 130.3161362890850512, 0.2363542639706543158 ) ) ;
#28924=AXIS2_PLACEMENT_3D ( 'NONE', #435, #32577, #38559 ) ;
#28925=ORIENTED_EDGE ( 'NONE', *, *, #19182, .F. ) ;
#28926=CARTESIAN_POINT ( 'NONE',  ( 1.054772537320672887, 158.2739225783580537, 1.630455200628576851 ) ) ;
#28928=CARTESIAN_POINT ( 'NONE',  ( -21.97872426622829067, 150.5960492154097778, 0.7309654607748480304 ) ) ;
#28929=B_SPLINE_CURVE_WITH_KNOTS ( 'NONE', 3,
 ( #541, #36728, #39085, #29492, #333, #29910 ),
 .UNSPECIFIED., .F., .F.,
 ( 4, 2, 4 ),
 ( 0.000000000000000000, 0.4999999999999998890, 0.5010344700412979746 ),
 .UNSPECIFIED. ) ;
#28930=CARTESIAN_POINT ( 'NONE',  ( 4.987388792096843382, 117.4712839033013694, -0.8196840828292851766 ) ) ;
#28931=CARTESIAN_POINT ( 'NONE',  ( 22.86474403352223561, 150.1122123445777277, -0.1353427831800515235 ) ) ;
#28932=CARTESIAN_POINT ( 'NONE',  ( -5.217562798876929975, 115.7029491485453576, -1.133914326198557587 ) ) ;
#28933=DIRECTION ( 'NONE',  ( 5.206863593109713661E-17, -1.000000000000000000, 1.077750396879097183E-30 ) ) ;
#28935=CARTESIAN_POINT ( 'NONE',  ( 1.913489507893775698, -15.20816560145711627, 5.407669831558338913 ) ) ;
#28939=CARTESIAN_POINT ( 'NONE',  ( -4.689025485151536721, 118.0064216981434129, 0.5872937155463054948 ) ) ;
#28942=ORIENTED_EDGE ( 'NONE', *, *, #25895, .F. ) ;
#28943=CARTESIAN_POINT ( 'NONE',  ( -1.580745382963060441, 115.6909491485438650, -1.732186872891357421 ) ) ;
#28944=CARTESIAN_POINT ( 'NONE',  ( -3.461366646325571672, 118.6363893151611393, -0.9320101371334748031 ) ) ;
#28945=CARTESIAN_POINT ( 'NONE',  ( -5.292905998138487611, 116.9650601603920279, -0.9543338394691547322 ) ) ;
#28946=CARTESIAN_POINT ( 'NONE',  ( 4.666052514813301855, 117.8348563039157000, 1.040256194233742937 ) ) ;
#28947=CARTESIAN_POINT ( 'NONE',  ( 3.026662605148213725, -13.87242449132548217, 1.205013440933411228 ) ) ;
#28948=CARTESIAN_POINT ( 'NONE',  ( -9.710114326862248291, 153.9716628027005925, -1.336640340121901360 ) ) ;
#28949=CARTESIAN_POINT ( 'NONE',  ( -0.1058213901579529159, 105.9761915687834914, 5.295735085524055030 ) ) ;
#28950=FACE_OUTER_BOUND ( 'NONE', #25617, .T. ) ;
#28951=CARTESIAN_POINT ( 'NONE',  ( 6.300894124712196565, 120.0808430858776887, -0.2013153013476511599 ) ) ;
#28952=CARTESIAN_POINT ( 'NONE',  ( -3.458815983099662539, 120.0787590019544098, -0.7189451402107607247 ) ) ;
#28954=CARTESIAN_POINT ( 'NONE',  ( 15.47023807670824525, 120.6682698389898576, 0.3091321738930620788 ) ) ;
#28955=CARTESIAN_POINT ( 'NONE',  ( -6.341522686457216729, 28.91400451575042752, 0.4646910016499272156 ) ) ;
#28958=CARTESIAN_POINT ( 'NONE',  ( -2.070226828232369254, -8.352695179381779411, -4.151654383260235726 ) ) ;
#28959=CARTESIAN_POINT ( 'NONE',  ( 3.814135102937691979, 116.8938343318378088, 0.4443717020561036013 ) ) ;
#28962=CARTESIAN_POINT ( 'NONE',  ( 2.500182370989485925, -15.36189011820890471, 4.810483652035355107 ) ) ;
#28963=CARTESIAN_POINT ( 'NONE',  ( -19.45999741126005489, 148.3988719805327037, 1.735632530687203579 ) ) ;
#28964=CARTESIAN_POINT ( 'NONE',  ( 0.9435450883166688341, 2.505659174922684418, 0.2465458143858453577 ) ) ;
#28965=CARTESIAN_POINT ( 'NONE',  ( 0.8400667230086624748, -1.857414735510459547, 0.5005776846920441114 ) ) ;
#28969=CARTESIAN_POINT ( 'NONE',  ( 2.840201032364488842, 114.3344743418335128, 2.128718819835312637 ) ) ;
#28970=CARTESIAN_POINT ( 'NONE',  ( -7.149839403334910415, 121.7184703992695773, 0.4778388566947555649 ) ) ;
#28971=CARTESIAN_POINT ( 'NONE',  ( 3.948573903914379457, -12.48127506095717010, 1.805458641749257520 ) ) ;
#28972=CARTESIAN_POINT ( 'NONE',  ( 5.873652769538419527, 120.2771794157441008, -0.8114825934776856986 ) ) ;
#28973=CARTESIAN_POINT ( 'NONE',  ( -10.78248307147206475, 155.9024031350590462, -2.169211330499415613 ) ) ;
#28975=CARTESIAN_POINT ( 'NONE',  ( 1.852819980464847305, -15.24972552306870455, 5.408883774200016425 ) ) ;
#28976=CARTESIAN_POINT ( 'NONE',  ( -3.409494081961937706, 34.07961874667937963, 1.512047642211102216 ) ) ;
#28978=CARTESIAN_POINT ( 'NONE',  ( 1.588992450109044663, 120.9073379818811134, -0.1002710119552033263 ) ) ;
#28981=ADVANCED_FACE ( 'NONE', ( #33109 ), #825, .F. ) ;
#28985=CARTESIAN_POINT ( 'NONE',  ( -4.580899860306842264, 27.87760619330545708, 0.5121266511161914892 ) ) ;
#28987=CARTESIAN_POINT ( 'NONE',  ( 3.555938004931198382, 120.5283240077024800, 0.5587344792657806813 ) ) ;
#28989=CARTESIAN_POINT ( 'NONE',  ( 21.90557141593800949, 151.4352167165723415, 0.3614719721193419555 ) ) ;
#28990=AXIS2_PLACEMENT_3D ( 'NONE', #1096, #16843, #23210 ) ;
#28991=CARTESIAN_POINT ( 'NONE',  ( -7.500421786656923828, 123.6595150816924047, -0.1155007223820209428 ) ) ;
#28992=CARTESIAN_POINT ( 'NONE',  ( -4.645572480595541620, 117.9340260526530813, 0.7769932229682322555 ) ) ;
#28993=DIRECTION ( 'NONE',  ( 0.9998004120163608288, 0.000000000000000000, 0.01997839162482736852 ) ) ;
#28994=CARTESIAN_POINT ( 'NONE',  ( -4.761417829420920178, 31.88590546210041410, 0.3075751490760140205 ) ) ;
#28995=CARTESIAN_POINT ( 'NONE',  ( 3.096092393556910238, 118.0390668470448929, 0.8277768005040343491 ) ) ;
#28996=CARTESIAN_POINT ( 'NONE',  ( 4.103230867730633058, 22.16771668783608007, 2.168033597859526651 ) ) ;
#28997=CARTESIAN_POINT ( 'NONE',  ( -8.368269197548203309, 31.49133049583987187, -0.7708832981534754492 ) ) ;
#28998=CARTESIAN_POINT ( 'NONE',  ( -8.723683256387298357, 117.9901670288953284, -0.7589823086946332342 ) ) ;
#28999=CARTESIAN_POINT ( 'NONE',  ( -1.733652500133141983, 120.5851793143259130, -0.4713357653683601378 ) ) ;
#29002=CARTESIAN_POINT ( 'NONE',  ( 0.7256241136818852855, 104.6144662015456959, 4.780927069660905637 ) ) ;
#29003=CARTESIAN_POINT ( 'NONE',  ( -3.366035089439492811, 13.68705809737886447, 3.178168622443589886 ) ) ;
#29006=CARTESIAN_POINT ( 'NONE',  ( 2.768561164044480272, -13.57843041371762460, 0.3119852368007841603 ) ) ;
#29007=CARTESIAN_POINT ( 'NONE',  ( 0.5468943487520009361, 107.2171362991012842, -4.774625097732313250 ) ) ;
#29008=CARTESIAN_POINT ( 'NONE',  ( -2.881812722985489295, 116.8851979753409580, 0.3221759108904498903 ) ) ;
#29011=EDGE_LOOP ( 'NONE', ( #12118, #22724, #12555, #14091 ) ) ;
#29013=CARTESIAN_POINT ( 'NONE',  ( 5.875553665316252783, -14.89341971632543427, 0.3075322240006022056 ) ) ;
#29014=CARTESIAN_POINT ( 'NONE',  ( -13.04666149862689828, 122.0079276396459704, 1.242691380407616286 ) ) ;
#29015=CARTESIAN_POINT ( 'NONE',  ( 3.032027503100430899, 117.5448765310053005, -0.5892388327060570363 ) ) ;
#29016=CARTESIAN_POINT ( 'NONE',  ( -3.609430071560130848, 3.966570591990036032, 2.889066364458971137 ) ) ;
#29018=EDGE_CURVE ( 'NONE', #23764, #40944, #11693, .T. ) ;
#29019=ORIENTED_EDGE ( 'NONE', *, *, #790, .T. ) ;
#29021=AXIS2_PLACEMENT_3D ( 'NONE', #33518, #39705, #16890 ) ;
#29022=CARTESIAN_POINT ( 'NONE',  ( 0.3576380314657462423, 120.7331730230137623, 0.5311352847986058334 ) ) ;
#29023=CARTESIAN_POINT ( 'NONE',  ( -4.801647862234980302, 117.4032733357427105, 1.015449305853463491 ) ) ;
#29024=CARTESIAN_POINT ( 'NONE',  ( -17.55799248491159759, 146.4615580561186050, 1.465990265564338868 ) ) ;
#29026=CARTESIAN_POINT ( 'NONE',  ( 5.876330432687248084, 119.7498067647950961, -0.9241301181796094388 ) ) ;
#29027=CARTESIAN_POINT ( 'NONE',  ( -11.89465070410510883, 120.7721054874162974, -1.583610710261881049 ) ) ;
#29030=CARTESIAN_POINT ( 'NONE',  ( 4.466647412601136402, 118.1267704881138769, -0.5518082194138826946 ) ) ;
#29031=CARTESIAN_POINT ( 'NONE',  ( 16.17919469456363757, 146.7365623387580342, -0.6462428564100393125 ) ) ;
#29033=CARTESIAN_POINT ( 'NONE',  ( -0.8526219981722428232, 157.1001331247151143, -1.466586365881669352 ) ) ;
#29034=CARTESIAN_POINT ( 'NONE',  ( 2.939911579247540541, -15.51555475658629391, 4.434558482745560859 ) ) ;
#29035=CARTESIAN_POINT ( 'NONE',  ( -4.065972646788793554, 118.2429491485453070, -0.3080848862740693250 ) ) ;
#29040=CARTESIAN_POINT ( 'NONE',  ( -4.947839762289965471, 117.6245774892788205, 0.7566444795842055537 ) ) ;
#29041=CARTESIAN_POINT ( 'NONE',  ( 6.534901955148902708, 120.8223817900871495, 1.022280983926979303 ) ) ;
#29044=CARTESIAN_POINT ( 'NONE',  ( 4.815508964495446520, -10.08105153662837061, -6.929324068793707880 ) ) ;
#29045=CARTESIAN_POINT ( 'NONE',  ( 10.42406139656909758, 153.0845720789597522, 0.4157246174923903692 ) ) ;
#29047=CIRCLE ( 'NONE', #16795, 3.683000000000001162 ) ;
#29049=CARTESIAN_POINT ( 'NONE',  ( -0.1313276950969750889, 117.9394518359770530, 1.405280662291707339 ) ) ;
#29052=CARTESIAN_POINT ( 'NONE',  ( -8.314080580956096256, 119.9198965104016565, -1.454033707264238195 ) ) ;
#29057=CARTESIAN_POINT ( 'NONE',  ( -5.816519783795449428, 117.0096406922080376, 0.1181936270109639059 ) ) ;
#29060=CARTESIAN_POINT ( 'NONE',  ( 7.817500836422443200, 122.5000612203145778, -0.1730797909992374539 ) ) ;
#29061=EDGE_LOOP ( 'NONE', ( #22001, #33636, #37886, #5115 ) ) ;
#29062=CARTESIAN_POINT ( 'NONE',  ( 3.014263063806961185, 115.7029722995355741, -1.552917389829764572 ) ) ;
#29063=CARTESIAN_POINT ( 'NONE',  ( -9.045001602728936163, 123.9859359328134190, -0.2652644514531632969 ) ) ;
#29064=CARTESIAN_POINT ( 'NONE',  ( 4.978007909399718045, -14.21992039213325398, 4.057701602070913793 ) ) ;
#29065=CARTESIAN_POINT ( 'NONE',  ( -15.22748671137947518, 123.1171956318823533, 1.061527106655570707 ) ) ;
#29067=CARTESIAN_POINT ( 'NONE',  ( 23.26558566580226639, 149.3390083238215595, 0.6953334291057012839 ) ) ;
#29068=AXIS2_PLACEMENT_3D ( 'NONE', #34577, #27958, #34364 ) ;
#29069=CARTESIAN_POINT ( 'NONE',  ( 1.634769624693551027, 120.9957931938675841, 0.1332809887664035686 ) ) ;
#29071=CARTESIAN_POINT ( 'NONE',  ( 0.8411255309083253140, 9.366862202269544468, -0.4933303560167117130 ) ) ;
#29072=CARTESIAN_POINT ( 'NONE',  ( -20.68667083660097816, 152.5691845998198346, -0.5628278541506290811 ) ) ;
#29075=ORIENTED_EDGE ( 'NONE', *, *, #16675, .T. ) ;
#29076=CARTESIAN_POINT ( 'NONE',  ( 5.537890225724539484, 117.2894663389777463, 0.8086631719369541393 ) ) ;
#29077=ORIENTED_EDGE ( 'NONE', *, *, #13171, .F. ) ;
#29078=DIRECTION ( 'NONE',  ( 0.9998004120163608288, 0.000000000000000000, 0.01997839162482760791 ) ) ;
#29079=CARTESIAN_POINT ( 'NONE',  ( 20.92851329017031148, 150.0074445146613584, 2.223361304733721955 ) ) ;
#29080=CARTESIAN_POINT ( 'NONE',  ( 5.018689047519269586, 118.8869175073591578, -0.8997529482361044106 ) ) ;
#29081=CARTESIAN_POINT ( 'NONE',  ( -3.928768625441322104, 16.54256788600693895, -7.448509604454663702 ) ) ;
#29082=CARTESIAN_POINT ( 'NONE',  ( -4.887760029584870658, 117.7409041207840090, -0.8724161813180755232 ) ) ;
#29083=CARTESIAN_POINT ( 'NONE',  ( 4.706159131466354673, 117.8933722103456887, -0.8009178487074127828 ) ) ;
#29086=CARTESIAN_POINT ( 'NONE',  ( -14.67586190579459604, 148.8475317811793559, -0.2426438148417037477 ) ) ;
#29087=CARTESIAN_POINT ( 'NONE',  ( -12.85862358090732194, 153.8477531742089468, -2.225956515383983092 ) ) ;
#29089=CARTESIAN_POINT ( 'NONE',  ( 4.032098335577404491, -15.72255795053374783, 4.298576634473052493 ) ) ;
#29090=CARTESIAN_POINT ( 'NONE',  ( 4.726447923106682047, 118.5931160184169073, 1.020546415897938708 ) ) ;
#29091=ADVANCED_FACE ( 'NONE', ( #23700 ), #28688, .T. ) ;
#29094=CARTESIAN_POINT ( 'NONE',  ( 18.30884121703834921, 147.6341482083243761, 2.394331140672893099 ) ) ;
#29098=CARTESIAN_POINT ( 'NONE',  ( -4.981054720647350109, 121.2162878128435892, 0.1538846217318252940 ) ) ;
#29099=CARTESIAN_POINT ( 'NONE',  ( -1.630640499631123452, 19.93121390510496838, -8.274862188801900942 ) ) ;
#29100=CARTESIAN_POINT ( 'NONE',  ( 9.448695200928735716, 153.9068681542131856, 1.043141309954137563 ) ) ;
#29101=CARTESIAN_POINT ( 'NONE',  ( 6.911158149689221375, 117.5201695557886410, -0.4259063301137958613 ) ) ;
#29102=CARTESIAN_POINT ( 'NONE',  ( 5.332935392244917416, 115.7029491189645825, 0.1065647408284378928 ) ) ;
#29103=CARTESIAN_POINT ( 'NONE',  ( 4.581731014592691054, -15.30239759458089388, -0.5121113081912510578 ) ) ;
#29104=UNCERTAINTY_MEASURE_WITH_UNIT (LENGTH_MEASURE( 1.000000000000000082E-05 ), #24013, 'distance_accuracy_value', 'NONE');
#29105=CARTESIAN_POINT ( 'NONE',  ( -14.90010799439755651, 120.3262451489332818, -0.2810636626631669022 ) ) ;
#29107=CARTESIAN_POINT ( 'NONE',  ( 4.708107117004457720, 119.7860639267805283, -0.7247629778888364793 ) ) ;
#29108=CARTESIAN_POINT ( 'NONE',  ( 4.376067305622965975, -15.09428741806564034, 4.801372945859158747 ) ) ;
#29109=CARTESIAN_POINT ( 'NONE',  ( -9.499123264218946261, 124.0643708016488063, -0.7086372128104243551 ) ) ;
#29110=CARTESIAN_POINT ( 'NONE',  ( 3.889980283446199838, -12.05568003970028457, 1.127423567058935205 ) ) ;
#29112=CARTESIAN_POINT ( 'NONE',  ( 14.89944180985295574, 120.3262451489332818, 0.3144022614128134108 ) ) ;
#29114=CARTESIAN_POINT ( 'NONE',  ( -4.374560056058969693, 13.03735028915297534, 1.504755201125916875 ) ) ;
#29115=CARTESIAN_POINT ( 'NONE',  ( -1.165688202727937828, 105.1231265544458466, 5.215447108397309073 ) ) ;
#29117=CARTESIAN_POINT ( 'NONE',  ( 0.4456520612264974202, 105.8204370143460693, 5.321309051583069660 ) ) ;
#29119=CARTESIAN_POINT ( 'NONE',  ( 6.106687141107508765, 121.1151792713842781, 0.7286823287528870763 ) ) ;
#29120=CARTESIAN_POINT ( 'NONE',  ( 3.912982837994093188, 14.17146771520798332, -2.459658384584827218 ) ) ;
#29121=CARTESIAN_POINT ( 'NONE',  ( 5.838122194618472705, 117.4684171610355747, 0.7518181979692857286 ) ) ;
#29123=CARTESIAN_POINT ( 'NONE',  ( 2.697962015452238571, 107.8418472309013794, 4.476687650674952224 ) ) ;
#29124=CARTESIAN_POINT ( 'NONE',  ( 7.864631202759840178, 118.9574329095587757, -0.9664042006415772823 ) ) ;
#29125=CARTESIAN_POINT ( 'NONE',  ( -4.422273941422524501, 8.986318502778324557, 1.404945367500548548 ) ) ;
#29126=CARTESIAN_POINT ( 'NONE',  ( -22.82453445504512857, 148.6346580502994073, -1.538154475459324821 ) ) ;
#29128=CARTESIAN_POINT ( 'NONE',  ( -7.884012465051817742, 154.6027768716304820, 0.2197914096094752134 ) ) ;
#29129=CARTESIAN_POINT ( 'NONE',  ( 4.359322289182287591, -14.87073230766630694, 4.862486896750754184 ) ) ;
#29131=EDGE_CURVE ( 'NONE', #2172, #16499, #30062, .T. ) ;
#29133=CARTESIAN_POINT ( 'NONE',  ( -0.03212618750959795461, 158.2819368290249713, 1.607725792532325615 ) ) ;
#29134=DIRECTION ( 'NONE',  ( -0.9998004120163610509, -4.016384292689131511E-17, -0.01997839162482749689 ) ) ;
#29137=CARTESIAN_POINT ( 'NONE',  ( -22.86776170061665425, 148.6346580502994073, 0.6251136566479099654 ) ) ;
#29138=CARTESIAN_POINT ( 'NONE',  ( 4.865100810417520627, 117.4776273858779234, -0.9871917231070708176 ) ) ;
#29139=CARTESIAN_POINT ( 'NONE',  ( 5.699072711719705531, 159.1209727096294273, -0.1881040421785056538 ) ) ;
#29140=( BOUNDED_SURFACE ( )  B_SPLINE_SURFACE ( 3, 3, ( 
 ( #7657, #20614, #33644, #4471, #17429, #1273, #28282, #8903, #11885, #17845, #21241, #8488, #37447, #27649, #34271, #15493, #21038, #27859, #2317, #8271, #5099, #30844, #41077, #41289, #18681, #34681, #2102, #5307, #18051, #24874, #31054, #37869, #8693, #1691, #12093, #12307, #21656, #5510, #14855, #21444, #1893, #34473, #18468, #40867, #31689, #24443, #28066, #15278, #25295, #18256, #14646, #11668, #24655, #31260, #25081, #2531, #4890, #37664, #41500, #15066, #34063, #31473, #21869, #38088, #34895, #5726, #28491, #8063, #40660, #11452, #5932, #9322, #38716, #25506, #15694, #22285, #3581, #9118, #15905, #32529, #38506, #35310, #18893, #29114, #29333, #6759, #22705, #32318, #35521, #6138, #42132, #19102, #12929, #38927, #31902, #174, #387, #25919, #35107, #22080, #19727, #6342, #32110, #2941, #9526, #22494, #3147, #9737, #16543, #28905, #13144, #13353, #41920, #35735, #19313, #6547, #29553, #12720, #16110, #2738, #19521, #3360, #38298, #28700, #16327, #26136, #35947, #9943, #25710, #39137, #22915, #41709, #32748, #12515, #30376, #802, #23341, #13777, #20567, #7195, #36998, #23124, #39566, #36789, #33804, #26774, #33595, #4428, #13570, #1015, #29758, #32968, #29962, #17386, #1431, #39784, #1226, #4632, #10370, #14185, #20780, #23557, #10579, #7394, #36161, #27188, #3793, #26984, #20153, #13979, #4004, #40203, #10999, #17175, #36578, #33176, #16962, #20355, #597, #6977, #33379, #26559, #4213, #36379, #30174, #39994, #23979, #7818, #10785, #19949, #17588, #30591, #26343, #23765, #39350, #10153, #7606, #16753 ),
 ( #2271, #12045, #28234, #40611, #21395, #1844, #37198, #18209, #34849, #18421, #31001, #11410, #14808, #8645, #37401, #25034, #11203, #27601, #24823, #21821, #27810, #21606, #34634, #1642, #31210, #17795, #20990, #18004, #5461, #31644, #40818, #31429, #5681, #24397, #15235, #8857, #11619, #24606, #37611, #24188, #2053, #21193, #8437, #8220, #34422, #15018, #5049, #38037, #30792, #5255, #41240, #18639, #28018, #34012, #34219, #41028, #11836, #14390, #27397, #8019, #37818, #40408, #4841, #14596, #35475, #16280, #38879, #12679, #19270, #42090, #22658, #3314, #6299, #12259, #15650, #2900, #31854, #22038, #28655, #9895, #15446, #22243, #9691, #2693, #41667, #25251, #32277, #35691, #13094, #35269, #28449, #3107, #29285, #6500, #25669, #16068, #12885, #19478, #129, #29071, #38256, #12475, #15862, #25469, #35066, #38465, #22868, #41454, #6093, #32486, #9283, #19056, #9073, #25873, #26086, #39093, #35906, #38676, #41880, #32061, #6715, #28868, #19684, #2484, #5888, #18849, #9482, #22446, #29501, #16495, #14137, #757, #32915, #3745, #33127, #3957, #26726, #7349, #40152, #19900, #36736, #8333, #26512, #23502, #13732, #967, #11517, #29708, #39734, #341, #20308, #36529, #24502, #26294, #10533, #20519, #30328, #4380, #16703, #33334, #20103, #13307, #4164, #37507, #7559, #7146, #550, #16918, #26932, #13524, #1174, #39302, #39517, #13936, #32700, #29918, #39944, #10736, #10323, #17127, #36115, #10110, #36330, #23717, #3536, #30128, #33549, #23081, #23292, #17338, #27139, #6929, #24937, #2382, #31119, #8967, #28130, #21720 ),
 ( #41356, #28557, #25564, #31538, #27920, #5368, #11946, #34744, #38366, #15759, #18114, #2168, #12577, #31324, #5576, #21935, #37935, #2801, #37725, #12159, #41565, #38568, #15342, #40926, #18322, #8759, #18533, #9180, #28763, #1956, #15127, #21303, #28347, #34332, #25151, #35166, #15555, #38154, #34964, #18742, #12374, #22137, #5787, #14916, #34541, #31752, #8549, #11732, #41140, #41777, #5160, #2595, #25361, #21508, #5993, #24721, #18956, #31962, #20006, #36005, #3420, #6608, #9587, #232, #32378, #26191, #10003, #3007, #13415, #13625, #13209, #6198, #35368, #33023, #19579, #22556, #35586, #9797, #22763, #16387, #39195, #16816, #38776, #26404, #26616, #3207, #22975, #32587, #19787, #29818, #6403, #29392, #19168, #6817, #32806, #657, #15966, #3637, #39409, #7038, #23182, #19372, #16602, #38987, #32171, #29610, #9381, #10212, #25979, #16169, #35796, #445, #29174, #3852, #28964, #20, #36217, #22345, #41980, #12779, #25769, #12986, #14242, #862, #4064, #1070, #30650, #14658, #14038, #1494, #17857, #10637, #17648, #34076, #36850, #27042, #20626, #7250, #27249, #4272, #40051, #33863, #39840, #26833, #20209, #30438, #14450, #8077, #24043, #33656, #7668, #23616, #1284, #20417, #40265, #11058, #33236, #27460, #1703, #37058, #36431, #23400, #21050, #4481, #36637, #7459, #10844, #23830, #17441, #7876, #4903, #33445, #40473, #39623, #17235, #20839, #4693, #11264, #30858, #30231, #24250, #17024, #37258, #10429, #30022, #13835, #8706, #15505, #25307, #41513, #11681, #34693, #15078, #8284, #31485, #5946, #31702, #2115 ),
 ( #40880, #38100, #35119, #28078, #21881, #5739, #14869, #2330, #31067, #34283, #31272, #18692, #2752, #41089, #2544, #18905, #24667, #28506, #22092, #24886, #11897, #21670, #37459, #15290, #34486, #37883, #37676, #5523, #28295, #18270, #9131, #1905, #18480, #34907, #31916, #41302, #5112, #8499, #12106, #25096, #12320, #27662, #24455, #21456, #40673, #8915, #11466, #38311, #21253, #18064, #27871, #5318, #13155, #35957, #16554, #19532, #25518, #28916, #16122, #2953, #35323, #41931, #23133, #28712, #35535, #6771, #15916, #32539, #19116, #22298, #19325, #19737, #32977, #32329, #32759, #36172, #12732, #3592, #10165, #12939, #3158, #38937, #38518, #3372, #22506, #29125, #25721, #42145, #16338, #6354, #39360, #32122, #35745, #22926, #19959, #25930, #6149, #38729, #9749, #22717, #29562, #6989, #12527, #9536, #15708, #6557, #41722, #29344, #398, #9953, #185, #26147, #39149, #13365, #26354, #9335, #13581, #16973, #4226, #33188, #23352, #29972, #11215, #16764, #23567, #40213, #4016, #813, #26569, #36800, #37010, #14401, #30388, #40006, #1026, #13788, #7619, #26785, #20579, #4438, #39577, #7828, #8030, #33606, #607, #29771, #27409, #13990, #39795, #10589, #17186, #30185, #10797, #17396, #24199, #36589, #20790, #21001, #7407, #1239, #26995, #14195, #37210, #20369, #23779, #10382, #27200, #11011, #3802, #36389, #23990, #33815, #1441, #17599, #33391, #4642, #30603, #7205, #40420, #20163, #38047, #8448, #31013, #21405, #28245, #14819, #2494, #30804, #5061, #2280, #41464, #34433, #41249, #37624, #8867, #12271, #18016, #12055 ),
 ( #1856, #28458, #14608, #27821, #5267, #31438, #38265, #18648, #15244, #2064, #9082, #40623, #40830, #11629, #25044, #15457, #34858, #11421, #34231, #24616, #18219, #31220, #15028, #28028, #31654, #27613, #18430, #24407, #41038, #11848, #25260, #24834, #37829, #5690, #17807, #34026, #4851, #8656, #21205, #21616, #8232, #34643, #5471, #37413, #21829, #1654, #2703, #16292, #15872, #32497, #15660, #29081, #19067, #16077, #32073, #9702, #19488, #19280, #38686, #2909, #28879, #12689, #12484, #31863, #41891, #25479, #9492, #38474, #25679, #22253, #29296, #3325, #22457, #28664, #9907, #35702, #139, #35486, #6513, #13106, #9292, #41676, #6308, #39104, #35279, #6104, #26098, #32288, #35076, #3117, #42100, #12895, #25883, #38890, #22669, #22879, #35917, #22048, #5897, #18859, #5395, #37539, #38184, #2413, #34776, #9001, #5188, #1776, #8362, #21329, #11973, #22169, #14737, #21749, #21968, #37751, #31145, #12190, #27740, #41596, #28164, #18141, #1986, #18351, #31357, #24966, #5610, #25398, #14948, #34998, #35200, #11763, #8791, #41169, #28378, #38400, #27948, #37966, #40750, #18566, #31573, #9212, #11547, #15373, #5818, #15583, #31784, #40957, #41385, #2200, #24530, #25184, #17934, #18774, #34568, #24752, #15158, #2624, #8575, #28588, #34356, #21538, #12406, #30937, #35618, #264, #26222, #35401, #22794, #9409, #12608, #9618, #39226, #23215, #22586, #10036, #26437, #19199, #23008, #476, #3243, #6432, #29207, #15790, #35829, #12810, #19406, #15998, #32413, #6645, #38806, #29639, #22375, #26010, #13238, #10244, #16202, #25595 ),
 ( #28997, #39441, #50, #18988, #39019, #19820, #36036, #13016, #19609, #3455, #6851, #32837, #9827, #28798, #32207, #32622, #6228, #38603, #3040, #13449, #31992, #25800, #3666, #42014, #16417, #41812, #29423, #16632, #6026, #2830, #30260, #33476, #36458, #27072, #17053, #10875, #36882, #29847, #40295, #40500, #40080, #33052, #23863, #11088, #13867, #7277, #30469, #14270, #11296, #26861, #7700, #20661, #36668, #1101, #20239, #33687, #3882, #33265, #30677, #16847, #4094, #7489, #4511, #36248, #20869, #17472, #4306, #7069, #685, #30055, #893, #1314, #4723, #37087, #13657, #39869, #10665, #23646, #20449, #17269, #14068, #33893, #26647, #27281, #39655, #24075, #7905, #17676, #1525, #14481, #27492, #20033, #10459, #23429, #10927, #4779, #17107, #37340, #11350, #17321, #4361, #26911, #7957, #8159, #27747, #1580, #11140, #14323, #30311, #20925, #40135, #33948, #17729, #10717, #21128, #21335, #30731, #13918, #949, #40757, #27334, #1155, #14120, #17524, #30524, #24126, #14537, #24538, #27120, #34157, #34362, #23916, #27546, #40346, #40552, #37546, #36932, #37136, #39924, #24336, #4984, #8369, #23698, #17942, #30944, #14745, #1784, #7751, #11554, #4565, #36718, #30109, #7540, #20501, #33741, #20717, #1364, #33528, #28171, #15795, #1992, #18357, #15588, #12614, #34783, #41602, #25404, #34574, #21972, #9007, #14954, #31363, #5616, #5400, #24758, #41175, #35004, #5194, #38406, #12411, #2206, #15164, #27955, #38190, #9217, #28803, #31790, #41391, #2419, #11979, #5823, #24973, #18779, #2629, #40963, #22174, #9415, #28593 ),
 ( #18572, #31580, #12196, #35205, #25601, #37972, #6031, #22382, #8797, #18993, #15379, #31997, #38609, #21755, #28385, #31151, #2836, #41820, #18148, #11768, #25188, #37757, #8581, #21544, #19412, #270, #22800, #16004, #39232, #13663, #39447, #9833, #32419, #35835, #29645, #16209, #3889, #32213, #6438, #3673, #690, #6651, #483, #13456, #22592, #10041, #38811, #42020, #39025, #26443, #10466, #19615, #10250, #26655, #3249, #23223, #29853, #32628, #3461, #16425, #3046, #23014, #56, #29429, #29213, #13244, #36042, #26016, #16853, #9625, #26228, #36255, #39662, #6857, #12817, #13024, #19828, #32843, #7076, #35407, #29003, #16637, #6235, #20039, #19205, #33058, #25805, #35624, #33693, #40302, #20876, #1532, #24287, #40708, #17277, #14277, #4517, #33901, #1737, #20455, #17479, #7284, #11095, #27287, #14695, #17059, #30476, #11302, #21084, #37292, #7495, #1320, #10882, #4100, #24082, #27701, #27500, #40086, #33483, #23869, #17682, #4313, #34109, #20245, #36674, #4730, #30897, #36889, #30683, #14487, #10672, #37093, #26867, #30063, #27078, #40507, #23435, #7706, #8110, #36464, #30266, #4936, #17895, #20669, #7911, #33271, #900, #13874, #1107, #39875, #14075, #23653, #12143, #2152, #35153, #27906, #31523, #18727, #15744, #21704, #18102, #37711, #15112, #24922, #28543, #5979, #8320, #34527, #2787, #28115, #24490, #2367, #25347, #5773, #34729, #28332, #8953, #31737, #12359, #15325, #21291, #24706, #11930, #40913, #31106, #5352, #41341, #11504, #2581, #15542, #11719, #8534, #34319, #25135, #41551, #22123, #38138, #5560 ) ),
 .UNSPECIFIED., .T., .F., .F. ) 
 B_SPLINE_SURFACE_WITH_KNOTS ( ( 4, 3, 4 ),
 ( 4, 1, 1, 1, 1, 1, 1, 1, 1, 1, 1, 1, 1, 1, 1, 1, 1, 1, 1, 1, 1, 1, 1, 1, 1, 1, 1, 1, 1, 1, 1, 1, 1, 1, 1, 1, 1, 1, 1, 1, 1, 1, 1, 1, 1, 1, 1, 1, 1, 1, 1, 1, 1, 1, 1, 1, 1, 1, 1, 1, 1, 1, 1, 1, 1, 1, 1, 1, 1, 1, 1, 1, 1, 1, 1, 1, 1, 1, 1, 1, 1, 1, 1, 1, 1, 1, 1, 1, 1, 1, 1, 1, 1, 1, 1, 1, 1, 1, 1, 1, 1, 1, 1, 1, 1, 1, 1, 1, 1, 1, 1, 1, 1, 1, 1, 1, 1, 1, 1, 1, 1, 1, 1, 1, 1, 1, 1, 1, 1, 1, 1, 1, 1, 1, 1, 1, 1, 1, 1, 1, 1, 1, 1, 1, 1, 1, 1, 1, 1, 1, 1, 1, 1, 1, 1, 1, 1, 1, 1, 1, 1, 1, 1, 1, 1, 1, 1, 1, 1, 1, 1, 1, 1, 1, 1, 1, 1, 1, 1, 1, 1, 1, 1, 1, 1, 1, 1, 1, 1, 1, 1, 1, 3, 4 ),
 ( 0.000000000000000000, 0.5000000000000000000, 1.000000000000000000 ),
 ( 0.000000000000000000, 0.007812500000000423273, 0.01388888888888889506, 0.01562500000000000000, 0.02343749999999998959, 0.02777777777777778317, 0.03125000000000092981, 0.03906249999999999306, 0.04166666666666667823, 0.04687500000000000000, 0.05468749999999999306, 0.05555555555555556635, 0.06249999999999997918, 0.06944444444444446141, 0.07031250000000000000, 0.07812500000000000000, 0.08333333333333334259, 0.08593749999999998612, 0.09374999999999603095, 0.09722222222222223764, 0.1015625000000000139, 0.1093750000000000000, 0.1111111111111111188, 0.1171875000000000000, 0.1250000000000000000, 0.1328125000000000000, 0.1388888888888889228, 0.1406250000000000000, 0.1484375000000000000, 0.1527777777777778179, 0.1562500000000039690, 0.1640625000000000000, 0.1666666666666666852, 0.1718750000000000000, 0.1796875000000000000, 0.1805555555555555802, 0.1875000000000000000, 0.1944444444444444753, 0.1953125000000000000, 0.2031250000000000000, 0.2083333333333333703, 0.2109375000000000000, 0.2187499999999960310, 0.2222222222222222376, 0.2265625000000000000, 0.2343750000000000000, 0.2361111111111111327, 0.2421875000000000000, 0.2500000000000000000, 0.2578125000000000000, 0.2638888888888888951, 0.2656250000000000000, 0.2734375000000000000, 0.2777777777777777346, 0.2812500000000039968, 0.2890625000000000000, 0.2916666666666665741, 0.2968750000000000000, 0.3046875000000000000, 0.3055555555555554692, 0.3125000000000000000, 0.3194444444444443088, 0.3203125000000000000, 0.3281250000000000000, 0.3333333333333332038, 0.3359375000000000000, 0.3437499999999960587, 0.3472222222222220434, 0.3515625000000000000, 0.3593750000000000000, 0.3611111111111109384, 0.3671875000000000000, 0.3750000000000000000, 0.3828125000000000000, 0.3888888888888886175, 0.3906250000000000000, 0.3984375000000000000, 0.4027777777777775126, 0.4062500000000039968, 0.4140625000000000000, 0.4166666666666663521, 0.4218750000000000000, 0.4296875000000000000, 0.4305555555555552472, 0.4375000000000000000, 0.4444444444444440867, 0.4453125000000000000, 0.4531250000000000000, 0.4583333333333329818, 0.4609375000000000000, 0.4687499999999960587, 0.4722222222222218768, 0.4765625000000000000, 0.4843750000000000000, 0.4861111111111107719, 0.4921875000000000000, 0.5000000000000000000, 0.5078125000000000000, 0.5138888888888886175, 0.5156250000000000000, 0.5234375000000000000, 0.5277777777777775681, 0.5312500000000039968, 0.5390625000000000000, 0.5416666666666664076, 0.5468750000000000000, 0.5546875000000000000, 0.5555555555555553582, 0.5625000000000000000, 0.5694444444444443088, 0.5703125000000000000, 0.5781250000000000000, 0.5833333333333331483, 0.5859375000000000000, 0.5937499999999960032, 0.5972222222222220989, 0.6015625000000000000, 0.6093750000000000000, 0.6111111111111110494, 0.6171875000000000000, 0.6250000000000000000, 0.6328125000000000000, 0.6388888888888888395, 0.6406250000000000000, 0.6484375000000000000, 0.6527777777777777901, 0.6562500000000039968, 0.6640625000000000000, 0.6666666666666666297, 0.6718750000000000000, 0.6796875000000000000, 0.6805555555555555802, 0.6875000000000000000, 0.6944444444444445308, 0.6953125000000000000, 0.7031250000000000000, 0.7083333333333333703, 0.7109375000000000000, 0.7187499999999960032, 0.7222222222222223209, 0.7265625000000000000, 0.7343750000000000000, 0.7361111111111111605, 0.7421875000000000000, 0.7500000000000000000, 0.7578125000000000000, 0.7638888888888889506, 0.7656250000000000000, 0.7734375000000000000, 0.7777777777777779011, 0.7812500000000039968, 0.7890625000000000000, 0.7916666666666668517, 0.7968750000000000000, 0.8046875000000000000, 0.8055555555555556912, 0.8125000000000000000, 0.8194444444444446418, 0.8203125000000000000, 0.8281250000000000000, 0.8333333333333335924, 0.8359375000000000000, 0.8437499999999960032, 0.8472222222222224319, 0.8515625000000000000, 0.8593750000000000000, 0.8611111111111113825, 0.8671875000000000000, 0.8750000000000000000, 0.8828125000000000000, 0.8888888888888891726, 0.8906250000000000000, 0.8984375000000000000, 0.9027777777777781232, 0.9062500000000039968, 0.9140625000000000000, 0.9166666666666670737, 0.9218750000000000000, 0.9296875000000000000, 0.9305555555555559133, 0.9375000000000000000, 0.9444444444444447528, 0.9453125000000000000, 0.9531250000000000000, 0.9583333333333335924, 0.9609375000000000000, 0.9687499999999991118, 0.9722222222222224319, 0.9765625000000000000, 0.9843750000000000000, 0.9861111111111111605, 0.9921874999999995559, 1.000000000000000000, 1.000012325855852646 ),
 .UNSPECIFIED. ) 
 GEOMETRIC_REPRESENTATION_ITEM ( )  RATIONAL_B_SPLINE_SURFACE ( (
 ( 1.000000000000000000, 1.000000000000000000, 1.000000000000000000, 1.000000000000000000, 1.000000000000000000, 1.000000000000000000, 0.9999999999999998890, 0.9999999999999997780, 1.000000000000000000, 1.000000000000000000, 1.000000000000000000, 1.000000000000000000, 1.000000000000000000, 1.000000000000000000, 0.9999999999999998890, 1.000000000000000000, 1.000000000000000222, 1.000000000000000000, 1.000000000000000000, 1.000000000000000000, 1.000000000000000000, 1.000000000000000000, 0.9999999999999998890, 0.9999999999999997780, 1.000000000000000000, 1.000000000000000222, 1.000000000000000000, 1.000000000000000000, 1.000000000000000000, 1.000000000000000000, 0.9999999999999998890, 0.9999999999999997780, 1.000000000000000000, 0.9999999999999998890, 0.9999999999999997780, 1.000000000000000000, 1.000000000000000222, 1.000000000000000222, 1.000000000000000000, 1.000000000000000000, 1.000000000000000222, 1.000000000000000000, 0.9999999999999997780, 1.000000000000000000, 1.000000000000000000, 1.000000000000000000, 1.000000000000000000, 1.000000000000000000, 1.000000000000000000, 1.000000000000000222, 1.000000000000000222, 1.000000000000000000, 1.000000000000000000, 1.000000000000000222, 1.000000000000000222, 1.000000000000000222, 1.000000000000000000, 1.000000000000000000, 1.000000000000000222, 1.000000000000000000, 1.000000000000000000, 1.000000000000000222, 1.000000000000000000, 1.000000000000000000, 1.000000000000000222, 1.000000000000000000, 1.000000000000000000, 0.9999999999999997780, 0.9999999999999998890, 1.000000000000000000, 1.000000000000000000, 1.000000000000000000, 1.000000000000000000, 1.000000000000000222, 1.000000000000000222, 1.000000000000000000, 1.000000000000000000, 1.000000000000000222, 1.000000000000000222, 1.000000000000000222, 1.000000000000000000, 1.000000000000000000, 1.000000000000000222, 1.000000000000000000, 1.000000000000000000, 1.000000000000000222, 1.000000000000000000, 1.000000000000000000, 1.000000000000000222, 1.000000000000000000, 1.000000000000000000, 0.9999999999999997780, 0.9999999999999998890, 1.000000000000000000, 1.000000000000000000, 1.000000000000000000, 1.000000000000000000, 1.000000000000000222, 1.000000000000000222, 1.000000000000000000, 1.000000000000000000, 1.000000000000000222, 1.000000000000000222, 1.000000000000000222, 1.000000000000000000, 1.000000000000000000, 1.000000000000000222, 1.000000000000000000, 0.9999999999999998890, 1.000000000000000222, 1.000000000000000000, 1.000000000000000000, 1.000000000000000222, 1.000000000000000000, 1.000000000000000000, 1.000000000000000222, 1.000000000000000000, 1.000000000000000000, 1.000000000000000000, 1.000000000000000000, 1.000000000000000000, 1.000000000000000222, 1.000000000000000222, 1.000000000000000000, 1.000000000000000000, 1.000000000000000222, 1.000000000000000222, 1.000000000000000222, 1.000000000000000000, 1.000000000000000222, 1.000000000000000222, 1.000000000000000000, 1.000000000000000000, 1.000000000000000222, 1.000000000000000000, 1.000000000000000000, 1.000000000000000222, 1.000000000000000000, 1.000000000000000000, 1.000000000000000222, 1.000000000000000222, 1.000000000000000000, 1.000000000000000000, 1.000000000000000222, 1.000000000000000000, 1.000000000000000222, 1.000000000000000222, 1.000000000000000000, 1.000000000000000000, 1.000000000000000222, 1.000000000000000222, 1.000000000000000222, 1.000000000000000000, 1.000000000000000000, 1.000000000000000222, 1.000000000000000000, 0.9999999999999998890, 1.000000000000000222, 1.000000000000000000, 1.000000000000000000, 1.000000000000000222, 1.000000000000000000, 1.000000000000000000, 1.000000000000000222, 1.000000000000000000, 1.000000000000000000, 1.000000000000000000, 1.000000000000000000, 1.000000000000000000, 1.000000000000000222, 1.000000000000000222, 1.000000000000000000, 1.000000000000000000, 1.000000000000000222, 1.000000000000000222, 1.000000000000000222, 1.000000000000000000, 1.000000000000000000, 1.000000000000000222, 1.000000000000000000, 1.000000000000000000, 1.000000000000000222, 1.000000000000000000, 1.000000000000000000, 1.000000000000000222, 1.000000000000000000, 0.9999999999999996669, 0.9999999999999996669, 1.000000000000000000, 1.000000000000000222, 1.000000000000000000, 1.000000000000000000, 1.000000000000000000, 1.000000000000000000, 1.000000000000000000, 1.000000000000000000, 1.000000000000000000, 1.000000000000000000),
 ( 0.3333333333333333703, 0.3333333333333333703, 0.3333333333333333703, 0.3333333333333334259, 0.3333333333333334259, 0.3333333333333334259, 0.3333333333333333703, 0.3333333333333333148, 0.3333333333333333703, 0.3333333333333333703, 0.3333333333333333148, 0.3333333333333333703, 0.3333333333333333703, 0.3333333333333334814, 0.3333333333333333703, 0.3333333333333333703, 0.3333333333333334259, 0.3333333333333333703, 0.3333333333333333148, 0.3333333333333333703, 0.3333333333333333703, 0.3333333333333333703, 0.3333333333333333703, 0.3333333333333333703, 0.3333333333333333148, 0.3333333333333334259, 0.3333333333333333703, 0.3333333333333333703, 0.3333333333333333703, 0.3333333333333334259, 0.3333333333333333703, 0.3333333333333333703, 0.3333333333333333703, 0.3333333333333333703, 0.3333333333333333148, 0.3333333333333333703, 0.3333333333333334259, 0.3333333333333333703, 0.3333333333333333703, 0.3333333333333333703, 0.3333333333333333703, 0.3333333333333333703, 0.3333333333333333703, 0.3333333333333333703, 0.3333333333333333703, 0.3333333333333333148, 0.3333333333333333703, 0.3333333333333333703, 0.3333333333333333703, 0.3333333333333334259, 0.3333333333333333703, 0.3333333333333333703, 0.3333333333333333703, 0.3333333333333333703, 0.3333333333333333703, 0.3333333333333334259, 0.3333333333333333703, 0.3333333333333333703, 0.3333333333333333703, 0.3333333333333333703, 0.3333333333333334259, 0.3333333333333333703, 0.3333333333333333703, 0.3333333333333333703, 0.3333333333333333703, 0.3333333333333333703, 0.3333333333333333703, 0.3333333333333333148, 0.3333333333333333148, 0.3333333333333333148, 0.3333333333333333703, 0.3333333333333333703, 0.3333333333333333148, 0.3333333333333334259, 0.3333333333333333703, 0.3333333333333333703, 0.3333333333333333703, 0.3333333333333333703, 0.3333333333333333703, 0.3333333333333333703, 0.3333333333333333703, 0.3333333333333333703, 0.3333333333333333703, 0.3333333333333334259, 0.3333333333333334259, 0.3333333333333333703, 0.3333333333333333703, 0.3333333333333333703, 0.3333333333333333703, 0.3333333333333333703, 0.3333333333333333703, 0.3333333333333333703, 0.3333333333333333148, 0.3333333333333333148, 0.3333333333333333703, 0.3333333333333333703, 0.3333333333333333148, 0.3333333333333334259, 0.3333333333333333703, 0.3333333333333333703, 0.3333333333333333703, 0.3333333333333333703, 0.3333333333333333703, 0.3333333333333333703, 0.3333333333333333703, 0.3333333333333333703, 0.3333333333333333703, 0.3333333333333333703, 0.3333333333333333703, 0.3333333333333333148, 0.3333333333333333703, 0.3333333333333333703, 0.3333333333333333703, 0.3333333333333333703, 0.3333333333333333148, 0.3333333333333333703, 0.3333333333333333703, 0.3333333333333333148, 0.3333333333333333703, 0.3333333333333333703, 0.3333333333333333148, 0.3333333333333334259, 0.3333333333333333703, 0.3333333333333333703, 0.3333333333333333703, 0.3333333333333333703, 0.3333333333333333703, 0.3333333333333334259, 0.3333333333333333703, 0.3333333333333333703, 0.3333333333333334259, 0.3333333333333334259, 0.3333333333333334259, 0.3333333333333333703, 0.3333333333333333703, 0.3333333333333333703, 0.3333333333333333703, 0.3333333333333333703, 0.3333333333333333703, 0.3333333333333333703, 0.3333333333333333703, 0.3333333333333333703, 0.3333333333333334259, 0.3333333333333333703, 0.3333333333333333148, 0.3333333333333334259, 0.3333333333333333703, 0.3333333333333333703, 0.3333333333333333703, 0.3333333333333333703, 0.3333333333333333703, 0.3333333333333334259, 0.3333333333333333703, 0.3333333333333333703, 0.3333333333333333703, 0.3333333333333334259, 0.3333333333333333703, 0.3333333333333333703, 0.3333333333333333703, 0.3333333333333333703, 0.3333333333333333703, 0.3333333333333333703, 0.3333333333333333148, 0.3333333333333334259, 0.3333333333333333703, 0.3333333333333333148, 0.3333333333333333703, 0.3333333333333333703, 0.3333333333333333703, 0.3333333333333334259, 0.3333333333333333703, 0.3333333333333333703, 0.3333333333333333703, 0.3333333333333333703, 0.3333333333333333703, 0.3333333333333334259, 0.3333333333333333703, 0.3333333333333333703, 0.3333333333333333703, 0.3333333333333333703, 0.3333333333333334259, 0.3333333333333333703, 0.3333333333333333703, 0.3333333333333333703, 0.3333333333333333703, 0.3333333333333333703, 0.3333333333333333703, 0.3333333333333333148, 0.3333333333333333703, 0.3333333333333333703, 0.3333333333333333703, 0.3333333333333333703, 0.3333333333333333148, 0.3333333333333333703, 0.3333333333333333703, 0.3333333333333333703, 0.3333333333333333703, 0.3333333333333333703),
 ( 0.3333333333333333703, 0.3333333333333333703, 0.3333333333333333703, 0.3333333333333334259, 0.3333333333333334259, 0.3333333333333334259, 0.3333333333333333703, 0.3333333333333333148, 0.3333333333333333703, 0.3333333333333333703, 0.3333333333333333148, 0.3333333333333333703, 0.3333333333333333703, 0.3333333333333334814, 0.3333333333333333703, 0.3333333333333333703, 0.3333333333333334259, 0.3333333333333333703, 0.3333333333333333148, 0.3333333333333333703, 0.3333333333333333703, 0.3333333333333333703, 0.3333333333333333703, 0.3333333333333333703, 0.3333333333333333148, 0.3333333333333334259, 0.3333333333333333703, 0.3333333333333333703, 0.3333333333333333703, 0.3333333333333334259, 0.3333333333333333703, 0.3333333333333333703, 0.3333333333333333703, 0.3333333333333333703, 0.3333333333333333148, 0.3333333333333333703, 0.3333333333333334259, 0.3333333333333333703, 0.3333333333333333703, 0.3333333333333333703, 0.3333333333333333703, 0.3333333333333333703, 0.3333333333333333703, 0.3333333333333333703, 0.3333333333333333703, 0.3333333333333333148, 0.3333333333333333703, 0.3333333333333333703, 0.3333333333333333703, 0.3333333333333334259, 0.3333333333333333703, 0.3333333333333333703, 0.3333333333333333703, 0.3333333333333333703, 0.3333333333333333703, 0.3333333333333334259, 0.3333333333333333703, 0.3333333333333333703, 0.3333333333333333703, 0.3333333333333333703, 0.3333333333333334259, 0.3333333333333333703, 0.3333333333333333703, 0.3333333333333333703, 0.3333333333333333703, 0.3333333333333333703, 0.3333333333333333703, 0.3333333333333333148, 0.3333333333333333148, 0.3333333333333333148, 0.3333333333333333703, 0.3333333333333333703, 0.3333333333333333148, 0.3333333333333334259, 0.3333333333333333703, 0.3333333333333333703, 0.3333333333333333703, 0.3333333333333333703, 0.3333333333333333703, 0.3333333333333333703, 0.3333333333333333703, 0.3333333333333333703, 0.3333333333333333703, 0.3333333333333334259, 0.3333333333333334259, 0.3333333333333333703, 0.3333333333333333703, 0.3333333333333333703, 0.3333333333333333703, 0.3333333333333333703, 0.3333333333333333703, 0.3333333333333333703, 0.3333333333333333148, 0.3333333333333333148, 0.3333333333333333703, 0.3333333333333333703, 0.3333333333333333148, 0.3333333333333334259, 0.3333333333333333703, 0.3333333333333333703, 0.3333333333333333703, 0.3333333333333333703, 0.3333333333333333703, 0.3333333333333333703, 0.3333333333333333703, 0.3333333333333333703, 0.3333333333333333703, 0.3333333333333333703, 0.3333333333333333703, 0.3333333333333333148, 0.3333333333333333703, 0.3333333333333333703, 0.3333333333333333703, 0.3333333333333333703, 0.3333333333333333148, 0.3333333333333333703, 0.3333333333333333703, 0.3333333333333333148, 0.3333333333333333703, 0.3333333333333333703, 0.3333333333333333148, 0.3333333333333334259, 0.3333333333333333703, 0.3333333333333333703, 0.3333333333333333703, 0.3333333333333333703, 0.3333333333333333703, 0.3333333333333334259, 0.3333333333333333703, 0.3333333333333333703, 0.3333333333333334259, 0.3333333333333334259, 0.3333333333333334259, 0.3333333333333333703, 0.3333333333333333703, 0.3333333333333333703, 0.3333333333333333703, 0.3333333333333333703, 0.3333333333333333703, 0.3333333333333333703, 0.3333333333333333703, 0.3333333333333333703, 0.3333333333333334259, 0.3333333333333333703, 0.3333333333333333148, 0.3333333333333334259, 0.3333333333333333703, 0.3333333333333333703, 0.3333333333333333703, 0.3333333333333333703, 0.3333333333333333703, 0.3333333333333334259, 0.3333333333333333703, 0.3333333333333333703, 0.3333333333333333703, 0.3333333333333334259, 0.3333333333333333703, 0.3333333333333333703, 0.3333333333333333703, 0.3333333333333333703, 0.3333333333333333703, 0.3333333333333333703, 0.3333333333333333148, 0.3333333333333334259, 0.3333333333333333703, 0.3333333333333333148, 0.3333333333333333703, 0.3333333333333333703, 0.3333333333333333703, 0.3333333333333334259, 0.3333333333333333703, 0.3333333333333333703, 0.3333333333333333703, 0.3333333333333333703, 0.3333333333333333703, 0.3333333333333334259, 0.3333333333333333703, 0.3333333333333333703, 0.3333333333333333703, 0.3333333333333333703, 0.3333333333333334259, 0.3333333333333333703, 0.3333333333333333703, 0.3333333333333333703, 0.3333333333333333703, 0.3333333333333333703, 0.3333333333333333703, 0.3333333333333333148, 0.3333333333333333703, 0.3333333333333333703, 0.3333333333333333703, 0.3333333333333333703, 0.3333333333333333148, 0.3333333333333333703, 0.3333333333333333703, 0.3333333333333333703, 0.3333333333333333703, 0.3333333333333333703),
 ( 1.000000000000000000, 1.000000000000000000, 1.000000000000000000, 1.000000000000000000, 1.000000000000000000, 1.000000000000000000, 0.9999999999999998890, 0.9999999999999997780, 1.000000000000000000, 1.000000000000000000, 1.000000000000000000, 1.000000000000000000, 1.000000000000000000, 1.000000000000000000, 0.9999999999999998890, 1.000000000000000000, 1.000000000000000222, 1.000000000000000000, 1.000000000000000000, 1.000000000000000000, 1.000000000000000000, 1.000000000000000000, 0.9999999999999998890, 0.9999999999999997780, 1.000000000000000000, 1.000000000000000222, 1.000000000000000000, 1.000000000000000000, 1.000000000000000000, 1.000000000000000000, 0.9999999999999998890, 0.9999999999999997780, 1.000000000000000000, 0.9999999999999998890, 0.9999999999999997780, 1.000000000000000000, 1.000000000000000222, 1.000000000000000222, 1.000000000000000000, 1.000000000000000000, 1.000000000000000222, 1.000000000000000000, 0.9999999999999997780, 1.000000000000000000, 1.000000000000000000, 1.000000000000000000, 1.000000000000000000, 1.000000000000000000, 1.000000000000000000, 1.000000000000000222, 1.000000000000000222, 1.000000000000000000, 1.000000000000000000, 1.000000000000000222, 1.000000000000000222, 1.000000000000000222, 1.000000000000000000, 1.000000000000000000, 1.000000000000000222, 1.000000000000000000, 1.000000000000000000, 1.000000000000000222, 1.000000000000000000, 1.000000000000000000, 1.000000000000000222, 1.000000000000000000, 1.000000000000000000, 0.9999999999999997780, 0.9999999999999998890, 1.000000000000000000, 1.000000000000000000, 1.000000000000000000, 1.000000000000000000, 1.000000000000000222, 1.000000000000000222, 1.000000000000000000, 1.000000000000000000, 1.000000000000000222, 1.000000000000000222, 1.000000000000000222, 1.000000000000000000, 1.000000000000000000, 1.000000000000000222, 1.000000000000000000, 1.000000000000000000, 1.000000000000000222, 1.000000000000000000, 1.000000000000000000, 1.000000000000000222, 1.000000000000000000, 1.000000000000000000, 0.9999999999999997780, 0.9999999999999998890, 1.000000000000000000, 1.000000000000000000, 1.000000000000000000, 1.000000000000000000, 1.000000000000000222, 1.000000000000000222, 1.000000000000000000, 1.000000000000000000, 1.000000000000000222, 1.000000000000000222, 1.000000000000000222, 1.000000000000000000, 1.000000000000000000, 1.000000000000000222, 1.000000000000000000, 0.9999999999999998890, 1.000000000000000222, 1.000000000000000000, 1.000000000000000000, 1.000000000000000222, 1.000000000000000000, 1.000000000000000000, 1.000000000000000222, 1.000000000000000000, 1.000000000000000000, 1.000000000000000000, 1.000000000000000000, 1.000000000000000000, 1.000000000000000222, 1.000000000000000222, 1.000000000000000000, 1.000000000000000000, 1.000000000000000222, 1.000000000000000222, 1.000000000000000222, 1.000000000000000000, 1.000000000000000222, 1.000000000000000222, 1.000000000000000000, 1.000000000000000000, 1.000000000000000222, 1.000000000000000000, 1.000000000000000000, 1.000000000000000222, 1.000000000000000000, 1.000000000000000000, 1.000000000000000222, 1.000000000000000222, 1.000000000000000000, 1.000000000000000000, 1.000000000000000222, 1.000000000000000000, 1.000000000000000222, 1.000000000000000222, 1.000000000000000000, 1.000000000000000000, 1.000000000000000222, 1.000000000000000222, 1.000000000000000222, 1.000000000000000000, 1.000000000000000000, 1.000000000000000222, 1.000000000000000000, 0.9999999999999998890, 1.000000000000000222, 1.000000000000000000, 1.000000000000000000, 1.000000000000000222, 1.000000000000000000, 1.000000000000000000, 1.000000000000000222, 1.000000000000000000, 1.000000000000000000, 1.000000000000000000, 1.000000000000000000, 1.000000000000000000, 1.000000000000000222, 1.000000000000000222, 1.000000000000000000, 1.000000000000000000, 1.000000000000000222, 1.000000000000000222, 1.000000000000000222, 1.000000000000000000, 1.000000000000000000, 1.000000000000000222, 1.000000000000000000, 1.000000000000000000, 1.000000000000000222, 1.000000000000000000, 1.000000000000000000, 1.000000000000000222, 1.000000000000000000, 0.9999999999999996669, 0.9999999999999996669, 1.000000000000000000, 1.000000000000000222, 1.000000000000000000, 1.000000000000000000, 1.000000000000000000, 1.000000000000000000, 1.000000000000000000, 1.000000000000000000, 1.000000000000000000, 1.000000000000000000),
 ( 0.3333333333333333703, 0.3333333333333333703, 0.3333333333333333703, 0.3333333333333334259, 0.3333333333333334259, 0.3333333333333334259, 0.3333333333333333703, 0.3333333333333333148, 0.3333333333333333703, 0.3333333333333333703, 0.3333333333333333148, 0.3333333333333333703, 0.3333333333333333703, 0.3333333333333334814, 0.3333333333333333703, 0.3333333333333333703, 0.3333333333333334259, 0.3333333333333333703, 0.3333333333333333148, 0.3333333333333333703, 0.3333333333333333703, 0.3333333333333333703, 0.3333333333333333703, 0.3333333333333333703, 0.3333333333333333148, 0.3333333333333334259, 0.3333333333333333703, 0.3333333333333333703, 0.3333333333333333703, 0.3333333333333334259, 0.3333333333333333703, 0.3333333333333333703, 0.3333333333333333703, 0.3333333333333333703, 0.3333333333333333148, 0.3333333333333333703, 0.3333333333333334259, 0.3333333333333333703, 0.3333333333333333703, 0.3333333333333333703, 0.3333333333333333703, 0.3333333333333333703, 0.3333333333333333703, 0.3333333333333333703, 0.3333333333333333703, 0.3333333333333333148, 0.3333333333333333703, 0.3333333333333333703, 0.3333333333333333703, 0.3333333333333334259, 0.3333333333333333703, 0.3333333333333333703, 0.3333333333333333703, 0.3333333333333333703, 0.3333333333333333703, 0.3333333333333334259, 0.3333333333333333703, 0.3333333333333333703, 0.3333333333333333703, 0.3333333333333333703, 0.3333333333333334259, 0.3333333333333333703, 0.3333333333333333703, 0.3333333333333333703, 0.3333333333333333703, 0.3333333333333333703, 0.3333333333333333703, 0.3333333333333333148, 0.3333333333333333148, 0.3333333333333333148, 0.3333333333333333703, 0.3333333333333333703, 0.3333333333333333148, 0.3333333333333334259, 0.3333333333333333703, 0.3333333333333333703, 0.3333333333333333703, 0.3333333333333333703, 0.3333333333333333703, 0.3333333333333333703, 0.3333333333333333703, 0.3333333333333333703, 0.3333333333333333703, 0.3333333333333334259, 0.3333333333333334259, 0.3333333333333333703, 0.3333333333333333703, 0.3333333333333333703, 0.3333333333333333703, 0.3333333333333333703, 0.3333333333333333703, 0.3333333333333333703, 0.3333333333333333148, 0.3333333333333333148, 0.3333333333333333703, 0.3333333333333333703, 0.3333333333333333148, 0.3333333333333334259, 0.3333333333333333703, 0.3333333333333333703, 0.3333333333333333703, 0.3333333333333333703, 0.3333333333333333703, 0.3333333333333333703, 0.3333333333333333703, 0.3333333333333333703, 0.3333333333333333703, 0.3333333333333333703, 0.3333333333333333703, 0.3333333333333333148, 0.3333333333333333703, 0.3333333333333333703, 0.3333333333333333703, 0.3333333333333333703, 0.3333333333333333148, 0.3333333333333333703, 0.3333333333333333703, 0.3333333333333333148, 0.3333333333333333703, 0.3333333333333333703, 0.3333333333333333148, 0.3333333333333334259, 0.3333333333333333703, 0.3333333333333333703, 0.3333333333333333703, 0.3333333333333333703, 0.3333333333333333703, 0.3333333333333334259, 0.3333333333333333703, 0.3333333333333333703, 0.3333333333333334259, 0.3333333333333334259, 0.3333333333333334259, 0.3333333333333333703, 0.3333333333333333703, 0.3333333333333333703, 0.3333333333333333703, 0.3333333333333333703, 0.3333333333333333703, 0.3333333333333333703, 0.3333333333333333703, 0.3333333333333333703, 0.3333333333333334259, 0.3333333333333333703, 0.3333333333333333148, 0.3333333333333334259, 0.3333333333333333703, 0.3333333333333333703, 0.3333333333333333703, 0.3333333333333333703, 0.3333333333333333703, 0.3333333333333334259, 0.3333333333333333703, 0.3333333333333333703, 0.3333333333333333703, 0.3333333333333334259, 0.3333333333333333703, 0.3333333333333333703, 0.3333333333333333703, 0.3333333333333333703, 0.3333333333333333703, 0.3333333333333333703, 0.3333333333333333148, 0.3333333333333334259, 0.3333333333333333703, 0.3333333333333333148, 0.3333333333333333703, 0.3333333333333333703, 0.3333333333333333703, 0.3333333333333334259, 0.3333333333333333703, 0.3333333333333333703, 0.3333333333333333703, 0.3333333333333333703, 0.3333333333333333703, 0.3333333333333334259, 0.3333333333333333703, 0.3333333333333333703, 0.3333333333333333703, 0.3333333333333333703, 0.3333333333333334259, 0.3333333333333333703, 0.3333333333333333703, 0.3333333333333333703, 0.3333333333333333703, 0.3333333333333333703, 0.3333333333333333703, 0.3333333333333333148, 0.3333333333333333703, 0.3333333333333333703, 0.3333333333333333703, 0.3333333333333333703, 0.3333333333333333148, 0.3333333333333333703, 0.3333333333333333703, 0.3333333333333333703, 0.3333333333333333703, 0.3333333333333333703),
 ( 0.3333333333333333703, 0.3333333333333333703, 0.3333333333333333703, 0.3333333333333334259, 0.3333333333333334259, 0.3333333333333334259, 0.3333333333333333703, 0.3333333333333333148, 0.3333333333333333703, 0.3333333333333333703, 0.3333333333333333148, 0.3333333333333333703, 0.3333333333333333703, 0.3333333333333334814, 0.3333333333333333703, 0.3333333333333333703, 0.3333333333333334259, 0.3333333333333333703, 0.3333333333333333148, 0.3333333333333333703, 0.3333333333333333703, 0.3333333333333333703, 0.3333333333333333703, 0.3333333333333333703, 0.3333333333333333148, 0.3333333333333334259, 0.3333333333333333703, 0.3333333333333333703, 0.3333333333333333703, 0.3333333333333334259, 0.3333333333333333703, 0.3333333333333333703, 0.3333333333333333703, 0.3333333333333333703, 0.3333333333333333148, 0.3333333333333333703, 0.3333333333333334259, 0.3333333333333333703, 0.3333333333333333703, 0.3333333333333333703, 0.3333333333333333703, 0.3333333333333333703, 0.3333333333333333703, 0.3333333333333333703, 0.3333333333333333703, 0.3333333333333333148, 0.3333333333333333703, 0.3333333333333333703, 0.3333333333333333703, 0.3333333333333334259, 0.3333333333333333703, 0.3333333333333333703, 0.3333333333333333703, 0.3333333333333333703, 0.3333333333333333703, 0.3333333333333334259, 0.3333333333333333703, 0.3333333333333333703, 0.3333333333333333703, 0.3333333333333333703, 0.3333333333333334259, 0.3333333333333333703, 0.3333333333333333703, 0.3333333333333333703, 0.3333333333333333703, 0.3333333333333333703, 0.3333333333333333703, 0.3333333333333333148, 0.3333333333333333148, 0.3333333333333333148, 0.3333333333333333703, 0.3333333333333333703, 0.3333333333333333148, 0.3333333333333334259, 0.3333333333333333703, 0.3333333333333333703, 0.3333333333333333703, 0.3333333333333333703, 0.3333333333333333703, 0.3333333333333333703, 0.3333333333333333703, 0.3333333333333333703, 0.3333333333333333703, 0.3333333333333334259, 0.3333333333333334259, 0.3333333333333333703, 0.3333333333333333703, 0.3333333333333333703, 0.3333333333333333703, 0.3333333333333333703, 0.3333333333333333703, 0.3333333333333333703, 0.3333333333333333148, 0.3333333333333333148, 0.3333333333333333703, 0.3333333333333333703, 0.3333333333333333148, 0.3333333333333334259, 0.3333333333333333703, 0.3333333333333333703, 0.3333333333333333703, 0.3333333333333333703, 0.3333333333333333703, 0.3333333333333333703, 0.3333333333333333703, 0.3333333333333333703, 0.3333333333333333703, 0.3333333333333333703, 0.3333333333333333703, 0.3333333333333333148, 0.3333333333333333703, 0.3333333333333333703, 0.3333333333333333703, 0.3333333333333333703, 0.3333333333333333148, 0.3333333333333333703, 0.3333333333333333703, 0.3333333333333333148, 0.3333333333333333703, 0.3333333333333333703, 0.3333333333333333148, 0.3333333333333334259, 0.3333333333333333703, 0.3333333333333333703, 0.3333333333333333703, 0.3333333333333333703, 0.3333333333333333703, 0.3333333333333334259, 0.3333333333333333703, 0.3333333333333333703, 0.3333333333333334259, 0.3333333333333334259, 0.3333333333333334259, 0.3333333333333333703, 0.3333333333333333703, 0.3333333333333333703, 0.3333333333333333703, 0.3333333333333333703, 0.3333333333333333703, 0.3333333333333333703, 0.3333333333333333703, 0.3333333333333333703, 0.3333333333333334259, 0.3333333333333333703, 0.3333333333333333148, 0.3333333333333334259, 0.3333333333333333703, 0.3333333333333333703, 0.3333333333333333703, 0.3333333333333333703, 0.3333333333333333703, 0.3333333333333334259, 0.3333333333333333703, 0.3333333333333333703, 0.3333333333333333703, 0.3333333333333334259, 0.3333333333333333703, 0.3333333333333333703, 0.3333333333333333703, 0.3333333333333333703, 0.3333333333333333703, 0.3333333333333333703, 0.3333333333333333148, 0.3333333333333334259, 0.3333333333333333703, 0.3333333333333333148, 0.3333333333333333703, 0.3333333333333333703, 0.3333333333333333703, 0.3333333333333334259, 0.3333333333333333703, 0.3333333333333333703, 0.3333333333333333703, 0.3333333333333333703, 0.3333333333333333703, 0.3333333333333334259, 0.3333333333333333703, 0.3333333333333333703, 0.3333333333333333703, 0.3333333333333333703, 0.3333333333333334259, 0.3333333333333333703, 0.3333333333333333703, 0.3333333333333333703, 0.3333333333333333703, 0.3333333333333333703, 0.3333333333333333703, 0.3333333333333333148, 0.3333333333333333703, 0.3333333333333333703, 0.3333333333333333703, 0.3333333333333333703, 0.3333333333333333148, 0.3333333333333333703, 0.3333333333333333703, 0.3333333333333333703, 0.3333333333333333703, 0.3333333333333333703),
 ( 1.000000000000000000, 1.000000000000000000, 1.000000000000000000, 1.000000000000000000, 1.000000000000000000, 1.000000000000000000, 0.9999999999999998890, 0.9999999999999997780, 1.000000000000000000, 1.000000000000000000, 1.000000000000000000, 1.000000000000000000, 1.000000000000000000, 1.000000000000000000, 0.9999999999999998890, 1.000000000000000000, 1.000000000000000222, 1.000000000000000000, 1.000000000000000000, 1.000000000000000000, 1.000000000000000000, 1.000000000000000000, 0.9999999999999998890, 0.9999999999999997780, 1.000000000000000000, 1.000000000000000222, 1.000000000000000000, 1.000000000000000000, 1.000000000000000000, 1.000000000000000000, 0.9999999999999998890, 0.9999999999999997780, 1.000000000000000000, 0.9999999999999998890, 0.9999999999999997780, 1.000000000000000000, 1.000000000000000222, 1.000000000000000222, 1.000000000000000000, 1.000000000000000000, 1.000000000000000222, 1.000000000000000000, 0.9999999999999997780, 1.000000000000000000, 1.000000000000000000, 1.000000000000000000, 1.000000000000000000, 1.000000000000000000, 1.000000000000000000, 1.000000000000000222, 1.000000000000000222, 1.000000000000000000, 1.000000000000000000, 1.000000000000000222, 1.000000000000000222, 1.000000000000000222, 1.000000000000000000, 1.000000000000000000, 1.000000000000000222, 1.000000000000000000, 1.000000000000000000, 1.000000000000000222, 1.000000000000000000, 1.000000000000000000, 1.000000000000000222, 1.000000000000000000, 1.000000000000000000, 0.9999999999999997780, 0.9999999999999998890, 1.000000000000000000, 1.000000000000000000, 1.000000000000000000, 1.000000000000000000, 1.000000000000000222, 1.000000000000000222, 1.000000000000000000, 1.000000000000000000, 1.000000000000000222, 1.000000000000000222, 1.000000000000000222, 1.000000000000000000, 1.000000000000000000, 1.000000000000000222, 1.000000000000000000, 1.000000000000000000, 1.000000000000000222, 1.000000000000000000, 1.000000000000000000, 1.000000000000000222, 1.000000000000000000, 1.000000000000000000, 0.9999999999999997780, 0.9999999999999998890, 1.000000000000000000, 1.000000000000000000, 1.000000000000000000, 1.000000000000000000, 1.000000000000000222, 1.000000000000000222, 1.000000000000000000, 1.000000000000000000, 1.000000000000000222, 1.000000000000000222, 1.000000000000000222, 1.000000000000000000, 1.000000000000000000, 1.000000000000000222, 1.000000000000000000, 0.9999999999999998890, 1.000000000000000222, 1.000000000000000000, 1.000000000000000000, 1.000000000000000222, 1.000000000000000000, 1.000000000000000000, 1.000000000000000222, 1.000000000000000000, 1.000000000000000000, 1.000000000000000000, 1.000000000000000000, 1.000000000000000000, 1.000000000000000222, 1.000000000000000222, 1.000000000000000000, 1.000000000000000000, 1.000000000000000222, 1.000000000000000222, 1.000000000000000222, 1.000000000000000000, 1.000000000000000222, 1.000000000000000222, 1.000000000000000000, 1.000000000000000000, 1.000000000000000222, 1.000000000000000000, 1.000000000000000000, 1.000000000000000222, 1.000000000000000000, 1.000000000000000000, 1.000000000000000222, 1.000000000000000222, 1.000000000000000000, 1.000000000000000000, 1.000000000000000222, 1.000000000000000000, 1.000000000000000222, 1.000000000000000222, 1.000000000000000000, 1.000000000000000000, 1.000000000000000222, 1.000000000000000222, 1.000000000000000222, 1.000000000000000000, 1.000000000000000000, 1.000000000000000222, 1.000000000000000000, 0.9999999999999998890, 1.000000000000000222, 1.000000000000000000, 1.000000000000000000, 1.000000000000000222, 1.000000000000000000, 1.000000000000000000, 1.000000000000000222, 1.000000000000000000, 1.000000000000000000, 1.000000000000000000, 1.000000000000000000, 1.000000000000000000, 1.000000000000000222, 1.000000000000000222, 1.000000000000000000, 1.000000000000000000, 1.000000000000000222, 1.000000000000000222, 1.000000000000000222, 1.000000000000000000, 1.000000000000000000, 1.000000000000000222, 1.000000000000000000, 1.000000000000000000, 1.000000000000000222, 1.000000000000000000, 1.000000000000000000, 1.000000000000000222, 1.000000000000000000, 0.9999999999999996669, 0.9999999999999996669, 1.000000000000000000, 1.000000000000000222, 1.000000000000000000, 1.000000000000000000, 1.000000000000000000, 1.000000000000000000, 1.000000000000000000, 1.000000000000000000, 1.000000000000000000, 1.000000000000000000) ) ) 
 REPRESENTATION_ITEM ( '' )  SURFACE ( )  );
#29141=CARTESIAN_POINT ( 'NONE',  ( -6.442348895218290093E-14, 63.84746620154572838, 4.408874939877717575E-29 ) ) ;
#29147=CARTESIAN_POINT ( 'NONE',  ( -4.667303623731948292, 118.0255731622509643, 0.5720496121413468638 ) ) ;
#29150=VERTEX_POINT ( 'NONE', #4567 ) ;
#29153=CARTESIAN_POINT ( 'NONE',  ( 8.403226289273074912, 119.7337369526196369, -1.096787843810197893 ) ) ;
#29154=CARTESIAN_POINT ( 'NONE',  ( -1.365700293149888278, 106.2535611835979239, -5.166841330979377034 ) ) ;
#29155=CARTESIAN_POINT ( 'NONE',  ( 4.704201265585868263, 117.9644370305355210, 0.8021818384322239037 ) ) ;
#29158=CARTESIAN_POINT ( 'NONE',  ( -15.33786013020733563, 149.0334586719817764, -1.566117276479743303 ) ) ;
#29159=CARTESIAN_POINT ( 'NONE',  ( -3.908125678941627879, 115.7034627620156044, -1.591772151217179188 ) ) ;
#29162=CARTESIAN_POINT ( 'NONE',  ( 5.086085965935678743, 114.3657942991566472, -1.756424186875608751 ) ) ;
#29163=CARTESIAN_POINT ( 'NONE',  ( -8.769168840778196028, 122.1986804192922875, -1.175795117382457455 ) ) ;
#29164=LINE ( 'NONE', #39615, #35339 ) ;
#29165=FACE_OUTER_BOUND ( 'NONE', #8428, .T. ) ;
#29166=CARTESIAN_POINT ( 'NONE',  ( -0.6420072254102160425, 156.3034662015458593, 0.02290919489485064575 ) ) ;
#29167=EDGE_CURVE ( 'NONE', #17268, #5804, #40348, .T. ) ;
#29168=CARTESIAN_POINT ( 'NONE',  ( -3.974385726840726107, -7.478117039488521023, -2.359557994316856533 ) ) ;
#29169=CARTESIAN_POINT ( 'NONE',  ( 11.45183593531609745, 118.8698716516685465, 0.7694570404682200548 ) ) ;
#29170=ORIENTED_EDGE ( 'NONE', *, *, #10346, .T. ) ;
#29172=CARTESIAN_POINT ( 'NONE',  ( 3.340243159461592448, -15.49156354636899202, 3.813188716183662397 ) ) ;
#29173=CARTESIAN_POINT ( 'NONE',  ( -1.037157837436492702, 157.7941190989783991, 1.604419329240822201 ) ) ;
#29174=CARTESIAN_POINT ( 'NONE',  ( 0.9749890475506259868, 2.950361319068162569, -0.03356295239053608964 ) ) ;
#29175=CARTESIAN_POINT ( 'NONE',  ( -23.12711913739495984, 149.5941399179437781, -0.9155080916133789826 ) ) ;
#29176=CARTESIAN_POINT ( 'NONE',  ( -0.9350042896817728488, 3.318609271805546435, -0.2773724203853295545 ) ) ;
#29177=ORIENTED_EDGE ( 'NONE', *, *, #35448, .F. ) ;
#29180=CARTESIAN_POINT ( 'NONE',  ( 4.970930975556632880, 121.2162878128435892, 0.3527489803516246081 ) ) ;
#29182=CARTESIAN_POINT ( 'NONE',  ( -10.46017523140589134, 124.8149993102252182, 0.6249645713522344881 ) ) ;
#29183=CARTESIAN_POINT ( 'NONE',  ( 4.087908758852305091, -13.37781719547838399, 3.422002167429263331 ) ) ;
#29184=CARTESIAN_POINT ( 'NONE',  ( 6.603469437764709404, 120.5225452898634728, -0.8609044167644230861 ) ) ;
#29185=CARTESIAN_POINT ( 'NONE',  ( 0.03245814172805068509, 158.1186941186938952, -1.624338139048501217 ) ) ;
#29188=CARTESIAN_POINT ( 'NONE',  ( 2.460727335429193197, -15.06314154744310585, 4.845259171755021299 ) ) ;
#29189=CARTESIAN_POINT ( 'NONE',  ( -0.01249116623180959208, 38.87185441664305330, -1.227828225846576471 ) ) ;
#29190=CARTESIAN_POINT ( 'NONE',  ( 10.40586874195270362, 126.0814211662656419, -0.04952998093763438803 ) ) ;
#29192=CARTESIAN_POINT ( 'NONE',  ( 0.1909974646900941819, 105.7854974534635346, 5.338829247572753900 ) ) ;
#29196=CARTESIAN_POINT ( 'NONE',  ( 4.878702690786834495, 117.7581303304119729, -0.7584199409633860522 ) ) ;
#29199=CARTESIAN_POINT ( 'NONE',  ( 23.35271726849051177, 148.8653451956335516, 0.3123667622787954512 ) ) ;
#29201=DIRECTION ( 'NONE',  ( -0.9998004120163608288, 0.000000000000000000, -0.01997839162482749342 ) ) ;
#29202=CARTESIAN_POINT ( 'NONE',  ( -0.8472427164685307766, -8.777537934218566207, -4.544909406875613733 ) ) ;
#29203=CARTESIAN_POINT ( 'NONE',  ( 1.104298428969494816, 36.37359162847545235, -0.6925126829677044071 ) ) ;
#29204=CARTESIAN_POINT ( 'NONE',  ( 21.07518769967733974, 148.4376209648218321, 2.358402543220756264 ) ) ;
#29206=CARTESIAN_POINT ( 'NONE',  ( 0.4006815055314144058, 20.64345356492705719, 4.603752038498275745 ) ) ;
#29207=CARTESIAN_POINT ( 'NONE',  ( -0.9165671635830696662, -12.81903285835614525, -8.372742598224451882 ) ) ;
#29208=CARTESIAN_POINT ( 'NONE',  ( 8.740654271741430392, 118.0242495335989759, -0.4400757740126230444 ) ) ;
#29209=CARTESIAN_POINT ( 'NONE',  ( -0.7595712053401582065, 120.2878791493615296, -0.5727019010319392978 ) ) ;
#29211=CARTESIAN_POINT ( 'NONE',  ( 1.351374093494389417, 106.2781030281888235, -5.112228481377823819 ) ) ;
#29212=CARTESIAN_POINT ( 'NONE',  ( 3.260699289383273136, 104.6144662015456959, 3.570726652201047013 ) ) ;
#29213=CARTESIAN_POINT ( 'NONE',  ( 4.636458409304901274, 17.36039413176390411, -0.09481320587925551324 ) ) ;
#29216=CARTESIAN_POINT ( 'NONE',  ( 3.149239739297259533, -13.85570235734440203, 1.885463239856044027 ) ) ;
#29217=ADVANCED_FACE ( 'NONE', ( #30312, #1366 ), #20927, .F. ) ;
#29218=CARTESIAN_POINT ( 'NONE',  ( 0.1833862045735744073, 106.0860833631645193, -5.249533627824054527 ) ) ;
#29219=CARTESIAN_POINT ( 'NONE',  ( -15.31827776641181060, 121.1074504348956964, 0.3839962087354599762 ) ) ;
#29220=AXIS2_PLACEMENT_3D ( 'NONE', #14155, #7577, #33568 ) ;
#29224=ORIENTED_EDGE ( 'NONE', *, *, #41697, .F. ) ;
#29225=CARTESIAN_POINT ( 'NONE',  ( 5.586884702347362897, 136.3644662015457527, 0.1116392523995368563 ) ) ;
#29226=CARTESIAN_POINT ( 'NONE',  ( 4.032098335577404491, -15.72255795053374783, 4.298576634473052493 ) ) ;
#29227=CARTESIAN_POINT ( 'NONE',  ( -8.870548826841627488, 119.8693228481767932, 1.115469810106635595 ) ) ;
#29228=CARTESIAN_POINT ( 'NONE',  ( 6.863242444369292983, 118.1252062928739832, -0.7545491157480663791 ) ) ;
#29229=EDGE_CURVE ( 'NONE', #22232, #40883, #13023, .T. ) ;
#29230=CARTESIAN_POINT ( 'NONE',  ( 2.551540157903699146, -0.3564265548712530207, -3.854280124997286450 ) ) ;
#29233=CARTESIAN_POINT ( 'NONE',  ( 7.784012320830338005, 122.6313477005580665, 0.1555430910899518460 ) ) ;
#29235=CARTESIAN_POINT ( 'NONE',  ( -11.13866856781930359, 123.6647009725989648, 1.091370626813936706 ) ) ;
#29237=CARTESIAN_POINT ( 'NONE',  ( 19.00012635448478449, 147.0452383304005082, -1.727400128179959804 ) ) ;
#29238=CARTESIAN_POINT ( 'NONE',  ( -1.134298505455661354, 158.7113841514841681, -1.516915449716996767 ) ) ;
#29241=CARTESIAN_POINT ( 'NONE',  ( 4.493133734558046655, 118.1300458714410269, -0.5260358870164894007 ) ) ;
#29242=CARTESIAN_POINT ( 'NONE',  ( 10.87798892776812210, 126.1616406593870607, -0.4640774846651394281 ) ) ;
#29244=CARTESIAN_POINT ( 'NONE',  ( -9.109784082438133979, 121.7740273863187923, -1.385347505406782087 ) ) ;
#29245=CARTESIAN_POINT ( 'NONE',  ( 2.557542807212066283, -15.51814986354871451, 4.851437248720891660 ) ) ;
#29249=TOROIDAL_SURFACE ( 'NONE', #17687, 5.080000000000005400, 0.5080000000000000071 ) ;
#29250=CARTESIAN_POINT ( 'NONE',  ( -4.818488311985083428, 117.7362444359860945, 0.8718948188861159743 ) ) ;
#29251=CARTESIAN_POINT ( 'NONE',  ( 0.5297590882381500998, 119.7690751942239729, 0.5117926329762008120 ) ) ;
#29253=CARTESIAN_POINT ( 'NONE',  ( -3.685501180670149424, 30.72893705507438611, -2.802369389919810772 ) ) ;
#29254=CARTESIAN_POINT ( 'NONE',  ( 1.603837441938149144, 120.9755568995931156, 0.09629321774905875986 ) ) ;
#29259=CARTESIAN_POINT ( 'NONE',  ( -8.798071503329609300, 117.6842349159552867, -0.1758064076808953657 ) ) ;
#29263=CARTESIAN_POINT ( 'NONE',  ( -8.243407495045023126, 120.2654484654224092, -1.445016461426329224 ) ) ;
#29269=CARTESIAN_POINT ( 'NONE',  ( -15.14699153459433845, 156.1345691653134509, -0.01578391296358631554 ) ) ;
#29270=VERTEX_POINT ( 'NONE', #30733 ) ;
#29272=CARTESIAN_POINT ( 'NONE',  ( 7.791101006339050450, 122.6066354939652570, 0.05439624365677588058 ) ) ;
#29277=CARTESIAN_POINT ( 'NONE',  ( -15.53993717541254149, 147.5346097818530211, -0.5395553097850841473 ) ) ;
#29278=CARTESIAN_POINT ( 'NONE',  ( 4.583978111877545558, -14.49189839317011064, 4.572462404262108038 ) ) ;
#29279=CARTESIAN_POINT ( 'NONE',  ( -13.10001109591399349, 121.1598417376693533, 1.052633080380691144 ) ) ;
#29281=CARTESIAN_POINT ( 'NONE',  ( 13.37536684427238320, 156.9592627042916604, 0.5421920129525309440 ) ) ;
#29282=EDGE_CURVE ( 'NONE', #35171, #10724, #35542, .T. ) ;
#29283=CARTESIAN_POINT ( 'NONE',  ( 8.978876846644611831, 124.0550666853292086, 0.2683953620638208637 ) ) ;
#29285=CARTESIAN_POINT ( 'NONE',  ( -0.08510646190747463147, 11.08924109716144280, -0.9717149503703566005 ) ) ;
#29286=CARTESIAN_POINT ( 'NONE',  ( -1.824897337458840640, 116.5125207362610951, -0.1392185346034942595 ) ) ;
#29290=CARTESIAN_POINT ( 'NONE',  ( -2.623632515124386444, 116.9061775504940641, 0.4731523196332259040 ) ) ;
#29291=EDGE_LOOP ( 'NONE', ( #23546, #23493 ) ) ;
#29293=CARTESIAN_POINT ( 'NONE',  ( 13.21493909911900033, 121.0513591912305316, 1.522979426720440843 ) ) ;
#29294=CARTESIAN_POINT ( 'NONE',  ( 16.44572402506187103, 128.5611466799914240, -1.520858254922803354 ) ) ;
#29295=CARTESIAN_POINT ( 'NONE',  ( -0.2870776928289196506, 5.753151106566044781, -0.9307745581249481370 ) ) ;
#29296=CARTESIAN_POINT ( 'NONE',  ( 6.828157356468467221, 12.44753447943134184, 4.948315318077098901 ) ) ;
#29297=CARTESIAN_POINT ( 'NONE',  ( -13.91935487398219529, 155.8415165211600595, -1.849969996916311699 ) ) ;
#29298=CARTESIAN_POINT ( 'NONE',  ( 4.890857177472106798, 117.7454522775086758, -0.7293204476797061631 ) ) ;
#29301=CARTESIAN_POINT ( 'NONE',  ( 10.33346200648606050, 123.4707319107414492, -0.9080611472405731854 ) ) ;
#29302=CARTESIAN_POINT ( 'NONE',  ( -9.007539097974415654, 123.9742709865185191, -0.1460878630902625874 ) ) ;
#29304=CARTESIAN_POINT ( 'NONE',  ( -18.13772925547832315, 148.8986565181125457, -2.425799293919265409 ) ) ;
#29305=CARTESIAN_POINT ( 'NONE',  ( 2.988498945533646367, -15.63929389023541106, 5.494461050752756925 ) ) ;
#29306=CARTESIAN_POINT ( 'NONE',  ( 4.787223994907250813, 118.5931160184169073, 0.9409944917690892252 ) ) ;
#29311=CARTESIAN_POINT ( 'NONE',  ( 11.58192335640127446, 123.0696236843973281, 1.706247406239837616 ) ) ;
#29312=CARTESIAN_POINT ( 'NONE',  ( -15.76285804746350649, 145.9067145067647857, -0.3149794173055759927 ) ) ;
#29315=CARTESIAN_POINT ( 'NONE',  ( -4.584908976608091713, 124.7699485019152945, -0.08702032153807684467 ) ) ;
#29316=CARTESIAN_POINT ( 'NONE',  ( 4.725500162001525339, -13.89046571553399900, -6.993667195001821213 ) ) ;
#29317=CARTESIAN_POINT ( 'NONE',  ( 8.743035643995668238, 123.3024417045633498, 0.5730362264965975783 ) ) ;
#29318=CARTESIAN_POINT ( 'NONE',  ( 3.877771370679228280, 117.0975898859979054, -0.4181078409183315303 ) ) ;
#29321=CARTESIAN_POINT ( 'NONE',  ( -3.707388773974424900, 116.6237204831772232, -0.06043239539139034361 ) ) ;
#29323=CARTESIAN_POINT ( 'NONE',  ( 6.381125341793176808, 120.0353217841789331, -0.9518924694056809521 ) ) ;
#29324=CARTESIAN_POINT ( 'NONE',  ( 3.843300253784490028, -15.24301522717705026, 5.225518813476231372 ) ) ;
#29325=CARTESIAN_POINT ( 'NONE',  ( -15.83096054209209136, 147.2950763206921181, -1.041347660067663217 ) ) ;
#29326=CARTESIAN_POINT ( 'NONE',  ( 2.954207113090831616, -14.52495373116942368, 5.111795949899043734 ) ) ;
#29327=CARTESIAN_POINT ( 'NONE',  ( -5.153942072456670687, 116.8381265693619895, -0.06466201385226102993 ) ) ;
#29329=CARTESIAN_POINT ( 'NONE',  ( 4.716951831472176337, 116.7562497393984415, 0.1081823505139637015 ) ) ;
#29333=CARTESIAN_POINT ( 'NONE',  ( -4.544942180623752215, 12.81246518813932589, 0.8472608254572608910 ) ) ;
#29334=CARTESIAN_POINT ( 'NONE',  ( -4.713631738767456447, 116.7564862437112794, -0.09418957996065560612 ) ) ;
#29337=CARTESIAN_POINT ( 'NONE',  ( 6.993874078755136559, 121.7930633702997341, 0.5635671808028978047 ) ) ;
#29338=CARTESIAN_POINT ( 'NONE',  ( -2.394960105286914942, 16.54535949628658997, -3.951836011466995036 ) ) ;
#29339=CARTESIAN_POINT ( 'NONE',  ( 16.14352587498443015, 122.8183540351560907, 1.297681478882586337 ) ) ;
#29340=FACE_OUTER_BOUND ( 'NONE', #9935, .T. ) ;
#29341=CARTESIAN_POINT ( 'NONE',  ( 3.150244473240279675, -14.07033042043420146, 1.813758411523331393 ) ) ;
#29342=CARTESIAN_POINT ( 'NONE',  ( 18.67489051167924785, 151.9584835496716266, -1.528205706551668319 ) ) ;
#29344=CARTESIAN_POINT ( 'NONE',  ( 4.531904421025400254, 4.026177021345840323, -0.9239884639389631671 ) ) ;
#29345=CARTESIAN_POINT ( 'NONE',  ( -5.835170694357168841, 117.3723397083485622, -0.6929373658347460774 ) ) ;
#29347=CARTESIAN_POINT ( 'NONE',  ( -3.695597174622082370, 120.9852966486377710, 0.1212977071129683060 ) ) ;
#29348=CARTESIAN_POINT ( 'NONE',  ( 2.834973442847717351, -15.21714937722351557, 5.773325752997570781 ) ) ;
#29350=CYLINDRICAL_SURFACE ( 'NONE', #33619, 3.175000000000001155 ) ;
#29351=CARTESIAN_POINT ( 'NONE',  ( -1.698985622072688884, 106.4942957007677649, -5.056388078100372496 ) ) ;
#29353=CARTESIAN_POINT ( 'NONE',  ( 1.258058525836107444, 118.8689652838214244, 0.6902481975293249805 ) ) ;
#29355=CARTESIAN_POINT ( 'NONE',  ( 9.163388821854780986, 124.2347608867413413, 0.1831063163140475014 ) ) ;
#29358=CARTESIAN_POINT ( 'NONE',  ( -22.64859486804675726, 149.7032342875954498, 0.6240689893612101358 ) ) ;
#29360=CARTESIAN_POINT ( 'NONE',  ( 4.789291700406207219, 116.8922783744782379, -0.1888386708474939224 ) ) ;
#29364=CARTESIAN_POINT ( 'NONE',  ( 1.934325240867707629, -15.05852118660004635, 5.638101517764280146 ) ) ;
#29366=CARTESIAN_POINT ( 'NONE',  ( 2.666490510518176649, -13.49855353256042712, 0.05227394649444803282 ) ) ;
#29367=CARTESIAN_POINT ( 'NONE',  ( -4.613770077645467538, 118.0656789020681998, 0.5556151127989765737 ) ) ;
#29370=EDGE_LOOP ( 'NONE', ( #26881, #22390, #17534, #5321 ) ) ;
#29371=CARTESIAN_POINT ( 'NONE',  ( -0.9749357855001491435, 115.6909491485452435, -1.750966270793492541 ) ) ;
#29372=CARTESIAN_POINT ( 'NONE',  ( 5.997780686918567028, 119.2096731566373364, -1.027357156148055228 ) ) ;
#29373=CARTESIAN_POINT ( 'NONE',  ( -4.366878780879607014, 111.2667756541687538, -3.131538613950388239 ) ) ;
#29374=CARTESIAN_POINT ( 'NONE',  ( 4.661500840997910622, 117.9823968663990144, 0.8616593033297639259 ) ) ;
#29376=CARTESIAN_POINT ( 'NONE',  ( -13.09552101555883574, 130.8944540161131442, -1.428626934261719050 ) ) ;
#29377=CARTESIAN_POINT ( 'NONE',  ( -2.395404871435389271, 115.7029496080882467, -1.700622835054004023 ) ) ;
#29380=CARTESIAN_POINT ( 'NONE',  ( 7.643874070029819556, 124.9344662015457317, 0.1527427953284561379 ) ) ;
#29381=CARTESIAN_POINT ( 'NONE',  ( -3.477534164838183006, 156.5024071230465097, -1.413294873543960106 ) ) ;
#29383=CARTESIAN_POINT ( 'NONE',  ( -0.01887828017123771920, 156.5412816204240301, 0.9447463363288814975 ) ) ;
#29385=CARTESIAN_POINT ( 'NONE',  ( -7.778077869716700121, 154.6678004290674266, -0.09965222998851200331 ) ) ;
#29386=CARTESIAN_POINT ( 'NONE',  ( 3.501419995798253915, -2.955197114699519734, 3.043391175950921568 ) ) ;
#29387=CARTESIAN_POINT ( 'NONE',  ( 23.06261834269074029, 146.6371693212631158, 1.324134011023373025 ) ) ;
#29390=CARTESIAN_POINT ( 'NONE',  ( 3.520778385322295811, -15.02221911624387829, 1.583774285062736986 ) ) ;
#29391=CARTESIAN_POINT ( 'NONE',  ( -18.66004122726579695, 149.2887123452801745, 1.736808470001687255 ) ) ;
#29392=CARTESIAN_POINT ( 'NONE',  ( -0.9744428630873758213, 7.697845052497760854, 0.001242513977635927719 ) ) ;
#29393=CARTESIAN_POINT ( 'NONE',  ( -22.44855437653378871, 150.5824416163731314, -1.170575646458954067 ) ) ;
#29394=VECTOR ( 'NONE', #37922, 1000.000000000000000 ) ;
#29395=CARTESIAN_POINT ( 'NONE',  ( 0.3393679441828953980, -8.777600141791896959, -0.9147772600509928020 ) ) ;
#29396=ORIENTED_EDGE ( 'NONE', *, *, #39977, .F. ) ;
#29399=CARTESIAN_POINT ( 'NONE',  ( 4.994922087954005718, 114.3796182124986984, 1.954983995200229030 ) ) ;
#29400=CARTESIAN_POINT ( 'NONE',  ( -4.574562528865663502, 155.9125706774115940, 0.7527123864290743427 ) ) ;
#29401=CARTESIAN_POINT ( 'NONE',  ( 2.780001287168888613, -14.74817992026429536, 5.465600930587551254 ) ) ;
#29402=CARTESIAN_POINT ( 'NONE',  ( 9.357607378341723958, 155.0893615026619159, -1.530462696531121214 ) ) ;
#29403=CARTESIAN_POINT ( 'NONE',  ( -13.64693284513013793, 123.6869008171703541, -1.914747182567867023 ) ) ;
#29405=CARTESIAN_POINT ( 'NONE',  ( 2.858040400949144022, -14.78363303536489681, 4.300485631455113200 ) ) ;
#29406=CARTESIAN_POINT ( 'NONE',  ( -4.993862003731174504, 32.72552215703572642, 2.980277739178222252 ) ) ;
#29407=CARTESIAN_POINT ( 'NONE',  ( 5.925782188533577965, 121.5237468798633955, -0.003878672073842357685 ) ) ;
#29408=ORIENTED_EDGE ( 'NONE', *, *, #19550, .T. ) ;
#29414=B_SPLINE_CURVE_WITH_KNOTS ( 'NONE', 3,
 ( #161, #9312, #12710, #35936 ),
 .UNSPECIFIED., .F., .F.,
 ( 4, 4 ),
 ( 0.0001462341759615505836, 0.0005711421393943891126 ),
 .UNSPECIFIED. ) ;
#29415=CARTESIAN_POINT ( 'NONE',  ( 14.84180086987428382, 120.3134675335783754, 0.1939203138368898183 ) ) ;
#29416=CARTESIAN_POINT ( 'NONE',  ( -6.742182786529062000, 121.2177056076135528, 0.07361405433131856801 ) ) ;
#29418=CARTESIAN_POINT ( 'NONE',  ( -1.144953672747696993, 115.6909491485452435, 1.703244984983935506 ) ) ;
#29420=CARTESIAN_POINT ( 'NONE',  ( 0.4700063951662839523, 38.82598460892266701, -1.223737656376347127 ) ) ;
#29421=CARTESIAN_POINT ( 'NONE',  ( 13.39049918543318185, 121.7711344121973411, 1.690880791723282428 ) ) ;
#29422=CARTESIAN_POINT ( 'NONE',  ( 4.233688895176465294, 13.94658232072815807, -1.861163356065342001 ) ) ;
#29423=CARTESIAN_POINT ( 'NONE',  ( 6.528609751734300914, 25.78175851779908356, 5.377075232920663694 ) ) ;
#29424=CARTESIAN_POINT ( 'NONE',  ( -2.168094803691708705, 116.7617983115602840, -0.5049745822317547317 ) ) ;
#29425=CARTESIAN_POINT ( 'NONE',  ( -1.155499320159524723, 111.9985432423065959, -2.960082065640199822 ) ) ;
#29427=DIRECTION ( 'NONE',  ( 4.017660918040594346E-17, -1.000000000000000000, -2.376309959284834438E-19 ) ) ;
#29428=CARTESIAN_POINT ( 'NONE',  ( -2.879560631192479292, 105.1244045648011678, 4.501302620457409809 ) ) ;
#29429=CARTESIAN_POINT ( 'NONE',  ( 4.573446973487649281, 17.56025517495590904, -0.6989348988664985107 ) ) ;
#29431=CARTESIAN_POINT ( 'NONE',  ( -17.31377588638430964, 122.7721875394316555, -0.3459704467065360944 ) ) ;
#29432=CARTESIAN_POINT ( 'NONE',  ( 2.664052010559913253, -13.52006206191685322, 0.08958796903007473778 ) ) ;
#29435=CARTESIAN_POINT ( 'NONE',  ( 1.751097875588997654, 120.5851793143259130, -0.4017021596164529473 ) ) ;
#29436=CARTESIAN_POINT ( 'NONE',  ( -11.47343314416685978, 118.8698716516685465, 0.3113556051519841272 ) ) ;
#29438=ORIENTED_EDGE ( 'NONE', *, *, #4529, .F. ) ;
#29442=CARTESIAN_POINT ( 'NONE',  ( 5.792286216032899837, -14.99041835605292938, 0.9165201714659111376 ) ) ;
#29443=CARTESIAN_POINT ( 'NONE',  ( -12.99265913520525473, 122.2940260782629451, 1.284300974089672920 ) ) ;
#29444=CARTESIAN_POINT ( 'NONE',  ( 14.33513709641994893, 121.5541609676003389, -0.9327927267376098230 ) ) ;
#29445=CARTESIAN_POINT ( 'NONE',  ( -0.2084201458593382406, 5.265951782950084592, 4.622859108429906883 ) ) ;
#29448=LINE ( 'NONE', #29871, #41537 ) ;
#29449=CARTESIAN_POINT ( 'NONE',  ( 0.3561418115364049508, 119.9741034315941732, 0.6738560125758275010 ) ) ;
#29451=CARTESIAN_POINT ( 'NONE',  ( -17.03225580939810158, 146.4457527449227143, 1.249628170391535731 ) ) ;
#29452=CARTESIAN_POINT ( 'NONE',  ( -6.642767299088215313E-14, 101.1854662015457365, -1.199848199765585135E-18 ) ) ;
#29453=CARTESIAN_POINT ( 'NONE',  ( 18.22015820038723533, 148.8986565181125457, -1.699282175587853327 ) ) ;
#29454=CARTESIAN_POINT ( 'NONE',  ( -6.788760123629518972, 157.9234729166680040, -1.828055096104673538 ) ) ;
#29456=VECTOR ( 'NONE', #66, 1000.000000000000000 ) ;
#29458=CARTESIAN_POINT ( 'NONE',  ( 4.517430400727893591, 118.1170754611382137, -0.5419986605907590738 ) ) ;
#29459=CARTESIAN_POINT ( 'NONE',  ( 16.12610658153775489, 147.0533492130506943, -0.6457432798159421505 ) ) ;
#29460=ORIENTED_EDGE ( 'NONE', *, *, #27896, .T. ) ;
#29461=CARTESIAN_POINT ( 'NONE',  ( -7.341258159293269081, 120.8389031223305352, -1.207285925005196603 ) ) ;
#29462=CARTESIAN_POINT ( 'NONE',  ( 3.752486096903807855, -15.17702595220350759, -0.4382564666907802220 ) ) ;
#29463=CARTESIAN_POINT ( 'NONE',  ( -6.654617103318593247E-14, 104.6144662015457243, 1.534725424433578570E-31 ) ) ;
#29465=EDGE_CURVE ( 'NONE', #11359, #12283, #34844, .T. ) ;
#29467=CARTESIAN_POINT ( 'NONE',  ( -4.757398851944955709, 117.7257754445831921, 0.9114319017062125772 ) ) ;
#29468=CARTESIAN_POINT ( 'NONE',  ( 11.08617792162969096, 123.6647009725989648, 1.535475951868171984 ) ) ;
#29469=CARTESIAN_POINT ( 'NONE',  ( -1.209753656675892186, 31.97884461091921082, 1.539940357435441776 ) ) ;
#29470=CARTESIAN_POINT ( 'NONE',  ( 2.889066315880882030, 25.55657059589919911, 3.609430016826872478 ) ) ;
#29471=CARTESIAN_POINT ( 'NONE',  ( 9.045001602728808265, 123.9859359328134190, 0.2652644514531634634 ) ) ;
#29479=CARTESIAN_POINT ( 'NONE',  ( -8.547848780159753801, 118.8034570524430933, -1.212240055924699966 ) ) ;
#29486=CARTESIAN_POINT ( 'NONE',  ( -18.64921795038435803, 125.2334963081946313, -0.1144521110716926748 ) ) ;
#29488=ORIENTED_EDGE ( 'NONE', *, *, #39980, .F. ) ;
#29490=CARTESIAN_POINT ( 'NONE',  ( 6.056944315494892983, 121.4421416482665421, 0.1030667194366131911 ) ) ;
#29491=EDGE_LOOP ( 'NONE', ( #39721, #40809, #31680, #4918 ) ) ;
#29492=CARTESIAN_POINT ( 'NONE',  ( -5.332909801388204585, 115.7029491485453718, -0.1078398302286824040 ) ) ;
#29493=CARTESIAN_POINT ( 'NONE',  ( -0.6438746309741667506, 120.9974662015465867, -0.01286614746332115887 ) ) ;
#29494=CARTESIAN_POINT ( 'NONE',  ( 4.440325138859688714, -14.57630248335078882, 4.728313687495418804 ) ) ;
#29495=CARTESIAN_POINT ( 'NONE',  ( -21.36815210116614949, 148.0064520001644723, 1.462276224275804060 ) ) ;
#29497=CIRCLE ( 'NONE', #27462, 0.5080000000000002292 ) ;
#29498=CARTESIAN_POINT ( 'NONE',  ( 16.04055624107191491, 121.3766923467913585, 0.6455242483069041359 ) ) ;
#29499=CARTESIAN_POINT ( 'NONE',  ( 2.159762389889169132, -15.63309910277781078, 5.565077868897359004 ) ) ;
#29500=CARTESIAN_POINT ( 'NONE',  ( 4.831409462241198050, 118.5266822147775940, -0.7504941915039914369 ) ) ;
#29501=CARTESIAN_POINT ( 'NONE',  ( -0.8226642509504364931, 2.890957568680109446, -0.5268263738024351328 ) ) ;
#29502=CARTESIAN_POINT ( 'NONE',  ( -22.52498503541054120, 150.7873321363286152, -0.6028683204863920508 ) ) ;
#29505=LINE ( 'NONE', #22661, #19307 ) ;
#29507=CARTESIAN_POINT ( 'NONE',  ( -8.743388953545744968, 118.0097374530782588, 0.4280054902111584125 ) ) ;
#29509=CARTESIAN_POINT ( 'NONE',  ( -18.17603978048573765, 146.7121067869193496, 1.621728993581971867 ) ) ;
#29511=CARTESIAN_POINT ( 'NONE',  ( 18.79035964875395237, 131.8417273817641444, 2.102833481017198469 ) ) ;
#29512=CARTESIAN_POINT ( 'NONE',  ( 15.12798499870458535, 125.5446871707752763, -1.421763802809897115 ) ) ;
#29513=CARTESIAN_POINT ( 'NONE',  ( -0.01718310852247704676, 5.323846764136113130, -0.9747645957998940514 ) ) ;
#29514=CARTESIAN_POINT ( 'NONE',  ( -7.226289359486380626, 158.3006260280594404, -1.552328403643544963 ) ) ;
#29515=CARTESIAN_POINT ( 'NONE',  ( 4.613544267573807645, 118.0656495166530817, -0.5557507275274983227 ) ) ;
#29516=CARTESIAN_POINT ( 'NONE',  ( 7.694663930960251363, 124.9344662015457317, 0.1537576976229974857 ) ) ;
#29517=CARTESIAN_POINT ( 'NONE',  ( 14.42666092703562875, 134.5679602169015254, -1.107736707283930810 ) ) ;
#29518=CARTESIAN_POINT ( 'NONE',  ( -0.6418402141072927503, 156.3034662015456888, 0.01455126635812875602 ) ) ;
#29520=CARTESIAN_POINT ( 'NONE',  ( -2.417314592637459736, 119.3768144667271542, -0.7569762546260363489 ) ) ;
#29521=CARTESIAN_POINT ( 'NONE',  ( 3.601051898931722395, -15.74651769575186044, 4.782909482641136911 ) ) ;
#29522=CIRCLE ( 'NONE', #28814, 3.175000000000001155 ) ;
#29527=CARTESIAN_POINT ( 'NONE',  ( 11.45041423386206425, 122.9335272575421669, 1.692945391654126608 ) ) ;
#29530=CARTESIAN_POINT ( 'NONE',  ( 4.799643950526473191, 115.7029491485453292, 1.472414092453835588 ) ) ;
#29532=CARTESIAN_POINT ( 'NONE',  ( -1.889402974298121762, 108.8931014686503289, 4.028630146538900725 ) ) ;
#29534=CARTESIAN_POINT ( 'NONE',  ( 7.497756367663003019, 26.09243224653669913, 3.946719672664338319 ) ) ;
#29535=CARTESIAN_POINT ( 'NONE',  ( 9.301285777573523816, 153.8845013697122965, 0.8210809464416258807 ) ) ;
#29536=CARTESIAN_POINT ( 'NONE',  ( 0.01289612358321921490, 159.5048567107479585, -0.6453747585945881493 ) ) ;
#29537=LINE ( 'NONE', #28895, #32879 ) ;
#29541=CARTESIAN_POINT ( 'NONE',  ( -4.725057015249868542, 116.7592613395855352, -0.05262260997884638664 ) ) ;
#29544=CARTESIAN_POINT ( 'NONE',  ( 6.768164194442967130, 121.0451091176095559, -0.7116084776782327648 ) ) ;
#29545=CARTESIAN_POINT ( 'NONE',  ( 5.914793047224296885, -14.26696172101640414, 2.399059881747223955 ) ) ;
#29547=CARTESIAN_POINT ( 'NONE',  ( -13.71401989163329027, 150.2158912636999730, -0.8490545446796917695 ) ) ;
#29548=CARTESIAN_POINT ( 'NONE',  ( 3.761132227337853351, -14.12294213130394027, 4.617837385609514733 ) ) ;
#29549=CARTESIAN_POINT ( 'NONE',  ( -2.057861540686834800, 117.3535355059730705, 0.5007145131239727487 ) ) ;
#29550=DIRECTION ( 'NONE',  ( 4.017660918040594346E-17, -1.000000000000000000, -2.376309959284834438E-19 ) ) ;
#29551=CARTESIAN_POINT ( 'NONE',  ( -0.0007535234283137855638, 116.4338605912342786, 0.03770939363766613595 ) ) ;
#29553=CARTESIAN_POINT ( 'NONE',  ( 1.068493265602401987, 5.690783753869971484, 4.496582723949734017 ) ) ;
#29554=CARTESIAN_POINT ( 'NONE',  ( -3.789105058680120042, 105.1231779575318228, 3.768300612546575667 ) ) ;
#29556=CARTESIAN_POINT ( 'NONE',  ( 1.906794157568332038, 106.4600999034464195, 4.997634466524000452 ) ) ;
#29557=CARTESIAN_POINT ( 'NONE',  ( -8.076703871748769359, 121.3095967058478095, 0.9279539172270194758 ) ) ;
#29558=CARTESIAN_POINT ( 'NONE',  ( -1.792273654952471595, 16.32048121479114045, -4.264856162967389785 ) ) ;
#29559=CARTESIAN_POINT ( 'NONE',  ( 14.63850908477041202, 156.0817623197167450, 1.342817726712510540 ) ) ;
#29561=CARTESIAN_POINT ( 'NONE',  ( 0.01051220311278149022, 117.9844940561907265, -0.5260736299896251467 ) ) ;
#29562=CARTESIAN_POINT ( 'NONE',  ( 1.748379858460863856, 5.525481214791113871, -4.283037568778763848 ) ) ;
#29563=CARTESIAN_POINT ( 'NONE',  ( -22.77131365710839717, 149.1304179266472261, -1.534847161028223939 ) ) ;
#29566=ORIENTED_EDGE ( 'NONE', *, *, #22719, .T. ) ;
#29568=CARTESIAN_POINT ( 'NONE',  ( -2.792630161979596348, 120.9517662584847102, 0.08501465617163909971 ) ) ;
#29569=CARTESIAN_POINT ( 'NONE',  ( 3.633732803939692335, -15.12841498804032270, 5.400629595854979037 ) ) ;
#29570=CARTESIAN_POINT ( 'NONE',  ( -5.078986093043186045, 79.34146620154574236, -0.1014902294541237954 ) ) ;
#29571=CARTESIAN_POINT ( 'NONE',  ( -0.1816225517746203333, 105.8842979884732785, -5.338741224315539213 ) ) ;
#29572=ORIENTED_EDGE ( 'NONE', *, *, #26904, .T. ) ;
#29573=CARTESIAN_POINT ( 'NONE',  ( 15.73670139478151242, 128.5598958631237565, 2.193363351549679319 ) ) ;
#29575=CARTESIAN_POINT ( 'NONE',  ( 11.03183784343224616, 128.0124916018596650, 0.2204423744267036411 ) ) ;
#29576=CARTESIAN_POINT ( 'NONE',  ( -20.24728863611177587, 152.4988772720997190, 0.6427007754482431112 ) ) ;
#29577=ADVANCED_FACE ( 'NONE', ( #25190 ), #37974, .T. ) ;
#29578=CARTESIAN_POINT ( 'NONE',  ( 8.421720897435127640, 23.01747231734997357, -0.09500337383513672573 ) ) ;
#29580=CARTESIAN_POINT ( 'NONE',  ( 22.41683308396147822, 150.7562895891929031, -0.1409227600426839200 ) ) ;
#29584=CARTESIAN_POINT ( 'NONE',  ( 1.800280022787231538, -15.11108451883692894, 5.570910438324009561 ) ) ;
#29587=CARTESIAN_POINT ( 'NONE',  ( -4.463662862426327038, 118.1585627870778410, 0.4268197071713389912 ) ) ;
#29589=ORIENTED_EDGE ( 'NONE', *, *, #10189, .F. ) ;
#29591=CARTESIAN_POINT ( 'NONE',  ( -4.999645142055948455, 117.4030427321881263, 0.8338872319069162709 ) ) ;
#29592=CARTESIAN_POINT ( 'NONE',  ( 8.342983529710069845, 120.0295035570879207, -1.117190174572594730 ) ) ;
#29593=CARTESIAN_POINT ( 'NONE',  ( -0.6634819590976430703, 105.9515744484354371, -5.309451348557705508 ) ) ;
#29594=CARTESIAN_POINT ( 'NONE',  ( 4.478158499223182432, 118.1173218799454077, 0.7357564059813932467 ) ) ;
#29596=CARTESIAN_POINT ( 'NONE',  ( -4.636268038904913347, 155.9604050671876792, -1.079575001969328873 ) ) ;
#29597=CARTESIAN_POINT ( 'NONE',  ( -3.040433582521969047, 115.7029506960217731, -1.666328479974650945 ) ) ;
#29598=CARTESIAN_POINT ( 'NONE',  ( -3.174366308152012373, 78.32546620154573702, -0.06343139340882732180 ) ) ;
#29599=CARTESIAN_POINT ( 'NONE',  ( 0.8750585742502747788, 105.9515744484354371, -5.278707647178442208 ) ) ;
#29600=CARTESIAN_POINT ( 'NONE',  ( -3.490201360801296726, 120.2313485970928326, -0.6717870626964185243 ) ) ;
#29602=CARTESIAN_POINT ( 'NONE',  ( -0.006534791579925431325, 156.3267223255430167, 0.3270276925529296275 ) ) ;
#29603=CARTESIAN_POINT ( 'NONE',  ( -4.825036788391023457, 63.33946620154573282, -0.09641571798141691796 ) ) ;
#29604=CARTESIAN_POINT ( 'NONE',  ( -15.76299236085137956, 145.9019260673938163, -0.1804967559267895705 ) ) ;
#29605=CARTESIAN_POINT ( 'NONE',  ( -0.2095918955067871126, -8.989892990265463624, -4.636818132431064221 ) ) ;
#29606=CARTESIAN_POINT ( 'NONE',  ( 14.89898862929382517, 156.1361208441215922, 1.045442070961571934 ) ) ;
#29607=CARTESIAN_POINT ( 'NONE',  ( 4.722078295102365431, 104.6144662015457527, -1.046302231095662671 ) ) ;
#29608=CARTESIAN_POINT ( 'NONE',  ( 3.096790694169950342, -14.35231825047024401, 1.054797312298405121 ) ) ;
#29609=CARTESIAN_POINT ( 'NONE',  ( -8.556073751109543934, 120.5511696877957775, 1.121754095281913610 ) ) ;
#29610=CARTESIAN_POINT ( 'NONE',  ( 0.5118484794875378663, 4.451237885527871363, -0.8280682483750020362 ) ) ;
#29611=CARTESIAN_POINT ( 'NONE',  ( -5.820459347748656143, 117.1115750087645608, -0.4818200784724923635 ) ) ;
#29612=CARTESIAN_POINT ( 'NONE',  ( -0.2306771026100957467, -3.802149480603859377, 0.9475509996518236555 ) ) ;
#29613=VERTEX_POINT ( 'NONE', #38408 ) ;
#29614=ORIENTED_EDGE ( 'NONE', *, *, #30969, .F. ) ;
#29616=CARTESIAN_POINT ( 'NONE',  ( 3.549733929829893331, 110.1236525333376619, 3.577684766704721575 ) ) ;
#29618=CARTESIAN_POINT ( 'NONE',  ( -9.647033449255159709, 123.8920215319950842, 0.4922632944252962606 ) ) ;
#29619=CARTESIAN_POINT ( 'NONE',  ( 3.866302502687585907, -14.02971062843458228, 4.478402296968817531 ) ) ;
#29620=CARTESIAN_POINT ( 'NONE',  ( 1.409223554827445213, 119.7856413326322667, -0.5222593444346081970 ) ) ;
#29621=CARTESIAN_POINT ( 'NONE',  ( -1.216597929035328374, 118.5604221528582372, -0.6894197161374837624 ) ) ;
#29623=CARTESIAN_POINT ( 'NONE',  ( 3.205191379615736746, -14.47393913169138102, 3.051678166811226500 ) ) ;
#29624=CARTESIAN_POINT ( 'NONE',  ( -5.652088634484938368, 31.23120021444162475, -0.6296991705779479975 ) ) ;
#29625=CARTESIAN_POINT ( 'NONE',  ( 0.6395209782508930463, 120.9735524437166561, -0.05055770394172658805 ) ) ;
#29627=CARTESIAN_POINT ( 'NONE',  ( -3.155498692175132458, 108.3452252202363724, 4.146548619333099595 ) ) ;
#29628=FACE_OUTER_BOUND ( 'NONE', #41887, .T. ) ;
#29630=CARTESIAN_POINT ( 'NONE',  ( -5.019283203953386341, 117.3993836733805693, 0.7004435676391351784 ) ) ;
#29631=CARTESIAN_POINT ( 'NONE',  ( 9.807059279559947385, 117.9968303279965340, 0.1034500883390726267 ) ) ;
#29632=CARTESIAN_POINT ( 'NONE',  ( -5.270289556066668268, 116.2365830367532595, 0.9655167061512666127 ) ) ;
#29633=CARTESIAN_POINT ( 'NONE',  ( -0.4045686510384880474, 118.1564795008688407, 0.9043423984889817913 ) ) ;
#29634=CARTESIAN_POINT ( 'NONE',  ( -5.008552712180506461, 117.3993836135855560, 0.7755994290793736257 ) ) ;
#29635=CARTESIAN_POINT ( 'NONE',  ( 2.241275201495271929, 37.45550410866057689, -1.120274590453292030 ) ) ;
#29636=CARTESIAN_POINT ( 'NONE',  ( 6.881618033700585890, 158.0090104422344268, 1.782742279240755678 ) ) ;
#29638=CARTESIAN_POINT ( 'NONE',  ( 1.653223041919489544, 21.06826514481450729, 4.324967054831568625 ) ) ;
#29639=CARTESIAN_POINT ( 'NONE',  ( 7.747546812250076798, -14.76477644359806973, -3.309085904616556384 ) ) ;
#29640=CARTESIAN_POINT ( 'NONE',  ( -5.484865810345498360, 117.1958023522216337, -0.7988316295375470499 ) ) ;
#29641=CARTESIAN_POINT ( 'NONE',  ( -1.417747896749580017, 115.2915405621345144, -1.855271064302983053 ) ) ;
#29644=CARTESIAN_POINT ( 'NONE',  ( 2.144155271412940156, 104.6144662015412905, 4.896541268869996522 ) ) ;
#29645=CARTESIAN_POINT ( 'NONE',  ( -1.471791394198959102, 24.03230288535706549, 4.399545648925609065 ) ) ;
#29648=CARTESIAN_POINT ( 'NONE',  ( 2.917951099372082080, -14.56804730652265434, 4.441407531948645904 ) ) ;
#29649=CARTESIAN_POINT ( 'NONE',  ( 1.667199326422575512, 119.8612358676174949, -0.5251152081720655840 ) ) ;
#29650=CARTESIAN_POINT ( 'NONE',  ( -17.93297959639536288, 125.1504969321615164, 0.5028613125471301792 ) ) ;
#29651=CARTESIAN_POINT ( 'NONE',  ( 4.801298031305056391, 117.4006795940419892, -1.015947262250491478 ) ) ;
#29654=VERTEX_POINT ( 'NONE', #18781 ) ;
#29655=CARTESIAN_POINT ( 'NONE',  ( 5.552702978602249040, -15.16724029374752547, 2.010675452401557095 ) ) ;
#29656=CARTESIAN_POINT ( 'NONE',  ( -19.62644950592621385, 149.4594839399872512, 1.701416438606882187 ) ) ;
#29657=CARTESIAN_POINT ( 'NONE',  ( 14.62453491845899833, 121.8773232776577942, -0.9418922607927827650 ) ) ;
#29658=CARTESIAN_POINT ( 'NONE',  ( -4.515506726787251068, -6.291224493951820484, 1.111903093310195212 ) ) ;
#29659=LINE ( 'NONE', #3905, #42007 ) ;
#29662=CARTESIAN_POINT ( 'NONE',  ( 0.7406220848564354364, 119.3684187487962305, 0.7644009012486649990 ) ) ;
#29663=CARTESIAN_POINT ( 'NONE',  ( -3.430652046320729731, 156.3978305292817481, 1.152991164011112568 ) ) ;
#29666=CARTESIAN_POINT ( 'NONE',  ( 17.48755558824488787, 140.3598469681121514, -1.687825538285184557 ) ) ;
#29667=CARTESIAN_POINT ( 'NONE',  ( -20.88630183647693173, 148.3608207065297222, -2.399927473325582650 ) ) ;
#29669=ORIENTED_EDGE ( 'NONE', *, *, #19359, .T. ) ;
#29670=CARTESIAN_POINT ( 'NONE',  ( 4.478503255188988952, 118.1112075284179923, -0.5788684376435218049 ) ) ;
#29671=CARTESIAN_POINT ( 'NONE',  ( 1.553919893302579958, 120.7289827521893670, -0.2132023499116272869 ) ) ;
#29673=CARTESIAN_POINT ( 'NONE',  ( -2.063908814988777873, 157.0334531201187644, -1.539797002863052988 ) ) ;
#29674=CARTESIAN_POINT ( 'NONE',  ( 1.977593594988821479, -15.25598227308876176, 5.283756247048868815 ) ) ;
#29675=FACE_OUTER_BOUND ( 'NONE', #29879, .T. ) ;
#29677=CARTESIAN_POINT ( 'NONE',  ( 1.100877510726109954, 5.750359496286542971, -4.487862572965156005 ) ) ;
#29678=CARTESIAN_POINT ( 'NONE',  ( 3.458815983099534197, 120.0787590019544098, 0.7189451402107608358 ) ) ;
#29679=CARTESIAN_POINT ( 'NONE',  ( -3.151918684035726947, 30.94949030248789867, -0.3028545185056354394 ) ) ;
#29680=CARTESIAN_POINT ( 'NONE',  ( -3.789191232057584902, 13.46218022696137773, 2.646434746401360893 ) ) ;
#29681=CARTESIAN_POINT ( 'NONE',  ( 11.10900461081871704, 128.0707465396788507, 0.3225556591789271454 ) ) ;
#29684=CARTESIAN_POINT ( 'NONE',  ( 2.184895159611915716, 116.1856596408759970, 0.02067325796152543957 ) ) ;
#29685=CARTESIAN_POINT ( 'NONE',  ( 22.46755768833288158, 150.8526571111528654, 0.4489552724284878171 ) ) ;
#29687=FACE_OUTER_BOUND ( 'NONE', #31798, .T. ) ;
#29691=CARTESIAN_POINT ( 'NONE',  ( -6.654617103318593247E-14, 104.6144662015457243, 1.534725424433578570E-31 ) ) ;
#29695=CARTESIAN_POINT ( 'NONE',  ( -20.30088961563517458, 128.9598305440861452, -0.1271185223121272523 ) ) ;
#29698=CARTESIAN_POINT ( 'NONE',  ( -7.793677643169202973, 122.5633063490366084, -0.3701003583587130774 ) ) ;
#29701=CARTESIAN_POINT ( 'NONE',  ( -10.40089755570045149, 153.1126597504080280, -0.2539288847195827481 ) ) ;
#29702=CARTESIAN_POINT ( 'NONE',  ( 2.112423120037338453, -15.42067558999450583, 5.959086572354191702 ) ) ;
#29703=CARTESIAN_POINT ( 'NONE',  ( -7.037849409249396615, 158.0922581832940921, 1.451942896407524497 ) ) ;
#29704=CARTESIAN_POINT ( 'NONE',  ( 2.889066315880882030, 25.55657059589919911, 3.609430016826872478 ) ) ;
#29705=CARTESIAN_POINT ( 'NONE',  ( 3.269635511691603380, 159.4655167044000166, 0.2664280249078423424 ) ) ;
#29706=FACE_OUTER_BOUND ( 'NONE', #28413, .T. ) ;
#29708=CARTESIAN_POINT ( 'NONE',  ( 0.9436028068379492817, -1.428137797730904879, 0.2459283266283248115 ) ) ;
#29709=CARTESIAN_POINT ( 'NONE',  ( -3.288660796955225951, 159.4686222989141697, -0.1587487428767532793 ) ) ;
#29712=CARTESIAN_POINT ( 'NONE',  ( -2.264966102306270379, 116.3304222186488772, 0.1531678969014962921 ) ) ;
#29714=CARTESIAN_POINT ( 'NONE',  ( -3.856066505249651222, 156.9018388488748883, 1.546468145409084061 ) ) ;
#29716=CARTESIAN_POINT ( 'NONE',  ( 13.04750228320297367, 121.1598417376693533, 1.575122625318853053 ) ) ;
#29717=CARTESIAN_POINT ( 'NONE',  ( 12.38900849369184520, 122.4057692182592092, -1.312116060471626211 ) ) ;
#29718=CARTESIAN_POINT ( 'NONE',  ( -0.7897743334665792148, -0.9462621144725560374, 0.5691593732151654095 ) ) ;
#29719=CARTESIAN_POINT ( 'NONE',  ( -7.361208496634311871, 158.3992165788449711, -1.430753602065345076 ) ) ;
#29720=AXIS2_PLACEMENT_3D ( 'NONE', #25780, #22568, #6006 ) ;
#29721=CARTESIAN_POINT ( 'NONE',  ( 4.618524016831645262, 118.0632027795112862, -0.5485634799004409645 ) ) ;
#29722=CARTESIAN_POINT ( 'NONE',  ( -6.606344270946872901E-14, 95.34346620154573770, 1.014423412895214384E-29 ) ) ;
#29723=CARTESIAN_POINT ( 'NONE',  ( 16.07945855365731092, 143.8376908863262997, -0.9680047772055856425 ) ) ;
#29724=CARTESIAN_POINT ( 'NONE',  ( -1.617373050801775625, 120.9968702744464366, -0.03231896268895501773 ) ) ;
#29726=CARTESIAN_POINT ( 'NONE',  ( -5.834672723501299174, 119.9178398404649926, -1.129903066036337833 ) ) ;
#29727=CARTESIAN_POINT ( 'NONE',  ( 5.310739065812000170, -15.29705283487872691, 0.1354967992945097788 ) ) ;
#29730=CARTESIAN_POINT ( 'NONE',  ( -4.542182964463529871, 118.0343140766884034, -0.8604455232648324792 ) ) ;
#29735=CARTESIAN_POINT ( 'NONE',  ( 16.01586142131289492, 150.9843922791743296, 2.313278988710850914 ) ) ;
#29736=CARTESIAN_POINT ( 'NONE',  ( -5.208855653336853742, 31.38455280743060527, -0.6720767434146609487 ) ) ;
#29737=CARTESIAN_POINT ( 'NONE',  ( 3.302029177305205732, 159.4671159221996959, 0.06598240135525389183 ) ) ;
#29738=CARTESIAN_POINT ( 'NONE',  ( -4.036547470782467784, 117.2022048034790487, 0.8857695023546175994 ) ) ;
#29739=CARTESIAN_POINT ( 'NONE',  ( 7.747546812250076798, -14.76477644359806973, -3.309085904616556384 ) ) ;
#29740=CARTESIAN_POINT ( 'NONE',  ( 12.37067103324079476, 130.6617397222824479, 0.9131297178954279614 ) ) ;
#29741=ADVANCED_FACE ( 'NONE', ( #15797 ), #9417, .F. ) ;
#29742=CARTESIAN_POINT ( 'NONE',  ( 14.14567801931314328, 120.5239346615589540, -0.5295366371686059948 ) ) ;
#29743=CARTESIAN_POINT ( 'NONE',  ( 5.327964288879288191, 105.1224761950569331, -0.2707926473889318286 ) ) ;
#29745=CARTESIAN_POINT ( 'NONE',  ( 5.535770207902783291, -15.30306967536979457, -0.4932718738389492708 ) ) ;
#29747=CARTESIAN_POINT ( 'NONE',  ( -15.54847974360328067, 120.7212560704218589, -0.2938029371637448928 ) ) ;
#29750=CARTESIAN_POINT ( 'NONE',  ( -6.728599971069020746, 121.0446882272744489, -0.9798701814483349315 ) ) ;
#29752=CARTESIAN_POINT ( 'NONE',  ( -15.44350913713192064, 147.8441550597069352, -0.7585189891071871804 ) ) ;
#29753=CARTESIAN_POINT ( 'NONE',  ( 3.873131646279637241, -11.92617534808754165, 0.9134907789774980857 ) ) ;
#29754=CARTESIAN_POINT ( 'NONE',  ( -20.10769848529519166, 132.0867704272472452, 0.9164310550120231547 ) ) ;
#29756=CARTESIAN_POINT ( 'NONE',  ( 10.82257311662882948, 157.9086237439880733, 0.2761350859956696047 ) ) ;
#29758=CARTESIAN_POINT ( 'NONE',  ( 4.574821423538755205, -2.080616851812391310, 0.6590154617212384824 ) ) ;
#29760=FACE_OUTER_BOUND ( 'NONE', #3572, .T. ) ;
#29763=CIRCLE ( 'NONE', #5962, 5.080000000000006288 ) ;
#29764=CARTESIAN_POINT ( 'NONE',  ( -8.106797866231710614, 121.1670163920446157, 0.9708022562603837446 ) ) ;
#29766=CARTESIAN_POINT ( 'NONE',  ( -3.632229383214316876, 17.08265688572556584, -2.901706292871565562 ) ) ;
#29767=CARTESIAN_POINT ( 'NONE',  ( 14.69745991766241033, 121.6338672040446767, 1.430666218478179763 ) ) ;
#29768=CARTESIAN_POINT ( 'NONE',  ( 15.70103477329399766, 145.5797129992483292, 0.3137440411564567100 ) ) ;
#29770=CARTESIAN_POINT ( 'NONE',  ( 17.34031924846174988, 128.5728276651957742, -1.378292450406111147 ) ) ;
#29771=CARTESIAN_POINT ( 'NONE',  ( 2.901706292870370518, -4.507343114274551255, -3.632229383212865592 ) ) ;
#29772=CARTESIAN_POINT ( 'NONE',  ( -18.04579964447635376, 154.0913862843578670, -1.474566393615006632 ) ) ;
#29775=CARTESIAN_POINT ( 'NONE',  ( -0.004910621514806326471, 156.3161161488371533, 0.2457475809811482670 ) ) ;
#29776=CARTESIAN_POINT ( 'NONE',  ( 6.098373624802439608, -13.52034412102339012, 1.767782016118699895 ) ) ;
#29778=AXIS2_PLACEMENT_3D ( 'NONE', #21993, #24561, #37565 ) ;
#29779=CARTESIAN_POINT ( 'NONE',  ( 3.212496809824684441, -14.25148094350509353, 2.370051959060230473 ) ) ;
#29781=CARTESIAN_POINT ( 'NONE',  ( 6.675970744194591688, 119.4737997143703012, 1.289985488916530310 ) ) ;
#29784=CARTESIAN_POINT ( 'NONE',  ( -7.717559979892335775, 158.5863655655865330, 0.7470610436598877913 ) ) ;
#29785=CARTESIAN_POINT ( 'NONE',  ( -6.181412921142831252, 19.34218365691531361, 5.729511908899769246 ) ) ;
#29786=CARTESIAN_POINT ( 'NONE',  ( 9.210551279805565983, 123.0263237342149978, 1.033454686166954239 ) ) ;
#29787=CARTESIAN_POINT ( 'NONE',  ( 10.74909004363686194, 157.9381345072164038, -0.1376009798949087704 ) ) ;
#29791=CARTESIAN_POINT ( 'NONE',  ( -3.403764228135175429, 117.9394517900196888, 1.153273866709463302 ) ) ;
#29794=CARTESIAN_POINT ( 'NONE',  ( -4.415952317727478871, 118.1645917943391169, 0.4804988017228924990 ) ) ;
#29798=CARTESIAN_POINT ( 'NONE',  ( -3.946513987435433357, 118.7629491485454309, -1.103369079102947348 ) ) ;
#29799=CARTESIAN_POINT ( 'NONE',  ( -6.098125870537236537, 119.5354672635397719, -1.256037220562212786 ) ) ;
#29801=CARTESIAN_POINT ( 'NONE',  ( -5.349033702192389050, 117.2069880336854197, -0.8964318704791015557 ) ) ;
#29802=CARTESIAN_POINT ( 'NONE',  ( 4.503537194581884506, 118.0666071354895053, 0.8214503418453174000 ) ) ;
#29803=CARTESIAN_POINT ( 'NONE',  ( 0.005430166084267442142, 120.5648899400503069, -0.2717477157510628794 ) ) ;
#29805=CARTESIAN_POINT ( 'NONE',  ( -0.6068508678446015159, 115.7030933504832149, -1.759829434126405356 ) ) ;
#29806=CARTESIAN_POINT ( 'NONE',  ( 3.341374452869265710, 118.1651003929687960, -0.6417180735543650538 ) ) ;
#29807=FACE_OUTER_BOUND ( 'NONE', #37844, .T. ) ;
#29808=CARTESIAN_POINT ( 'NONE',  ( -16.88761465400188300, 147.3835828867039766, -1.922606999130501260 ) ) ;
#29809=CARTESIAN_POINT ( 'NONE',  ( -0.003550357976012296669, 159.5989787797044812, 0.1776744311461875836 ) ) ;
#29810=CARTESIAN_POINT ( 'NONE',  ( 7.886551735269857311, 122.1946728851203261, -0.4945421293698765153 ) ) ;
#29811=CARTESIAN_POINT ( 'NONE',  ( -8.982416536893675030, 124.0550639507465291, -0.09049447817662507887 ) ) ;
#29813=CARTESIAN_POINT ( 'NONE',  ( -3.416230376366909294, -5.529048218071860532, 3.121479803864907865 ) ) ;
#29814=CARTESIAN_POINT ( 'NONE',  ( 3.159869787290094933, 159.3937097445585778, 0.6918644357365444364 ) ) ;
#29815=CARTESIAN_POINT ( 'NONE',  ( 4.780953720317446809, 104.6144662015457669, -0.7304112483795474065 ) ) ;
#29816=CARTESIAN_POINT ( 'NONE',  ( 3.275654002680270960, -14.73162568742410272, 0.7099577593494145189 ) ) ;
#29817=CARTESIAN_POINT ( 'NONE',  ( -14.75721126660351601, 152.8628051715174365, 1.735400109512247102 ) ) ;
#29818=CARTESIAN_POINT ( 'NONE',  ( -0.9353260110528880400, 8.126651709021682990, 0.2714574413461035007 ) ) ;
#29819=CARTESIAN_POINT ( 'NONE',  ( -18.48423909989039871, 154.1703991122031994, -0.9245180971295517969 ) ) ;
#29820=EDGE_CURVE ( 'NONE', #32583, #1712, #33899, .T. ) ;
#29821=CARTESIAN_POINT ( 'NONE',  ( 0.4636875340052978300, -8.988401195314681402, -0.8615772474383697199 ) ) ;
#29824=CARTESIAN_POINT ( 'NONE',  ( 0.6634819590975142845, 105.9515744484354371, 5.309451348557705508 ) ) ;
#29825=CARTESIAN_POINT ( 'NONE',  ( -16.15477348297523719, 145.8839827664328368, 0.6502963436359734395 ) ) ;
#29826=CARTESIAN_POINT ( 'NONE',  ( 2.954207113090831616, -14.52495373116942368, 5.111795949899043734 ) ) ;
#29827=CARTESIAN_POINT ( 'NONE',  ( 17.48603724727278674, 147.5992144370567871, -1.461888717290057871 ) ) ;
#29828=CARTESIAN_POINT ( 'NONE',  ( -12.32670121879468716, 122.4057692182592092, -1.805994760647165354 ) ) ;
#29830=CARTESIAN_POINT ( 'NONE',  ( 0.09871621325710944195, 104.6144662015456674, 4.835249534204173472 ) ) ;
#29831=CARTESIAN_POINT ( 'NONE',  ( 3.176652145978316355, -13.92691374863060183, 2.072386176210903486 ) ) ;
#29832=CARTESIAN_POINT ( 'NONE',  ( -4.916573287661055502, 117.5420315621613554, -1.049119472579290058 ) ) ;
#29833=CARTESIAN_POINT ( 'NONE',  ( 8.883181220021160840, 123.7004864364556909, 0.02116515827996235527 ) ) ;
#29835=CARTESIAN_POINT ( 'NONE',  ( -5.114121277772293084, 113.8198996839817454, 1.623722780927329135 ) ) ;
#29836=CARTESIAN_POINT ( 'NONE',  ( 1.769790122373364527, 106.3931338143381424, 5.031734874205501029 ) ) ;
#29838=CARTESIAN_POINT ( 'NONE',  ( 23.28495812418880462, 149.3453998935430604, 0.3112269551726871697 ) ) ;
#29839=CIRCLE ( 'NONE', #613, 5.080000000000006288 ) ;
#29840=CARTESIAN_POINT ( 'NONE',  ( -4.861212978143241159, 112.7561542417671916, 2.378900599183503051 ) ) ;
#29842=CARTESIAN_POINT ( 'NONE',  ( -2.015348138122511568, 118.7629491485454167, 1.152895576627283925 ) ) ;
#29844=CARTESIAN_POINT ( 'NONE',  ( 2.014642110472020242, 39.20946620154573026, -1.229996183391246944 ) ) ;
#29845=CARTESIAN_POINT ( 'NONE',  ( 13.38228307180514776, 122.0388263298542739, 1.742221313037096486 ) ) ;
#29846=CARTESIAN_POINT ( 'NONE',  ( -2.133573495637306916, 19.78131850274109382, 4.120466288703205748 ) ) ;
#29847=CARTESIAN_POINT ( 'NONE',  ( -5.323917895073306816, 23.39377214425099893, 6.572471397932490689 ) ) ;
#29848=CARTESIAN_POINT ( 'NONE',  ( 8.658313298994691820, 118.4528737239894269, -0.7179955298477456171 ) ) ;
#29849=CARTESIAN_POINT ( 'NONE',  ( -2.900991945634804114, 122.3314979878274045, -0.2533474610292539841 ) ) ;
#29852=CARTESIAN_POINT ( 'NONE',  ( -4.540852303063954487, 104.6144662015457243, 1.644315252756900714 ) ) ;
#29853=CARTESIAN_POINT ( 'NONE',  ( 1.893578447776079754, 19.08455809737888487, -4.224370802633358402 ) ) ;
#29855=CARTESIAN_POINT ( 'NONE',  ( -4.757346424997288103, 117.3993836135861386, -1.207075064218979810 ) ) ;
#29856=CARTESIAN_POINT ( 'NONE',  ( 2.576299636888586875, -14.89815494326314571, 4.769281578164155100 ) ) ;
#29857=CARTESIAN_POINT ( 'NONE',  ( 2.330098105383510809, 118.9955205646042344, -0.6366692849230544127 ) ) ;
#29858=CARTESIAN_POINT ( 'NONE',  ( -13.10540794497634565, 156.9444350391594014, 0.5617278846626186928 ) ) ;
#29864=CARTESIAN_POINT ( 'NONE',  ( 3.308369008328103433, -15.71782228035249673, 4.479361047165574483 ) ) ;
#29865=CARTESIAN_POINT ( 'NONE',  ( -18.88973499030882763, 150.3568762430427910, 1.706130117709411476 ) ) ;
#29866=CARTESIAN_POINT ( 'NONE',  ( 14.39412078427922914, 121.9874158357064857, -1.026313471838276481 ) ) ;
#29868=CARTESIAN_POINT ( 'NONE',  ( 4.636249899789679496, -11.37698174978397958, -0.2454043791197063895 ) ) ;
#29869=DIRECTION ( 'NONE',  ( -5.206863593109713661E-17, 1.000000000000000000, -1.077750396879097183E-30 ) ) ;
#29871=CARTESIAN_POINT ( 'NONE',  ( 2.958531772299236362, 39.20946620154573736, 1.329372033065076453 ) ) ;
#29872=CARTESIAN_POINT ( 'NONE',  ( 0.7524737301089851060, 120.0979018405971175, 0.6085003676253140092 ) ) ;
#29873=CARTESIAN_POINT ( 'NONE',  ( -13.78713281179563666, 131.0408573235120571, 1.173264656791310756 ) ) ;
#29874=CARTESIAN_POINT ( 'NONE',  ( -4.856515155028523267, 117.4075056128946386, -1.171047894592366356 ) ) ;
#29876=CARTESIAN_POINT ( 'NONE',  ( 17.21863486588922143, 149.7102054596878702, -1.666570748255499002 ) ) ;
#29877=CARTESIAN_POINT ( 'NONE',  ( -12.61233984701559407, 121.4495935343099688, -1.683034450629873557 ) ) ;
#29878=CARTESIAN_POINT ( 'NONE',  ( -6.045080874924777230E-14, 85.18346620154574111, 1.015827583860198862E-16 ) ) ;
#29879=EDGE_LOOP ( 'NONE', ( #6289, #32739, #34960, #10100 ) ) ;
#29880=CARTESIAN_POINT ( 'NONE',  ( 4.476806822841735034, 118.1289215581870877, -0.5424833475171277897 ) ) ;
#29881=CARTESIAN_POINT ( 'NONE',  ( 6.226794683659739427, 155.3658059236344684, -0.5518929715360436639 ) ) ;
#29883=CARTESIAN_POINT ( 'NONE',  ( 3.248418650160624033, -14.57852055173261618, 2.075358651653527620 ) ) ;
#29884=CARTESIAN_POINT ( 'NONE',  ( 3.794317479684171879, 105.1231002567820241, -3.763369276752646098 ) ) ;
#29886=CARTESIAN_POINT ( 'NONE',  ( 2.198398128136354934, 2.077049112184502278, 4.064154346441791965 ) ) ;
#29887=CARTESIAN_POINT ( 'NONE',  ( 16.92358334414607768, 148.6336825499269310, 2.141768463193927996 ) ) ;
#29888=CARTESIAN_POINT ( 'NONE',  ( -2.941155235503680743, 30.72646416932365909, -0.2232678871262771536 ) ) ;
#29889=CARTESIAN_POINT ( 'NONE',  ( 3.874746376330849618, 18.20996518813934628, -2.522041008920607563 ) ) ;
#29890=CARTESIAN_POINT ( 'NONE',  ( 15.53993717541241359, 147.5346097818530211, 0.5395553097850843693 ) ) ;
#29891=CARTESIAN_POINT ( 'NONE',  ( -0.3821431882137919511, 105.7852416002251204, 5.327472155929901199 ) ) ;
#29895=CARTESIAN_POINT ( 'NONE',  ( -2.175382718649831126, 116.2302060928067675, -0.1775962133206757110 ) ) ;
#29896=CARTESIAN_POINT ( 'NONE',  ( 3.682264917456191888, 104.1064662015457287, 0.07358041635424013294 ) ) ;
#29900=B_SPLINE_CURVE_WITH_KNOTS ( 'NONE', 3,
 ( #39663, #34320, #8744, #17896, #21292, #1738, #21706, #5774, #28333, #5148, #18103, #34528, #2582, #24491, #18728, #27702 ),
 .UNSPECIFIED., .F., .F.,
 ( 4, 2, 1, 1, 2, 2, 2, 2, 4 ),
 ( 0.000000000000000000, 0.06250000000000000000, 0.1250000000000000000, 0.2500000000000000000, 0.5000000000000000000, 0.6250000000000000000, 0.7500000000000000000, 0.8750000000000000000, 1.000000000000000000 ),
 .UNSPECIFIED. ) ;
#29902=DIRECTION ( 'NONE',  ( -0.9998004120163608288, 0.000000000000000000, -0.01997839162482749342 ) ) ;
#29905=CARTESIAN_POINT ( 'NONE',  ( -8.004298179822360026, 158.6817341734954425, 0.1651967042931135332 ) ) ;
#29908=CARTESIAN_POINT ( 'NONE',  ( -6.973042344651466884, 121.9479208601376286, -0.2102655371621303393 ) ) ;
#29910=CARTESIAN_POINT ( 'NONE',  ( -5.332935381406168851, 115.7029491485442634, -0.1065653510733624160 ) ) ;
#29911=CARTESIAN_POINT ( 'NONE',  ( -14.17736129766413100, 138.8817910697950140, -0.3341079978015792928 ) ) ;
#29912=CARTESIAN_POINT ( 'NONE',  ( 6.471342906213767066, -13.19865009487615559, 0.2853922585125314715 ) ) ;
#29913=CARTESIAN_POINT ( 'NONE',  ( -21.19479858968374941, 149.1058327099893290, 1.460163390594825028 ) ) ;
#29914=DIRECTION ( 'NONE',  ( -4.017660918040594346E-17, 1.000000000000000000, 2.376309959284834438E-19 ) ) ;
#29915=CARTESIAN_POINT ( 'NONE',  ( -0.003550357976009695018, 159.5989787797044812, 0.1776744311461876391 ) ) ;
#29916=CARTESIAN_POINT ( 'NONE',  ( 9.053714358506876891, 124.2128128113216121, 0.3155815647710615846 ) ) ;
#29917=CARTESIAN_POINT ( 'NONE',  ( 2.163044864548389956, 28.58015952483584954, -4.087059112497700042 ) ) ;
#29918=CARTESIAN_POINT ( 'NONE',  ( -0.3362158861861603287, -7.698726726604804504, -0.9163890413163552351 ) ) ;
#29919=CARTESIAN_POINT ( 'NONE',  ( 0.003550357975880899172, 159.5989787797044812, -0.1776744311461874171 ) ) ;
#29923=CARTESIAN_POINT ( 'NONE',  ( 2.196830523109587929, 116.2217898966666638, 0.1075589129066046312 ) ) ;
#29924=CARTESIAN_POINT ( 'NONE',  ( -2.165411683282754574, 157.1282018749678002, 1.500011447693321287 ) ) ;
#29926=CARTESIAN_POINT ( 'NONE',  ( 4.923251988582125982, 158.4862278396301178, 1.623903838676621580 ) ) ;
#29927=CARTESIAN_POINT ( 'NONE',  ( 14.84283187390155589, 125.6006210965460781, -1.448481940162723136 ) ) ;
#29928=CARTESIAN_POINT ( 'NONE',  ( 0.7725151586569730666, -15.29989167607388900, -0.5872501270430795506 ) ) ;
#29929=CARTESIAN_POINT ( 'NONE',  ( 0.02156508032615568615, 159.2730288250082538, -1.079204802879467406 ) ) ;
#29930=CARTESIAN_POINT ( 'NONE',  ( 4.656685402655694972, 118.0313236345014758, -0.5883047702015815617 ) ) ;
#29932=CARTESIAN_POINT ( 'NONE',  ( 16.33516936551314558, 148.1602266505728380, -1.109112510451941702 ) ) ;
#29933=CARTESIAN_POINT ( 'NONE',  ( -7.552512487614272629, 122.4261604937442485, -0.1509171734833087142 ) ) ;
#29935=CARTESIAN_POINT ( 'NONE',  ( -12.63334184343655586, 124.0847267554996591, -1.843480660383216563 ) ) ;
#29936=CARTESIAN_POINT ( 'NONE',  ( 4.901850132730561249, -15.30225767492697564, -0.5056678198325348372 ) ) ;
#29938=CARTESIAN_POINT ( 'NONE',  ( -4.642601932456255298, 117.9634981682017383, -0.9174702582142799656 ) ) ;
#29940=CARTESIAN_POINT ( 'NONE',  ( 4.105367864036007397, 118.2429491485453354, 0.3529617804329867603 ) ) ;
#29941=CARTESIAN_POINT ( 'NONE',  ( 12.85862358090719404, 153.8477531742089468, 2.225956515383983092 ) ) ;
#29943=CARTESIAN_POINT ( 'NONE',  ( 8.217147260422391852, 117.5004391570743394, 0.1493243188240319652 ) ) ;
#29944=CARTESIAN_POINT ( 'NONE',  ( 5.540715274600516160, 6.338079305180906786, 6.343128766557815545 ) ) ;
#29945=CARTESIAN_POINT ( 'NONE',  ( 9.627236290563381260, 124.2480737032941533, 0.7173579674491836755 ) ) ;
#29946=CARTESIAN_POINT ( 'NONE',  ( 9.536130858165876134, 118.4542681464805298, -0.5810392422064987183 ) ) ;
#29947=EDGE_CURVE ( 'NONE', #5326, #16499, #2366, .T. ) ;
#29949=ORIENTED_EDGE ( 'NONE', *, *, #8453, .F. ) ;
#29950=CARTESIAN_POINT ( 'NONE',  ( 0.7729263974008259153, 115.6909491485452719, 1.757288066092038914 ) ) ;
#29951=CARTESIAN_POINT ( 'NONE',  ( -2.757293845589700698, 116.5489981622532127, 0.01971897987843778538 ) ) ;
#29953=CARTESIAN_POINT ( 'NONE',  ( 5.365375985982141493, 120.5163311419836134, -0.5829208649569685985 ) ) ;
#29954=CARTESIAN_POINT ( 'NONE',  ( -8.675687895398477067, 118.3610464811752081, 0.6699752535086661576 ) ) ;
#29955=CARTESIAN_POINT ( 'NONE',  ( 0.003052472355820575779, 120.8426702770480148, -0.1527581987772197447 ) ) ;
#29956=CARTESIAN_POINT ( 'NONE',  ( 4.137648320759505616, -13.26899632091267733, 3.249298663494996298 ) ) ;
#29957=CARTESIAN_POINT ( 'NONE',  ( -22.12005076447816876, 142.1041199125429557, 1.010629163944517739 ) ) ;
#29959=CARTESIAN_POINT ( 'NONE',  ( 0.8904708500336536714, 116.4394364983335493, 0.05634004476769405995 ) ) ;
#29961=ORIENTED_EDGE ( 'NONE', *, *, #15150, .F. ) ;
#29962=CARTESIAN_POINT ( 'NONE',  ( 4.224370802630715183, -2.505441902618962935, 1.893578447770203566 ) ) ;
#29963=CARTESIAN_POINT ( 'NONE',  ( 5.326133827267389265, 105.1224662015456772, 0.4469431379364897094 ) ) ;
#29964=DIRECTION ( 'NONE',  ( 0.9998004120163608288, 0.000000000000000000, 0.01997839162482762526 ) ) ;
#29966=CARTESIAN_POINT ( 'NONE',  ( 8.032877371522001653, 121.3111410846650244, 1.249454745935258071 ) ) ;
#29967=CARTESIAN_POINT ( 'NONE',  ( -4.449009123739010363, -11.09185097514761331, -1.246716907482375847 ) ) ;
#29968=CARTESIAN_POINT ( 'NONE',  ( 22.31562366552497068, 146.3189071340513294, 1.902122558187540280 ) ) ;
#29971=CARTESIAN_POINT ( 'NONE',  ( 11.66006228966214486, 156.3395478113760362, -1.582478695429108129 ) ) ;
#29972=CARTESIAN_POINT ( 'NONE',  ( -1.290833045837797455, 0.8901568857254957834, 4.466177308409287505 ) ) ;
#29973=CARTESIAN_POINT ( 'NONE',  ( -20.52999062792650165, 132.2049894596293313, -1.489094535601872993 ) ) ;
#29975=ORIENTED_EDGE ( 'NONE', *, *, #27204, .F. ) ;
#29976=CARTESIAN_POINT ( 'NONE',  ( -0.6667004703452847902, 156.3175253132196190, 0.2457982560305636555 ) ) ;
#29977=CARTESIAN_POINT ( 'NONE',  ( 5.913917015499376539, -14.05268412609835060, 2.470677959447274308 ) ) ;
#29980=B_SPLINE_CURVE_WITH_KNOTS ( 'NONE', 3,
 ( #36510, #1156, #24128, #30945, #21129, #11141 ),
 .UNSPECIFIED., .F., .F.,
 ( 4, 2, 4 ),
 ( 0.000000000000000000, 0.5000000000000000000, 0.5009815572441199683 ),
 .UNSPECIFIED. ) ;
#29983=CARTESIAN_POINT ( 'NONE',  ( 12.11054887026057081, 155.0146010091537221, 2.232606363771872715 ) ) ;
#29984=CARTESIAN_POINT ( 'NONE',  ( -4.883848590450072358, 117.7607009110569862, 0.7127853619805604168 ) ) ;
#29986=CARTESIAN_POINT ( 'NONE',  ( -22.60445334873329415, 148.5212373274837319, 0.8566365145943201087 ) ) ;
#29987=CARTESIAN_POINT ( 'NONE',  ( 6.778223571145144177, 14.38247674671404752, -5.057098040585858989 ) ) ;
#29989=CARTESIAN_POINT ( 'NONE',  ( 10.17133788503921110, 124.0743415861677903, 1.120692231141951156 ) ) ;
#29990=FACE_OUTER_BOUND ( 'NONE', #34748, .T. ) ;
#29991=CARTESIAN_POINT ( 'NONE',  ( 15.13173320725175763, 120.7387302883610118, -0.2100629019518969742 ) ) ;
#29996=CARTESIAN_POINT ( 'NONE',  ( 2.483772768628635497, 106.8193809087893271, -4.725234424128872845 ) ) ;
#29999=CARTESIAN_POINT ( 'NONE',  ( -4.459999047083514689, 118.1598764511204536, 0.4313593223247962349 ) ) ;
#30004=CARTESIAN_POINT ( 'NONE',  ( -3.682509200627861468, 118.8507421139248379, -0.9352261960797142448 ) ) ;
#30005=CARTESIAN_POINT ( 'NONE',  ( -4.381926848744128300, 111.2539628214143903, -3.135495374750700392 ) ) ;
#30007=CARTESIAN_POINT ( 'NONE',  ( 4.451861420862569751, 118.1112095268316011, 0.7573049349207229275 ) ) ;
#30008=CARTESIAN_POINT ( 'NONE',  ( -0.5945828676176249106, 120.5739061664170606, -0.2962085107056580680 ) ) ;
#30009=CARTESIAN_POINT ( 'NONE',  ( -1.214571177347494313, 115.7029375466994736, -1.741462126173494385 ) ) ;
#30010=CARTESIAN_POINT ( 'NONE',  ( 1.005691866306313464, 118.1651004085809831, -0.8396654685810295282 ) ) ;
#30011=CARTESIAN_POINT ( 'NONE',  ( 5.434281097240408087, 117.1681999988027911, -0.6838767007579789059 ) ) ;
#30012=CARTESIAN_POINT ( 'NONE',  ( -5.844382469225037902, 120.7327493588883840, -0.8888191899821258346 ) ) ;
#30014=CARTESIAN_POINT ( 'NONE',  ( -0.002459401150367294953, 159.6023738651833810, 0.1230784904792620454 ) ) ;
#30015=CARTESIAN_POINT ( 'NONE',  ( 8.348968351561811829, 120.0002459142761921, -1.116349756213213640 ) ) ;
#30016=CARTESIAN_POINT ( 'NONE',  ( -4.205176885578073787, 155.8715900735512605, 0.01157140856383978393 ) ) ;
#30017=CARTESIAN_POINT ( 'NONE',  ( 5.008145224984434485, 117.3993836135855418, -0.7758584094373792706 ) ) ;
#30018=CARTESIAN_POINT ( 'NONE',  ( 10.49915001570426476, 157.9057380314836223, 0.9855651801815568103 ) ) ;
#30020=CARTESIAN_POINT ( 'NONE',  ( 2.678036876842718517, -15.12020262989130437, 4.533791366373512766 ) ) ;
#30021=CARTESIAN_POINT ( 'NONE',  ( -12.95103886519486558, 123.9867020804889961, 1.362965731555215054 ) ) ;
#30022=CARTESIAN_POINT ( 'NONE',  ( -0.4041098725243945644, -13.24273492701920141, -0.8882236940730178221 ) ) ;
#30023=CARTESIAN_POINT ( 'NONE',  ( -16.70755423740151713, 155.2649736186859570, -0.8698744534657079086 ) ) ;
#30024=CARTESIAN_POINT ( 'NONE',  ( -0.5845540250341307864, -7.254922367050685494, -0.7839501960785225654 ) ) ;
#30028=CARTESIAN_POINT ( 'NONE',  ( 3.975629016401896809, 111.5999093057820772, 3.028662833142258037 ) ) ;
#30029=CARTESIAN_POINT ( 'NONE',  ( -5.210205730215736963, 121.0352659167314755, 0.3424523703800272934 ) ) ;
#30030=CARTESIAN_POINT ( 'NONE',  ( 2.939725130288969979, -14.94165859211278580, 5.651657094137466864 ) ) ;
#30031=CARTESIAN_POINT ( 'NONE',  ( 17.81274246965180197, 147.0764175921665640, -1.531068679518140518 ) ) ;
#30032=CARTESIAN_POINT ( 'NONE',  ( -15.73670139478164387, 128.5598958631237565, -2.193363351549679319 ) ) ;
#30033=CARTESIAN_POINT ( 'NONE',  ( -2.049604525191627502, 104.6144662015457243, 4.378607431551252205 ) ) ;
#30034=AXIS2_PLACEMENT_3D ( 'NONE', #19635, #3487, #38213 ) ;
#30035=CARTESIAN_POINT ( 'NONE',  ( 3.162791966164926638, -14.44121541014482801, 3.416220915275241854 ) ) ;
#30036=CARTESIAN_POINT ( 'NONE',  ( -4.784543075752243801, 117.4060574113812265, -1.200192385861798883 ) ) ;
#30037=CARTESIAN_POINT ( 'NONE',  ( 9.177823364990439714, 124.0935018032023436, 0.02293427522457985521 ) ) ;
#30038=EDGE_LOOP ( 'NONE', ( #34557, #11207, #14896, #6679 ) ) ;
#30039=ADVANCED_FACE ( 'NONE', ( #37095 ), #36827, .F. ) ;
#30040=EDGE_CURVE ( 'NONE', #2591, #17780, #6965, .T. ) ;
#30041=CARTESIAN_POINT ( 'NONE',  ( -5.150313346575406293, 114.9389534560005472, 1.533160836946849459 ) ) ;
#30042=CARTESIAN_POINT ( 'NONE',  ( 3.279000889525665485, 108.1634925278680868, 4.199033572238965561 ) ) ;
#30044=CARTESIAN_POINT ( 'NONE',  ( 0.7701797417504300247, 117.3993836066060226, 1.486317275820449257 ) ) ;
#30046=CARTESIAN_POINT ( 'NONE',  ( 23.33610279681219879, 149.0590277239482475, 0.3121099645145855028 ) ) ;
#30051=CARTESIAN_POINT ( 'NONE',  ( 1.877814291165026628, -15.55177680042434041, 5.422881654991738465 ) ) ;
#30053=CARTESIAN_POINT ( 'NONE',  ( 7.783141725463699423, 119.0983413489662297, 1.312215641098252172 ) ) ;
#30055=CARTESIAN_POINT ( 'NONE',  ( 6.775881838314501415, 16.25650946394821617, 5.045332117489572887 ) ) ;
#30056=CARTESIAN_POINT ( 'NONE',  ( -5.497210702263359394, 117.7329109126123967, -1.024491283099325356 ) ) ;
#30057=CARTESIAN_POINT ( 'NONE',  ( -2.331513492273154853, 111.1666841684333633, -3.236375129800145967 ) ) ;
#30060=CARTESIAN_POINT ( 'NONE',  ( -2.565436166410399288, 107.6373832812085425, -4.562490956761092953 ) ) ;
#30061=CARTESIAN_POINT ( 'NONE',  ( -4.815265214305837205, 105.1215022376130150, 2.303391734824050463 ) ) ;
#30062=CIRCLE ( 'NONE', #10337, 1.000000000000000000 ) ;
#30063=CARTESIAN_POINT ( 'NONE',  ( -3.426874451426485724, 1.805113900313119357, -3.130497002818263930 ) ) ;
#30066=CARTESIAN_POINT ( 'NONE',  ( 1.985452195540454934, -15.12483337350742296, 5.348831821476924375 ) ) ;
#30067=CARTESIAN_POINT ( 'NONE',  ( 5.575611629171946859, 123.3023672762779910, 0.03632235649590544874 ) ) ;
#30068=CARTESIAN_POINT ( 'NONE',  ( -22.99243123797629096, 146.5883926500602001, 0.5216133500896585895 ) ) ;
#30072=ORIENTED_EDGE ( 'NONE', *, *, #30873, .F. ) ;
#30073=CARTESIAN_POINT ( 'NONE',  ( -3.151918684035726947, 30.94949030248789157, -0.3028545185056354394 ) ) ;
#30074=CARTESIAN_POINT ( 'NONE',  ( 5.204094786718133747, -15.42339607600888485, 1.288180339967581967 ) ) ;
#30075=CARTESIAN_POINT ( 'NONE',  ( -7.743227489916900907, 119.4405053107883958, 1.058161572703685938 ) ) ;
#30076=CARTESIAN_POINT ( 'NONE',  ( 4.349802767100347189, -10.92635770930747796, -1.576909098649299512 ) ) ;
#30079=CARTESIAN_POINT ( 'NONE',  ( 1.682799138809720096, 120.1914007830323214, 0.5335993566373052888 ) ) ;
#30080=CARTESIAN_POINT ( 'NONE',  ( -1.968159265821259218, 156.7095495334699535, 1.232728320231047059 ) ) ;
#30081=CARTESIAN_POINT ( 'NONE',  ( 0.3680926247507866900, 118.1564734711614904, 0.9197955535796807913 ) ) ;
#30082=AXIS2_PLACEMENT_3D ( 'NONE', #8795, #35002, #2417 ) ;
#30083=CARTESIAN_POINT ( 'NONE',  ( 8.398523874639428399, 120.8878392079396065, -1.065324388190682647 ) ) ;
#30084=CARTESIAN_POINT ( 'NONE',  ( -20.26628159282173414, 149.4216517587604756, -2.427422966980313124 ) ) ;
#30086=ORIENTED_EDGE ( 'NONE', *, *, #21990, .T. ) ;
#30087=CARTESIAN_POINT ( 'NONE',  ( 4.118047298989734095, 118.2429491485453354, -0.1865688736171002005 ) ) ;
#30088=EDGE_CURVE ( 'NONE', #30817, #36646, #2154, .T. ) ;
#30089=CARTESIAN_POINT ( 'NONE',  ( 15.99593626731837048, 146.6619865182943272, -0.4079709740032105847 ) ) ;
#30091=CARTESIAN_POINT ( 'NONE',  ( 3.065366080762625955, -14.95244456720379311, 3.762810261076596330 ) ) ;
#30092=CARTESIAN_POINT ( 'NONE',  ( -1.828502361677136534, 105.1241263439060418, -5.020304316456576821 ) ) ;
#30093=AXIS2_PLACEMENT_3D ( 'NONE', #31310, #18944, #34321 ) ;
#30095=CARTESIAN_POINT ( 'NONE',  ( -4.623654898565560778, 8.549082320728111029, 0.09932813335659773646 ) ) ;
#30096=CARTESIAN_POINT ( 'NONE',  ( 10.57849499609981514, 123.4307455932968765, 1.421577474458307400 ) ) ;
#30097=CARTESIAN_POINT ( 'NONE',  ( 2.933835436169716537, 38.64483070579829871, -0.5563684569531323065 ) ) ;
#30099=CARTESIAN_POINT ( 'NONE',  ( -3.453265078539333288, 21.00871511114837276, -3.102408547967784092 ) ) ;
#30100=CARTESIAN_POINT ( 'NONE',  ( 9.115475939616047185, 153.9201329141909866, 0.2944159349489394728 ) ) ;
#30104=CARTESIAN_POINT ( 'NONE',  ( 2.170524884126211251, 116.2984658183265623, -0.1645159270875201085 ) ) ;
#30109=CARTESIAN_POINT ( 'NONE',  ( 8.218723488459346527, -2.309819447571417772, 1.932697321913255717 ) ) ;
#30113=FACE_OUTER_BOUND ( 'NONE', #8551, .T. ) ;
#30114=CARTESIAN_POINT ( 'NONE',  ( -1.406537315630193463, 159.5914066142653098, 0.2310332007158444334 ) ) ;
#30117=CARTESIAN_POINT ( 'NONE',  ( -7.788296088720038313, 122.5980079112661940, -0.2833033014985410492 ) ) ;
#30119=CARTESIAN_POINT ( 'NONE',  ( 3.646513112444593752, 115.7029492782878037, -1.479418030874811052 ) ) ;
#30120=CARTESIAN_POINT ( 'NONE',  ( -10.40832821182528001, 153.0987333575537548, -0.3246753324606910796 ) ) ;
#30121=CARTESIAN_POINT ( 'NONE',  ( 6.419191409189793696, -13.32337952207179832, 0.5587850172365541601 ) ) ;
#30122=CARTESIAN_POINT ( 'NONE',  ( -21.09608681602927760, 148.7375953542188256, 1.514114011542639693 ) ) ;
#30123=CARTESIAN_POINT ( 'NONE',  ( -0.9950013725589796909, 29.65466048987409309, -4.513790593961638287 ) ) ;
#30125=CARTESIAN_POINT ( 'NONE',  ( 20.61342602778648825, 152.5829384802601396, 0.8505107393516945224 ) ) ;
#30126=CARTESIAN_POINT ( 'NONE',  ( 15.52406135986475277, 147.5381818669338827, 0.5105160171526207380 ) ) ;
#30128=CARTESIAN_POINT ( 'NONE',  ( 0.8486417380921021936, -9.850041244260159701, -0.4793021190969105616 ) ) ;
#30129=CARTESIAN_POINT ( 'NONE',  ( -15.16003043525278215, 156.1230782244120121, -0.5028385762316637253 ) ) ;
#30130=DIRECTION ( 'NONE',  ( -0.9998004120163609398, 0.000000000000000000, -0.01997839162482749689 ) ) ;
#30131=CARTESIAN_POINT ( 'NONE',  ( 4.756879258228443597, 117.4006795747281586, 1.206942419589918991 ) ) ;
#30133=CARTESIAN_POINT ( 'NONE',  ( 5.546876812502214982, 116.7824702235449621, 0.3920729990857263481 ) ) ;
#30134=CARTESIAN_POINT ( 'NONE',  ( -5.507840079722835291, 156.5946142756450570, 1.582329182567088210 ) ) ;
#30136=CARTESIAN_POINT ( 'NONE',  ( 12.12330053995811774, 120.5818589831333441, 1.513795679345424583 ) ) ;
#30137=CARTESIAN_POINT ( 'NONE',  ( 19.45999741125991989, 148.3988719805327037, -1.735632530687203356 ) ) ;
#30138=CARTESIAN_POINT ( 'NONE',  ( -0.8818152078519037040, -12.16566588317193265, -0.4137299969793124532 ) ) ;
#30139=CARTESIAN_POINT ( 'NONE',  ( -5.844449987888692633, 118.2031694463412634, -1.045635565433329361 ) ) ;
#30142=CARTESIAN_POINT ( 'NONE',  ( 4.505160425060487306, 105.1215147309967080, 2.878549663133488590 ) ) ;
#30144=CARTESIAN_POINT ( 'NONE',  ( 8.566376370482780445, 122.4751019636825049, -0.6322842599711310241 ) ) ;
#30145=CARTESIAN_POINT ( 'NONE',  ( -9.163388821854908883, 124.2347608867413413, -0.1831063163140473071 ) ) ;
#30147=CARTESIAN_POINT ( 'NONE',  ( -11.17842967653879249, 122.9575399027323073, -1.639653439019827186 ) ) ;
#30148=CARTESIAN_POINT ( 'NONE',  ( 3.739721301978734314, -15.76301488427489517, 4.305968564470687987 ) ) ;
#30149=CARTESIAN_POINT ( 'NONE',  ( -4.557225192774990497, 118.0384377347435958, -0.8496051783353677500 ) ) ;
#30152=CARTESIAN_POINT ( 'NONE',  ( 4.261081698622550817, 119.8084884740358547, 0.9035344350157261673 ) ) ;
#30155=CARTESIAN_POINT ( 'NONE',  ( 6.896656464550490639, 117.1676486657671177, 0.1232935741316918549 ) ) ;
#30156=CARTESIAN_POINT ( 'NONE',  ( 2.469379016249674486, 9.589258615745848147, -8.089366445887874235 ) ) ;
#30157=CARTESIAN_POINT ( 'NONE',  ( 7.076231864619158429, 121.9239394581621809, 0.5528764260536548347 ) ) ;
#30158=CARTESIAN_POINT ( 'NONE',  ( 14.01781138111942404, 120.5923583732999873, -0.6175494627556293858 ) ) ;
#30162=CARTESIAN_POINT ( 'NONE',  ( -23.21350185287846912, 149.6290410902582551, -0.3868015801638792772 ) ) ;
#30163=ORIENTED_EDGE ( 'NONE', *, *, #22929, .F. ) ;
#30164=CARTESIAN_POINT ( 'NONE',  ( 8.121995431296815227, 121.0945329078791843, -0.9875153719367453231 ) ) ;
#30165=CARTESIAN_POINT ( 'NONE',  ( -6.538176131568015962E-14, 82.13546620154573930, -1.207165459078370276E-19 ) ) ;
#30168=CARTESIAN_POINT ( 'NONE',  ( -6.044022022451821741, 155.3491655920357459, -0.4731370799734935795 ) ) ;
#30169=CARTESIAN_POINT ( 'NONE',  ( 4.970078376064472003, -11.71998231623441100, 0.7442660586517341192 ) ) ;
#30170=CARTESIAN_POINT ( 'NONE',  ( -6.877630800715581749, 117.9658002137636856, 0.6876290806823444068 ) ) ;
#30172=CARTESIAN_POINT ( 'NONE',  ( -0.0002734175339891707266, 159.6054662015457382, 0.01368293144939998138 ) ) ;
#30174=CARTESIAN_POINT ( 'NONE',  ( 1.686640475165922748, -9.627085671684914914, -4.319569293544198274 ) ) ;
#30175=CARTESIAN_POINT ( 'NONE',  ( -23.44919332464161599, 146.8469795362756258, -0.4944523877934683953 ) ) ;
#30179=CARTESIAN_POINT ( 'NONE',  ( -8.304993556123838161, 120.2147940885562889, 1.117492704526953817 ) ) ;
#30180=CARTESIAN_POINT ( 'NONE',  ( 0.8067276567327370529, -3.745225398377231674, -4.556403025205434609 ) ) ;
#30181=CARTESIAN_POINT ( 'NONE',  ( 14.73734951358248857, 121.3346631531286164, 1.319546682830233797 ) ) ;
#30183=DIRECTION ( 'NONE',  ( -0.9998004120163608288, 0.000000000000000000, -0.01997839162482749342 ) ) ;
#30184=CARTESIAN_POINT ( 'NONE',  ( 13.31748376333897532, 121.6721647909590303, -1.150164054616430453 ) ) ;
#30185=CARTESIAN_POINT ( 'NONE',  ( 4.628409624684510781, -5.919234854628785847, 0.1277143096542201761 ) ) ;
#30186=CARTESIAN_POINT ( 'NONE',  ( -22.31420326625529782, 142.2114994846844240, -1.760598597564681622 ) ) ;
#30188=CARTESIAN_POINT ( 'NONE',  ( -8.883181220021290514, 123.7004864364556909, -0.02116515827996221996 ) ) ;
#30189=CARTESIAN_POINT ( 'NONE',  ( 5.719270376754757912, -14.62604927220606577, 2.811085246033490304 ) ) ;
#30192=CARTESIAN_POINT ( 'NONE',  ( -4.038290521723881810, 111.0900967538891564, -3.207870893326146167 ) ) ;
#30193=ORIENTED_EDGE ( 'NONE', *, *, #34997, .F. ) ;
#30194=CARTESIAN_POINT ( 'NONE',  ( 11.06681148537619563, 121.4866960210745503, 1.697623966824489683 ) ) ;
#30195=CARTESIAN_POINT ( 'NONE',  ( 4.962772945303370875, 117.4661736183843317, 0.9732638675253090232 ) ) ;
#30198=CARTESIAN_POINT ( 'NONE',  ( -0.01645572339173941370, 159.4324016994384010, 0.8235116888278194436 ) ) ;
#30199=CARTESIAN_POINT ( 'NONE',  ( 7.912908961612729719, 12.87109176889305928, 2.878135455392844655 ) ) ;
#30200=CARTESIAN_POINT ( 'NONE',  ( 16.40115699206375410, 147.1833543704171348, 1.602497317185074710 ) ) ;
#30202=CARTESIAN_POINT ( 'NONE',  ( 22.47739742037821031, 150.5824416163731314, -0.2728482117335694346 ) ) ;
#30207=CARTESIAN_POINT ( 'NONE',  ( -4.829600922136632946, 117.3993836135881423, 1.010428145333803540 ) ) ;
#30210=CARTESIAN_POINT ( 'NONE',  ( -4.421375971199002386, 118.1651973794024855, 0.4750358156669655663 ) ) ;
#30214=CARTESIAN_POINT ( 'NONE',  ( 4.007742253885239414, 119.1179171808522312, -0.7639785333703686954 ) ) ;
#30215=CARTESIAN_POINT ( 'NONE',  ( -7.613751273744924219, 124.2930771091975117, -0.1610855651276038303 ) ) ;
#30216=CARTESIAN_POINT ( 'NONE',  ( 4.578501332539032909, 118.0757660871476986, 0.7069378206079117710 ) ) ;
#30217=CARTESIAN_POINT ( 'NONE',  ( -16.29504633872605268, 146.4745453488731357, -1.441742819671184561 ) ) ;
#30218=CARTESIAN_POINT ( 'NONE',  ( -0.7365778754629619396, 115.7029383710874839, -1.756171452946359013 ) ) ;
#30220=CARTESIAN_POINT ( 'NONE',  ( 4.503688181905097565, 111.2539628214143903, -2.957939639849824331 ) ) ;
#30221=CARTESIAN_POINT ( 'NONE',  ( -15.56955422694819902, 149.1167355181319181, -1.737459915651670128 ) ) ;
#30222=FACE_OUTER_BOUND ( 'NONE', #35479, .T. ) ;
#30225=CARTESIAN_POINT ( 'NONE',  ( -0.001967380068485734355, 120.9974662015458620, 0.09845574358318300023 ) ) ;
#30226=CARTESIAN_POINT ( 'NONE',  ( 4.529186081025091681, -11.15152372915077095, -0.9203776863585164669 ) ) ;
#30227=CARTESIAN_POINT ( 'NONE',  ( 15.06876432237280206, 120.9194639129320734, 0.9861043747356995626 ) ) ;
#30229=CARTESIAN_POINT ( 'NONE',  ( 2.368424984008928202, -15.31393412036581658, 4.927583237414308037 ) ) ;
#30230=CARTESIAN_POINT ( 'NONE',  ( -17.82416131750972355, 140.4837523222294351, 1.726486987461786082 ) ) ;
#30231=CARTESIAN_POINT ( 'NONE',  ( -0.8818152078519037040, -12.16566588317193265, -0.4137299969793124532 ) ) ;
#30232=CARTESIAN_POINT ( 'NONE',  ( -15.11126220171611045, 120.7387302883610118, -0.8143899245520163088 ) ) ;
#30233=CARTESIAN_POINT ( 'NONE',  ( -0.4283232389533950801, 25.18001705023179326, -0.8778289364919926729 ) ) ;
#30234=ORIENTED_EDGE ( 'NONE', *, *, #18395, .T. ) ;
#30236=CARTESIAN_POINT ( 'NONE',  ( 7.618479139564603209, 124.7215218652630710, 0.1522353441811852559 ) ) ;
#30237=CARTESIAN_POINT ( 'NONE',  ( -3.624202338748801377, 120.7384399880717467, 0.3073100964232673427 ) ) ;
#30238=CARTESIAN_POINT ( 'NONE',  ( 2.037655544652288597, -15.20941935993469585, 5.943311982828837436 ) ) ;
#30239=CARTESIAN_POINT ( 'NONE',  ( 17.81417655509802955, 146.7645792007554633, -1.532459167469646388 ) ) ;
#30241=CARTESIAN_POINT ( 'NONE',  ( -6.675970744194720474, 119.4737997143703012, -1.289985488916530088 ) ) ;
#30242=CARTESIAN_POINT ( 'NONE',  ( 3.722615052411291980, 115.7030845075131964, 1.610880590277100621 ) ) ;
#30243=CARTESIAN_POINT ( 'NONE',  ( 3.216700609619024931, -14.42020774479446921, 2.887214088933996337 ) ) ;
#30245=CARTESIAN_POINT ( 'NONE',  ( 4.254723467274340365, 155.8413357349917021, -0.07908073517333519264 ) ) ;
#30247=CARTESIAN_POINT ( 'NONE',  ( -4.076413542934153256, 109.5187692929430483, 3.449420018115528563 ) ) ;
#30248=CARTESIAN_POINT ( 'NONE',  ( 0.9487982336569755759, 106.1808064897677468, 5.207608974602796259 ) ) ;
#30249=CARTESIAN_POINT ( 'NONE',  ( -2.094298925633724995, 29.77768649804257350, -0.07299356519333505267 ) ) ;
#30252=CARTESIAN_POINT ( 'NONE',  ( 20.68286957925295511, 152.5754960671270055, 0.1900957434528340873 ) ) ;
#30254=CARTESIAN_POINT ( 'NONE',  ( 1.790609531311249336, -15.35462110475191366, 5.967943360138708186 ) ) ;
#30256=CARTESIAN_POINT ( 'NONE',  ( -2.960856320778833872, 31.17411798999470918, 0.6378382452821288462 ) ) ;
#30257=EDGE_CURVE ( 'NONE', #5241, #4233, #21891, .T. ) ;
#30258=CARTESIAN_POINT ( 'NONE',  ( 11.75177080394823825, 120.8928578745602209, 1.619740935434792473 ) ) ;
#30259=ORIENTED_EDGE ( 'NONE', *, *, #19599, .T. ) ;
#30260=CARTESIAN_POINT ( 'NONE',  ( 2.561087359964590249, 24.90515699240134495, 8.022552078460996938 ) ) ;
#30261=CARTESIAN_POINT ( 'NONE',  ( 8.651708239172382520, 118.4867078446797564, -0.7346615941013865392 ) ) ;
#30262=CARTESIAN_POINT ( 'NONE',  ( -0.2359694434510269667, 106.4201689084969047, -5.118158396747612748 ) ) ;
#30263=CARTESIAN_POINT ( 'NONE',  ( 4.918189655395446280, 117.4102201643931664, 1.103006975100219167 ) ) ;
#30264=DIRECTION ( 'NONE',  ( 0.9998004120163610509, 4.016384292689131511E-17, 0.01997839162482749689 ) ) ;
#30266=CARTESIAN_POINT ( 'NONE',  ( 0.7336086519982951692, 0.2932837538699786251, -4.563195415240439701 ) ) ;
#30268=CARTESIAN_POINT ( 'NONE',  ( -0.9670243388409863750, 105.9610423702829962, -5.250383317772386427 ) ) ;
#30269=CARTESIAN_POINT ( 'NONE',  ( 3.073681112652024261, -14.41515119294017921, 4.164397941202722109 ) ) ;
#30270=CARTESIAN_POINT ( 'NONE',  ( 5.284455934299999491, 122.2451909684448310, -0.05007199584899529876 ) ) ;
#30271=CARTESIAN_POINT ( 'NONE',  ( -21.54968253652557664, 151.3526640061693342, 0.5241015958777710537 ) ) ;
#30272=CARTESIAN_POINT ( 'NONE',  ( 2.866728174840395216, 37.98889525090484653, 1.397978221435858703 ) ) ;
#30273=CIRCLE ( 'NONE', #12607, 3.175000000000001155 ) ;
#30275=EDGE_LOOP ( 'NONE', ( #709, #10167 ) ) ;
#30276=CARTESIAN_POINT ( 'NONE',  ( -4.507527029703037869, 105.1215318987586187, -2.874941136914541229 ) ) ;
#30277=CARTESIAN_POINT ( 'NONE',  ( 4.580902669819289841, -15.62468711146633460, 2.622166941725792899 ) ) ;
#30278=CARTESIAN_POINT ( 'NONE',  ( -0.03212618750959882197, 158.2819368290249713, 1.607725792532325393 ) ) ;
#30279=CARTESIAN_POINT ( 'NONE',  ( -4.637963820743935983, -6.603494994175692412, 0.1710436084038768345 ) ) ;
#30281=VERTEX_POINT ( 'NONE', #11721 ) ;
#30282=CARTESIAN_POINT ( 'NONE',  ( 3.009276887026298031, 39.20946620154573736, -1.210121013456480599 ) ) ;
#30283=CARTESIAN_POINT ( 'NONE',  ( 0.7855309748068020070, 120.8419495465347069, 0.4764688261655856683 ) ) ;
#30284=CARTESIAN_POINT ( 'NONE',  ( -13.22964523056198161, 152.2904283036577908, 1.375236710735038281 ) ) ;
#30285=CARTESIAN_POINT ( 'NONE',  ( 4.227135066434014377, 117.9852780145697011, 0.9714402365040194498 ) ) ;
#30287=CARTESIAN_POINT ( 'NONE',  ( 1.346530140708997347, 119.3298839580929638, -0.5995503221117500781 ) ) ;
#30288=CARTESIAN_POINT ( 'NONE',  ( -15.63125989577342878, 125.4375369430449609, -1.961567602338091243 ) ) ;
#30291=CARTESIAN_POINT ( 'NONE',  ( 4.158644871452826131, 118.2391781275531883, -0.2328945661949778645 ) ) ;
#30292=CARTESIAN_POINT ( 'NONE',  ( 15.96529520877005481, 145.8030804522035737, -0.4114451159501716360 ) ) ;
#30294=CARTESIAN_POINT ( 'NONE',  ( 3.071204355543858178, -15.18643405355604692, 3.901769932616943493 ) ) ;
#30298=CARTESIAN_POINT ( 'NONE',  ( -4.609865753310859127, 8.349128549105346409, -0.5081561704775721111 ) ) ;
#30299=CARTESIAN_POINT ( 'NONE',  ( 6.520514997712263394, 120.9817801663137971, 0.9553606176145343909 ) ) ;
#30300=CARTESIAN_POINT ( 'NONE',  ( 2.870896314602991328, 37.68923040074404440, 0.3265960267205035295 ) ) ;
#30301=B_SPLINE_CURVE_WITH_KNOTS ( 'NONE', 3,
 ( #12364, #34955, #15118, #28121, #41131, #2373, #24928, #15332 ),
 .UNSPECIFIED., .F., .F.,
 ( 4, 2, 2, 4 ),
 ( 1.176555559258168665E-05, 0.0004666053235290343283, 0.0006940252074972603916, 0.0009214450914654865633 ),
 .UNSPECIFIED. ) ;
#30302=CARTESIAN_POINT ( 'NONE',  ( 4.458631606973747274, 16.91056413504885825, 1.251853190366734259 ) ) ;
#30303=CARTESIAN_POINT ( 'NONE',  ( 11.83578944268984934, 152.0103986367769551, 0.2843524715992695739 ) ) ;
#30306=CARTESIAN_POINT ( 'NONE',  ( -5.556137103167946734, 116.7241256494533275, -0.2898596823833969882 ) ) ;
#30309=CARTESIAN_POINT ( 'NONE',  ( 2.079616623477895221, -15.54617723206732371, 5.925385729176053218 ) ) ;
#30311=CARTESIAN_POINT ( 'NONE',  ( 8.331117840153179799, 7.414970825009634225, 1.249357972265521255 ) ) ;
#30312=FACE_BOUND ( 'NONE', #2237, .T. ) ;
#30315=CARTESIAN_POINT ( 'NONE',  ( -22.98897055778776632, 149.8455236008688303, 0.1339715990509171561 ) ) ;
#30316=EDGE_CURVE ( 'NONE', #1745, #22781, #6295, .T. ) ;
#30317=ORIENTED_EDGE ( 'NONE', *, *, #30088, .T. ) ;
#30319=CARTESIAN_POINT ( 'NONE',  ( 6.992757797159352862, 121.9549134519901656, 0.1079654902816031131 ) ) ;
#30321=ORIENTED_EDGE ( 'NONE', *, *, #35539, .T. ) ;
#30323=CARTESIAN_POINT ( 'NONE',  ( -2.828086164579570294, 121.0305217392013759, -0.08274239724663733087 ) ) ;
#30324=CARTESIAN_POINT ( 'NONE',  ( 6.240488881946434141, -13.64759869265259873, 1.419018975165988294 ) ) ;
#30325=CARTESIAN_POINT ( 'NONE',  ( -13.94573646207672013, 122.0315337860429423, 1.127490061167130797 ) ) ;
#30326=CARTESIAN_POINT ( 'NONE',  ( 3.254034125433558522, 159.4600617640778353, 0.3425454502237992860 ) ) ;
#30327=CARTESIAN_POINT ( 'NONE',  ( 0.6391523125838497466, 156.3034662015460583, 0.1199623171637351216 ) ) ;
#30328=CARTESIAN_POINT ( 'NONE',  ( 0.03652159268533760467, -3.380040448513521589, 0.9750733386546841519 ) ) ;
#30329=CARTESIAN_POINT ( 'NONE',  ( -23.29193865421797938, 149.0397177335360652, -0.7969840597304522767 ) ) ;
#30330=CARTESIAN_POINT ( 'NONE',  ( 4.862311738186619436, 117.4092090646522308, 1.165993606892455903 ) ) ;
#30332=CARTESIAN_POINT ( 'NONE',  ( -2.204606251742418088, 116.2294481778856152, 0.03196190806868362544 ) ) ;
#30333=CARTESIAN_POINT ( 'NONE',  ( -18.18950303832469828, 147.2296321676236062, 1.619102437044615428 ) ) ;
#30335=CARTESIAN_POINT ( 'NONE',  ( 16.12894526037916521, 128.5601350900737998, -1.548733376446669086 ) ) ;
#30336=CARTESIAN_POINT ( 'NONE',  ( 0.4015916885733669117, -14.54189033959780808, -0.8905040343298938899 ) ) ;
#30337=CARTESIAN_POINT ( 'NONE',  ( -9.605778978211169772, 157.4977751962898083, -1.777432263976032489 ) ) ;
#30340=CARTESIAN_POINT ( 'NONE',  ( 4.756737841188980020, 105.1215164090288425, 2.421843111834511397 ) ) ;
#30341=CARTESIAN_POINT ( 'NONE',  ( 16.75300165896958404, 146.9696287467501179, -1.108775417838742783 ) ) ;
#30342=CARTESIAN_POINT ( 'NONE',  ( -4.936883229164080511, 117.6536490159478774, 0.7443082606323431216 ) ) ;
#30344=CARTESIAN_POINT ( 'NONE',  ( -7.396903380747485102, 120.6159063994810055, -1.271367681336521782 ) ) ;
#30345=CARTESIAN_POINT ( 'NONE',  ( 4.698461193529555935, -15.58032547337365159, 2.177983573914926030 ) ) ;
#30346=CARTESIAN_POINT ( 'NONE',  ( -4.801729350823258358, 117.4006813127757027, 1.015859690946131932 ) ) ;
#30347=CARTESIAN_POINT ( 'NONE',  ( -4.489008837794409956, 118.1174813940656492, -0.7254504362431349884 ) ) ;
#30349=CARTESIAN_POINT ( 'NONE',  ( 4.065926199369043204, 118.2429491485453354, 0.3080910687088499467 ) ) ;
#30350=B_SPLINE_SURFACE_WITH_KNOTS ( 'NONE', 1, 3, ( 
 ( #4975, #15728, #40338, #25537, #9353, #12547 ),
 ( #24119, #35138, #28317, #18502, #7949, #12129 ) ),
 .UNSPECIFIED., .F., .F., .F.,
 ( 2, 2 ),
 ( 4, 2, 4 ),
 ( 0.000000000000000000, 1.000000000000000000 ),
 ( 0.000000000000000000, 0.5000000000000000000, 1.000000000000000000 ),
 .UNSPECIFIED. ) ;
#30351=CARTESIAN_POINT ( 'NONE',  ( 9.271712722858115541, 121.5662863950884400, 1.459403803239323727 ) ) ;
#30352=DIRECTION ( 'NONE',  ( 0.003125310045138050483, -0.9876883405951376593, -0.1564032425800216952 ) ) ;
#30353=CARTESIAN_POINT ( 'NONE',  ( 15.97340373827820947, 121.0409387471171101, 0.3191866212789525314 ) ) ;
#30354=AXIS2_PLACEMENT_3D ( 'NONE', #34067, #31477, #30642 ) ;
#30355=CARTESIAN_POINT ( 'NONE',  ( 3.617035938018385632, 9.361278981710560387, -7.607506385697127449 ) ) ;
#30356=CARTESIAN_POINT ( 'NONE',  ( 13.71401989163316237, 150.2158912636999730, 0.8490545446796919915 ) ) ;
#30358=CARTESIAN_POINT ( 'NONE',  ( 22.75813664408058301, 148.5871737753741115, -0.7284712318767730954 ) ) ;
#30361=CARTESIAN_POINT ( 'NONE',  ( -6.606029807653651701E-14, 92.04146620154574521, -3.372746026535634231E-18 ) ) ;
#30363=CARTESIAN_POINT ( 'NONE',  ( -11.72569139212704137, 118.7251779360019270, -0.1869994294823656700 ) ) ;
#30364=ORIENTED_EDGE ( 'NONE', *, *, #14365, .T. ) ;
#30366=CARTESIAN_POINT ( 'NONE',  ( -8.033132201554776586, 121.3102024099959380, -1.246334813644621953 ) ) ;
#30370=CARTESIAN_POINT ( 'NONE',  ( -13.11017186724486372, 133.9996589410087324, -0.6993036124459156566 ) ) ;
#30371=CARTESIAN_POINT ( 'NONE',  ( 2.708195657389492084, -14.88772387794683105, 5.660366118324242635 ) ) ;
#30372=CARTESIAN_POINT ( 'NONE',  ( -11.01560508856928067, 119.3804150619309468, 0.7804404673305009865 ) ) ;
#30373=CARTESIAN_POINT ( 'NONE',  ( -6.517733866319332394E-14, 78.32546620154573702, 2.848871684924056535E-29 ) ) ;
#30374=CARTESIAN_POINT ( 'NONE',  ( 23.40402153822879683, 142.8142681763856388, 0.5431523703306526674 ) ) ;
#30376=CARTESIAN_POINT ( 'NONE',  ( -2.948169924849943335, 1.592661447142720732, -3.562413953034572867 ) ) ;
#30377=CARTESIAN_POINT ( 'NONE',  ( -21.90559427349704080, 151.4293160993575498, -0.4377259060014663805 ) ) ;
#30378=DIRECTION ( 'NONE',  ( 4.017660918040594346E-17, -1.000000000000000000, -2.376309959284834438E-19 ) ) ;
#30380=ORIENTED_EDGE ( 'NONE', *, *, #28217, .T. ) ;
#30381=CARTESIAN_POINT ( 'NONE',  ( 5.000577394074683824, 119.1797654937509492, 1.102527082765531352 ) ) ;
#30383=CARTESIAN_POINT ( 'NONE',  ( -0.05192310401019068627, -8.293124787585329116, 4.627658001227512585 ) ) ;
#30384=CARTESIAN_POINT ( 'NONE',  ( 4.872874520552131550, 117.5843641943970681, 0.8145397704027566022 ) ) ;
#30387=CARTESIAN_POINT ( 'NONE',  ( 13.13885824085852860, 121.7804325175133755, -1.194399340605180049 ) ) ;
#30388=CARTESIAN_POINT ( 'NONE',  ( -4.360315236241580017, -1.596229544307166348, -1.535301415559372940 ) ) ;
#30389=CARTESIAN_POINT ( 'NONE',  ( -3.876365344914242783, 117.1932757116604762, -0.6224469224293305292 ) ) ;
#30391=ORIENTED_EDGE ( 'NONE', *, *, #24786, .T. ) ;
#30394=CARTESIAN_POINT ( 'NONE',  ( -14.28939804845289707, 138.9852717218771261, 0.04639197223238064605 ) ) ;
#30395=CARTESIAN_POINT ( 'NONE',  ( 5.121635214396401459, -14.94813357331645243, 3.889196783476005059 ) ) ;
#30398=EDGE_LOOP ( 'NONE', ( #11428, #1647, #19332, #21911 ) ) ;
#30399=CARTESIAN_POINT ( 'NONE',  ( 12.88625155327537541, 123.9867020804889961, 1.879256283450041254 ) ) ;
#30400=CARTESIAN_POINT ( 'NONE',  ( -3.174366308152013705, 104.6144662015457243, -0.06343139340882732180 ) ) ;
#30401=DIRECTION ( 'NONE',  ( -0.9998004120163608288, 0.000000000000000000, -0.01997839162482747608 ) ) ;
#30404=CARTESIAN_POINT ( 'NONE',  ( -22.12956052442025978, 150.1365687424457178, 0.8564216397177744078 ) ) ;
#30405=CARTESIAN_POINT ( 'NONE',  ( -8.372926607701892010, 8.771278641329313785, 0.9163881402227073147 ) ) ;
#30406=CARTESIAN_POINT ( 'NONE',  ( 9.931348751161650057, 124.0638329749226330, 0.9965119107524912367 ) ) ;
#30408=CARTESIAN_POINT ( 'NONE',  ( 23.09710566998031922, 146.6371693212631158, -0.4017528712124324164 ) ) ;
#30410=AXIS2_PLACEMENT_3D ( 'NONE', #18444, #9506, #6321 ) ;
#30415=CARTESIAN_POINT ( 'NONE',  ( -4.401147469462643791, 118.1832779091558905, 0.4087992378694457751 ) ) ;
#30416=CARTESIAN_POINT ( 'NONE',  ( 0.6996515051864370394, 105.8266127453863987, -5.294619967806604599 ) ) ;
#30420=CARTESIAN_POINT ( 'NONE',  ( 8.337297254786394163, 120.0572855657016049, -1.117728404394529917 ) ) ;
#30421=CARTESIAN_POINT ( 'NONE',  ( -0.1515127994570748815, 105.8822825325953261, -5.338933990912773098 ) ) ;
#30422=CARTESIAN_POINT ( 'NONE',  ( 4.534812482471024531, 118.1057876144154193, 0.6733639414384589017 ) ) ;
#30423=CARTESIAN_POINT ( 'NONE',  ( -4.456531362648609829, 120.8671296916768227, -0.5026912216012410228 ) ) ;
#30424=CARTESIAN_POINT ( 'NONE',  ( -0.2925749420451331240, 115.7029491485453150, -1.764546101263113398 ) ) ;
#30426=CARTESIAN_POINT ( 'NONE',  ( 1.972857920798343212, 118.1651004355878456, -0.7713121312975299571 ) ) ;
#30427=CARTESIAN_POINT ( 'NONE',  ( 5.379991719817613038, 116.9256180743815179, -0.7442756809649815342 ) ) ;
#30428=CARTESIAN_POINT ( 'NONE',  ( -10.39772550536733675, 123.9810924921358151, -1.245468829273463252 ) ) ;
#30432=CARTESIAN_POINT ( 'NONE',  ( -2.874620413851559420, 156.1036891334628933, 0.02956450310463179867 ) ) ;
#30434=CARTESIAN_POINT ( 'NONE',  ( 8.117713882137667980, 117.8329967196738153, 0.7633534655057000462 ) ) ;
#30435=DIRECTION ( 'NONE',  ( -0.01997839162482737546, -1.040247600000940825E-18, 0.9998004120163610509 ) ) ;
#30436=CARTESIAN_POINT ( 'NONE',  ( 3.259035188333455846, -14.62011735832338744, 2.262668647611313588 ) ) ;
#30437=CARTESIAN_POINT ( 'NONE',  ( -18.44328704050468914, 144.7751241387205425, 1.717333923880829838 ) ) ;
#30438=CARTESIAN_POINT ( 'NONE',  ( 0.1324238259082184954, -4.506001423838159603, -0.9708255322318050107 ) ) ;
#30439=CARTESIAN_POINT ( 'NONE',  ( -4.801439827634331081, 117.0090399748681875, -0.4924919612534519042 ) ) ;
#30441=CARTESIAN_POINT ( 'NONE',  ( 0.8415213475290624912, 13.30065917492326122, -0.4928529130785159751 ) ) ;
#30442=VERTEX_POINT ( 'NONE', #41553 ) ;
#30443=ADVANCED_FACE ( 'NONE', ( #5149 ), #8351, .F. ) ;
#30445=CARTESIAN_POINT ( 'NONE',  ( 3.406460098309076923, 108.6786390861269922, 4.123178694279357792 ) ) ;
#30446=CARTESIAN_POINT ( 'NONE',  ( -15.67979071779219602, 147.9168465093495399, 0.5330609057418903562 ) ) ;
#30447=CARTESIAN_POINT ( 'NONE',  ( 4.676120195389507295, -12.14821529611620576, 1.449936329584695649 ) ) ;
#30448=CARTESIAN_POINT ( 'NONE',  ( 15.03323000681557708, 150.5987129668814077, -1.374706190065595468 ) ) ;
#30450=CARTESIAN_POINT ( 'NONE',  ( -11.61050889437352751, 122.1450671466348439, -1.749762830748087694 ) ) ;
#30451=EDGE_CURVE ( 'NONE', #11376, #36618, #24924, .T. ) ;
#30452=CARTESIAN_POINT ( 'NONE',  ( 4.303750855783647467, 104.6144662015457953, 2.191315715000266895 ) ) ;
#30453=CARTESIAN_POINT ( 'NONE',  ( 3.073681112652024261, -14.41515119294017921, 4.164397941202722109 ) ) ;
#30454=CARTESIAN_POINT ( 'NONE',  ( -4.918661145027864556, 117.4102335145295370, -1.102851133234106662 ) ) ;
#30455=CARTESIAN_POINT ( 'NONE',  ( 9.568355480995425211, 124.8108731098830049, 0.1557749891131964270 ) ) ;
#30457=CARTESIAN_POINT ( 'NONE',  ( 2.213841846844817329, 118.2767885243204944, 0.7726204694312127641 ) ) ;
#30458=CARTESIAN_POINT ( 'NONE',  ( 3.611552524025655853, 109.1680412998471610, 3.931639664578665982 ) ) ;
#30459=CARTESIAN_POINT ( 'NONE',  ( -8.798071503382049130, 117.6842349159514640, -0.1758064068840608507 ) ) ;
#30460=CARTESIAN_POINT ( 'NONE',  ( -4.864318412922314039, 27.89189352517958298, 0.5016899395801051043 ) ) ;
#30461=CARTESIAN_POINT ( 'NONE',  ( 0.3092006194327232005, 116.5226405152084652, -0.1184213420814130696 ) ) ;
#30464=CARTESIAN_POINT ( 'NONE',  ( 1.773284331787727819, -15.30902614633587788, 5.947961136908312518 ) ) ;
#30467=CARTESIAN_POINT ( 'NONE',  ( 20.33492986670560043, 149.7738053052645171, 2.379138827545466128 ) ) ;
#30468=EDGE_LOOP ( 'NONE', ( #26997, #12795, #21611, #7596 ) ) ;
#30469=CARTESIAN_POINT ( 'NONE',  ( -7.836836066720379357, 21.45871166075947656, -3.113543590022962881 ) ) ;
#30471=CARTESIAN_POINT ( 'NONE',  ( 2.436681026199804201, 117.3681707349357879, -0.6167178112848459293 ) ) ;
#30472=CARTESIAN_POINT ( 'NONE',  ( -2.562387952376977029, 120.6526784328644339, -0.4448203013800773875 ) ) ;
#30473=CARTESIAN_POINT ( 'NONE',  ( 4.966734726183148041, 117.4023932319876877, 1.002418842663953980 ) ) ;
#30475=CARTESIAN_POINT ( 'NONE',  ( -5.220201361148701480, 105.1221159690571056, 1.151354633625773394 ) ) ;
#30476=CARTESIAN_POINT ( 'NONE',  ( 4.627880361116947228, 7.839802885307131319, -0.3238752845059330032 ) ) ;
#30479=CARTESIAN_POINT ( 'NONE',  ( 2.356490753556696571, -15.00856118213019030, 5.009515689243722925 ) ) ;
#30480=CARTESIAN_POINT ( 'NONE',  ( 4.551932963793348108, 124.4408722044843927, 0.07212455616362449529 ) ) ;
#30482=CARTESIAN_POINT ( 'NONE',  ( -3.918109666403713831, 29.36550307138034910, 3.251447169634396062 ) ) ;
#30485=CARTESIAN_POINT ( 'NONE',  ( -3.896500353948071815, 104.6144662015455253, -2.865913902984364103 ) ) ;
#30486=CARTESIAN_POINT ( 'NONE',  ( 1.975136073220363553, -15.70315947173593685, 5.621751108460156132 ) ) ;
#30487=CARTESIAN_POINT ( 'NONE',  ( -13.91587783890489760, 154.2684476645699760, 1.737230819368874579 ) ) ;
#30488=CARTESIAN_POINT ( 'NONE',  ( -1.825063964020108065, -4.879331645356781877, 4.256838567046823840 ) ) ;
#30489=EDGE_CURVE ( 'NONE', #13569, #37741, #9034, .T. ) ;
#30493=CARTESIAN_POINT ( 'NONE',  ( 1.451835205608120294, 110.3135721340718334, 3.567596948272937940 ) ) ;
#30495=CARTESIAN_POINT ( 'NONE',  ( -0.01887828017123771920, 156.5412816204240301, 0.9447463363288814975 ) ) ;
#30497=CARTESIAN_POINT ( 'NONE',  ( 2.489404145489803266, 119.6096776070104681, -0.6201668936895530226 ) ) ;
#30498=CARTESIAN_POINT ( 'NONE',  ( -3.119203903361180252, 118.1710492231644736, -0.8508709904442464111 ) ) ;
#30500=CARTESIAN_POINT ( 'NONE',  ( 4.303426754916820585, 118.2142125059335456, -0.3398192420404221314 ) ) ;
#30502=CARTESIAN_POINT ( 'NONE',  ( 15.94455450784139749, 146.9815093338748966, -0.4077454470555674781 ) ) ;
#30504=CARTESIAN_POINT ( 'NONE',  ( 2.913544029416218262, -15.22775915604775143, 4.213357497968500454 ) ) ;
#30505=AXIS2_PLACEMENT_3D ( 'NONE', #29896, #13285, #26270 ) ;
#30508=CARTESIAN_POINT ( 'NONE',  ( 4.615940417482057967, 3.801270455692813410, -0.2501868467277520436 ) ) ;
#30509=CARTESIAN_POINT ( 'NONE',  ( 9.541807374902186112, 122.7780075402122151, 1.248600054375463619 ) ) ;
#30511=CARTESIAN_POINT ( 'NONE',  ( 2.935476374454474513, 38.79430649453939850, 1.140240003322550155 ) ) ;
#30512=CARTESIAN_POINT ( 'NONE',  ( -1.980640663884833064, 106.8720524443079967, 4.823141945187445323 ) ) ;
#30514=CARTESIAN_POINT ( 'NONE',  ( 4.203610184846851894, 17.99761390031315500, -1.968029828111186319 ) ) ;
#30515=CARTESIAN_POINT ( 'NONE',  ( 5.974701571114410470, 155.3719879121972838, 0.2191910023528571561 ) ) ;
#30519=CARTESIAN_POINT ( 'NONE',  ( -5.551613292181984072, 116.7425018655093396, -0.3404755252327396065 ) ) ;
#30520=FACE_OUTER_BOUND ( 'NONE', #7976, .T. ) ;
#30522=CARTESIAN_POINT ( 'NONE',  ( -1.392417755420867209, 106.2993931590560237, 5.100690970918774880 ) ) ;
#30524=CARTESIAN_POINT ( 'NONE',  ( -7.020956707233273697, 3.738713905105897517, 4.673168047251142099 ) ) ;
#30525=EDGE_CURVE ( 'NONE', #1729, #29613, #6626, .T. ) ;
#30526=CARTESIAN_POINT ( 'NONE',  ( 3.682264917456193221, 76.29346620154572634, 0.07358041635423968885 ) ) ;
#30527=DIRECTION ( 'NONE',  ( -0.01997839790104462970, 0.000000000000000000, 0.9998004118909472604 ) ) ;
#30529=CARTESIAN_POINT ( 'NONE',  ( 0.005880675322188773195, 122.2435587914035295, -0.2942930402745068674 ) ) ;
#30530=CARTESIAN_POINT ( 'NONE',  ( -4.789291700406336005, 116.8922783744782379, 0.1888386708474940334 ) ) ;
#30533=CARTESIAN_POINT ( 'NONE',  ( -6.994921376011119740, 121.9522545830452458, -0.1472782700081636809 ) ) ;
#30534=AXIS2_PLACEMENT_3D ( 'NONE', #590, #20557, #16955 ) ;
#30535=ORIENTED_EDGE ( 'NONE', *, *, #5534, .F. ) ;
#30537=CARTESIAN_POINT ( 'NONE',  ( -8.463766287105334740, 123.3219012665576315, -0.1265466038023452533 ) ) ;
#30538=CARTESIAN_POINT ( 'NONE',  ( 5.379112111825198106, -14.48849916137785776, 3.594839802689186570 ) ) ;
#30540=CARTESIAN_POINT ( 'NONE',  ( -9.409928955097594638, 157.3305555497073271, 1.526371511294253525 ) ) ;
#30541=CARTESIAN_POINT ( 'NONE',  ( 13.35680032055081057, 119.7032035076741465, 0.7543780172957895713 ) ) ;
#30542=CARTESIAN_POINT ( 'NONE',  ( 22.36672427266394791, 142.2114994846844240, -0.8677673306393176578 ) ) ;
#30543=CARTESIAN_POINT ( 'NONE',  ( 1.580769961479467911, 28.79261460129497863, -4.363931058323818668 ) ) ;
#30544=CARTESIAN_POINT ( 'NONE',  ( -20.65160272637294625, 152.5811724025633112, -0.7328296130731978275 ) ) ;
#30546=CARTESIAN_POINT ( 'NONE',  ( 4.812176722015626851, 117.4067824616802511, 1.197034441852249609 ) ) ;
#30547=ORIENTED_EDGE ( 'NONE', *, *, #1457, .T. ) ;
#30548=CARTESIAN_POINT ( 'NONE',  ( 2.192666673048648818, 116.2158040591487804, 0.09658723973292125675 ) ) ;
#30549=CARTESIAN_POINT ( 'NONE',  ( -17.34190353359467451, 148.5513402141484391, 1.530992562556359182 ) ) ;
#30551=CARTESIAN_POINT ( 'NONE',  ( 14.55733092780580051, 125.6573275863457866, -1.461954306844538642 ) ) ;
#30552=CARTESIAN_POINT ( 'NONE',  ( 0.7703063551133444431, -5.692625084440793515, -0.5956917769006077057 ) ) ;
#30553=CARTESIAN_POINT ( 'NONE',  ( -21.23477820244549363, 149.4807732621110006, -2.233729070194449218 ) ) ;
#30556=CARTESIAN_POINT ( 'NONE',  ( 0.5902664527119602100, 120.3589971203204669, -0.3461335206401334186 ) ) ;
#30559=CARTESIAN_POINT ( 'NONE',  ( -14.20821676177101267, 128.5469532985352714, -2.008711173933038996 ) ) ;
#30560=CARTESIAN_POINT ( 'NONE',  ( 3.609959606426583978, -15.77075149864894144, 4.467226954163184161 ) ) ;
#30562=CARTESIAN_POINT ( 'NONE',  ( -4.504028277950688164, 118.0871507785312815, -0.7872802139486386741 ) ) ;
#30565=CARTESIAN_POINT ( 'NONE',  ( 0.8698789912701805349, 157.1975648536147787, 1.511617766987151557 ) ) ;
#30567=AXIS2_PLACEMENT_3D ( 'NONE', #15488, #21438, #25076 ) ;
#30569=CARTESIAN_POINT ( 'NONE',  ( 6.894732321505262718, 117.1676844715483270, 0.1377731603346603051 ) ) ;
#30570=CARTESIAN_POINT ( 'NONE',  ( 4.698174212119619497, 9.136213905105968536, -7.004248122051734526 ) ) ;
#30571=CARTESIAN_POINT ( 'NONE',  ( 6.481656071630105487, 121.7133186976561205, 0.3761587846782802891 ) ) ;
#30572=CARTESIAN_POINT ( 'NONE',  ( 12.94589274040318472, 156.9034992427187376, -0.7570359663163892527 ) ) ;
#30573=EDGE_CURVE ( 'NONE', #1213, #35331, #1218, .T. ) ;
#30578=CARTESIAN_POINT ( 'NONE',  ( -13.67717291712373751, 119.6429072192227494, -0.2244666789651031946 ) ) ;
#30579=VERTEX_POINT ( 'NONE', #9369 ) ;
#30581=CARTESIAN_POINT ( 'NONE',  ( 5.882867916042628487, 121.3061504640725587, -0.1808544764108790948 ) ) ;
#30584=CARTESIAN_POINT ( 'NONE',  ( 2.811900354768880117, 118.7629491485453883, -1.088252837335328627 ) ) ;
#30585=CARTESIAN_POINT ( 'NONE',  ( -0.6512579105866077578, 156.3106852680424765, -0.2006220687487342003 ) ) ;
#30586=CARTESIAN_POINT ( 'NONE',  ( 4.342152980699533593, -13.79257992285246104, 4.116713196511041950 ) ) ;
#30587=CARTESIAN_POINT ( 'NONE',  ( -14.62453491845912623, 121.8773232776577942, 0.9418922607927827650 ) ) ;
#30588=CARTESIAN_POINT ( 'NONE',  ( -9.104209967888042598, 153.9432936505793066, -0.1819237819739442652 ) ) ;
#30589=CARTESIAN_POINT ( 'NONE',  ( 14.83769995734835412, 120.3134675335783754, 0.3991467459773894166 ) ) ;
#30591=CARTESIAN_POINT ( 'NONE',  ( 4.529186081025091681, -11.15152372915077095, -0.9203776863585164669 ) ) ;
#30592=CARTESIAN_POINT ( 'NONE',  ( -16.86202032626315628, 155.2029898760372646, -0.3369432954968343275 ) ) ;
#30597=CARTESIAN_POINT ( 'NONE',  ( 8.253395472087738938, 120.2163864936747331, 1.448344939060297154 ) ) ;
#30599=CARTESIAN_POINT ( 'NONE',  ( -4.567530434605131084, -10.44214056487004250, 0.7003524306260878740 ) ) ;
#30600=CARTESIAN_POINT ( 'NONE',  ( 11.09758427587538954, 119.2389763063149388, 1.130321237809625456 ) ) ;
#30602=CARTESIAN_POINT ( 'NONE',  ( 13.44735859403575873, 121.7711344121973411, -1.154596522737721953 ) ) ;
#30603=CARTESIAN_POINT ( 'NONE',  ( -3.942997264624582776, -11.51663297089948479, -2.426127359622226809 ) ) ;
#30604=CARTESIAN_POINT ( 'NONE',  ( -22.22261828963542740, 149.8733841865972920, -1.744734864234218863 ) ) ;
#30606=CARTESIAN_POINT ( 'NONE',  ( -15.76950829013782496, 146.9135488020124001, 0.01503653553346940078 ) ) ;
#30607=CARTESIAN_POINT ( 'NONE',  ( 6.371418708240476292, -13.42079056852439578, 0.8326245159988630018 ) ) ;
#30608=CARTESIAN_POINT ( 'NONE',  ( 4.911219615879212519, 115.6909491485453145, 1.456365542632356513 ) ) ;
#30609=CARTESIAN_POINT ( 'NONE',  ( -4.438458786732819128, 110.9173261775273716, -3.021370786321469382 ) ) ;
#30611=CARTESIAN_POINT ( 'NONE',  ( 18.57576200519309495, 149.2887123452801745, 2.480868434872863570 ) ) ;
#30614=CARTESIAN_POINT ( 'NONE',  ( -14.01781138111955194, 120.5923583732999873, 0.6175494627556293858 ) ) ;
#30615=CARTESIAN_POINT ( 'NONE',  ( -7.798946185677827714, 9.198776092563324625, 3.184250115244839030 ) ) ;
#30616=CARTESIAN_POINT ( 'NONE',  ( 15.88363809060971654, 147.6644253265642135, 1.281895537487840686 ) ) ;
#30618=AXIS2_PLACEMENT_3D ( 'NONE', #8302, #21898, #38328 ) ;
#30619=CARTESIAN_POINT ( 'NONE',  ( 15.42235106321962768, 121.0727120035890323, -0.2994195231956989778 ) ) ;
#30622=SURFACE_STYLE_USAGE ( .BOTH. , #8049 ) ;
#30626=CARTESIAN_POINT ( 'NONE',  ( -4.163803051339170835, 118.2394256923515172, 0.2270854623594056043 ) ) ;
#30627=FACE_OUTER_BOUND ( 'NONE', #22284, .T. ) ;
#30630=CARTESIAN_POINT ( 'NONE',  ( -4.001816602806133716, 119.1496993116277423, -0.9235019185135577846 ) ) ;
#30631=CARTESIAN_POINT ( 'NONE',  ( -4.396974916608651363, 111.2411499886600268, -3.139452135551013434 ) ) ;
#30632=CARTESIAN_POINT ( 'NONE',  ( 4.154030820756847930, 118.2394444196112175, 0.3904055952957847242 ) ) ;
#30633=CARTESIAN_POINT ( 'NONE',  ( -0.7026863963000727908, 156.4221767039705071, -0.7130674712139343230 ) ) ;
#30634=CARTESIAN_POINT ( 'NONE',  ( -1.287351889385697445, 115.7028695692513622, -1.739237698640231145 ) ) ;
#30636=CARTESIAN_POINT ( 'NONE',  ( 0.5993613099093353380, 117.9496052370437837, -1.382670436843215889 ) ) ;
#30638=CARTESIAN_POINT ( 'NONE',  ( 5.634266555046360203, 117.9149360781225937, -0.5245629147119164060 ) ) ;
#30639=CARTESIAN_POINT ( 'NONE',  ( -1.480437121830183278, 120.3785564700922492, -0.4209679054048330316 ) ) ;
#30640=CARTESIAN_POINT ( 'NONE',  ( 5.329260751456349254, 104.6144662015457527, 0.2904590649852882289 ) ) ;
#30642=DIRECTION ( 'NONE',  ( 0.9998004120163609398, 0.000000000000000000, 0.01997839162482749689 ) ) ;
#30643=CARTESIAN_POINT ( 'NONE',  ( -0.6547363933663787883, 120.9971525928537801, 0.08613384396314510694 ) ) ;
#30644=CARTESIAN_POINT ( 'NONE',  ( 5.010184479710102501, 117.3993854065330851, 0.7504461923096029663 ) ) ;
#30645=CARTESIAN_POINT ( 'NONE',  ( 14.90772019895836742, 120.8072429308574414, 0.9794594453158805836 ) ) ;
#30647=CARTESIAN_POINT ( 'NONE',  ( 1.978641239374031136, -15.23252017110923795, 5.293569756250467329 ) ) ;
#30648=CARTESIAN_POINT ( 'NONE',  ( 0.4065252312483833563, 117.6538564835029206, -0.4930844833531825566 ) ) ;
#30649=CARTESIAN_POINT ( 'NONE',  ( -2.416701088390952101, 119.2205458019918751, 0.6800916218662637069 ) ) ;
#30650=CARTESIAN_POINT ( 'NONE',  ( -0.4837089014371968032, -0.2951250844416551944, 0.8451309203121293301 ) ) ;
#30651=CARTESIAN_POINT ( 'NONE',  ( -0.3303419930535180238, 116.8490449975401617, -0.2909865916005162645 ) ) ;
#30652=CARTESIAN_POINT ( 'NONE',  ( -0.9201843903949125103, 16.76996313919548598, -0.3265437062991076722 ) ) ;
#30653=ORIENTED_EDGE ( 'NONE', *, *, #22449, .F. ) ;
#30655=CARTESIAN_POINT ( 'NONE',  ( -15.56233417011326914, 148.0963874134046705, 0.5341686659567149720 ) ) ;
#30656=CARTESIAN_POINT ( 'NONE',  ( 3.467186027297813666, -14.69398785160878873, 5.340258725024584763 ) ) ;
#30657=CARTESIAN_POINT ( 'NONE',  ( 2.594326071755596264, 120.1437993944865354, -0.4899928688880347272 ) ) ;
#30659=DIRECTION ( 'NONE',  ( -0.9998004120163608288, 0.000000000000000000, -0.01997839162482749342 ) ) ;
#30660=CARTESIAN_POINT ( 'NONE',  ( 3.361318737587208005, -13.21634134694392415, 1.934622048986600840 ) ) ;
#30662=CARTESIAN_POINT ( 'NONE',  ( 1.612929917264537716, 120.9971453638330985, 0.006532979378300353239 ) ) ;
#30664=CARTESIAN_POINT ( 'NONE',  ( 2.584978638890189195, 158.3255140430775043, 1.682483135129623220 ) ) ;
#30665=CARTESIAN_POINT ( 'NONE',  ( 3.100266737524950855, 108.5668738132174980, 4.179634342183701001 ) ) ;
#30668=CARTESIAN_POINT ( 'NONE',  ( 0.02874440110933761117, 158.8294072187990196, -1.438487372358303151 ) ) ;
#30669=CARTESIAN_POINT ( 'NONE',  ( 16.06481930096618527, 121.2308719818149712, 0.1605585295567895088 ) ) ;
#30672=CARTESIAN_POINT ( 'NONE',  ( 1.867637906597176212, -15.52365582206542705, 5.409599005316564124 ) ) ;
#30673=CARTESIAN_POINT ( 'NONE',  ( 4.973152232786927307, 117.3993868326352015, 0.9753084504214339923 ) ) ;
#30675=CARTESIAN_POINT ( 'NONE',  ( -4.750738626650226948, 117.8973642380069009, 0.7609203212133225369 ) ) ;
#30676=ORIENTED_EDGE ( 'NONE', *, *, #37510, .T. ) ;
#30677=CARTESIAN_POINT ( 'NONE',  ( 5.158690622980511620, 18.63085216599767691, -6.696816702733363158 ) ) ;
#30678=CARTESIAN_POINT ( 'NONE',  ( 3.286808489197310390, 118.4247336556115755, -0.7816159185997836323 ) ) ;
#30679=CARTESIAN_POINT ( 'NONE',  ( -4.364892838101932071, 123.4689364668338385, -0.1663115080531033796 ) ) ;
#30680=CARTESIAN_POINT ( 'NONE',  ( 4.771985164551651337, 117.7362450968562513, 1.071331016765174393 ) ) ;
#30682=CARTESIAN_POINT ( 'NONE',  ( -0.005099097579550932770, 122.5569158606516993, 0.2551796940111170642 ) ) ;
#30683=CARTESIAN_POINT ( 'NONE',  ( -4.627450822138572839, 2.892058097378844117, -0.1328416527703782657 ) ) ;
#30684=CARTESIAN_POINT ( 'NONE',  ( -5.277062234826722431, 115.6909491485453003, 0.8093865127289260331 ) ) ;
#30685=CARTESIAN_POINT ( 'NONE',  ( 3.041920762657289057, -14.42862556718194078, 4.364129476586208867 ) ) ;
#30686=CARTESIAN_POINT ( 'NONE',  ( 4.148164184366611273, 118.0988315448752530, -0.6394906134413953502 ) ) ;
#30687=CARTESIAN_POINT ( 'NONE',  ( 1.995069716065772658, 37.04168019532015421, 1.843784556858777846 ) ) ;
#30688=CARTESIAN_POINT ( 'NONE',  ( -0.9905630945189539682, 115.7029491485453576, 1.712266955583646721 ) ) ;
#30690=CARTESIAN_POINT ( 'NONE',  ( -4.306318207249558938, 105.1217634520768343, -3.167947131901895030 ) ) ;
#30691=CARTESIAN_POINT ( 'NONE',  ( 3.858334187661429215, -15.75373651934012997, 4.144460154494749915 ) ) ;
#30692=CARTESIAN_POINT ( 'NONE',  ( -1.243168248769069617, 118.5604221528582372, 0.6402677339867958173 ) ) ;
#30694=CARTESIAN_POINT ( 'NONE',  ( -0.7403349074254782503, 24.03625360216656404, 0.6378939806667418555 ) ) ;
#30697=DIRECTION ( 'NONE',  ( -4.017660918040594346E-17, 1.000000000000000000, 2.376309959284834438E-19 ) ) ;
#30698=CARTESIAN_POINT ( 'NONE',  ( 1.417747896749451231, 115.2915405621345144, 1.855271064302983275 ) ) ;
#30700=CARTESIAN_POINT ( 'NONE',  ( -0.7813136802280215010, 156.5584078035761593, 0.9574549430346845913 ) ) ;
#30702=CARTESIAN_POINT ( 'NONE',  ( 4.577529327193063935, 118.0358422625909327, -0.6747486238782739454 ) ) ;
#30703=CARTESIAN_POINT ( 'NONE',  ( 17.70889067045657228, 148.6960320134204210, -1.618934763233637497 ) ) ;
#30705=CARTESIAN_POINT ( 'NONE',  ( -20.10333444936999214, 149.6821479856479300, -2.421853341415478145 ) ) ;
#30707=CARTESIAN_POINT ( 'NONE',  ( 4.166221732904972441, 118.2394651950648097, -0.2241750351714766332 ) ) ;
#30708=CARTESIAN_POINT ( 'NONE',  ( 10.55375732331616767, 153.0603347025997323, -0.3251829154788380416 ) ) ;
#30710=CARTESIAN_POINT ( 'NONE',  ( 2.460727335429193197, -15.06314154744310585, 4.845259171755021299 ) ) ;
#30714=CARTESIAN_POINT ( 'NONE',  ( 1.294644163514462987, -7.843371450943685375, 4.453423563430108700 ) ) ;
#30715=CARTESIAN_POINT ( 'NONE',  ( 13.21686059441242911, 128.5100244389050204, 1.738961528769450648 ) ) ;
#30716=CARTESIAN_POINT ( 'NONE',  ( 1.747231708741132872, 35.57765484641747378, 2.108037137287274820 ) ) ;
#30717=CARTESIAN_POINT ( 'NONE',  ( -6.300951452924162588, 121.9812576474260055, 0.03014847038595266579 ) ) ;
#30718=AXIS2_PLACEMENT_3D ( 'NONE', #34938, #41540, #8309 ) ;
#30720=CARTESIAN_POINT ( 'NONE',  ( -1.214995109038484067, 0.9429784454696930052, -4.460028654918597901 ) ) ;
#30721=CARTESIAN_POINT ( 'NONE',  ( 8.053145991180159058, 122.8529229587361442, 0.1924930237977969527 ) ) ;
#30724=CIRCLE ( 'NONE', #23135, 5.588000000000006295 ) ;
#30726=CARTESIAN_POINT ( 'NONE',  ( 2.165901765101517107, 116.3326876175183600, -0.1937117289139740073 ) ) ;
#30727=CARTESIAN_POINT ( 'NONE',  ( 0.005880675324072524163, 122.2435587914035295, -0.2942930402744691754 ) ) ;
#30729=CARTESIAN_POINT ( 'NONE',  ( 1.822811606207358492, -15.29362660170948374, 5.402418844745950466 ) ) ;
#30731=CARTESIAN_POINT ( 'NONE',  ( 2.430217625452450569, 5.689826410578260329, 8.062849060857743666 ) ) ;
#30732=DIRECTION ( 'NONE',  ( 0.01997839162482749689, 1.040247600000945640E-18, -0.9998004120163610509 ) ) ;
#30733=CARTESIAN_POINT ( 'NONE',  ( -15.19943428492320869, 148.1072807477730748, -0.3037208696559880461 ) ) ;
#30735=CARTESIAN_POINT ( 'NONE',  ( 0.004379098344251805552, 122.8649044353672934, -0.2191479880734040764 ) ) ;
#30736=CARTESIAN_POINT ( 'NONE',  ( -2.823947636868171074, 116.6946238705719594, 0.1909394059425172097 ) ) ;
#30740=DIRECTION ( 'NONE',  ( -0.9998004120163608288, 0.000000000000000000, -0.01997839162482750383 ) ) ;
#30741=CARTESIAN_POINT ( 'NONE',  ( -7.552512487614272629, 122.4261604937442485, -0.1509171734833087142 ) ) ;
#30742=CARTESIAN_POINT ( 'NONE',  ( 5.719270376754757912, -14.62604927220606577, 2.811085246033490304 ) ) ;
#30743=CARTESIAN_POINT ( 'NONE',  ( -0.01051220311291028477, 117.9844940561907265, 0.5260736299896252577 ) ) ;
#30744=CARTESIAN_POINT ( 'NONE',  ( 22.28974849274159453, 149.2301036976659816, -0.9981255638314733281 ) ) ;
#30745=CARTESIAN_POINT ( 'NONE',  ( -4.636761822055341042, 12.60011390031314349, 0.2095705037016724059 ) ) ;
#30746=CARTESIAN_POINT ( 'NONE',  ( -10.77008264951280836, 157.9328640892066460, -0.4716003899658737786 ) ) ;
#30749=CARTESIAN_POINT ( 'NONE',  ( 5.562477116651607822, 116.6983427989447648, 0.1303901686245120817 ) ) ;
#30750=CARTESIAN_POINT ( 'NONE',  ( -11.15120438727553420, 123.3376105302527037, 1.132373765670515509 ) ) ;
#30752=CARTESIAN_POINT ( 'NONE',  ( 8.255438862926419930, 156.5149677146980309, -1.736665298733278684 ) ) ;
#30753=CARTESIAN_POINT ( 'NONE',  ( -21.09420047167898460, 149.7512365312068709, -2.228874019815534346 ) ) ;
#30757=CARTESIAN_POINT ( 'NONE',  ( 9.877746432283215583, 123.9483309312939099, -0.5948279539607076449 ) ) ;
#30759=CARTESIAN_POINT ( 'NONE',  ( -5.054692016413513400, 119.8577235299091228, -1.014870397641471689 ) ) ;
#30760=CARTESIAN_POINT ( 'NONE',  ( 2.350550293776238586, -15.63281720864678803, 5.143235457246400522 ) ) ;
#30761=CARTESIAN_POINT ( 'NONE',  ( -4.478377892402201077, 118.1173504798736644, -0.7356672007679183611 ) ) ;
#30765=CARTESIAN_POINT ( 'NONE',  ( 18.11030164959022670, 147.2296321676236062, 2.344458923443068610 ) ) ;
#30768=CARTESIAN_POINT ( 'NONE',  ( 22.53594553814337687, 150.7843406352268687, 0.4248312833800683141 ) ) ;
#30769=ADVANCED_FACE ( 'NONE', ( #22333 ), #39648, .T. ) ;
#30770=CARTESIAN_POINT ( 'NONE',  ( -2.728255833603390190, 14.33847684266025801, 7.992727065595903291 ) ) ;
#30771=CARTESIAN_POINT ( 'NONE',  ( 15.59067940631263482, 147.5518517437054982, 0.7624272054715746094 ) ) ;
#30774=CARTESIAN_POINT ( 'NONE',  ( 0.07232897131671378599, 118.7629491485454025, 1.278895008221504037 ) ) ;
#30778=CARTESIAN_POINT ( 'NONE',  ( -8.216694157412884891, 117.5064756823292385, -0.07510791844681385943 ) ) ;
#30781=CARTESIAN_POINT ( 'NONE',  ( -7.857536959375756247, 122.2102078284459310, -0.7978630961384953757 ) ) ;
#30784=CARTESIAN_POINT ( 'NONE',  ( 0.6338829882054587417, 115.7029520802098688, -1.736985041732382440 ) ) ;
#30785=CARTESIAN_POINT ( 'NONE',  ( -8.124409605001968515, 122.8458379852381910, -0.3720714147651331127 ) ) ;
#30786=CARTESIAN_POINT ( 'NONE',  ( 2.266344692909419312, -15.23424214381746644, 5.932772278557574275 ) ) ;
#30787=CARTESIAN_POINT ( 'NONE',  ( -13.98214753592677795, 155.8415165211600595, 1.292431576881029054 ) ) ;
#30789=CARTESIAN_POINT ( 'NONE',  ( 8.209937203459256594, 117.5146787832509858, 0.2970838962712568088 ) ) ;
#30790=CARTESIAN_POINT ( 'NONE',  ( 8.462070910903001675, 123.3219020322049460, 0.2116625524504351652 ) ) ;
#30791=ORIENTED_EDGE ( 'NONE', *, *, #41566, .F. ) ;
#30792=CARTESIAN_POINT ( 'NONE',  ( -0.2901879621234837447, 21.01165217803846730, -0.9340445150429393939 ) ) ;
#30793=CARTESIAN_POINT ( 'NONE',  ( -21.67415503129015164, 132.7302833492884417, -0.4548691923922797420 ) ) ;
#30795=AXIS2_PLACEMENT_3D ( 'NONE', #41271, #5287, #18031 ) ;
#30798=ORIENTED_EDGE ( 'NONE', *, *, #4010, .T. ) ;
#30799=CARTESIAN_POINT ( 'NONE',  ( -3.652649686639886095, 117.9385129362550231, 0.7594146576452507347 ) ) ;
#30800=CARTESIAN_POINT ( 'NONE',  ( -4.503669762702418033, -0.7216326387320324276, 1.072590735790061922 ) ) ;
#30801=CARTESIAN_POINT ( 'NONE',  ( 15.42726980375949175, 123.0316835747794642, 1.591438994230371051 ) ) ;
#30803=CARTESIAN_POINT ( 'NONE',  ( 14.64490033095721344, 154.5799843816573684, -1.633817034445553817 ) ) ;
#30804=CARTESIAN_POINT ( 'NONE',  ( 2.362155674307470310, -13.89060443905824371, -3.983575812745122846 ) ) ;
#30805=CARTESIAN_POINT ( 'NONE',  ( -8.039955067133034206, 118.1206512225135015, -0.9611422114813541473 ) ) ;
#30806=CARTESIAN_POINT ( 'NONE',  ( 4.841609353578014918, 117.6754506260240731, -0.8982756364806089300 ) ) ;
#30809=CARTESIAN_POINT ( 'NONE',  ( -15.30649785019675768, 148.0176312819745874, 0.02196777213629045461 ) ) ;
#30811=CARTESIAN_POINT ( 'NONE',  ( 6.400388595320081642, -14.10124341269280990, -0.01754875274584842895 ) ) ;
#30813=DIRECTION ( 'NONE',  ( 0.9998004120163609398, 0.000000000000000000, 0.01997839162482749689 ) ) ;
#30815=ADVANCED_FACE ( 'NONE', ( #28950 ), #38833, .F. ) ;
#30816=CARTESIAN_POINT ( 'NONE',  ( -4.605933908340293925, 113.9922470800784424, -2.135287817726405191 ) ) ;
#30817=VERTEX_POINT ( 'NONE', #40400 ) ;
#30818=CARTESIAN_POINT ( 'NONE',  ( 16.38264815551527320, 131.4813445454897192, 2.297577408150382805 ) ) ;
#30822=CARTESIAN_POINT ( 'NONE',  ( -1.702772465368850519, 120.1914007830323214, 0.4659475787731968133 ) ) ;
#30823=CARTESIAN_POINT ( 'NONE',  ( 7.903470162808407196, 13.94468365673557742, -2.927854470364564587 ) ) ;
#30824=CARTESIAN_POINT ( 'NONE',  ( 16.25331603292275418, 145.9442052555630767, 1.443193537303810281 ) ) ;
#30826=CARTESIAN_POINT ( 'NONE',  ( 7.924482676426827688, 158.6683511845044734, -0.3722227806660350358 ) ) ;
#30829=DIRECTION ( 'NONE',  ( -0.9998004120163609398, 0.000000000000000000, -0.01997839162482749689 ) ) ;
#30831=DIRECTION ( 'NONE',  ( -4.017660918040594346E-17, 1.000000000000000000, 2.376309959284834438E-19 ) ) ;
#30832=CARTESIAN_POINT ( 'NONE',  ( -4.292345225184465818, 118.2141485745093803, 0.3519745603735880413 ) ) ;
#30833=CARTESIAN_POINT ( 'NONE',  ( 3.563749620457647538, 109.2372012348777304, -3.773699991306081802 ) ) ;
#30834=VERTEX_POINT ( 'NONE', #2045 ) ;
#30836=CARTESIAN_POINT ( 'NONE',  ( -6.193434541464478471, 119.7369822425514343, -1.238341368285690303 ) ) ;
#30837=CARTESIAN_POINT ( 'NONE',  ( -3.418449710216219906, 108.6681208952157078, -4.126741282752677265 ) ) ;
#30839=CARTESIAN_POINT ( 'NONE',  ( 4.262834682690650467, 118.2124901016074432, 0.5347958070508012085 ) ) ;
#30840=CARTESIAN_POINT ( 'NONE',  ( -10.66982511086002994, 153.0728289088170300, -0.9866062039827815378 ) ) ;
#30844=CARTESIAN_POINT ( 'NONE',  ( 4.619096255015035624, 27.05588869245799089, -0.3994036469054788596 ) ) ;
#30845=CARTESIAN_POINT ( 'NONE',  ( -9.825947633753887800, 123.3250567171901082, -1.189973159844530892 ) ) ;
#30849=EDGE_CURVE ( 'NONE', #5326, #3642, #36046, .T. ) ;
#30851=CARTESIAN_POINT ( 'NONE',  ( -7.802235114625140966, 122.5634249805564338, 0.05936801018636322924 ) ) ;
#30852=CARTESIAN_POINT ( 'NONE',  ( 3.682264917456193665, 65.62546620154573418, 0.07358041635424013294 ) ) ;
#30853=CARTESIAN_POINT ( 'NONE',  ( 14.69808362324402395, 120.8948172685174001, 1.121060376578428386 ) ) ;
#30855=CARTESIAN_POINT ( 'NONE',  ( 3.220330141560203696, -14.30903721375789317, 2.546581355196453345 ) ) ;
#30856=CARTESIAN_POINT ( 'NONE',  ( 5.880040083609218371, 118.0670013439590491, -0.7714800252663617242 ) ) ;
#30857=CARTESIAN_POINT ( 'NONE',  ( -13.69950719238985393, 125.8243951943327517, 1.418320022125399316 ) ) ;
#30858=CARTESIAN_POINT ( 'NONE',  ( -0.9317526520580600158, -11.96253880033681050, -0.2928614735302202954 ) ) ;
#30859=CARTESIAN_POINT ( 'NONE',  ( -15.60190333658779771, 121.2802728028965475, -0.9237637308081628751 ) ) ;
#30860=CARTESIAN_POINT ( 'NONE',  ( 0.9071407760921452734, 21.51634675185595924, 0.3571511405359465430 ) ) ;
#30863=CARTESIAN_POINT ( 'NONE',  ( -15.82779737147856025, 147.6293441119438512, 0.5318544519934518267 ) ) ;
#30864=CARTESIAN_POINT ( 'NONE',  ( 4.721845526343314781, -13.23797770169883670, 3.222865150663026590 ) ) ;
#30865=CARTESIAN_POINT ( 'NONE',  ( 5.134369219807886964, 120.3680889145531552, -0.6721547394862479319 ) ) ;
#30868=CARTESIAN_POINT ( 'NONE',  ( 0.5151297239306589226, 115.7029491485453434, 1.762079848971026763 ) ) ;
#30870=CARTESIAN_POINT ( 'NONE',  ( 3.254806331274714637, -13.89383896039994504, 2.504907480430248246 ) ) ;
#30871=CARTESIAN_POINT ( 'NONE',  ( -4.767505756759218727, 117.8468658059388900, -0.9622486164732443337 ) ) ;
#30872=CARTESIAN_POINT ( 'NONE',  ( 9.048378227557773101, 123.9859359328134190, 0.09628433740681516251 ) ) ;
#30873=EDGE_CURVE ( 'NONE', #18999, #12743, #4079, .T. ) ;
#30875=CARTESIAN_POINT ( 'NONE',  ( 15.34515231418505365, 125.4902479783272184, 1.998699669873516882 ) ) ;
#30880=CARTESIAN_POINT ( 'NONE',  ( 0.02156534543286487207, 156.6359106937186709, -1.079218069903262300 ) ) ;
#30881=CARTESIAN_POINT ( 'NONE',  ( 16.19138771800991350, 121.3864332154274877, 0.1624333549846388725 ) ) ;
#30884=CARTESIAN_POINT ( 'NONE',  ( 2.015967980637507928, -15.45937876265861277, 5.999498870620294966 ) ) ;
#30886=CARTESIAN_POINT ( 'NONE',  ( -6.682056005205734733E-14, 110.9644662015457328, 1.123945309419055369E-18 ) ) ;
#30887=CARTESIAN_POINT ( 'NONE',  ( -4.843431534479017309, 117.8278034786011972, 0.6983875874824077012 ) ) ;
#30891=CARTESIAN_POINT ( 'NONE',  ( 2.584482069992259490, 117.5998511199927776, -0.6690006159187619206 ) ) ;
#30892=CARTESIAN_POINT ( 'NONE',  ( -2.231675704589730191, 117.6064948828932444, -1.117935386608752024 ) ) ;
#30894=CARTESIAN_POINT ( 'NONE',  ( 4.804053917469309987, 117.6427837140938806, 1.111766096040093910 ) ) ;
#30895=CARTESIAN_POINT ( 'NONE',  ( -4.757248700628498916, 117.4032733054477973, -1.206458840162573543 ) ) ;
#30896=CARTESIAN_POINT ( 'NONE',  ( -0.8427018527672123227, 121.5536190086353372, 0.3367535922268983795 ) ) ;
#30897=CARTESIAN_POINT ( 'NONE',  ( -4.478778176974228309, 3.316883148187759645, 1.141857468124592101 ) ) ;
#30899=CARTESIAN_POINT ( 'NONE',  ( -3.204561054529846853, 108.0377196974498872, -4.255356325961729524 ) ) ;
#30900=CARTESIAN_POINT ( 'NONE',  ( 2.390819523577490280, -14.89105559343156848, 5.112470274569719919 ) ) ;
#30902=CARTESIAN_POINT ( 'NONE',  ( 3.905206024139304066, 115.3331674797404247, -1.578293011005953650 ) ) ;
#30903=CARTESIAN_POINT ( 'NONE',  ( -0.5637839999484974829, 35.87001837459851572, 2.917945788214682423 ) ) ;
#30904=CARTESIAN_POINT ( 'NONE',  ( -1.153367143837488618, 115.7029425286913238, 1.700742857507489214 ) ) ;
#30905=CARTESIAN_POINT ( 'NONE',  ( -3.453265078539333288, 21.00871511114837276, -3.102408547967784092 ) ) ;
#30907=CARTESIAN_POINT ( 'NONE',  ( -5.314278422745060126, 105.1224610256965235, 0.4583187270701635785 ) ) ;
#30908=AXIS2_PLACEMENT_3D ( 'NONE', #20107, #15992, #10031 ) ;
#30909=CARTESIAN_POINT ( 'NONE',  ( 4.539898764682361865, -15.38453816280940778, 0.3562021009913567959 ) ) ;
#30910=CARTESIAN_POINT ( 'NONE',  ( -0.01152893261320283441, 118.7114655739656257, 0.5769549317675700673 ) ) ;
#30911=CARTESIAN_POINT ( 'NONE',  ( 0.8015440831811396771, 19.08345756868062892, -0.5584349385947994238 ) ) ;
#30914=CARTESIAN_POINT ( 'NONE',  ( -3.743815577281074614, 31.31851751214970037, -0.6207396561878217867 ) ) ;
#30915=CARTESIAN_POINT ( 'NONE',  ( 0.5453179846284311738, 107.9696733310005214, 4.488644025489749723 ) ) ;
#30917=CARTESIAN_POINT ( 'NONE',  ( -16.77814054344329620, 146.6545634508490821, 1.109899152166417657 ) ) ;
#30918=FACE_OUTER_BOUND ( 'NONE', #37393, .T. ) ;
#30920=CARTESIAN_POINT ( 'NONE',  ( 4.567598822338898579, 118.0323598375720877, -0.6818831079871943146 ) ) ;
#30921=CARTESIAN_POINT ( 'NONE',  ( 13.17493328878353509, 125.9194590699508893, -1.341157253524417170 ) ) ;
#30922=CARTESIAN_POINT ( 'NONE',  ( -11.20355582914615233, 156.1341193432522800, -2.130866455309295748 ) ) ;
#30925=CARTESIAN_POINT ( 'NONE',  ( 4.416202647269503068, 118.1792123024622896, -0.3908220537550897711 ) ) ;
#30926=CARTESIAN_POINT ( 'NONE',  ( 7.938918103923345626, 154.5997988942315260, -0.3378123388718580200 ) ) ;
#30928=CARTESIAN_POINT ( 'NONE',  ( 1.978641239374031136, -15.23252017110923795, 5.293569756250467329 ) ) ;
#30931=CARTESIAN_POINT ( 'NONE',  ( 2.990331240142678482, -7.206181497205274233, 3.547999066060627094 ) ) ;
#30932=CARTESIAN_POINT ( 'NONE',  ( 10.68802918394754897, 123.5542795626547417, 1.432819001183019969 ) ) ;
#30933=CARTESIAN_POINT ( 'NONE',  ( -0.8015897017430366756, 32.12766266987975428, 3.088637291698237863 ) ) ;
#30934=CARTESIAN_POINT ( 'NONE',  ( -6.874578817172170453, 121.8312213470058225, 0.01890686361714006766 ) ) ;
#30935=CARTESIAN_POINT ( 'NONE',  ( -4.515506726787251068, -6.291224493951820484, 1.111903093310195212 ) ) ;
#30936=CARTESIAN_POINT ( 'NONE',  ( -0.001367086239828292421, 156.3041635968983485, 0.06841458569046213190 ) ) ;
#30937=CARTESIAN_POINT ( 'NONE',  ( -1.690137127919513649, -8.491432666745847513, 8.270632449787910900 ) ) ;
#30939=CARTESIAN_POINT ( 'NONE',  ( 8.789005074032305131, 117.7562713746568193, -0.1097197802411318257 ) ) ;
#30940=CARTESIAN_POINT ( 'NONE',  ( 0.01046636459289907069, 120.7331730230139755, -0.5237796829255388920 ) ) ;
#30942=CARTESIAN_POINT ( 'NONE',  ( 2.008732664060283390, -15.70244684250787870, 5.701976698490780926 ) ) ;
#30944=CARTESIAN_POINT ( 'NONE',  ( 5.270772580891830650, -0.5842219557417941411, -6.616342194954959233 ) ) ;
#30945=CARTESIAN_POINT ( 'NONE',  ( 5.332911103893867022, 115.7029491485453150, 0.1077752590139453570 ) ) ;
#30946=DIRECTION ( 'NONE',  ( -5.206863593109713661E-17, 1.000000000000000000, -1.077750396879097183E-30 ) ) ;
#30947=CARTESIAN_POINT ( 'NONE',  ( 2.460727335429193197, -15.06314154744310585, 4.845259171755021299 ) ) ;
#30948=CARTESIAN_POINT ( 'NONE',  ( 0.09934209768992387224, 106.7790779034713324, -4.971484795507160825 ) ) ;
#30949=CARTESIAN_POINT ( 'NONE',  ( -5.835061174465498546, 117.1115750087645608, 0.2489150398414471388 ) ) ;
#30950=ORIENTED_EDGE ( 'NONE', *, *, #33097, .F. ) ;
#30954=CARTESIAN_POINT ( 'NONE',  ( -7.783246152616193569, 154.6561476914895081, -0.1555277812256514736 ) ) ;
#30955=CARTESIAN_POINT ( 'NONE',  ( 3.779930934242227369, -15.54964480308611208, 5.049599803682278676 ) ) ;
#30956=CARTESIAN_POINT ( 'NONE',  ( -0.02969037535081191920, 158.7301711276701894, 1.485827791648137497 ) ) ;
#30957=CARTESIAN_POINT ( 'NONE',  ( 10.29385411648718396, 157.8242135995235458, -0.8711791838966669310 ) ) ;
#30958=CARTESIAN_POINT ( 'NONE',  ( 3.043391175932955495, 18.63480288530714191, -3.501419995799015528 ) ) ;
#30959=CARTESIAN_POINT ( 'NONE',  ( -15.60595500976395122, 121.0226940419799462, -0.7351363234501833155 ) ) ;
#30964=CARTESIAN_POINT ( 'NONE',  ( -7.383627470571842544, 120.8389031223305352, 0.9130476668403029183 ) ) ;
#30966=CARTESIAN_POINT ( 'NONE',  ( 12.45504352496358003, 122.8403290575659526, -1.325700600460794742 ) ) ;
#30967=CARTESIAN_POINT ( 'NONE',  ( -3.992970410919193025, 117.9114980025989752, -0.8736511219775315862 ) ) ;
#30969=EDGE_CURVE ( 'NONE', #2591, #11424, #28929, .T. ) ;
#30970=CARTESIAN_POINT ( 'NONE',  ( 1.739825554502939076, 156.3676537730497387, -0.7044751146431473821 ) ) ;
#30971=EDGE_LOOP ( 'NONE', ( #15735, #4446 ) ) ;
#30972=CARTESIAN_POINT ( 'NONE',  ( -18.24092514812192434, 147.9371514012413229, -2.391122828403475342 ) ) ;
#30973=CARTESIAN_POINT ( 'NONE',  ( 2.199016089875075686, -15.62526216655714428, 5.252760144517266916 ) ) ;
#30974=CARTESIAN_POINT ( 'NONE',  ( -4.345421273754075386, 118.1827543097632969, -0.6195030316670109283 ) ) ;
#30976=CARTESIAN_POINT ( 'NONE',  ( -4.953655876003494107, 117.5439441053769087, 0.8524319712158592299 ) ) ;
#30977=CARTESIAN_POINT ( 'NONE',  ( 11.39530606461018358, 123.1738952066917534, 1.661446624139454764 ) ) ;
#30978=DIRECTION ( 'NONE',  ( -4.017660918040594346E-17, 1.000000000000000000, 2.376309959284834438E-19 ) ) ;
#30979=CARTESIAN_POINT ( 'NONE',  ( 8.274862188802355689, -1.658786094895864149, -1.630640499628306372 ) ) ;
#30980=CARTESIAN_POINT ( 'NONE',  ( 15.39048793250114500, 143.5427300040290106, 0.9094471879209009568 ) ) ;
#30988=CARTESIAN_POINT ( 'NONE',  ( -17.17894352244484679, 122.7237354506536491, -0.1767255469942457524 ) ) ;
#30992=CARTESIAN_POINT ( 'NONE',  ( -5.768081145802491427, 121.1576386676896249, -0.5241667226324177031 ) ) ;
#30993=CARTESIAN_POINT ( 'NONE',  ( -7.931359276468322506, 121.9896588117074003, 0.6306316981394846088 ) ) ;
#30994=CARTESIAN_POINT ( 'NONE',  ( 2.857216417531940333, 115.6909491485452577, -1.572722873744161642 ) ) ;
#30995=CARTESIAN_POINT ( 'NONE',  ( -7.590630008422064812, 122.4062900713904440, -0.3515417406328248395 ) ) ;
#30996=CARTESIAN_POINT ( 'NONE',  ( 4.144384115003134639, -13.99490941865914806, 4.432938699676250316 ) ) ;
#30997=CARTESIAN_POINT ( 'NONE',  ( -1.273577801943225785, 159.1407128229522527, 1.197834500974594318 ) ) ;
#30999=CARTESIAN_POINT ( 'NONE',  ( 0.9036256862535075873, 116.4850453793277865, 0.1155468115323372985 ) ) ;
#31000=CARTESIAN_POINT ( 'NONE',  ( -0.0007136890092010687164, 156.3034662015457741, 0.03571591641522637445 ) ) ;
#31001=CARTESIAN_POINT ( 'NONE',  ( 0.4398701176286285985, 29.43434963188315834, -0.8729469796826672123 ) ) ;
#31002=CARTESIAN_POINT ( 'NONE',  ( -22.83278390340161934, 150.4073064562084880, -0.5330863269314417563 ) ) ;
#31003=CARTESIAN_POINT ( 'NONE',  ( 5.008145224984434485, 117.3993836135855418, -0.7758584094373792706 ) ) ;
#31006=CARTESIAN_POINT ( 'NONE',  ( -8.094215566179986610, 117.4700539287145631, -0.1617416914405450934 ) ) ;
#31008=CARTESIAN_POINT ( 'NONE',  ( 5.962972180698049129, 118.6887585580880398, 1.206927124751090208 ) ) ;
#31010=CARTESIAN_POINT ( 'NONE',  ( -0.008945125900511092729, 117.5133074443058945, 0.4476506782301716836 ) ) ;
#31012=CARTESIAN_POINT ( 'NONE',  ( 6.741874166124438794, 157.8130281244853279, -1.606654124060122424 ) ) ;
#31013=CARTESIAN_POINT ( 'NONE',  ( -0.7749869142727341398, -12.81603963768374044, -4.556214072895795830 ) ) ;
#31014=CARTESIAN_POINT ( 'NONE',  ( -21.15273274666908421, 151.2337125027825095, -1.710087910014103985 ) ) ;
#31015=CARTESIAN_POINT ( 'NONE',  ( 4.747437835475817103, 117.7228179995735502, -0.9150688999438771898 ) ) ;
#31016=EDGE_CURVE ( 'NONE', #13569, #14379, #4299, .T. ) ;
#31017=VERTEX_POINT ( 'NONE', #33326 ) ;
#31018=CARTESIAN_POINT ( 'NONE',  ( -9.164740666424060933, 153.8946005065304803, 0.1038620377607964856 ) ) ;
#31019=CARTESIAN_POINT ( 'NONE',  ( 4.434149479847604880, -15.45467793902401077, 4.427262213160148896 ) ) ;
#31020=( BOUNDED_SURFACE ( )  B_SPLINE_SURFACE ( 3, 2, ( 
 ( #20394, #8258, #40450 ),
 ( #14219, #14014, #4668 ),
 ( #20603, #27021, #30416 ),
 ( #7854, #23806, #20814 ),
 ( #33635, #34050, #36826 ),
 ( #10613, #7645, #37235 ),
 ( #14427, #11443, #11241 ),
 ( #27637, #24226, #34260 ),
 ( #4462, #7436, #17419 ),
 ( #4251, #27228, #8054 ),
 ( #17214, #40241, #11036 ),
 ( #24431, #21027, #27434 ),
 ( #1470, #33421, #18041 ),
 ( #30833, #37436, #26812 ),
 ( #840, #39820, #4880 ),
 ( #33840, #1680, #23595 ),
 ( #36617, #9314, #11658 ),
 ( #14844, #31892, #37654 ),
 ( #24864, #2520, #31464 ),
 ( #9108, #21860, #28272 ) ),
 .UNSPECIFIED., .F., .F., .T. ) 
 B_SPLINE_SURFACE_WITH_KNOTS ( ( 4, 2, 2, 2, 2, 2, 2, 2, 2, 4 ),
 ( 3, 3 ),
 ( 1.678480488279121552E-17, 0.0008043537003518050343, 0.001608707400703593372, 0.002413061101055381710, 0.003217414801407169830, 0.004021768501758958385, 0.004826122202110746939, 0.006434829602814323181, 0.009652244404221476531, 0.01286965920562862901 ),
 ( 0.000000000000000000, 1.000000000000000000 ),
 .UNSPECIFIED. ) 
 GEOMETRIC_REPRESENTATION_ITEM ( )  RATIONAL_B_SPLINE_SURFACE ( (
 ( 1.000000000000000000, 0.9815197824473206323, 1.000000000000000000),
 ( 1.000000000000000000, 0.9811767838555041088, 1.000000000000000000),
 ( 1.000000000000000000, 0.9804039767733835342, 1.000000000000000000),
 ( 1.000000000000000000, 0.9775760511973242695, 1.000000000000000000),
 ( 1.000000000000000000, 0.9755247961224483566, 1.000000000000000000),
 ( 1.000000000000000000, 0.9705275854478995212, 1.000000000000000000),
 ( 1.000000000000000000, 0.9675790768618311999, 1.000000000000000000),
 ( 1.000000000000000000, 0.9611010073753046834, 1.000000000000000000),
 ( 1.000000000000000000, 0.9576315359795163351, 1.000000000000000000),
 ( 1.000000000000000000, 0.9503812888595358777, 1.000000000000000000),
 ( 1.000000000000000000, 0.9466096088198014957, 1.000000000000000000),
 ( 1.000000000000000000, 0.9387890754370313839, 1.000000000000000000),
 ( 1.000000000000000000, 0.9347210935246765828, 1.000000000000000000),
 ( 1.000000000000000000, 0.9222591698861631881, 1.000000000000000000),
 ( 1.000000000000000000, 0.9133676415844801388, 1.000000000000000000),
 ( 1.000000000000000000, 0.8858621071945419478, 1.000000000000000000),
 ( 1.000000000000000000, 0.8667308185384640096, 1.000000000000000000),
 ( 1.000000000000000000, 0.8330124393854519971, 1.000000000000000000),
 ( 1.000000000000000000, 0.8190729568363664947, 1.000000000000000000),
 ( 1.000000000000000000, 0.8123912451051847894, 1.000000000000000000) ) ) 
 REPRESENTATION_ITEM ( '' )  SURFACE ( )  );
#31021=CARTESIAN_POINT ( 'NONE',  ( -6.405903822259908509, 29.15797647828624406, 0.04789268291063029231 ) ) ;
#31023=CARTESIAN_POINT ( 'NONE',  ( -2.549993051094809449, 117.9496054164201695, -1.337954177656600407 ) ) ;
#31026=ORIENTED_EDGE ( 'NONE', *, *, #38287, .F. ) ;
#31027=CARTESIAN_POINT ( 'NONE',  ( 17.42401203395154141, 135.4862447717955547, 2.417378365323842981 ) ) ;
#31030=CARTESIAN_POINT ( 'NONE',  ( -0.7241986523584001967, 107.9696733310005214, 4.463276061801071393 ) ) ;
#31031=CARTESIAN_POINT ( 'NONE',  ( -4.294125178196657622, -12.16697637372164564, -7.253078015393731981 ) ) ;
#31032=CARTESIAN_POINT ( 'NONE',  ( 10.97991518849985759, 126.1652090859982707, 0.9941924553172261092 ) ) ;
#31033=CARTESIAN_POINT ( 'NONE',  ( -4.792076001792309192, 115.6909491485453003, -1.475558552157980818 ) ) ;
#31034=CARTESIAN_POINT ( 'NONE',  ( 22.71566531765381569, 150.0520759213295889, -0.3958359165339124797 ) ) ;
#31041=DIRECTION ( 'NONE',  ( 4.017660918040594346E-17, -1.000000000000000000, -2.376309959284834438E-19 ) ) ;
#31042=CARTESIAN_POINT ( 'NONE',  ( -4.241115207526993558, 118.2240460336109464, 0.3200252020677880616 ) ) ;
#31043=CARTESIAN_POINT ( 'NONE',  ( 3.682264917456192332, 88.48546620154573361, 0.07358041635423968885 ) ) ;
#31044=ORIENTED_EDGE ( 'NONE', *, *, #33247, .T. ) ;
#31046=CARTESIAN_POINT ( 'NONE',  ( -6.136200860584644090, 119.6162947413529025, -1.249506624868057969 ) ) ;
#31047=CARTESIAN_POINT ( 'NONE',  ( -4.973569738608247803, 117.3993868453981548, -0.9750659555622913643 ) ) ;
#31048=CARTESIAN_POINT ( 'NONE',  ( 4.250260335411498502, 118.2244068006796169, 0.4633496807658996075 ) ) ;
#31049=CARTESIAN_POINT ( 'NONE',  ( -7.664053125822943180, 122.2986020547093915, -0.5896768268545020675 ) ) ;
#31050=DIRECTION ( 'NONE',  ( 0.01997839162482749342, 1.040247600000944484E-18, -0.9998004120163608288 ) ) ;
#31051=CARTESIAN_POINT ( 'NONE',  ( 17.31377588638417819, 122.7721875394316555, 0.3459704467065362055 ) ) ;
#31054=CARTESIAN_POINT ( 'NONE',  ( 1.141857472271699425, 24.90688314728939190, 4.478778191171412182 ) ) ;
#31055=CARTESIAN_POINT ( 'NONE',  ( -16.71293428529044078, 146.3384789841921361, -1.780605135160314045 ) ) ;
#31057=DIRECTION ( 'NONE',  ( -5.206863593109713661E-17, 1.000000000000000000, -1.077750396879097183E-30 ) ) ;
#31060=CARTESIAN_POINT ( 'NONE',  ( 6.069820211534818100, 121.4363512089535249, 0.2627894127678002678 ) ) ;
#31061=CARTESIAN_POINT ( 'NONE',  ( -0.2501726036287156840, 25.39126883368370002, -4.616104092076634302 ) ) ;
#31062=CARTESIAN_POINT ( 'NONE',  ( 22.48407052889629654, 149.9757045183965261, 1.524144198737067857 ) ) ;
#31064=CARTESIAN_POINT ( 'NONE',  ( 2.768784035434307178, -15.00486597294339930, 4.394545281259884639 ) ) ;
#31065=CARTESIAN_POINT ( 'NONE',  ( 4.947803190686594021, 118.0342071775839941, -0.7636311594363673905 ) ) ;
#31066=CARTESIAN_POINT ( 'NONE',  ( -8.076210525097467396, 156.3870133935118076, 1.723082682300313806 ) ) ;
#31067=CARTESIAN_POINT ( 'NONE',  ( -2.714482067202859561, 26.26591195808746448, -3.750338772627290762 ) ) ;
#31068=CARTESIAN_POINT ( 'NONE',  ( 0.008148259816488066104, 159.5682499516715040, -0.4077722408685185429 ) ) ;
#31069=CARTESIAN_POINT ( 'NONE',  ( 0.9467939684353117169, 21.72092434492431323, 0.2316696090552467224 ) ) ;
#31072=CARTESIAN_POINT ( 'NONE',  ( -7.714568708787910012, 122.2455405838764335, 0.3552802434219702321 ) ) ;
#31073=CARTESIAN_POINT ( 'NONE',  ( 5.309946395046844181, -12.59883844183437596, 1.960244440597288529 ) ) ;
#31074=CARTESIAN_POINT ( 'NONE',  ( 0.02400040557466523797, 156.7459281804771365, -1.201078436782489600 ) ) ;
#31077=CARTESIAN_POINT ( 'NONE',  ( 1.198181792750290464, 115.7029448766258781, 1.741964538748038027 ) ) ;
#31079=CARTESIAN_POINT ( 'NONE',  ( 2.120958618816386920, -15.04726689571640819, 5.287964242625700528 ) ) ;
#31080=CARTESIAN_POINT ( 'NONE',  ( -4.682896055009653224, 117.8402614876679309, -1.032663334385100384 ) ) ;
#31081=CARTESIAN_POINT ( 'NONE',  ( 9.076946558997631698, 124.0722828908287454, 0.1472919029216551157 ) ) ;
#31082=ORIENTED_EDGE ( 'NONE', *, *, #28468, .T. ) ;
#31083=CARTESIAN_POINT ( 'NONE',  ( 8.818906024077392658, 119.8693228481767932, 1.468947216590822391 ) ) ;
#31085=CARTESIAN_POINT ( 'NONE',  ( -6.603988835907287056E-14, 91.53346620154573543, -3.493462572467304738E-18 ) ) ;
#31087=ADVANCED_FACE ( 'NONE', ( #748 ), #35897, .F. ) ;
#31089=CARTESIAN_POINT ( 'NONE',  ( 15.61624682818904297, 120.8175431576145940, 0.1535658744814574483 ) ) ;
#31092=CARTESIAN_POINT ( 'NONE',  ( 1.782359092197000061, -15.48430479490869871, 5.418275911098993980 ) ) ;
#31094=CARTESIAN_POINT ( 'NONE',  ( -3.682264917456323339, 75.78546620154573077, -0.07358041635423923088 ) ) ;
#31095=CARTESIAN_POINT ( 'NONE',  ( -4.777430207200964674, 117.8484153795353393, 0.7997178450909804281 ) ) ;
#31100=CARTESIAN_POINT ( 'NONE',  ( 8.570152792252320850, 118.9011554048343129, -0.9064097239879936874 ) ) ;
#31101=CARTESIAN_POINT ( 'NONE',  ( -5.278237183132178600, 122.2451909684448310, -0.2611397421478203751 ) ) ;
#31102=CARTESIAN_POINT ( 'NONE',  ( 4.707096360283405723, 117.7228093591007365, 1.103996979757269514 ) ) ;
#31104=CARTESIAN_POINT ( 'NONE',  ( -1.034729067459851271, 124.2655319029901335, 0.03890078971358925525 ) ) ;
#31106=CARTESIAN_POINT ( 'NONE',  ( 1.686640475165922748, -9.627085671684914914, -4.319569293544198274 ) ) ;
#31110=CARTESIAN_POINT ( 'NONE',  ( 3.015147157152042290, -12.41699557045261670, 0.4662733852003331791 ) ) ;
#31111=CARTESIAN_POINT ( 'NONE',  ( 3.689824518792477637, 110.1236525333376619, -3.433021159709686909 ) ) ;
#31112=CARTESIAN_POINT ( 'NONE',  ( -3.748619050207897985, 28.91994025391836942, 2.520532616727765518 ) ) ;
#31113=CARTESIAN_POINT ( 'NONE',  ( -1.240271560838381637, 115.7029491485453576, 1.694587172447594936 ) ) ;
#31114=CARTESIAN_POINT ( 'NONE',  ( -2.707926769430928804, 11.08828375386998033, -3.745406074561137277 ) ) ;
#31116=CARTESIAN_POINT ( 'NONE',  ( -4.078417157467525200, 104.6144662015457811, -2.601001456789872712 ) ) ;
#31117=CARTESIAN_POINT ( 'NONE',  ( 4.228667402019948618, -15.40433107038223426, 0.8683934293704824725 ) ) ;
#31118=CARTESIAN_POINT ( 'NONE',  ( -11.07050914993725677, 156.0189320485970086, 1.715486126203028538 ) ) ;
#31119=CARTESIAN_POINT ( 'NONE',  ( 0.7511875256325919459, -11.68598654017788974, 0.6195722450943603743 ) ) ;
#31120=CARTESIAN_POINT ( 'NONE',  ( 0.7678286665867425365, 17.13787758575863762, 0.6011479000593502597 ) ) ;
#31125=CARTESIAN_POINT ( 'NONE',  ( -0.1065646865916383135, 105.8844662015456777, 5.332932678536313809 ) ) ;
#31126=CARTESIAN_POINT ( 'NONE',  ( -9.244484035386584253, 123.0263237342149978, 0.6646791600263458610 ) ) ;
#31128=CARTESIAN_POINT ( 'NONE',  ( 1.897380780832740532, -15.05783359004129984, 5.662421594695133287 ) ) ;
#31129=CARTESIAN_POINT ( 'NONE',  ( 8.333011053690729142, 121.0263440914440736, -1.031464938890432004 ) ) ;
#31130=CARTESIAN_POINT ( 'NONE',  ( -19.83855703208276466, 148.9191654756151024, -2.494779984669014183 ) ) ;
#31132=CARTESIAN_POINT ( 'NONE',  ( 4.123150137924818992, 118.2429491485453354, -0.1807919990337682747 ) ) ;
#31133=CARTESIAN_POINT ( 'NONE',  ( 7.065481736843126193, 122.0164807696326790, -0.1187983231582534355 ) ) ;
#31135=CARTESIAN_POINT ( 'NONE',  ( 1.822811606207361823, -15.29362660170947841, 5.402418844745947801 ) ) ;
#31136=CARTESIAN_POINT ( 'NONE',  ( -3.521685918548247418, 29.33394459973516888, 3.031038535435704340 ) ) ;
#31139=CARTESIAN_POINT ( 'NONE',  ( 4.587442282481145384, -5.694351208059624803, -0.5507456681084095251 ) ) ;
#31140=CARTESIAN_POINT ( 'NONE',  ( 0.7656893570837772778, 156.6562795458349910, 1.120391489380295535 ) ) ;
#31141=CARTESIAN_POINT ( 'NONE',  ( 0.8489375256178871565, 34.04538252295368039, 1.759639877157939347 ) ) ;
#31142=CARTESIAN_POINT ( 'NONE',  ( -7.618479139564732883, 124.9344662015457317, -0.1522353441811853947 ) ) ;
#31143=CARTESIAN_POINT ( 'NONE',  ( -2.948169924849943335, 1.592661447142720732, -3.562413953034572867 ) ) ;
#31144=CARTESIAN_POINT ( 'NONE',  ( 11.82813386268891165, 130.3161362890850512, 0.2363542639706544268 ) ) ;
#31145=CARTESIAN_POINT ( 'NONE',  ( 3.560122487986403517, 2.076091768892780909, 7.630420683349803390 ) ) ;
#31147=CARTESIAN_POINT ( 'NONE',  ( -5.523483301223560460, 116.8734833957022090, -0.5481978220757582898 ) ) ;
#31148=DIRECTION ( 'NONE',  ( -0.9998004120163608288, 0.000000000000000000, -0.01997839162482749342 ) ) ;
#31151=CARTESIAN_POINT ( 'NONE',  ( 2.739727753987758252, 28.35525327666260864, -3.728201022356329553 ) ) ;
#31153=CARTESIAN_POINT ( 'NONE',  ( 4.299309211086679738, 118.1588881536522564, 0.6869296180760711135 ) ) ;
#31154=DIRECTION ( 'NONE',  ( 0.9998004120163609398, 0.000000000000000000, 0.01997839162482749689 ) ) ;
#31156=CARTESIAN_POINT ( 'NONE',  ( 0.8039382690412617549, 120.8419495465347069, -0.4447074479469316222 ) ) ;
#31157=CARTESIAN_POINT ( 'NONE',  ( -22.28323889858847195, 137.0232865695268458, 0.2611169771296155684 ) ) ;
#31162=CARTESIAN_POINT ( 'NONE',  ( -0.6474952184382374298, 120.9973616653156512, 0.02013384967883425844 ) ) ;
#31163=CARTESIAN_POINT ( 'NONE',  ( 4.283822907657564016, -15.48171044555848930, 4.591852530049981063 ) ) ;
#31164=CARTESIAN_POINT ( 'NONE',  ( -13.43626322254348260, 155.6061939908119882, 1.534180175809178648 ) ) ;
#31165=CARTESIAN_POINT ( 'NONE',  ( 1.044861395163911411, 117.1967307433898640, -0.4172573962433456796 ) ) ;
#31166=CARTESIAN_POINT ( 'NONE',  ( 4.458631606973747274, 16.91056413504885825, 1.251853190366734259 ) ) ;
#31167=CARTESIAN_POINT ( 'NONE',  ( -23.02690842483890066, 149.8694456586574972, -0.9127416204503945307 ) ) ;
#31170=CARTESIAN_POINT ( 'NONE',  ( 8.789531458490529303, 117.7096508578360101, 0.3423636166664316693 ) ) ;
#31171=FACE_OUTER_BOUND ( 'NONE', #40723, .T. ) ;
#31172=CARTESIAN_POINT ( 'NONE',  ( -0.02768739821015298377, 156.9833357668885014, 1.385590625008459087 ) ) ;
#31174=CARTESIAN_POINT ( 'NONE',  ( 17.50667431346010972, 135.4862447717955547, -1.719380121689204177 ) ) ;
#31175=CARTESIAN_POINT ( 'NONE',  ( -13.87194369518297599, 121.7708260186165177, -1.632391212143505799 ) ) ;
#31177=CARTESIAN_POINT ( 'NONE',  ( 13.84625834149330359, 134.3516747369166069, -0.8047173373260269047 ) ) ;
#31178=EDGE_LOOP ( 'NONE', ( #11242, #14555, #10341, #27528 ) ) ;
#31179=CARTESIAN_POINT ( 'NONE',  ( -17.50950237657583131, 148.8653046532945723, -2.321071487785774767 ) ) ;
#31180=CARTESIAN_POINT ( 'NONE',  ( 3.954393197012034733, -15.56809308616131915, 2.853032214330836869 ) ) ;
#31181=CARTESIAN_POINT ( 'NONE',  ( -4.448382910831185200, 118.1283983457245625, -0.7237973005349965794 ) ) ;
#31183=CARTESIAN_POINT ( 'NONE',  ( -4.828569062062975092, 117.4060461567800786, 1.008118597039231235 ) ) ;
#31184=CARTESIAN_POINT ( 'NONE',  ( 7.383155613640851378, 155.9567503867590972, 1.861932028473976208 ) ) ;
#31186=CARTESIAN_POINT ( 'NONE',  ( -6.853500063829680577, -7.707324007402828414, -4.930749982112237362 ) ) ;
#31187=CARTESIAN_POINT ( 'NONE',  ( 12.24221062544593153, 130.6044139104978115, 0.7866602228194184976 ) ) ;
#31189=TOROIDAL_SURFACE ( 'NONE', #19636, 3.683000000000000718, 0.5080000000000000071 ) ;
#31191=ORIENTED_EDGE ( 'NONE', *, *, #12507, .T. ) ;
#31192=CARTESIAN_POINT ( 'NONE',  ( 0.3822965766165241086, 105.7854827256092420, -5.327377110122780479 ) ) ;
#31196=CARTESIAN_POINT ( 'NONE',  ( -6.908764576387383727, 117.1865127098105575, -0.01035743554829984120 ) ) ;
#31197=EDGE_LOOP ( 'NONE', ( #36682, #16606, #14353, #32687 ) ) ;
#31199=CARTESIAN_POINT ( 'NONE',  ( 5.943351980717774374, 121.3891827933073557, -0.07897414172417135947 ) ) ;
#31200=CARTESIAN_POINT ( 'NONE',  ( -8.511289907599598692, 119.1972314554215302, 1.000383355283217757 ) ) ;
#31202=CARTESIAN_POINT ( 'NONE',  ( 3.205182831369184804, 118.7629491485453741, -1.047990948762189456 ) ) ;
#31203=CARTESIAN_POINT ( 'NONE',  ( -4.265939155585104281, 155.8374496918941077, -0.3214930909109445234 ) ) ;
#31204=CARTESIAN_POINT ( 'NONE',  ( 5.472227756958008449, -13.43587746834383445, 2.852490916751204697 ) ) ;
#31205=CARTESIAN_POINT ( 'NONE',  ( -21.57210427006343423, 149.5883454796168621, 1.274511887596345039 ) ) ;
#31207=CARTESIAN_POINT ( 'NONE',  ( 23.20201897184725226, 149.6253602407241488, 0.6175280007103176594 ) ) ;
#31208=CARTESIAN_POINT ( 'NONE',  ( 4.218275339060157059, 155.8585684991085714, 0.08429118021179421438 ) ) ;
#31209=CARTESIAN_POINT ( 'NONE',  ( -4.988560382155355022, 117.5941865341327741, 0.6973410046930860196 ) ) ;
#31210=CARTESIAN_POINT ( 'NONE',  ( 0.6255416438669687551, 26.40915095058528905, 0.7518939258676016202 ) ) ;
#31211=CARTESIAN_POINT ( 'NONE',  ( -23.44243449907619237, 146.8400249081559537, -0.5456528120549730687 ) ) ;
#31215=CARTESIAN_POINT ( 'NONE',  ( 3.622559830352364507, 117.9414738143271109, 0.9055989021787060889 ) ) ;
#31217=CARTESIAN_POINT ( 'NONE',  ( 19.51124600060703784, 152.2820370773569323, 1.942483913431542364 ) ) ;
#31219=CARTESIAN_POINT ( 'NONE',  ( 0.4495176323322074285, 118.2558431149878402, -0.5768950177939177193 ) ) ;
#31220=CARTESIAN_POINT ( 'NONE',  ( 8.093748642744952093, 23.43776531741863423, -2.407353130276413733 ) ) ;
#31221=CARTESIAN_POINT ( 'NONE',  ( -22.07943683853339323, 148.3267584643486146, -2.032026126618132089 ) ) ;
#31222=CARTESIAN_POINT ( 'NONE',  ( 4.861667474615974704, 117.7348714202375248, -0.8247141752807952697 ) ) ;
#31223=CARTESIAN_POINT ( 'NONE',  ( 3.903247448917655849, 109.8183322527596602, 3.677532532511333052 ) ) ;
#31224=ORIENTED_EDGE ( 'NONE', *, *, #36551, .T. ) ;
#31225=CARTESIAN_POINT ( 'NONE',  ( -0.002459394113084579191, 156.3065584682211124, 0.1230781383047673677 ) ) ;
#31226=CARTESIAN_POINT ( 'NONE',  ( -12.62197313556529110, 122.7135068550949200, -1.834144044656287109 ) ) ;
#31228=CARTESIAN_POINT ( 'NONE',  ( 2.058067359092986326, -15.63668844659656187, 5.842422791592841946 ) ) ;
#31231=CARTESIAN_POINT ( 'NONE',  ( -3.153262279070554897, 117.9496044432466419, -1.302034589134676068 ) ) ;
#31232=ORIENTED_EDGE ( 'NONE', *, *, #6581, .T. ) ;
#31233=CARTESIAN_POINT ( 'NONE',  ( 2.358209769532786382, 119.0637060312156024, 0.7902384042126602282 ) ) ;
#31234=CARTESIAN_POINT ( 'NONE',  ( -5.332935381406168851, 115.7029491485442634, -0.1065653510733624160 ) ) ;
#31235=CARTESIAN_POINT ( 'NONE',  ( -4.834697789094183129, 118.7629491485453599, 0.4653049473571303496 ) ) ;
#31236=CARTESIAN_POINT ( 'NONE',  ( -1.603046668355913917, 118.6366899268033279, 0.8036507178775276206 ) ) ;
#31237=CARTESIAN_POINT ( 'NONE',  ( 7.363685156731384573, -6.572911479292511849, 4.144591825403105112 ) ) ;
#31238=CARTESIAN_POINT ( 'NONE',  ( 15.82363114525486836, 143.7482200480382346, 1.443160993194752217 ) ) ;
#31239=FACE_OUTER_BOUND ( 'NONE', #4367, .T. ) ;
#31240=CARTESIAN_POINT ( 'NONE',  ( 14.93494801707985609, 120.8072429308574414, -0.3831319127562621274 ) ) ;
#31248=CARTESIAN_POINT ( 'NONE',  ( -4.116494434418081383, 118.2429491485453354, 0.1883380258390151551 ) ) ;
#31253=CARTESIAN_POINT ( 'NONE',  ( -6.150511332855731261, 119.6465158254115835, -1.246810306309521943 ) ) ;
#31254=CARTESIAN_POINT ( 'NONE',  ( -5.336395407662996249, 116.0444662015457169, 0.06658830643601890142 ) ) ;
#31255=CARTESIAN_POINT ( 'NONE',  ( 4.364698422493899166, 118.1847547154890208, 0.6011634615692652561 ) ) ;
#31256=CARTESIAN_POINT ( 'NONE',  ( 0.004350076772674690319, 120.7058980590201429, -0.2176956299261763039 ) ) ;
#31258=CARTESIAN_POINT ( 'NONE',  ( 9.822473411059192472, 117.9943479623217399, 0.1962763949404991992 ) ) ;
#31259=EDGE_LOOP ( 'NONE', ( #9360, #2387, #11521, #33615, #40866, #134, #19421 ) ) ;
#31260=CARTESIAN_POINT ( 'NONE',  ( -0.01876340930523686876, 19.73428105357427853, -4.634220987317214657 ) ) ;
#31265=CARTESIAN_POINT ( 'NONE',  ( 6.989608668544338599, 121.8932936631570669, 0.4001562091357755979 ) ) ;
#31266=CARTESIAN_POINT ( 'NONE',  ( -3.618988008572157522, 19.14412854911201123, 2.900346660497036044 ) ) ;
#31267=CARTESIAN_POINT ( 'NONE',  ( 22.60558431049191697, 149.7032342875954498, 1.528355188309250545 ) ) ;
#31268=CARTESIAN_POINT ( 'NONE',  ( 4.780938538460484111, 104.6144662015456959, -0.7305874870394178933 ) ) ;
#31269=CARTESIAN_POINT ( 'NONE',  ( 1.824654213811243819, -15.25386490109567639, 5.420715704377902178 ) ) ;
#31270=CARTESIAN_POINT ( 'NONE',  ( 15.01775385910449145, 123.1914926142276130, -1.125269324988861896 ) ) ;
#31271=CARTESIAN_POINT ( 'NONE',  ( -18.38987645279124550, 147.6341482083243761, 1.661003423535650558 ) ) ;
#31272=CARTESIAN_POINT ( 'NONE',  ( -1.512449008193210931, 25.81601926892489018, -4.382106060783010903 ) ) ;
#31273=CARTESIAN_POINT ( 'NONE',  ( -16.56062761363025970, 155.2525159475892167, -1.104293791145709802 ) ) ;
#31274=CARTESIAN_POINT ( 'NONE',  ( 0.9735350199255810022, 12.44701472381428609, 0.02964292050307446719 ) ) ;
#31277=CARTESIAN_POINT ( 'NONE',  ( -4.393282770141167859, 155.8497297829079571, 0.4427821657071677741 ) ) ;
#31278=CARTESIAN_POINT ( 'NONE',  ( 5.341062828015524566, -12.45213391371734168, 1.712110018432928982 ) ) ;
#31279=CARTESIAN_POINT ( 'NONE',  ( 10.62684080304149603, 123.4307455932968765, -0.9978443992970126297 ) ) ;
#31281=CARTESIAN_POINT ( 'NONE',  ( 0.7313781531325286300, 115.7029491485453292, 1.756327035003194981 ) ) ;
#31283=CARTESIAN_POINT ( 'NONE',  ( -4.641629919619552957, 117.8847811183079841, -1.004318260171652266 ) ) ;
#31284=ADVANCED_FACE ( 'NONE', ( #2638, #15175 ), #22394, .F. ) ;
#31285=CARTESIAN_POINT ( 'NONE',  ( 8.074187567048884517, 122.8559727437779827, 0.08249527776860611505 ) ) ;
#31286=AXIS2_PLACEMENT_3D ( 'NONE', #18496, #15520, #34505 ) ;
#31288=CARTESIAN_POINT ( 'NONE',  ( 19.82367009662574375, 149.5711785761137662, 2.459487706365388604 ) ) ;
#31289=CARTESIAN_POINT ( 'NONE',  ( 1.561582345843624431, 156.2588034088681184, 0.03120413162939523685 ) ) ;
#31292=CARTESIAN_POINT ( 'NONE',  ( 23.25537431167556690, 149.3282167461061931, 0.1335628131362695814 ) ) ;
#31293=CARTESIAN_POINT ( 'NONE',  ( 0.03707542933077223601, 115.3931862868688398, -1.855406091731502505 ) ) ;
#31294=CARTESIAN_POINT ( 'NONE',  ( 1.989440554114935145, -15.14293609156945664, 5.899323384112847179 ) ) ;
#31297=CARTESIAN_POINT ( 'NONE',  ( -4.657380072211783073, 117.9834161660140381, 0.7123224875277872625 ) ) ;
#31299=ORIENTED_EDGE ( 'NONE', *, *, #14169, .T. ) ;
#31301=CARTESIAN_POINT ( 'NONE',  ( 5.174194766718689387, 115.7029491485453150, -1.071326111713503559 ) ) ;
#31302=CARTESIAN_POINT ( 'NONE',  ( 3.046135264910829754, 118.1726090481387814, -0.7595472998034786816 ) ) ;
#31303=CARTESIAN_POINT ( 'NONE',  ( -4.758673294993353231, 116.4582014290525507, -1.187054331573000665 ) ) ;
#31305=CARTESIAN_POINT ( 'NONE',  ( 4.796259625824248474, 117.7368196676605265, 1.049688617138287317 ) ) ;
#31307=CARTESIAN_POINT ( 'NONE',  ( -0.3929232564621699120, 123.1683257372383054, 0.1777898040562597426 ) ) ;
#31310=CARTESIAN_POINT ( 'NONE',  ( 3.682264917456191888, 101.6934662015457320, 0.07358041635423968885 ) ) ;
#31311=CARTESIAN_POINT ( 'NONE',  ( 3.325379330704291814, -12.45968715000887705, 0.9553361148970926919 ) ) ;
#31312=CARTESIAN_POINT ( 'NONE',  ( 6.118667329349966266, 121.4157903421748301, -0.08376844782033862624 ) ) ;
#31313=CARTESIAN_POINT ( 'NONE',  ( -17.50701641564917921, 146.6691408387931688, -2.165841098895500583 ) ) ;
#31318=CARTESIAN_POINT ( 'NONE',  ( 2.801506786573456420, 9.139157206818806500, -3.684590140147142368 ) ) ;
#31319=CARTESIAN_POINT ( 'NONE',  ( 14.58714721168222006, 120.3300541288867862, 0.7025926276034526463 ) ) ;
#31321=CARTESIAN_POINT ( 'NONE',  ( 2.186726956427079926, 104.6144662015457243, -4.302861239856920150 ) ) ;
#31322=CARTESIAN_POINT ( 'NONE',  ( 4.535010020878385895, -15.35856548043400238, 0.06517018677027014428 ) ) ;
#31323=CARTESIAN_POINT ( 'NONE',  ( -0.01147819631912393688, 118.8623374019222894, 0.5744158801423953076 ) ) ;
#31324=CARTESIAN_POINT ( 'NONE',  ( -0.4283232389533950801, 25.18001705023179326, -0.8778289364919926729 ) ) ;
#31325=CIRCLE ( 'NONE', #14988, 3.683000000000001162 ) ;
#31326=CARTESIAN_POINT ( 'NONE',  ( 0.4606059098249736805, 26.09511874640634943, 0.8667040019166204479 ) ) ;
#31329=FACE_BOUND ( 'NONE', #32265, .T. ) ;
#31330=CARTESIAN_POINT ( 'NONE',  ( 1.673685645604575445, 111.6436615656963909, 3.078281589618439895 ) ) ;
#31331=CARTESIAN_POINT ( 'NONE',  ( -9.903729432088850260, 123.6875948057429895, 0.6970279851166614193 ) ) ;
#31332=EDGE_CURVE ( 'NONE', #5382, #37727, #15111, .T. ) ;
#31334=CARTESIAN_POINT ( 'NONE',  ( 3.604966970014626959, -13.82400766246429136, 3.906450875976586801 ) ) ;
#31335=CARTESIAN_POINT ( 'NONE',  ( 14.02613073054668824, 152.5802402909829425, -1.631301951249304993 ) ) ;
#31336=CARTESIAN_POINT ( 'NONE',  ( -5.840405771877655638, 118.8996324090661147, -1.179527747254400349 ) ) ;
#31339=CARTESIAN_POINT ( 'NONE',  ( -15.21351360038804579, 143.4186079242267340, -0.3040022078858841126 ) ) ;
#31340=CARTESIAN_POINT ( 'NONE',  ( 4.074910602682932925, 118.2429491485453354, -0.1454311599470142491 ) ) ;
#31341=CARTESIAN_POINT ( 'NONE',  ( 15.88665273169769598, 145.7686330500600036, -0.2792794258574998745 ) ) ;
#31343=CARTESIAN_POINT ( 'NONE',  ( 2.915559332840946816, -14.19431184016030301, 0.3483797586856177686 ) ) ;
#31344=CARTESIAN_POINT ( 'NONE',  ( -5.994056581265662363E-14, 72.48346620154573827, 9.856484473772818746E-17 ) ) ;
#31350=CARTESIAN_POINT ( 'NONE',  ( -3.942997264624582776, -11.51663297089948479, -2.426127359622226809 ) ) ;
#31351=CARTESIAN_POINT ( 'NONE',  ( 0.5640265924886082027, 120.2131932824006526, 0.4111470527632634098 ) ) ;
#31352=CARTESIAN_POINT ( 'NONE',  ( -3.640095369667306180, 28.17176065243310390, 0.7113786998093643010 ) ) ;
#31353=CARTESIAN_POINT ( 'NONE',  ( -0.1065646865916160396, 105.8844662015456777, 5.332932678536313809 ) ) ;
#31354=CARTESIAN_POINT ( 'NONE',  ( 4.224370802630715183, -2.505441902618962935, 1.893578447770203566 ) ) ;
#31355=CARTESIAN_POINT ( 'NONE',  ( 10.39928917620358817, 153.1223395828141918, 0.2078025466733119664 ) ) ;
#31356=ADVANCED_FACE ( 'NONE', ( #15598 ), #20551, .T. ) ;
#31357=CARTESIAN_POINT ( 'NONE',  ( -6.277010209292351206, 0.1250379130781943404, 5.629075605414042727 ) ) ;
#31359=CARTESIAN_POINT ( 'NONE',  ( 8.786181581555666753, 117.7732179722915618, -0.1423289417060864537 ) ) ;
#31360=CARTESIAN_POINT ( 'NONE',  ( -0.9836305199215028550, 123.5966405200008325, -0.1412250206608574310 ) ) ;
#31362=DIRECTION ( 'NONE',  ( -0.9998004120163609398, 0.000000000000000000, -0.01997839162482749689 ) ) ;
#31363=CARTESIAN_POINT ( 'NONE',  ( -8.412600736458745843, -6.831223903669816799, -0.4304377746521336201 ) ) ;
#31364=CARTESIAN_POINT ( 'NONE',  ( 3.960059183279624140, 117.9394489435469211, 1.233284679773928971 ) ) ;
#31366=DIRECTION ( 'NONE',  ( 0.9998004120163608288, 0.000000000000000000, 0.01997839162482749342 ) ) ;
#31367=CARTESIAN_POINT ( 'NONE',  ( 0.7689147969092013923, 119.5055576915191580, -0.7020325503247994980 ) ) ;
#31368=CARTESIAN_POINT ( 'NONE',  ( -23.19190728264284829, 146.6831645211815101, 0.2733909575703943884 ) ) ;
#31374=CARTESIAN_POINT ( 'NONE',  ( -15.77133435453296606, 146.5691041611200660, -0.3151487940933135334 ) ) ;
#31375=CARTESIAN_POINT ( 'NONE',  ( 5.567940837815767097, -14.86657585147074734, 2.969021103613282531 ) ) ;
#31376=CARTESIAN_POINT ( 'NONE',  ( -16.52101850268839200, 153.5550899668227203, 1.581448849539220269 ) ) ;
#31377=CARTESIAN_POINT ( 'NONE',  ( 15.08259856265889809, 121.6710330000183546, -0.7362983101480767845 ) ) ;
#31378=CARTESIAN_POINT ( 'NONE',  ( -4.492784857928645792, 12.16275517495587977, -1.104450737933446725 ) ) ;
#31379=CARTESIAN_POINT ( 'NONE',  ( -23.20196384716143001, 149.3105122542552863, -0.9177021184322480263 ) ) ;
#31384=CARTESIAN_POINT ( 'NONE',  ( -8.798408483647307321, 117.6899343870790631, -0.1004539260620418706 ) ) ;
#31386=CARTESIAN_POINT ( 'NONE',  ( -0.5497817020643304131, 119.7690751942239729, 0.4902208388216632851 ) ) ;
#31388=CARTESIAN_POINT ( 'NONE',  ( 15.01676740740983007, 152.9649416503947634, -1.747251348416147820 ) ) ;
#31389=CARTESIAN_POINT ( 'NONE',  ( -10.54454712121203741, 119.9085704333771787, -1.450830856784145917 ) ) ;
#31391=CARTESIAN_POINT ( 'NONE',  ( 5.210205730215608178, 121.0352659167314755, -0.3424523703800271823 ) ) ;
#31392=VERTEX_POINT ( 'NONE', #2845 ) ;
#31393=CARTESIAN_POINT ( 'NONE',  ( -17.91131452944958014, 148.1388135707062474, -2.335088068787735782 ) ) ;
#31394=CARTESIAN_POINT ( 'NONE',  ( 1.897852064921616622, -15.54654116324019597, 5.408738352340563438 ) ) ;
#31396=CARTESIAN_POINT ( 'NONE',  ( 4.825036788390894671, 51.14746620154573264, 0.09641571798141809757 ) ) ;
#31397=AXIS2_PLACEMENT_3D ( 'NONE', #11556, #24540, #8371 ) ;
#31400=ADVANCED_FACE ( 'NONE', ( #22809 ), #13466, .T. ) ;
#31401=CARTESIAN_POINT ( 'NONE',  ( -4.815275531776046947, 117.4047736241515736, 1.012442419610674271 ) ) ;
#31402=CARTESIAN_POINT ( 'NONE',  ( 17.60198365394328590, 148.3509993576462307, 2.281626375285575659 ) ) ;
#31403=CARTESIAN_POINT ( 'NONE',  ( -5.586884702347497900, 136.3644662015457527, -0.1116392523995361485 ) ) ;
#31405=CARTESIAN_POINT ( 'NONE',  ( -3.848622047617309860, 1.169161361801722032, -7.524129562738414378 ) ) ;
#31406=CARTESIAN_POINT ( 'NONE',  ( 9.155891339183860111, 123.9989874199980022, 0.4132670667758964744 ) ) ;
#31407=CARTESIAN_POINT ( 'NONE',  ( 1.949857553418792744, 118.1238931878471448, -0.8604232605442251325 ) ) ;
#31409=CARTESIAN_POINT ( 'NONE',  ( -1.138279655186107187, 117.9394518318250107, 1.346695663613399097 ) ) ;
#31412=CARTESIAN_POINT ( 'NONE',  ( -6.615214180512292604E-14, 94.32746620154571815, -2.829521569843129660E-18 ) ) ;
#31414=CARTESIAN_POINT ( 'NONE',  ( -21.55438672983833825, 132.6250929350426020, -0.2276674992303580614 ) ) ;
#31417=CARTESIAN_POINT ( 'NONE',  ( -6.029124040440666299, 121.4385140814827651, -0.1554332074001965880 ) ) ;
#31420=CARTESIAN_POINT ( 'NONE',  ( 2.215630398121276823, 118.7629491485453883, -1.137602048208893768 ) ) ;
#31421=CARTESIAN_POINT ( 'NONE',  ( -6.012785076883673696, 155.3544091381320982, -0.3765917842305991914 ) ) ;
#31422=CARTESIAN_POINT ( 'NONE',  ( 4.441035242322985965, -14.03446645907663282, 4.353459135924754086 ) ) ;
#31423=CARTESIAN_POINT ( 'NONE',  ( -20.51279501983856690, 150.9797539340098069, 1.282250019969888077 ) ) ;
#31426=CARTESIAN_POINT ( 'NONE',  ( 21.59686147024584102, 132.6646020023713959, 0.5653344646799389750 ) ) ;
#31427=CARTESIAN_POINT ( 'NONE',  ( 15.72253002844083447, 146.8976288395060124, 0.3811693606321951422 ) ) ;
#31429=CARTESIAN_POINT ( 'NONE',  ( -0.4102451260098727293, 24.68626973166569982, 0.8857237506759965129 ) ) ;
#31430=CARTESIAN_POINT ( 'NONE',  ( -13.67522198567664482, 119.6429072192227494, -0.3220992662749118107 ) ) ;
#31432=DIRECTION ( 'NONE',  ( 0.9998004120163608288, 0.000000000000000000, 0.01997839162482736852 ) ) ;
#31433=ORIENTED_EDGE ( 'NONE', *, *, #34997, .T. ) ;
#31434=CARTESIAN_POINT ( 'NONE',  ( -4.022005995279760882, 118.2573117515256911, 0.8180388012835972944 ) ) ;
#31435=DIRECTION ( 'NONE',  ( 4.017660918040594346E-17, -1.000000000000000000, -2.376309959284834438E-19 ) ) ;
#31436=CARTESIAN_POINT ( 'NONE',  ( 16.77501307560209654, 125.2521365416322254, 1.703383479906432685 ) ) ;
#31437=CARTESIAN_POINT ( 'NONE',  ( 2.242939865367092001, 118.2767885243204944, -0.6835633642702234614 ) ) ;
#31438=CARTESIAN_POINT ( 'NONE',  ( -7.074087999897446188, 26.91573472731666783, -4.615267515785972385 ) ) ;
#31439=CARTESIAN_POINT ( 'NONE',  ( -22.29769713523688779, 148.9358926463403918, -1.890714429241201699 ) ) ;
#31440=CARTESIAN_POINT ( 'NONE',  ( 4.866058426851059160, 117.6757764595213018, -0.8743054753177306182 ) ) ;
#31441=CARTESIAN_POINT ( 'NONE',  ( 5.028795574735070772, 114.3519703858145959, 1.961426316196308361 ) ) ;
#31442=CARTESIAN_POINT ( 'NONE',  ( -14.69813734295233232, 148.8396455022467535, -0.06702550439777849034 ) ) ;
#31443=CARTESIAN_POINT ( 'NONE',  ( -16.83022555070514770, 151.2926467857828072, -2.419188160499602613 ) ) ;
#31445=CARTESIAN_POINT ( 'NONE',  ( 4.355571528211143573, -15.30747929803376373, 4.711715777764150737 ) ) ;
#31446=CARTESIAN_POINT ( 'NONE',  ( -6.571239715384261478E-14, 88.48546620154573361, -1.207165459146770882E-19 ) ) ;
#31447=CARTESIAN_POINT ( 'NONE',  ( -1.551677701541317234, 118.1651005044952285, -0.8611336031554802650 ) ) ;
#31448=ORIENTED_EDGE ( 'NONE', *, *, #10721, .F. ) ;
#31449=CARTESIAN_POINT ( 'NONE',  ( 5.029336563146884487, 119.5555251685854330, 1.067692183578045073 ) ) ;
#31453=CARTESIAN_POINT ( 'NONE',  ( -2.219425127536600151, 123.7320667226965867, 0.04105829392232424740 ) ) ;
#31454=CARTESIAN_POINT ( 'NONE',  ( -7.958381229837070414, -11.09356959825496247, -2.748999415197344476 ) ) ;
#31455=CARTESIAN_POINT ( 'NONE',  ( 6.199776539618373938, 155.3658059236344684, 0.8002054381730366872 ) ) ;
#31457=CARTESIAN_POINT ( 'NONE',  ( 1.382728874883415449, 159.5452856091935132, -0.4834108180186508230 ) ) ;
#31461=CARTESIAN_POINT ( 'NONE',  ( -6.571239715384261478E-14, 88.48546620154573361, -1.207165459146770882E-19 ) ) ;
#31462=CARTESIAN_POINT ( 'NONE',  ( -4.119378102468195912, 118.2429491485453354, 0.1851105702619638971 ) ) ;
#31464=CARTESIAN_POINT ( 'NONE',  ( 5.219047500496350800, 114.8007926982748614, -1.212193980527778603 ) ) ;
#31467=CARTESIAN_POINT ( 'NONE',  ( 8.274444664989344389, 120.3629719553960769, -1.109322312946052103 ) ) ;
#31468=CARTESIAN_POINT ( 'NONE',  ( 4.304052292061569140, 104.6144662015457385, -3.992357259174772466 ) ) ;
#31469=CARTESIAN_POINT ( 'NONE',  ( -2.729962743039006323, 120.7841308545065431, -0.3244322735474264308 ) ) ;
#31470=CARTESIAN_POINT ( 'NONE',  ( -5.586884702347496123, 87.97746620154572383, -0.1116392523995361624 ) ) ;
#31473=CARTESIAN_POINT ( 'NONE',  ( 4.203610184846851894, 17.99761390031315500, -1.968029828111186319 ) ) ;
#31477=DIRECTION ( 'NONE',  ( -4.017660918040594346E-17, 1.000000000000000000, 2.376309959284834438E-19 ) ) ;
#31478=CARTESIAN_POINT ( 'NONE',  ( -6.991984101104667282, 121.9387022086022654, -0.02476450050892398808 ) ) ;
#31479=CARTESIAN_POINT ( 'NONE',  ( 2.233585966345281282, 24.54162662436292308, -4.064490141941544898 ) ) ;
#31480=CARTESIAN_POINT ( 'NONE',  ( 3.857972943339615046, 117.0975898859979054, 0.5726864223607190940 ) ) ;
#31481=CARTESIAN_POINT ( 'NONE',  ( -1.939077340875614341, 104.6144662015454543, -4.428395887593343794 ) ) ;
#31482=CARTESIAN_POINT ( 'NONE',  ( 2.349528287245666647, -15.15257587461875310, 4.947206973663434759 ) ) ;
#31483=CARTESIAN_POINT ( 'NONE',  ( 21.30706188252186450, 149.4807732621110006, -1.383641861344254931 ) ) ;
#31484=CARTESIAN_POINT ( 'NONE',  ( -6.628409759327085204, 120.2999964176511014, 0.9194780514890086298 ) ) ;
#31485=CARTESIAN_POINT ( 'NONE',  ( 0.7724745873405186591, -15.29971413243098688, -0.5873327843062005060 ) ) ;
#31486=CARTESIAN_POINT ( 'NONE',  ( 0.005915287708642085092, 116.9295063353193882, -0.2960251855814708399 ) ) ;
#31488=CARTESIAN_POINT ( 'NONE',  ( -0.6899137464274212039, -3.097154947502566813, -0.6881565663087282347 ) ) ;
#31489=ORIENTED_EDGE ( 'NONE', *, *, #39691, .T. ) ;
#31491=CARTESIAN_POINT ( 'NONE',  ( -14.45325548908966695, 139.0941462050048187, 0.3122831254358890418 ) ) ;
#31492=CARTESIAN_POINT ( 'NONE',  ( 5.397943591185104140, -12.01093657298729589, 0.9516947191793155847 ) ) ;
#31493=CARTESIAN_POINT ( 'NONE',  ( 8.784047514290564962, 154.8283212766472445, -1.235621501372049513 ) ) ;
#31494=ORIENTED_EDGE ( 'NONE', *, *, #20898, .F. ) ;
#31495=CARTESIAN_POINT ( 'NONE',  ( 1.801784832236646094, 115.7029148924688116, 1.722822550453829482 ) ) ;
#31496=CARTESIAN_POINT ( 'NONE',  ( -4.726758526000762295, 117.7280786527958156, -1.096802179199823035 ) ) ;
#31497=CARTESIAN_POINT ( 'NONE',  ( 5.966562942537897207, 155.3820107761045790, 0.07923228615413213660 ) ) ;
#31498=ORIENTED_EDGE ( 'NONE', *, *, #24127, .F. ) ;
#31499=CARTESIAN_POINT ( 'NONE',  ( 11.23789960528888443, 121.3367100885591015, 1.694033198309416122 ) ) ;
#31500=CARTESIAN_POINT ( 'NONE',  ( 3.174366308151881366, 84.67546620154573134, 0.06343139340882768262 ) ) ;
#31504=CARTESIAN_POINT ( 'NONE',  ( 3.772649051594905156, 116.7207137014398626, -0.1335598970234344318 ) ) ;
#31505=FACE_OUTER_BOUND ( 'NONE', #19274, .T. ) ;
#31506=CIRCLE ( 'NONE', #36975, 5.080000000000006288 ) ;
#31508=CARTESIAN_POINT ( 'NONE',  ( 1.969151417587075681, -15.07365727821173529, 5.800531510698589521 ) ) ;
#31512=CARTESIAN_POINT ( 'NONE',  ( -4.807805788012706749, 117.8776837157520561, 0.6743155973055370289 ) ) ;
#31516=CARTESIAN_POINT ( 'NONE',  ( -5.564994385194649062, 118.1214215447172080, -1.127427256207502948 ) ) ;
#31517=B_SPLINE_CURVE_WITH_KNOTS ( 'NONE', 3,
 ( #16893, #16681, #39493, #20080, #13709, #36505, #23268, #32464, #6693, #36091 ),
 .UNSPECIFIED., .F., .F.,
 ( 4, 2, 2, 2, 4 ),
 ( -5.999999999944513512E-08, 0.0006000059959409705622, 0.001200071991881940551, 0.002400203983763880312, 0.004800467967527762003 ),
 .UNSPECIFIED. ) ;
#31518=CARTESIAN_POINT ( 'NONE',  ( -4.275575466068185726, 118.7880935209305591, -0.6699701396488103589 ) ) ;
#31519=CARTESIAN_POINT ( 'NONE',  ( 4.772772660974615277, 117.5405024988783396, 1.172286739505868702 ) ) ;
#31521=CARTESIAN_POINT ( 'NONE',  ( -0.2185697341917780256, 107.6766875080336376, 4.612355970162428598 ) ) ;
#31523=CARTESIAN_POINT ( 'NONE',  ( 2.522041008973656240, -3.380034811851383214, 3.874746376371965617 ) ) ;
#31526=CARTESIAN_POINT ( 'NONE',  ( 2.973740295910565212, -14.46567735677360744, 4.831635400698222504 ) ) ;
#31527=CARTESIAN_POINT ( 'NONE',  ( 7.618479139564603209, 124.7215218652630710, 0.1522353441811858110 ) ) ;
#31528=CARTESIAN_POINT ( 'NONE',  ( -8.045112435069388113, 121.5393406094847819, -1.176871282714906153 ) ) ;
#31531=CARTESIAN_POINT ( 'NONE',  ( -0.8204882251181495612, 115.7029491485453292, 1.724334212604217820 ) ) ;
#31532=CARTESIAN_POINT ( 'NONE',  ( -2.923568588381722844, 13.88697512809157786, 3.594856661414283394 ) ) ;
#31533=CARTESIAN_POINT ( 'NONE',  ( 3.798364743159144741, 116.8316721669309572, 0.3950458664356922833 ) ) ;
#31534=EDGE_LOOP ( 'NONE', ( #31918, #31494, #22117, #23043 ) ) ;
#31535=CARTESIAN_POINT ( 'NONE',  ( 4.653077788127276904, 104.6144662015412905, -2.613629344544315281 ) ) ;
#31536=CARTESIAN_POINT ( 'NONE',  ( 3.946041497568072653, -15.66665589675640646, 3.498282510246776500 ) ) ;
#31537=CARTESIAN_POINT ( 'NONE',  ( -12.16919611748930308, 122.5392882283422864, 1.309229788656695037 ) ) ;
#31538=CARTESIAN_POINT ( 'NONE',  ( -0.9274737138984842089, 27.34353985424608524, 0.2860612317039745167 ) ) ;
#31539=CARTESIAN_POINT ( 'NONE',  ( -0.8918910426314872186, 22.31184809748591391, -0.3959014520797728975 ) ) ;
#31540=ORIENTED_EDGE ( 'NONE', *, *, #11028, .F. ) ;
#31541=ORIENTED_EDGE ( 'NONE', *, *, #25110, .F. ) ;
#31543=CARTESIAN_POINT ( 'NONE',  ( 4.398525312957987765, 119.2572634999566930, 0.5937511404893220934 ) ) ;
#31544=CARTESIAN_POINT ( 'NONE',  ( -16.07945855365744592, 143.8376908863262997, 0.9680047772055858646 ) ) ;
#31546=CARTESIAN_POINT ( 'NONE',  ( 2.454477138217164178, -14.79624793513299785, 5.258896552041426808 ) ) ;
#31547=CARTESIAN_POINT ( 'NONE',  ( 7.451643811072074186, 155.9567503867590972, -1.565497431107723880 ) ) ;
#31549=CARTESIAN_POINT ( 'NONE',  ( -20.37866581877395689, 147.6366098820875266, -2.483541293540720396 ) ) ;
#31552=CARTESIAN_POINT ( 'NONE',  ( -14.16569067496518564, 138.8670163227233161, -0.2830642121559646673 ) ) ;
#31553=CARTESIAN_POINT ( 'NONE',  ( -6.530520361951679398, 29.76765211936704247, -0.1582873856006195845 ) ) ;
#31554=CARTESIAN_POINT ( 'NONE',  ( 15.41453346427784155, 143.5427300040290106, -0.2938895485367987725 ) ) ;
#31555=AXIS2_PLACEMENT_3D ( 'NONE', #25648, #39494, #28848 ) ;
#31556=ORIENTED_EDGE ( 'NONE', *, *, #6503, .T. ) ;
#31563=CARTESIAN_POINT ( 'NONE',  ( 2.357476308904321360, 24.96372521773390929, -8.086248583043326832 ) ) ;
#31564=CARTESIAN_POINT ( 'NONE',  ( 16.15947664645532100, 148.3349945484709451, 1.756847814979443756 ) ) ;
#31565=CARTESIAN_POINT ( 'NONE',  ( -2.958531772299361151, 39.20946620154573736, -1.329372033065077119 ) ) ;
#31566=CARTESIAN_POINT ( 'NONE',  ( 8.075779052176489614, 158.6620026115301698, 0.1430648235678990965 ) ) ;
#31567=CARTESIAN_POINT ( 'NONE',  ( -7.669306984062492560, 124.7206709383052043, -0.1533317827557519053 ) ) ;
#31569=AXIS2_PLACEMENT_3D ( 'NONE', #22512, #9141, #2959 ) ;
#31570=CARTESIAN_POINT ( 'NONE',  ( -0.8823465807374654135, 5.041073445128725794, 4.537322665494407659 ) ) ;
#31571=CARTESIAN_POINT ( 'NONE',  ( 5.945776936743700780, 121.5465042053001667, 0.1188107733588234238 ) ) ;
#31573=CARTESIAN_POINT ( 'NONE',  ( -0.3690887223898375868, -3.321408231106627973, -8.411989387140767604 ) ) ;
#31575=CARTESIAN_POINT ( 'NONE',  ( 5.518167891550173287, 117.1006821660659227, -0.5215187594908856639 ) ) ;
#31576=CARTESIAN_POINT ( 'NONE',  ( -0.8775954529457390407, 122.2453746293775652, -0.2818696459738748716 ) ) ;
#31579=CARTESIAN_POINT ( 'NONE',  ( -3.164706401634815869, 50.63946620154572997, -1.543954388298182101 ) ) ;
#31580=CARTESIAN_POINT ( 'NONE',  ( -4.507778648822867495, 31.37953541088120346, -1.025544427737863362 ) ) ;
#31581=CARTESIAN_POINT ( 'NONE',  ( 0.9908229604283667058, 117.3993836601774490, 1.479714518555806491 ) ) ;
#31584=EDGE_CURVE ( 'NONE', #4990, #1598, #23883, .T. ) ;
#31585=CARTESIAN_POINT ( 'NONE',  ( 0.8427018527670834258, 121.5536190086353372, -0.3367535922268982129 ) ) ;
#31586=CARTESIAN_POINT ( 'NONE',  ( -1.399407963385900899, 159.5796833544862352, 0.3162364300534757922 ) ) ;
#31592=CARTESIAN_POINT ( 'NONE',  ( -11.75644783568344209, 130.2587663741292658, -0.1212624266273917006 ) ) ;
#31593=CARTESIAN_POINT ( 'NONE',  ( 2.058067359092986326, -15.63668844659656187, 5.842422791592841946 ) ) ;
#31594=CARTESIAN_POINT ( 'NONE',  ( -5.883429839103577308, 118.5625182843610617, 0.8957466683066146462 ) ) ;
#31596=CARTESIAN_POINT ( 'NONE',  ( 22.10195095183540204, 148.8299554149626260, -1.146864445019731171 ) ) ;
#31597=CARTESIAN_POINT ( 'NONE',  ( 1.141857472271699425, 24.90688314728939190, 4.478778191171412182 ) ) ;
#31598=CARTESIAN_POINT ( 'NONE',  ( -15.47334368943532290, 120.8153160915142337, -0.6283931236857891456 ) ) ;
#31600=EDGE_LOOP ( 'NONE', ( #12465, #22042, #25127, #10961, #18958, #34034, #39309, #21678, #39455, #26837 ) ) ;
#31601=CARTESIAN_POINT ( 'NONE',  ( 0.3702369378893882734, 122.2435587914033022, 0.3018087652966767731 ) ) ;
#31603=CARTESIAN_POINT ( 'NONE',  ( -1.430496892223491079, 119.9358631726476574, 0.4886406555826711684 ) ) ;
#31605=CARTESIAN_POINT ( 'NONE',  ( 17.18700207657765944, 151.3967157021085654, -1.745027292404997432 ) ) ;
#31606=CARTESIAN_POINT ( 'NONE',  ( -9.094277710717381780, 119.2843051134756536, -1.347562189204172034 ) ) ;
#31608=CARTESIAN_POINT ( 'NONE',  ( 7.125763582822450815, 121.8059686962219672, -0.4001172506815711127 ) ) ;
#31610=CARTESIAN_POINT ( 'NONE',  ( -18.07470265256061381, 147.5382818419693649, -2.342107984669389520 ) ) ;
#31611=CARTESIAN_POINT ( 'NONE',  ( 4.393930847168488363, -15.54918382657802312, 2.099248807845041309 ) ) ;
#31612=CARTESIAN_POINT ( 'NONE',  ( -4.065972646788793554, 118.2429491485453070, -0.3080848862740693250 ) ) ;
#31614=CARTESIAN_POINT ( 'NONE',  ( -4.897933694818515704, 117.4787572636957265, 0.9608329789684921796 ) ) ;
#31615=CARTESIAN_POINT ( 'NONE',  ( 11.27861017918422526, 123.5700555580090594, 1.596916299002706818 ) ) ;
#31617=CARTESIAN_POINT ( 'NONE',  ( -2.691543149356179665, 0.9405793051805824145, -7.980626778548312927 ) ) ;
#31618=CARTESIAN_POINT ( 'NONE',  ( 10.44459398727714472, 153.0728660266736370, 0.5066767128784235297 ) ) ;
#31623=EDGE_CURVE ( 'NONE', #20434, #3752, #9016, .T. ) ;
#31624=CARTESIAN_POINT ( 'NONE',  ( -0.8481206146765604137, 117.9394518213541403, 1.367598340852225425 ) ) ;
#31626=CARTESIAN_POINT ( 'NONE',  ( -7.976708347975113078, 121.5957277616080745, -1.139915918955932694 ) ) ;
#31629=CARTESIAN_POINT ( 'NONE',  ( -22.65077213736933004, 150.6401102206664291, -0.2239908233986876995 ) ) ;
#31632=CARTESIAN_POINT ( 'NONE',  ( 7.810646221566016401, 122.5288342873456031, -0.1253198868880078809 ) ) ;
#31635=CARTESIAN_POINT ( 'NONE',  ( 0.8204245609312718068, 115.7029491485453718, -1.724338730900728534 ) ) ;
#31636=CARTESIAN_POINT ( 'NONE',  ( -15.73024628025059712, 145.6958675726371553, -0.4429222902984590871 ) ) ;
#31637=CARTESIAN_POINT ( 'NONE',  ( 4.992311776856191763, -13.37494578157311054, 3.269494339340476952 ) ) ;
#31638=CARTESIAN_POINT ( 'NONE',  ( -15.35657197080329084, 154.8698957928756954, 1.403577372161787906 ) ) ;
#31640=CARTESIAN_POINT ( 'NONE',  ( 23.29193865421784793, 149.0397177335360652, 0.7969840597304524987 ) ) ;
#31641=EDGE_CURVE ( 'NONE', #37473, #40423, #13883, .T. ) ;
#31642=CARTESIAN_POINT ( 'NONE',  ( 15.26080815366967869, 148.0236959631692173, 0.4380210713017328450 ) ) ;
#31644=CARTESIAN_POINT ( 'NONE',  ( -0.1409938471676187022, 25.13008524939761656, 0.9676832235670267401 ) ) ;
#31645=CARTESIAN_POINT ( 'NONE',  ( -2.754305024641401367, 116.5489981622532127, -0.1298538421819643296 ) ) ;
#31649=( GEOMETRIC_REPRESENTATION_CONTEXT ( 3 ) GLOBAL_UNCERTAINTY_ASSIGNED_CONTEXT ( ( #29104 ) ) GLOBAL_UNIT_ASSIGNED_CONTEXT ( ( #24013, #14423, #1465 ) ) REPRESENTATION_CONTEXT ( 'NONE', 'WORKASPACE' ) );
#31650=CARTESIAN_POINT ( 'NONE',  ( 5.999509053885005549, 118.7663675842279787, 1.217167017065042822 ) ) ;
#31651=CARTESIAN_POINT ( 'NONE',  ( 2.362155674307470310, -13.89060443905824194, -3.983575812745123290 ) ) ;
#31652=CARTESIAN_POINT ( 'NONE',  ( 12.43770564682699842, 156.7420262770442037, 1.659670365993107355 ) ) ;
#31653=CARTESIAN_POINT ( 'NONE',  ( 19.16692462419648280, 150.4642993720107143, -1.670612363451736027 ) ) ;
#31654=CARTESIAN_POINT ( 'NONE',  ( 8.378134419073882455, 22.78949214230337006, 1.148743996083190888 ) ) ;
#31655=EDGE_CURVE ( 'NONE', #28135, #1100, #7607, .T. ) ;
#31656=CARTESIAN_POINT ( 'NONE',  ( 0.01887972822138463125, 159.3676309965788960, -0.9448188026860500077 ) ) ;
#31657=CARTESIAN_POINT ( 'NONE',  ( 4.858182150843307845, 117.6759154865132899, -0.8826695618964555123 ) ) ;
#31658=CARTESIAN_POINT ( 'NONE',  ( 7.669269000495035904, 124.9344662015457317, 0.1532502464757268257 ) ) ;
#31659=CARTESIAN_POINT ( 'NONE',  ( -5.933842156842998428, 121.5392726388429168, -0.04747900449317086352 ) ) ;
#31660=CARTESIAN_POINT ( 'NONE',  ( -19.21961548592749836, 147.3692480224366079, -2.508364867928685626 ) ) ;
#31661=CARTESIAN_POINT ( 'NONE',  ( 2.825551972395176303, -15.60239892947398666, 5.624417742107700846 ) ) ;
#31663=CARTESIAN_POINT ( 'NONE',  ( -4.379091697861483112, 117.3993836135479967, -1.268018312266817160 ) ) ;
#31664=EDGE_LOOP ( 'NONE', ( #7230, #18972, #35372, #16268 ) ) ;
#31665=B_SPLINE_SURFACE_WITH_KNOTS ( 'NONE', 3, 3, ( 
 ( #8900, #18679, #40865, #34471, #27444, #5304, #21442, #14435, #18253, #40460, #31258, #8268, #34269, #5097, #28064, #41074, #11883, #8691, #18049, #31051, #1890, #172, #9941, #2736, #13142, #38713, #41498, #6136, #19725, #31899, #12926, #9735, #12718, #28903, #38925, #16325, #22492, #16108, #41918, #19100, #9116, #15902, #9320, #32315, #26134, #2939, #35733 ),
 ( #6544, #25708, #22912, #12304, #32108, #9524, #29329, #35519, #22703, #19519, #6340, #5929, #32527, #29112, #19311, #18891, #25504, #41706, #39135, #3358, #3145, #42130, #22282, #35945, #6757, #2529, #15692, #15491, #28489, #12513, #38504, #25917, #25292, #28698, #38296, #22078, #35105, #35308, #3578, #385, #26557, #20353, #6975, #20151, #26772, #33174, #30172 ),
 ( #29551, #26341, #29959, #39991, #23122, #23977, #39347, #800, #10151, #36159, #23763, #1013, #19946, #36376, #36786, #7816, #7604, #36995, #13567, #20564, #16541, #13775, #32746, #33593, #30374, #4426, #32966, #4002, #39782, #13351, #36576, #10997, #17384, #7392, #10783, #39564, #1223, #3791, #16751, #10576, #14183, #29756, #595, #10368, #23555, #23339, #7193 ),
 ( #16960, #33377, #27186, #4210, #40200, #17173, #13977, #26981, #33802, #18001, #12041, #8216, #1841, #30589, #8434, #27598, #25031, #14593, #8016, #1428, #14387, #18206, #31426, #38034, #2050, #41024, #17585, #11833, #27394, #31207, #40405, #8641, #21603, #1639, #40608, #11199, #11407, #4630, #11616, #34631, #24394, #24185, #4838, #27807, #15015, #15231, #24820 ),
 ( #28231, #37195, #30999, #24602, #20987, #37399, #34008, #28015, #17792, #30789, #21190, #14805, #2268, #41237, #20778, #37815, #5458, #34217, #40815, #5046, #18418, #37608, #21392, #34419, #5252, #22443, #6090, #2897, #29067, #15647, #38462, #38876, #15859, #12676, #5884, #25665, #16277, #38253, #12881, #2481, #19053, #25249, #31851, #28865, #32274, #26083, #18846 ),
 ( #9688, #9070, #15442, #32058, #28446, #41451, #42087, #19267, #12256, #12472, #25870, #8854, #22655, #13091, #2690, #35688, #21818, #41877, #126, #9280, #38672, #18636, #9479, #28652, #34845, #41664, #22035, #31640, #35063, #6296, #19475, #5678, #3104, #6497, #25466, #32482, #22238, #16065, #35266, #3311, #29281, #35472, #19896, #32697, #29705, #9892, #29915 ),
 ( #3532, #23078, #3953, #7345, #33545, #17124, #33331, #33124, #4377, #6712, #7143, #754, #19681, #546, #16492, #4161, #39299, #26291, #29498, #20100, #7556, #17335, #20516, #13933, #26928, #6926, #16915, #22865, #39941, #10733, #338, #26723, #13304, #10529, #36326, #13729, #30125, #3742, #26509, #23715, #39731, #23499, #36112, #36526, #30326, #10107, #964 ),
 ( #1170, #36733, #32912, #39090, #14134, #16700, #13521, #23289, #35902, #39514, #10320, #20305, #10942, #31319, #40149, #36947, #21503, #15337, #1379, #15122, #21715, #28125, #25145, #21930, #2377, #5988, #18317, #8544, #27347, #40360, #5570, #34536, #24716, #37930, #11941, #34959, #41560, #18528, #41351, #24932, #2163, #33755, #41135, #5362, #28342, #25356, #8753 ),
 ( #17539, #31747, #34739, #35161, #23931, #31533, #12153, #12368, #38149, #5782, #18737, #8962, #30541, #2590, #15550, #28552, #14337, #38360, #37720, #9175, #22132, #18951, #31957, #2796, #27136, #7768, #20731, #11155, #4581, #36000, #12774, #25764, #15, #10208, #32166, #13411, #35363, #41771, #19367, #28758, #25559, #9582, #3415, #3001, #3202, #9790, #16164 ),
 ( #32582, #36213, #6397, #38771, #15961, #28959, #35791, #22551, #35581, #13202, #16597, #29169, #41975, #19574, #19783, #32373, #12981, #25974, #441, #22758, #38982, #32802, #23178, #6603, #16382, #29387, #227, #38563, #26186, #9376, #39190, #26400, #7034, #9998, #22970, #12572, #6813, #3633, #39405, #29606, #20001, #33019, #15753, #22340, #6193, #19162, #1066 ),
 ( #23612, #13831, #17231, #1488, #11259, #4060, #14445, #40047, #653, #7455, #21045, #33232, #14238, #11054, #30645, #30227, #24039, #37054, #20412, #7246, #40260, #17437, #33441, #20205, #26829, #858, #27455, #33858, #4268, #14034, #10633, #7872, #24245, #40468, #17019, #3848, #20834, #39836, #36633, #27038, #37253, #30018, #8071, #23395, #29814, #10840, #16812 ),
 ( #23825, #36845, #7664, #20622, #1280, #4687, #33652, #13621, #4477, #30434, #27244, #17643, #26612, #39619, #10425, #36427, #34902, #5313, #34278, #37878, #38095, #11675, #5107, #21451, #18687, #41084, #18059, #8910, #41509, #18264, #31267, #31062, #34688, #1698, #1900, #27657, #5517, #31697, #28500, #34481, #11892, #4897, #24881, #2109, #2539, #8701, #25302 ),
 ( #12314, #8278, #21664, #15073, #18475, #31480, #24662, #14863, #28073, #15500, #38305, #27866, #9126, #2325, #30853, #37671, #34070, #21248, #15285, #41297, #28290, #12101, #25090, #5734, #21876, #17852, #14653, #8494, #40668, #11460, #40874, #24450, #37454, #22501, #13150, #5941, #12522, #26143, #35531, #29559, #18900, #38724, #6351, #32325, #19321, #16334, #35953 ),
 ( #3154, #25717, #28707, #16118, #28912, #9744, #19733, #29121, #39145, #31910, #25513, #9949, #42140, #394, #2747, #9532, #12935, #6766, #25925, #29339, #22922, #38934, #38513, #181, #35741, #22713, #9330, #2948, #19111, #32754, #3588, #6553, #19528, #41927, #16549, #13361, #26350, #22293, #22087, #39356, #32118, #15912, #32535, #35114, #35318, #15702, #41716 ),
 ( #6145, #12728, #3367, #40002, #26565, #39791, #4221, #10585, #7614, #4435, #26991, #30600, #808, #33184, #10378, #23347, #30181, #16969, #7201, #20576, #11008, #23563, #36385, #13987, #14192, #29968, #20159, #36585, #37006, #17182, #4012, #27197, #17596, #7403, #20365, #13784, #10793, #19955, #26780, #3798, #23775, #7825, #4639, #33387, #1022, #23130, #36796 ),
 ( #33602, #1438, #17393, #23987, #14398, #39572, #30384, #1235, #40210, #20787, #33811, #27406, #10160, #36167, #6985, #32973, #16760, #29767, #603, #13577, #15454, #27610, #8653, #5469, #11626, #24404, #41035, #8027, #11418, #34023, #11844, #38045, #34856, #40827, #18216, #11212, #31217, #24613, #25042, #2061, #31652, #5263, #12052, #5688, #14605, #15025, #37621 ),
 ( #31010, #24196, #28025, #8865, #1852, #4848, #37410, #24831, #21614, #18645, #18428, #34641, #34430, #2492, #20998, #8444, #37826, #17804, #14816, #30801, #31436, #40619, #8229, #1650, #21402, #21827, #40416, #37206, #15242, #28243, #21202, #2278, #34228, #41247, #5057, #18013, #27818, #2701, #42098, #25677, #22455, #6510, #35277, #15870, #16289, #35484, #32286 ),
 ( #35914, #15658, #32494, #22045, #38684, #28662, #9290, #6306, #9700, #3543, #38472, #6724, #13103, #29293, #41674, #35074, #9490, #136, #26095, #39101, #12482, #28876, #19278, #9080, #3115, #19692, #3322, #16075, #19485, #22251, #9904, #25258, #5895, #29079, #35699, #18856, #32709, #31861, #12893, #25476, #6102, #22876, #38888, #19065, #32071, #28456, #41462 ),
 ( #2907, #12269, #38263, #25881, #41889, #12687, #22666, #4172, #20526, #10745, #19909, #16504, #30136, #29716, #558, #33135, #33556, #32924, #23726, #36124, #350, #23301, #29511, #10119, #10331, #36537, #3755, #3965, #13740, #16926, #17134, #975, #23510, #17346, #36338, #39527, #13533, #26521, #39742, #7154, #20113, #13942, #36745, #29926, #764, #7356, #26940 ),
 ( #26734, #7566, #10541, #20315, #39951, #13317, #33342, #4388, #26303, #39312, #16713, #23090, #6938, #13014, #10034, #6849, #12807, #32411, #25397, #3241, #25798, #39224, #16200, #3664, #19403, #26219, #19818, #28797, #29204, #9616, #48, #39017, #32205, #22374, #38804, #23006, #32835, #12606, #36034, #6430, #9210, #15995, #29636, #41811, #22791, #19607, #22584 ),
 ( #16630, #26008, #9825, #35616, #28995, #18987, #35827, #19198, #6643, #12405, #32620, #3452, #38399, #2829, #16415, #29421, #22167, #35199, #42012, #262, #6025, #13236, #31991, #15789, #25594, #38601, #9408, #35400, #6227, #3038, #23427, #39653, #40293, #30467, #891, #20659, #39439, #36246, #39866, #7698, #33049, #33891, #7067, #10663, #20031, #3880, #33685 ),
 ( #4508, #17674, #17470, #4721, #36455, #1312, #13447, #23644, #474, #30053, #36666, #10242, #30258, #7275, #26435, #20237, #29845, #23213, #16845, #40078, #11086, #683, #23861, #14268, #13655, #27279, #26645, #10873, #10457, #24073, #37085, #33263, #4092, #17051, #13865, #26859, #33474, #7902, #7487, #20447, #4304, #17267, #36880, #20867, #1098, #14066, #27070 ),
 ( #4710, #27678, #8301, #30457, #4919, #24266, #27266, #34090, #27478, #21271, #18285, #21065, #11698, #4498, #11076, #24685, #17873, #28094, #17459, #37272, #30875, #5331, #1719, #27886, #37692, #8092, #24059, #14884, #34299, #14674, #37074, #1512, #17664, #31288, #8514, #40690, #11482, #40487, #40894, #41105, #2130, #20854, #20645, #21473, #30664, #14468, #24472 ),
 ( #15093, #40284, #1301, #37474, #33675, #14258, #11281, #5130, #7893, #18081, #31083, #1922, #34504, #11912, #24900, #37899, #33882, #6363, #9145, #41943, #34707, #41317, #12744, #22103, #16130, #5537, #25322, #35131, #35547, #5958, #15928, #25731, #12334, #12122, #2965, #22308, #38327, #25112, #31716, #5753, #19333, #38738, #18917, #31927, #15519, #28926, #29133 ),
 ( #8722, #9546, #18706, #2558, #2764, #3168, #38116, #32339, #28310, #18495, #15719, #21683, #31499, #28521, #38530, #8929, #28724, #41735, #12540, #6160, #22516, #25529, #42152, #41529, #9345, #21897, #34926, #35332, #19127, #32133, #12947, #25937, #2347, #15305, #620, #821, #16564, #9965, #26365, #23577, #3814, #22937, #13797, #4234, #23144, #10175, #35965 ),
 ( #6779, #32546, #39586, #36600, #33404, #39373, #16777, #9760, #29781, #36181, #7420, #13589, #30194, #26578, #10598, #17195, #13167, #10391, #7001, #23363, #36397, #29573, #19748, #19970, #20378, #1035, #39159, #14000, #32987, #35755, #409, #38947, #26157, #7214, #4025, #20173, #33199, #32768, #16983, #29983, #6570, #26795, #13377, #3381, #16348, #39805, #22725 ),
 ( #19540, #3600, #29353, #193, #14412, #21012, #27419, #24417, #21215, #1664, #5280, #17610, #7836, #27211, #40226, #4863, #33824, #24001, #37422, #27834, #40432, #11020, #30818, #31027, #4653, #37021, #11224, #11644, #34035, #20800, #1867, #34447, #24209, #37220, #30611, #27623, #36811, #1453, #20587, #40633, #24628, #21420, #8039, #17818, #40016, #14620, #11429 ),
 ( #18231, #8243, #40841, #31233, #1249, #34242, #5074, #18025, #14829, #37638, #8462, #2075, #27004, #10808, #23790, #7629, #33616, #4447, #17405, #30399, #14205, #25489, #22266, #25272, #41477, #41262, #22061, #2717, #24848, #12284, #18660, #21630, #28471, #21841, #15673, #12702, #15468, #6117, #41050, #5483, #19083, #38276, #22471, #11861, #31666, #9095, #41902 ),
 ( #32086, #2507, #18443, #9305, #28677, #35087, #31449, #38061, #12069, #25691, #2921, #5910, #18871, #34869, #35290, #35501, #38696, #15254, #15041, #15884, #25056, #8878, #31876, #9505, #2293, #5702, #41687, #37845, #28257, #8668, #12495, #6320, #19293, #38486, #28889, #28041, #32298, #34656, #29941, #6956, #36555, #10132, #16942, #39762, #19500, #19925, #366 ),
 ( #22893, #13121, #16519, #780, #10557, #3340, #13756, #39326, #42112, #6739, #20332, #32510, #13548, #10349, #13332, #29527, #29311, #23105, #32942, #12907, #26321, #19710, #9716, #36139, #9923, #3771, #26752, #3560, #36356, #29094, #35716, #7171, #16731, #23528, #25898, #32728, #29735, #7373, #574, #23319, #20130, #26539, #6524, #39545, #33155, #3983, #16308 ),
 ( #3128, #16089, #38904, #22682, #35929, #153, #26113, #39117, #33572, #33358, #11383, #30351, #1200, #17564, #27780, #7582, #30977, #10761, #17152, #36973, #4190, #994, #27163, #20964, #20542, #20756, #27374, #33781, #30765, #27577, #7996, #11592, #23955, #14160, #4406, #17363, #11178, #40176, #10971, #1615, #34195, #4609, #7795, #37172, #37376, #30565, #1405 ),
 ( #14361, #8193, #40792, #40383, #24163, #30152, #33985, #4813, #17980, #17766, #40585, #24370, #14572, #36763, #21162, #5019, #1817, #14781, #24575, #37581, #8408, #13958, #26957, #39971, #23742, #28625, #28839, #19027, #21579, #21368, #41639, #18391, #31402, #5654, #15833, #37790, #32033, #41000, #5228, #25009, #34395, #31184, #15202, #9042, #8617, #8831, #15415 ),
 ( #15621, #38228, #41852, #12014, #2244, #34606, #5435, #41425, #28205, #41213, #18817, #22210, #34819, #38009, #25222, #25438, #21791, #18609, #31615, #6066, #28419, #2454, #38439, #12651, #12232, #22008, #35039, #5859, #2026, #31825, #14991, #2662, #2871, #25638, #12446, #9254, #18183, #35240, #38646, #27992, #11804, #24795, #16461, #23260, #3926, #25841, #13278 ),
 ( #36083, #29251, #19448, #22836, #7114, #16886, #9660, #20073, #3502, #6270, #13062, #26694, #38849, #19867, #16673, #19652, #35874, #35662, #29468, #39272, #19241, #6685, #26052, #16039, #32668, #16247, #10078, #33095, #9866, #521, #35445, #42060, #13494, #308, #29887, #32455, #26262, #32882, #9452, #3286, #725, #36295, #39484, #22627, #3080, #23049, #10290 ),
 ( #6473, #6897, #3714, #32250, #29678, #13700, #26480, #22419, #29041, #95, #12854, #39063, #33304, #36919, #4764, #30096, #30932, #4134, #7737, #17093, #937, #30715, #7944, #13907, #1142, #1567, #14731, #14523, #1771, #20487, #27533, #10501, #20703, #39701, #27107, #33729, #7317, #27320, #4348, #23471, #33514, #26899, #20277, #39911, #37122, #8145, #36497 ),
 ( #10705, #17716, #23684, #20913, #36705, #40540, #11335, #17310, #30299, #7526, #14108, #40119, #30509, #24323, #10913, #23902, #4552, #17512, #33936, #34142, #37329, #21116, #1350, #4969, #14307, #40333, #11127, #17927, #24114, #8570, #21960, #27943, #14941, #37530, #8786, #38391, #35191, #9202, #2617, #15577, #37746, #21744, #11541, #28582, #41590, #31140, #15365 ),
 ( #18767, #31351, #1979, #34990, #41378, #2194, #40951, #21531, #24744, #25388, #12398, #28156, #41162, #34563, #5811, #11756, #27733, #31776, #5390, #18345, #11968, #22161, #15152, #6017, #5183, #24525, #24960, #40744, #8355, #37961, #28371, #34770, #5603, #18558, #31564, #25177, #18981, #2405, #31985, #12184, #38178, #8992, #2823, #21323, #34351, #18135, #13803 ),
 ( #15986, #20180, #20383, #35607, #28987, #3820, #1040, #23369, #42003, #33409, #23795, #625, #29786, #12800, #16988, #25587, #25791, #9402, #29989, #14005, #10814, #16783, #36402, #28790, #7219, #13595, #27011, #33204, #7635, #4030, #30200, #36816, #32197, #828, #26583, #26801, #39810, #6423, #38796, #39594, #40020, #20594, #9608, #33623, #10397, #12600, #19396 ),
 ( #10603, #23583, #36606, #7425, #22576, #4241, #17202, #38594, #15782, #32992, #22366, #41802, #35391, #6220, #19190, #3031, #37644, #30406, #37028, #8470, #4868, #11866, #1255, #21017, #17826, #31238, #30824, #11649, #21425, #8044, #7842, #40847, #18030, #34040, #20805, #27425, #1459, #2081, #34453, #1670, #14625, #11230, #24634, #24855, #15045, #27629, #40640 ),
 ( #24215, #34250, #28047, #11434, #5286, #14210, #33831, #18236, #24422, #37852, #27217, #37427, #8248, #41056, #21220, #8674, #21635, #5080, #4659, #4452, #31032, #1873, #17615, #40438, #14418, #17410, #40231, #14835, #27839, #37225, #11026, #24007, #30616, #34875, #34661, #12707, #31671, #2512, #18877, #29100, #8883, #32303, #12075, #18449, #38282, #5489, #2299 ),
 ( #21847, #22066, #28683, #35092, #32092, #28893, #9310, #12912, #25277, #15476, #5708, #18665, #12502, #41482, #28478, #2927, #35507, #5915, #12290, #38491, #38703, #9100, #31886, #2722, #19297, #41692, #15679, #9510, #42119, #25494, #22272, #35296, #6124, #15259, #19089, #28262, #15889, #3133, #25904, #41907, #25697, #31455, #22479, #6326, #16094, #38910, #9722 ),
 ( #41270, #25062, #38066, #10353, #7176, #371, #32734, #36146, #20337, #30157, #22897, #33362, #16736, #19505, #26326, #39975, #9928, #33159, #29945, #32949, #6961, #6746, #29740, #23325, #32516, #39767, #10561, #3565, #3778, #6529, #23534, #36561, #26119, #36360, #39122, #20136, #19932, #581, #785, #29535, #10139, #7377, #13553, #26543, #19714, #39550, #998 ),
 ( #16313, #3987, #35934, #16526, #16947, #13760, #22687, #13337, #13962, #4195, #17157, #39332, #29317, #26757, #26962, #35721, #3347, #23110, #159, #13129, #33576, #14576, #31187, #14784, #27581, #30980, #4613, #1820, #7586, #4410, #8000, #17983, #1204, #2032, #17367, #20969, #30356, #14164, #27786, #21168, #27171, #14367, #40796, #27995, #11596, #14995, #33785 ),
 ( #33991, #10768, #40387, #4819, #20547, #40589, #17568, #23748, #30571, #40182, #10976, #23960, #8197, #21372, #36767, #34200, #24579, #36978, #37585, #7799, #5025, #20761, #8413, #34398, #1411, #27377, #11182, #24167, #37177, #1620, #5231, #17773, #30771, #11389, #24374, #18186, #37382, #19031, #35244, #35042, #6273, #8620, #9046, #5657, #9455, #31829, #21796 ),
 ( #28209, #21582, #22012, #22422, #19244, #35450, #2457, #5439, #12235, #18613, #28629, #38649, #41428, #32037, #24800, #31406, #2874, #25226, #32254, #37794, #15420, #38231, #25642, #5862, #6069, #15836, #28423, #2247, #28843, #12449, #18822, #15206, #34824, #38012, #3083, #41856, #2666, #15625, #31618, #12653, #16043, #41003, #41217, #11809, #34610, #8834, #41642 ),
 ( #18397, #25443, #12019, #25012, #38442, #9257, #22214, #39275, #9664, #32885, #7321, #33099, #3718, #7119, #22839, #20076, #25844, #22630, #26265, #36298, #19451, #20280, #35666, #10081, #6476, #32460, #3929, #39488, #3289, #32671, #16889, #4137, #29890, #33307, #9869, #728, #42063, #23053, #29045, #16464, #36087, #38853, #16677, #35878, #12857, #6689, #16250 ),
 ( #26483, #39704, #29254, #10295, #13705, #99, #26698, #13065, #23263, #26056, #10505, #23475, #19656, #3506, #39067, #29471, #313, #19870, #36500, #13281, #6901, #29681, #524, #13497, #11545, #37333, #11341, #11131, #24529, #26902, #27326, #23908, #27738, #7948, #40124, #24327, #37536, #17516, #37127, #30100, #20917, #30515, #1775, #33940, #8360, #24118, #30936 ),
 ( #4768, #14313, #17720, #1571, #36923, #27112, #1354, #14736, #21328, #17313, #40748, #30721, #13910, #20708, #34355, #4352, #27537, #8149, #40337, #14528, #1145, #40544, #21120, #39915, #34148, #33733, #23689, #4974, #7741, #17933, #17097, #940, #10709, #36708, #7530, #20491, #33517, #30303, #14113, #4556, #10918, #31990, #18564, #12404, #38398, #8790, #8574 ),
 ( #21748, #21537, #28162, #2199, #2828, #35197, #5608, #31571, #11972, #25396, #12605, #15788, #5394, #5187, #9208, #15157, #41166, #2410, #41810, #34567, #28796, #24750, #31144, #34775, #18140, #14945, #24965, #34996, #18350, #15371, #41384, #28377, #2623, #41595, #21966, #25592, #37965, #12189, #31355, #25182, #38183, #9000, #5816, #15582, #6023, #18772, #31783 ) ),
 .UNSPECIFIED., .F., .F., .F.,
 ( 4, 1, 1, 1, 1, 1, 1, 1, 1, 1, 1, 1, 1, 1, 1, 1, 1, 1, 1, 1, 1, 1, 1, 1, 1, 1, 1, 1, 1, 1, 1, 1, 1, 1, 1, 1, 1, 1, 1, 1, 1, 1, 1, 1, 1, 1, 4 ),
 ( 4, 1, 1, 1, 1, 1, 1, 1, 1, 1, 1, 1, 2, 1, 1, 1, 2, 1, 1, 1, 1, 1, 2, 1, 1, 1, 1, 1, 1, 1, 2, 1, 1, 1, 1, 1, 1, 1, 1, 1, 4 ),
 ( 0.000000000000000000, 0.007812500000000000000, 0.01562500000000000000, 0.02343750000000000000, 0.03125000000000000000, 0.04687500000000000000, 0.06250000000000000000, 0.07812500000000000000, 0.09375000000000000000, 0.1093750000000000000, 0.1250000000000000000, 0.1406250000000000000, 0.1562500000000000000, 0.1875000000000000000, 0.2187500000000000000, 0.2500000000000000000, 0.2812500000000000000, 0.3125000000000000000, 0.3281250000000000000, 0.3437500000000000000, 0.3750000000000000000, 0.4062500000000000000, 0.4375000000000000000, 0.4687500000000000000, 0.5000000000000000000, 0.5312500000000000000, 0.5625000000000000000, 0.5937500000000000000, 0.6250000000000000000, 0.6562500000000000000, 0.6718750000000000000, 0.6875000000000000000, 0.7187500000000000000, 0.7500000000000000000, 0.7812500000000000000, 0.8125000000000000000, 0.8437500000000000000, 0.8750000000000000000, 0.8906250000000000000, 0.9062500000000000000, 0.9218750000000000000, 0.9375000000000000000, 0.9531250000000000000, 0.9687500000000000000, 0.9765625000000000000, 0.9843750000000000000, 1.000000000000000000 ),
 ( 0.000000000000000000, 0.01539374999999999945, 0.03078749999999999890, 0.04618125000000002089, 0.06157499999999999779, 0.07696875000000003020, 0.09236250000000004179, 0.1077562499999999979, 0.1231499999999999956, 0.1431375000000000008, 0.1631250000000000200, 0.1831125000000000114, 0.2031000000000000028, 0.2063375000000000070, 0.2095750000000000113, 0.2128125000000000155, 0.2160500000000000198, 0.2667375000000000163, 0.3174250000000000682, 0.3681125000000000647, 0.4188000000000000611, 0.5201750000000000540, 0.6215500000000000469, 0.6266374999999999584, 0.6317250000000000920, 0.6368124999999997815, 0.6418999999999999151, 0.6469874999999999376, 0.6520749999999999602, 0.6571624999999999828, 0.6622500000000000053, 0.7044687500000000879, 0.7466875000000001705, 0.7889062500000000311, 0.8010555555555555207, 0.8311249999999998916, 0.8733437499999998632, 0.9155625000000000568, 0.9403166666666666895, 0.9577812500000000284, 1.000000000000000000 ),
 .UNSPECIFIED. ) ;
#31666=CARTESIAN_POINT ( 'NONE',  ( 2.275810046414661336, 157.5529522918930638, 1.704261365023472363 ) ) ;
#31669=CARTESIAN_POINT ( 'NONE',  ( -2.271240278323964468, 124.1308405194309188, 0.008591128553798703035 ) ) ;
#31670=CARTESIAN_POINT ( 'NONE',  ( 3.135079784281773918, -3.970030566872769562, -7.817010796087090263 ) ) ;
#31671=CARTESIAN_POINT ( 'NONE',  ( 13.94748453383783193, 150.2679186505038160, 1.219128122479325560 ) ) ;
#31672=CARTESIAN_POINT ( 'NONE',  ( -4.732562794078051915, 118.5930653697794384, -1.019569371435221417 ) ) ;
#31674=CARTESIAN_POINT ( 'NONE',  ( 18.06489503062820390, 125.1493905788104684, -0.4137567899827961915 ) ) ;
#31678=CARTESIAN_POINT ( 'NONE',  ( -4.074955089416341991, 118.2429491485453497, 0.1454234154749720065 ) ) ;
#31679=CARTESIAN_POINT ( 'NONE',  ( -13.70496720262328161, 119.6480011847128253, -0.2738578607176473945 ) ) ;
#31680=ORIENTED_EDGE ( 'NONE', *, *, #36346, .T. ) ;
#31682=CARTESIAN_POINT ( 'NONE',  ( -4.428416584346161144, 119.5534643524533465, -0.9253073463357188722 ) ) ;
#31683=CARTESIAN_POINT ( 'NONE',  ( -5.329450492226126990, 104.6144662015457243, -0.2809636609891541514 ) ) ;
#31684=CARTESIAN_POINT ( 'NONE',  ( -3.075464349291260557, 156.1450793681712241, -0.7387695966741766318 ) ) ;
#31685=CARTESIAN_POINT ( 'NONE',  ( 3.174366308151882254, 63.84746620154572838, 0.06343139340882768262 ) ) ;
#31686=CARTESIAN_POINT ( 'NONE',  ( 0.1312748386005784529, 117.9496053154094994, -1.403673244313596857 ) ) ;
#31689=CARTESIAN_POINT ( 'NONE',  ( -4.563195415240126174, 21.88328375387019165, -0.7336086519975816289 ) ) ;
#31693=CARTESIAN_POINT ( 'NONE',  ( -4.543829802832370035, 27.87764462337559834, 0.5128545597630081998 ) ) ;
#31694=CARTESIAN_POINT ( 'NONE',  ( 6.992351373757773381, 121.9428086355924847, 0.2543945838518893998 ) ) ;
#31696=CARTESIAN_POINT ( 'NONE',  ( -3.199182136055901626, 19.34408232073488065, 3.339653329369344004 ) ) ;
#31697=CARTESIAN_POINT ( 'NONE',  ( 18.14731753714279705, 154.1160801429439857, 1.378418044792611541 ) ) ;
#31698=CARTESIAN_POINT ( 'NONE',  ( 1.155656144204274094, 104.6144662015457243, -4.695275792171453411 ) ) ;
#31699=CARTESIAN_POINT ( 'NONE',  ( 2.565602711990033313, 107.6377026157736765, 4.562358351827791481 ) ) ;
#31700=CARTESIAN_POINT ( 'NONE',  ( 17.06313393459302574, 153.7580772870718988, -1.402989014430432446 ) ) ;
#31701=CARTESIAN_POINT ( 'NONE',  ( -10.90225753734639547, 122.6724665872831679, 1.173089625842028472 ) ) ;
#31702=CARTESIAN_POINT ( 'NONE',  ( 0.7725557299734273631, -15.30006921971679112, -0.5871674697799584841 ) ) ;
#31703=CARTESIAN_POINT ( 'NONE',  ( -21.97734904378691567, 136.8935083344700558, -1.380722529463845438 ) ) ;
#31704=CARTESIAN_POINT ( 'NONE',  ( 0.6674325042100914818, 1.652014723813869823, 0.7093539244141242595 ) ) ;
#31708=CARTESIAN_POINT ( 'NONE',  ( -15.99593626731850371, 146.6619865182943272, 0.4079709740032108067 ) ) ;
#31709=CARTESIAN_POINT ( 'NONE',  ( 2.999908722124702720, -15.10219813539979938, 5.696538855611934515 ) ) ;
#31710=CARTESIAN_POINT ( 'NONE',  ( 16.95093959817310036, 147.3835828867039766, -1.246432153888628713 ) ) ;
#31711=ORIENTED_EDGE ( 'NONE', *, *, #19630, .F. ) ;
#31712=CARTESIAN_POINT ( 'NONE',  ( 0.9705268335128862667, 115.7029418470908979, 1.748962964377746898 ) ) ;
#31713=CARTESIAN_POINT ( 'NONE',  ( -4.666417123046072035, 117.8349074441706534, -1.040161417730997462 ) ) ;
#31714=CARTESIAN_POINT ( 'NONE',  ( 4.599243292695290641, 121.2024757821991159, 0.09190382657876458583 ) ) ;
#31716=CARTESIAN_POINT ( 'NONE',  ( 14.08011273344093972, 154.3735777161816429, 2.279704494881448884 ) ) ;
#31719=CARTESIAN_POINT ( 'NONE',  ( 4.837884815698807017, 117.5445328966380174, -0.9682318550270561097 ) ) ;
#31720=CARTESIAN_POINT ( 'NONE',  ( 23.26894437362528834, 149.0206351951634076, 0.01026395906018904604 ) ) ;
#31724=CARTESIAN_POINT ( 'NONE',  ( 2.101534993908720228, -15.10541647001627297, 5.790699435179030630 ) ) ;
#31727=CIRCLE ( 'NONE', #13368, 0.5079999999999997851 ) ;
#31728=CARTESIAN_POINT ( 'NONE',  ( -4.619290091002365095, 118.0409613858636817, 0.6362367808012175940 ) ) ;
#31730=ORIENTED_EDGE ( 'NONE', *, *, #5071, .T. ) ;
#31732=CARTESIAN_POINT ( 'NONE',  ( -8.348687675306351252, 119.7531329056243123, -1.433503554597048257 ) ) ;
#31733=CARTESIAN_POINT ( 'NONE',  ( -2.249496549248517496, 107.4436264546101967, -4.650814322000806911 ) ) ;
#31734=CARTESIAN_POINT ( 'NONE',  ( 4.811414313804822207, 117.8278363537766182, 0.8915698343676533577 ) ) ;
#31735=CARTESIAN_POINT ( 'NONE',  ( 2.102813808753936087, -15.18136450426021256, 5.202461169095355942 ) ) ;
#31736=CARTESIAN_POINT ( 'NONE',  ( -0.3827772581122253492, 119.9741034315941732, 0.6590906510345962976 ) ) ;
#31737=CARTESIAN_POINT ( 'NONE',  ( -2.646443841375008432, -8.127818987380491578, -3.789199236247322133 ) ) ;
#31738=DIRECTION ( 'NONE',  ( -0.01997839162482761832, -1.040247600000950455E-18, 0.9998004120163610509 ) ) ;
#31740=CARTESIAN_POINT ( 'NONE',  ( 1.676539183893630991, 107.1743931308027129, -4.723177562573835253 ) ) ;
#31741=CARTESIAN_POINT ( 'NONE',  ( -9.008986559116538118, 121.9018297702777858, -1.332107995734232109 ) ) ;
#31744=CARTESIAN_POINT ( 'NONE',  ( -6.343766875392317317, 29.24386013958156738, 0.9673776462358610884 ) ) ;
#31745=CARTESIAN_POINT ( 'NONE',  ( -3.248591992300019715, 115.7029686349078759, 1.528045359830205729 ) ) ;
#31746=CARTESIAN_POINT ( 'NONE',  ( -1.544744425833544099, 4.816215111148435923, 4.377641278133862279 ) ) ;
#31747=CARTESIAN_POINT ( 'NONE',  ( 0.3196863354298822846, 116.7093555017326452, 0.2333483032394377543 ) ) ;
#31748=VERTEX_POINT ( 'NONE', #33493 ) ;
#31749=CARTESIAN_POINT ( 'NONE',  ( 2.261452999203317216, 104.6144662015480549, -4.834054640181143725 ) ) ;
#31750=CARTESIAN_POINT ( 'NONE',  ( 4.504576368470070591, -15.30243295294880745, -0.5136648547128764841 ) ) ;
#31751=CARTESIAN_POINT ( 'NONE',  ( -16.46135582144571430, 131.4813445454897192, 1.641276044305395088 ) ) ;
#31752=CARTESIAN_POINT ( 'NONE',  ( -0.8578381542044509755, 18.04903173543935679, 0.4659799999690844019 ) ) ;
#31754=CARTESIAN_POINT ( 'NONE',  ( 0.05603342037570913786, 10.86776798020533086, -0.9749832093204870986 ) ) ;
#31757=CARTESIAN_POINT ( 'NONE',  ( -6.070593021754335294E-14, 91.53346620154573543, 1.030917152101657972E-16 ) ) ;
#31758=CARTESIAN_POINT ( 'NONE',  ( 5.278237183132049815, 122.2451909684448310, 0.2611397421478204861 ) ) ;
#31759=CARTESIAN_POINT ( 'NONE',  ( -16.09504119906512898, 148.0691544347876345, 0.9470067175600013210 ) ) ;
#31760=CARTESIAN_POINT ( 'NONE',  ( 2.948382749353823051, 50.13146620154573441, 1.837270642369387641 ) ) ;
#31761=CARTESIAN_POINT ( 'NONE',  ( 3.302240090359226610, -14.10740904597654399, 3.820541190522989350 ) ) ;
#31762=CARTESIAN_POINT ( 'NONE',  ( 11.48915734413142609, 123.4929228318607386, -1.183242792625787354 ) ) ;
#31764=CARTESIAN_POINT ( 'NONE',  ( -13.08242246048941304, 122.4605402651681487, -1.816276721775475611 ) ) ;
#31765=DIRECTION ( 'NONE',  ( -4.017660918040594346E-17, 1.000000000000000000, 2.376309959284834438E-19 ) ) ;
#31766=CARTESIAN_POINT ( 'NONE',  ( 8.198496980573445114, 120.4865852927236318, 1.425346789075751852 ) ) ;
#31767=CARTESIAN_POINT ( 'NONE',  ( 4.074910602682932925, 118.2429491485453497, -0.1454311599470143046 ) ) ;
#31768=CARTESIAN_POINT ( 'NONE',  ( 15.28873023128500463, 143.4753230507764670, -0.02859522846259918843 ) ) ;
#31771=CARTESIAN_POINT ( 'NONE',  ( -2.445982073634199949, 107.2195770060406659, -4.733624241319121850 ) ) ;
#31775=CARTESIAN_POINT ( 'NONE',  ( -2.092221094934305192, 20.21789226318614041, 8.165053130886693822 ) ) ;
#31776=CARTESIAN_POINT ( 'NONE',  ( 10.33865867007032335, 123.8962982355681817, 1.239266749756491093 ) ) ;
#31777=CYLINDRICAL_SURFACE ( 'NONE', #38269, 5.588000000000006295 ) ;
#31778=CARTESIAN_POINT ( 'NONE',  ( 22.73457742531292780, 137.3553536570635742, 0.3842032436244985916 ) ) ;
#31779=ADVANCED_FACE ( 'NONE', ( #14495 ), #33279, .T. ) ;
#31780=CARTESIAN_POINT ( 'NONE',  ( -7.280302209287178528, 123.0424313102424492, -0.07662657258806349070 ) ) ;
#31783=CARTESIAN_POINT ( 'NONE',  ( -6.439802323014594534E-14, 156.3034662015457172, 9.765829976239106842E-17 ) ) ;
#31784=CARTESIAN_POINT ( 'NONE',  ( 6.819937116507564845, -4.819529739946951885, -5.002256584970107056 ) ) ;
#31785=CARTESIAN_POINT ( 'NONE',  ( 5.532858221982281499, 116.9390490013607717, -0.3964132980606658307 ) ) ;
#31787=CARTESIAN_POINT ( 'NONE',  ( 0.01386859376750094325, 119.8383472832138779, -0.6940411431075127480 ) ) ;
#31788=DIRECTION ( 'NONE',  ( -5.206863593109713661E-17, 1.000000000000000000, -1.077750396879097183E-30 ) ) ;
#31789=CARTESIAN_POINT ( 'NONE',  ( 4.773405134497627600, 114.7515004814629691, -1.662930411550287868 ) ) ;
#31790=CARTESIAN_POINT ( 'NONE',  ( 4.815508964495446520, -10.08105153662837061, -6.929324068793707880 ) ) ;
#31791=CARTESIAN_POINT ( 'NONE',  ( 1.569714848522641537, 117.3993836557345389, 1.461722088477706460 ) ) ;
#31793=FACE_OUTER_BOUND ( 'NONE', #8487, .T. ) ;
#31795=CARTESIAN_POINT ( 'NONE',  ( 0.2858543223547244105, 109.4728569552520554, -3.914881836256076664 ) ) ;
#31796=CARTESIAN_POINT ( 'NONE',  ( -14.92885934485206079, 156.1361208441215922, 0.4494106821051805922 ) ) ;
#31798=EDGE_LOOP ( 'NONE', ( #7366, #7409, #23993, #6950 ) ) ;
#31802=CARTESIAN_POINT ( 'NONE',  ( -10.99239764355705695, 127.9870461113106472, -0.1667489162830026461 ) ) ;
#31803=CARTESIAN_POINT ( 'NONE',  ( 5.089472049306802859, -15.08631191614791334, 3.825519591672899455 ) ) ;
#31804=CARTESIAN_POINT ( 'NONE',  ( -12.66950698665823438, 121.4495935343099688, 1.177842983441548030 ) ) ;
#31805=CARTESIAN_POINT ( 'NONE',  ( 14.35401710045865009, 121.2650221238243944, -0.8333810220845707661 ) ) ;
#31806=CARTESIAN_POINT ( 'NONE',  ( 1.068493265602401987, 5.690783753869971484, 4.496582723949734017 ) ) ;
#31810=CARTESIAN_POINT ( 'NONE',  ( -6.504806966450658722E-14, 124.9344662015457317, 5.107768156065721555E-17 ) ) ;
#31812=CARTESIAN_POINT ( 'NONE',  ( -8.931878350220518570, 122.0520977060996586, 0.9029078837920736511 ) ) ;
#31813=DIRECTION ( 'NONE',  ( -4.017660918040594346E-17, 1.000000000000000000, 2.376309959284834438E-19 ) ) ;
#31814=CARTESIAN_POINT ( 'NONE',  ( 10.78346871132522189, 121.7859837122882283, -1.235232998807843874 ) ) ;
#31815=CARTESIAN_POINT ( 'NONE',  ( -9.459309661781173162, 157.4068808874136209, -1.850812122078211219 ) ) ;
#31817=CARTESIAN_POINT ( 'NONE',  ( 0.7132078119427314178, 156.3865044363621450, -0.5782112914057381259 ) ) ;
#31818=ORIENTED_EDGE ( 'NONE', *, *, #24021, .F. ) ;
#31819=CARTESIAN_POINT ( 'NONE',  ( -12.25802010074281512, 153.5964916033214820, -2.078998712700113938 ) ) ;
#31820=CARTESIAN_POINT ( 'NONE',  ( 3.758269890760038034, -15.41186319813359162, 2.599103203065302292 ) ) ;
#31821=CARTESIAN_POINT ( 'NONE',  ( -4.065972646788793554, 118.2429491485453070, -0.3080848862740693250 ) ) ;
#31822=EDGE_CURVE ( 'NONE', #39307, #13530, #14475, .T. ) ;
#31824=CARTESIAN_POINT ( 'NONE',  ( -4.805733446620805260, 117.6714400353627781, 0.9243893074020221867 ) ) ;
#31825=CARTESIAN_POINT ( 'NONE',  ( 17.70445710129698114, 147.3864036964934598, 2.239206817186280674 ) ) ;
#31828=CARTESIAN_POINT ( 'NONE',  ( 6.696816702757251605, -2.959147833993511778, 5.158690622954519078 ) ) ;
#31829=CARTESIAN_POINT ( 'NONE',  ( 0.6563489144270290288, 156.3175253132196190, 0.2722359314208552261 ) ) ;
#31839=CARTESIAN_POINT ( 'NONE',  ( -13.42085051059978618, 156.9389434127184018, -0.1400394208249337025 ) ) ;
#31842=CARTESIAN_POINT ( 'NONE',  ( -6.914645095069842817, 121.8817256395018518, -0.4219592037419029329 ) ) ;
#31843=CARTESIAN_POINT ( 'NONE',  ( 4.999708720184146138, 117.4026903937521382, -0.8309563775561717991 ) ) ;
#31844=ORIENTED_EDGE ( 'NONE', *, *, #27427, .F. ) ;
#31845=CARTESIAN_POINT ( 'NONE',  ( 0.7130887386421452812, 115.7031546128015833, -1.731733134274537456 ) ) ;
#31846=CARTESIAN_POINT ( 'NONE',  ( -7.044359374033601462, 122.0696255612902519, -0.2151282384624542410 ) ) ;
#31847=CARTESIAN_POINT ( 'NONE',  ( 5.778079093609060024, -12.78747091716041240, 1.651671850763037463 ) ) ;
#31848=CARTESIAN_POINT ( 'NONE',  ( -16.54768821719736138, 125.2933801378020888, 1.124873388181685252 ) ) ;
#31851=CARTESIAN_POINT ( 'NONE',  ( 8.041834545246983268, 158.6767594643193604, 0.3248513814034967306 ) ) ;
#31852=CARTESIAN_POINT ( 'NONE',  ( -0.001966947951488413372, 120.9974662015458620, 0.09843411867983418995 ) ) ;
#31853=CARTESIAN_POINT ( 'NONE',  ( -5.008392216835970245, 117.3993836135851865, 0.7767235299482659894 ) ) ;
#31854=CARTESIAN_POINT ( 'NONE',  ( -0.6963090749671848600, 14.53960050853193842, 0.6834203841726373962 ) ) ;
#31855=CARTESIAN_POINT ( 'NONE',  ( -17.26848747421932018, 122.7565812399420651, -0.3979830900422687834 ) ) ;
#31859=CARTESIAN_POINT ( 'NONE',  ( -5.551648636414652671, 117.0334030889854233, 0.4298500987717784882 ) ) ;
#31861=CARTESIAN_POINT ( 'NONE',  ( 16.99346516877617574, 153.7580772870718988, 2.083520914717074568 ) ) ;
#31862=CARTESIAN_POINT ( 'NONE',  ( 7.743227489916772122, 119.4405053107883958, -1.058161572703685938 ) ) ;
#31863=CARTESIAN_POINT ( 'NONE',  ( 7.903470162808407196, 13.94468365673557742, -2.927854470364564587 ) ) ;
#31864=CARTESIAN_POINT ( 'NONE',  ( -10.97563396989523099, 119.3804150619309468, -1.219877759958876595 ) ) ;
#31865=CARTESIAN_POINT ( 'NONE',  ( 4.844896927831375599, 117.8262454600737783, -0.6943141436239437247 ) ) ;
#31866=CARTESIAN_POINT ( 'NONE',  ( 5.227511188233168404, 116.2365830367532595, 1.175287748399642451 ) ) ;
#31867=B_SPLINE_CURVE_WITH_KNOTS ( 'NONE', 3,
 ( #25274, #40636, #18027, #15256, #24851, #14832, #2295, #8465, #12071, #41052 ),
 .UNSPECIFIED., .F., .F.,
 ( 4, 2, 2, 2, 4 ),
 ( 0.000000000000000000, 0.001159845853739277684, 0.002319691707478555368, 0.003479537561217833051, 0.004639383414957110735 ),
 .UNSPECIFIED. ) ;
#31868=CARTESIAN_POINT ( 'NONE',  ( -5.978688551911978344, 155.3719879121972838, -0.01966617979267111863 ) ) ;
#31869=EDGE_CURVE ( 'NONE', #17052, #17144, #39690, .T. ) ;
#31870=CARTESIAN_POINT ( 'NONE',  ( -18.41737859239644948, 149.0103496150362901, -2.461622840412570845 ) ) ;
#31871=CARTESIAN_POINT ( 'NONE',  ( 4.774069126156925691, -15.45330506282495442, 3.807469687449487772 ) ) ;
#31873=CARTESIAN_POINT ( 'NONE',  ( -4.862865218882401308, 117.4080073120805565, -1.166082678461140443 ) ) ;
#31874=CARTESIAN_POINT ( 'NONE',  ( -1.957980696025146017, 117.9496056077522752, -1.362940820082817694 ) ) ;
#31876=CARTESIAN_POINT ( 'NONE',  ( 15.71196619591391475, 131.3838724160208926, 2.228970979916469197 ) ) ;
#31877=CARTESIAN_POINT ( 'NONE',  ( -6.637366883016756296E-14, 101.1854662015457365, -1.207165459283692464E-19 ) ) ;
#31880=AXIS2_PLACEMENT_3D ( 'NONE', #38599, #15993, #28993 ) ;
#31882=CARTESIAN_POINT ( 'NONE',  ( -5.811537524186242365, 124.3836500214474654, -0.1011232793223458964 ) ) ;
#31885=CARTESIAN_POINT ( 'NONE',  ( -0.3690887223898375868, -3.321408231106627973, -8.411989387140767604 ) ) ;
#31886=CARTESIAN_POINT ( 'NONE',  ( 12.50622671840189604, 130.7145975665201831, 1.030918987520083707 ) ) ;
#31887=CARTESIAN_POINT ( 'NONE',  ( 22.62544200675479900, 150.0155710288180444, -0.5141704484958252719 ) ) ;
#31890=CARTESIAN_POINT ( 'NONE',  ( -5.558013820752536027, 116.7166910876666606, -0.2637059437321115918 ) ) ;
#31891=CARTESIAN_POINT ( 'NONE',  ( -4.074955089416341991, 118.2429491485453354, 0.1454234154749719787 ) ) ;
#31892=CARTESIAN_POINT ( 'NONE',  ( 5.023959273832318218, 113.9634657096167842, -1.916936035570479202 ) ) ;
#31895=CARTESIAN_POINT ( 'NONE',  ( -4.666616009249764829, 119.7854802332205537, -0.9105328040180735716 ) ) ;
#31896=CARTESIAN_POINT ( 'NONE',  ( 5.256943553860875973, 116.0444662015457027, 1.293952898321280021 ) ) ;
#31897=CARTESIAN_POINT ( 'NONE',  ( -15.89661694251515556, 145.9828583539951126, -0.9138632209041558374 ) ) ;
#31899=CARTESIAN_POINT ( 'NONE',  ( 23.21373371908085304, 149.6306211361744829, 0.4638656453230914356 ) ) ;
#31901=VERTEX_POINT ( 'NONE', #19576 ) ;
#31902=CARTESIAN_POINT ( 'NONE',  ( -1.576536484031922480, 10.66345178295009788, -4.350723848753511369 ) ) ;
#31903=CARTESIAN_POINT ( 'NONE',  ( -4.917116127314222318, 105.1214984364436020, 2.097186129389184917 ) ) ;
#31904=CARTESIAN_POINT ( 'NONE',  ( -4.923269767626008431, 117.4099945271726142, 0.9488514777737178107 ) ) ;
#31907=CARTESIAN_POINT ( 'NONE',  ( 6.999671179798840015, 121.6295281583065133, 0.7244140712011665206 ) ) ;
#31909=CARTESIAN_POINT ( 'NONE',  ( 3.724956840101937505, 21.94285949141939440, 2.734508905299370518 ) ) ;
#31910=CARTESIAN_POINT ( 'NONE',  ( 8.073283135001478428, 117.9965348323767671, 0.8851005009521595301 ) ) ;
#31911=CARTESIAN_POINT ( 'NONE',  ( 2.862426770350078531, 104.6144662015457101, -3.896337952179533826 ) ) ;
#31912=CARTESIAN_POINT ( 'NONE',  ( 4.224297255521886285, 111.8944766893745424, 2.913178037176576307 ) ) ;
#31913=CARTESIAN_POINT ( 'NONE',  ( 19.06828360855645599, 152.1029585079319020, -1.398049597035978087 ) ) ;
#31914=CARTESIAN_POINT ( 'NONE',  ( -11.27566272104538569, 154.5781333488962446, 1.670651684902624057 ) ) ;
#31916=CARTESIAN_POINT ( 'NONE',  ( -0.2796867633624597893, 20.41853924017881283, 4.627572958784220702 ) ) ;
#31917=CARTESIAN_POINT ( 'NONE',  ( -22.93196816944047001, 148.6798292920915117, -1.431318312106270252 ) ) ;
#31918=ORIENTED_EDGE ( 'NONE', *, *, #27142, .F. ) ;
#31919=EDGE_CURVE ( 'NONE', #7672, #38078, #32584, .T. ) ;
#31921=CARTESIAN_POINT ( 'NONE',  ( -9.326662024493499459, 153.8845013697122965, 0.4488502173044094379 ) ) ;
#31922=CARTESIAN_POINT ( 'NONE',  ( 2.071654280177509300, -15.34349575202162441, 5.977339193430266207 ) ) ;
#31924=CARTESIAN_POINT ( 'NONE',  ( -4.660057157337337941, 118.0075560824071630, -0.7769649848974667927 ) ) ;
#31925=CARTESIAN_POINT ( 'NONE',  ( 0.6438746309740379647, 120.9974662015465867, 0.01286614746332145724 ) ) ;
#31927=CARTESIAN_POINT ( 'NONE',  ( 4.492596771379812282, 157.9011380394538833, 1.833279187945892952 ) ) ;
#31931=CARTESIAN_POINT ( 'NONE',  ( 4.866147868668515564, 117.4089627612368076, -0.9906677743061890196 ) ) ;
#31932=CARTESIAN_POINT ( 'NONE',  ( 18.56067064112282594, 154.1690995007799927, -0.05235235476399361515 ) ) ;
#31933=AXIS2_PLACEMENT_3D ( 'NONE', #7198, #11208, #11414 ) ;
#31938=CARTESIAN_POINT ( 'NONE',  ( 2.032084454478232161, -15.08528485642818318, 5.800687065324998670 ) ) ;
#31941=CARTESIAN_POINT ( 'NONE',  ( -4.625339627765448824, 118.0227720238258087, 0.6694514315784764191 ) ) ;
#31943=CARTESIAN_POINT ( 'NONE',  ( -0.4613933488989553910, 118.7629491485454025, -1.278559111267616455 ) ) ;
#31944=CARTESIAN_POINT ( 'NONE',  ( -8.329558457569385510, 119.8456229460195885, -1.441662697695123008 ) ) ;
#31945=CARTESIAN_POINT ( 'NONE',  ( -4.398525312958116551, 119.2572634999566930, -0.5937511404893218714 ) ) ;
#31946=CARTESIAN_POINT ( 'NONE',  ( 4.599167112255276635, 117.9522226071726436, 0.9463719716926317638 ) ) ;
#31947=CARTESIAN_POINT ( 'NONE',  ( 3.198224922426783579, -14.19254063666773291, 2.189163805996276579 ) ) ;
#31948=CARTESIAN_POINT ( 'NONE',  ( -11.15578272721385211, 126.1638007343821641, -1.112962985253807657 ) ) ;
#31951=CARTESIAN_POINT ( 'NONE',  ( 5.362262919126890459, 116.9387654363850260, -0.7435593652664852504 ) ) ;
#31952=CARTESIAN_POINT ( 'NONE',  ( -10.79589323670149525, 123.3109526380878833, -1.504350731661493912 ) ) ;
#31953=CARTESIAN_POINT ( 'NONE',  ( 18.86374853661768825, 125.3403196291361610, 0.3769425889880999581 ) ) ;
#31954=CARTESIAN_POINT ( 'NONE',  ( 5.274109024393328404, 115.7029491485453150, -0.8140283081321302294 ) ) ;
#31956=CARTESIAN_POINT ( 'NONE',  ( 1.616848224653315569, 9.589005055319924864, -4.350374724214612243 ) ) ;
#31957=CARTESIAN_POINT ( 'NONE',  ( 21.11962238282686499, 132.3956117394162106, 1.087766252141818324 ) ) ;
#31959=CARTESIAN_POINT ( 'NONE',  ( 3.569197635593082563, 104.6144662015456959, -3.263097013630751775 ) ) ;
#31960=CARTESIAN_POINT ( 'NONE',  ( 1.983586949722073500, -15.35435952563934947, 5.265070481109153988 ) ) ;
#31961=CARTESIAN_POINT ( 'NONE',  ( -12.54292998015204752, 122.5542284311838870, 1.320227961537941086 ) ) ;
#31962=CARTESIAN_POINT ( 'NONE',  ( -0.2236011429256814231, 15.24623788552754888, -0.9474642044971398613 ) ) ;
#31963=CARTESIAN_POINT ( 'NONE',  ( 0.7290388503741822568, 0.07276798020498101427, -0.6497956273326017662 ) ) ;
#31965=AXIS2_PLACEMENT_3D ( 'NONE', #27158, #13544, #16725 ) ;
#31967=CARTESIAN_POINT ( 'NONE',  ( -4.973569738608247803, 117.3993868453981548, -0.9750659555622913643 ) ) ;
#31968=CARTESIAN_POINT ( 'NONE',  ( 4.275575466068057828, 118.7880935209305591, 0.6699701396488104699 ) ) ;
#31970=CARTESIAN_POINT ( 'NONE',  ( -9.727312926402552407, 123.7664141286412871, 0.5879621312111034115 ) ) ;
#31971=CARTESIAN_POINT ( 'NONE',  ( -8.981069108608934926, 123.9698733229553937, -0.1794631345465900474 ) ) ;
#31972=CARTESIAN_POINT ( 'NONE',  ( 3.119424175201863214, -14.34824051949108714, 4.229366443754182470 ) ) ;
#31973=CARTESIAN_POINT ( 'NONE',  ( 9.240212912644766519, 121.6705353891887995, -1.055487293716821817 ) ) ;
#31974=CARTESIAN_POINT ( 'NONE',  ( -12.43266001442903068, 122.1796674805547980, -1.793313828261402065 ) ) ;
#31976=LINE ( 'NONE', #22357, #8398 ) ;
#31977=CARTESIAN_POINT ( 'NONE',  ( -5.561288968297983359, 31.82205145332388341, 3.034443710062491917 ) ) ;
#31978=CARTESIAN_POINT ( 'NONE',  ( 15.33898570969095942, 143.5038931315047535, -0.1524207748662384510 ) ) ;
#31980=CARTESIAN_POINT ( 'NONE',  ( 3.177488185987922709, -14.13217061847354472, 2.003775387181677026 ) ) ;
#31984=CARTESIAN_POINT ( 'NONE',  ( -4.326994387844902867, 19.77997674669536465, 7.266063235268683584 ) ) ;
#31985=CARTESIAN_POINT ( 'NONE',  ( 11.23392777908751761, 153.2158294759273360, 1.564101052410651338 ) ) ;
#31986=CARTESIAN_POINT ( 'NONE',  ( -6.585902005698190595E-14, 91.53346620154573543, 1.207165459464729879E-19 ) ) ;
#31987=CARTESIAN_POINT ( 'NONE',  ( 9.815320032039958065, 117.9943556427423488, 0.1502691370658186254 ) ) ;
#31988=CARTESIAN_POINT ( 'NONE',  ( -4.033305401784485156, 109.8300753404742096, 3.515372713824419737 ) ) ;
#31990=CARTESIAN_POINT ( 'NONE',  ( 5.964965236245641123, 155.3820107761045790, 0.1591880423168910430 ) ) ;
#31991=CARTESIAN_POINT ( 'NONE',  ( 18.34395142906165077, 131.7683309214445728, 2.187682908440788054 ) ) ;
#31992=CARTESIAN_POINT ( 'NONE',  ( 8.062851560922409178, 27.27981867468588462, -2.430221966868060690 ) ) ;
#31993=CARTESIAN_POINT ( 'NONE',  ( 2.189084557043657675, 116.7689930370939919, -0.4207698416637195571 ) ) ;
#31994=CARTESIAN_POINT ( 'NONE',  ( -0.3588522330933500704, 120.9711055683163323, -0.4900691623393883534 ) ) ;
#31995=CARTESIAN_POINT ( 'NONE',  ( 4.560443946511397506, -11.68866997254031936, 0.6947937310338139216 ) ) ;
#31996=CARTESIAN_POINT ( 'NONE',  ( -0.1568781454184781377, 105.9760921070151767, -5.301024823544129738 ) ) ;
#31997=CARTESIAN_POINT ( 'NONE',  ( 0.2838385327444274964, 29.22985346960623332, -4.617364983570896086 ) ) ;
#31998=CARTESIAN_POINT ( 'NONE',  ( -4.800085724567980883, 115.7029491485352537, -1.472342921364584889 ) ) ;
#32000=CARTESIAN_POINT ( 'NONE',  ( 3.162461164278121739, -14.57801340048104777, 3.369881103115548893 ) ) ;
#32001=CARTESIAN_POINT ( 'NONE',  ( 0.3839444928496320020, 119.8383472832136931, -0.6866461459122011890 ) ) ;
#32002=CARTESIAN_POINT ( 'NONE',  ( -3.207477133065458563, 159.4163042773305676, 0.4796247595147200005 ) ) ;
#32007=CARTESIAN_POINT ( 'NONE',  ( 2.810429210790068133, -15.63944505633836712, 5.584101034811558506 ) ) ;
#32008=CARTESIAN_POINT ( 'NONE',  ( -13.26531225419064519, 121.8780043825237982, 1.199064809579205360 ) ) ;
#32010=CARTESIAN_POINT ( 'NONE',  ( 21.83021172428700751, 149.6930991844618291, -1.147003836765864371 ) ) ;
#32011=CARTESIAN_POINT ( 'NONE',  ( -2.948169924849943335, 1.592661447142720732, -3.562413953034572867 ) ) ;
#32013=ORIENTED_EDGE ( 'NONE', *, *, #10470, .T. ) ;
#32015=CARTESIAN_POINT ( 'NONE',  ( 0.3991458833604034084, 123.7646714092001190, 0.1312610764096186766 ) ) ;
#32017=B_SPLINE_SURFACE_WITH_KNOTS ( 'NONE', 3, 3, ( 
 ( #38600, #11761, #22373, #1984, #27947, #40956, #37750, #26434, #19197, #25797, #39438, #35826, #682, #32204, #9824, #6642, #20030 ),
 ( #32618, #29420, #13446, #47, #22790, #23211, #260, #39223, #32410, #10033, #13654, #22583, #10241, #28994, #3451, #9614, #16198 ),
 ( #16628, #10456, #3240, #26644, #33048, #36245, #35615, #42010, #16414, #7066, #3879, #16844, #6429, #19606, #13235, #15994, #23005 ),
 ( #29844, #36033, #39651, #29203, #35398, #3037, #12806, #26218, #473, #38803, #6226, #19402, #13013, #6847, #19817, #26006, #39016 ),
 ( #32834, #3663, #29635, #1522, #20446, #33473, #7697, #17884, #39865, #21074, #890, #7274, #27069, #36454, #33262, #17266, #11085 ),
 ( #10872, #17469, #23860, #20865, #17673, #40292, #1726, #14065, #4303, #23643, #36665, #1311, #30256, #1097, #33890, #24277, #36879 ) ),
 .UNSPECIFIED., .F., .F., .F.,
 ( 4, 2, 4 ),
 ( 4, 1, 1, 1, 1, 1, 1, 1, 1, 1, 1, 1, 1, 1, 4 ),
 ( 0.000000000000000000, 0.4999999999999997780, 1.000000000000000000 ),
 ( 0.000000000000000000, 0.08300113939718137268, 0.1732806554784933895, 0.2717672377176819087, 0.3752096606209606167, 0.4787223716043260135, 0.5772295444745598747, 0.6668133826162351285, 0.7470991451079272982, 0.7815930070524458317, 0.8169452614683294644, 0.8547689062991584708, 0.8968063284581728745, 0.9447228702782888288, 1.000000000000000000 ),
 .UNSPECIFIED. ) ;
#32018=CARTESIAN_POINT ( 'NONE',  ( -16.16280394421536215, 139.8573806175465961, 1.392748567604541909 ) ) ;
#32020=CARTESIAN_POINT ( 'NONE',  ( 18.96108613168456358, 147.8663216482595146, -1.723626476717959211 ) ) ;
#32022=CARTESIAN_POINT ( 'NONE',  ( -6.974227900756753584, 158.0922581832940921, -1.731937547952115297 ) ) ;
#32025=CARTESIAN_POINT ( 'NONE',  ( 3.641174103387447403, 120.8049117488720015, -0.2662595081522518559 ) ) ;
#32026=EDGE_LOOP ( 'NONE', ( #41780, #10116, #41653, #236 ) ) ;
#32027=CARTESIAN_POINT ( 'NONE',  ( -17.92322948971689911, 147.1528319293316542, -2.295422193410857403 ) ) ;
#32028=CARTESIAN_POINT ( 'NONE',  ( 2.500182370989485925, -15.36189011820890471, 4.810483652035355107 ) ) ;
#32029=CARTESIAN_POINT ( 'NONE',  ( -4.146183484540335584, 118.2391778865621745, -0.3987970906756914680 ) ) ;
#32032=CARTESIAN_POINT ( 'NONE',  ( -4.906328757273882957, 117.7163485839802064, 0.7384961846826334497 ) ) ;
#32033=CARTESIAN_POINT ( 'NONE',  ( 15.61558020634879007, 150.8349565870724120, 2.213412335539846509 ) ) ;
#32036=CARTESIAN_POINT ( 'NONE',  ( -2.768688662514669385, 30.30441277318858795, -3.700580903672975541 ) ) ;
#32037=CARTESIAN_POINT ( 'NONE',  ( 8.927705404389048027, 123.7033391712731145, 0.4040904458349093287 ) ) ;
#32040=CARTESIAN_POINT ( 'NONE',  ( -6.442660433036017764, 29.32943145771791649, -0.01012415147099491285 ) ) ;
#32041=AXIS2_PLACEMENT_3D ( 'NONE', #33254, #14058, #8094 ) ;
#32044=CARTESIAN_POINT ( 'NONE',  ( -8.631383859283502602, 118.4111954750946296, -1.057371476713716785 ) ) ;
#32047=CARTESIAN_POINT ( 'NONE',  ( -18.59469708476141747, 154.1615476314759974, -0.06268175667117097116 ) ) ;
#32050=CARTESIAN_POINT ( 'NONE',  ( -7.809620049061188674, 122.4698989756058864, -0.5308360719997577970 ) ) ;
#32053=CARTESIAN_POINT ( 'NONE',  ( 1.844371434233660345, 115.7029491485453718, -1.651278223000081757 ) ) ;
#32054=CARTESIAN_POINT ( 'NONE',  ( -15.72560005962105123, 146.8994026175788008, -0.4425663129111795380 ) ) ;
#32055=CARTESIAN_POINT ( 'NONE',  ( 5.397943591185104140, -12.01093657298729589, 0.9516947191793155847 ) ) ;
#32056=CARTESIAN_POINT ( 'NONE',  ( -14.39412078427935882, 121.9874158357064857, 1.026313471838276481 ) ) ;
#32058=CARTESIAN_POINT ( 'NONE',  ( 1.837930215757002772, 116.5452236745340429, 0.1764961812833933386 ) ) ;
#32059=CARTESIAN_POINT ( 'NONE',  ( 5.965539070479145778, 121.5454242706025383, 0.2305103670981815123 ) ) ;
#32060=CARTESIAN_POINT ( 'NONE',  ( 5.175750742582734709, 115.6909491485453145, -1.072434772098743716 ) ) ;
#32061=CARTESIAN_POINT ( 'NONE',  ( -0.6518678778066554491, 5.040965284779599820, 0.7259998264446282379 ) ) ;
#32063=CARTESIAN_POINT ( 'NONE',  ( -9.792313404876155758, 118.0024801742749929, -0.3345192158099827839 ) ) ;
#32064=B_SPLINE_CURVE_WITH_KNOTS ( 'NONE', 3,
 ( #22472, #13122, #19294, #16090, #9306, #42113, #3561, #12496, #29312, #2718, #35502 ),
 .UNSPECIFIED., .F., .F.,
 ( 4, 1, 1, 1, 1, 1, 1, 1, 4 ),
 ( 0.000000000000000000, 0.1250000000000006939, 0.2500000000000013878, 0.3750000000000020539, 0.5000000000000027756, 0.6250000000000061062, 0.7499999999999986677, 0.8750000000000019984, 1.000000000000000000 ),
 .UNSPECIFIED. ) ;
#32067=VERTEX_POINT ( 'NONE', #26613 ) ;
#32068=CARTESIAN_POINT ( 'NONE',  ( -5.607450786634617046, 117.5654562724977694, 0.7054197920332473393 ) ) ;
#32071=CARTESIAN_POINT ( 'NONE',  ( 2.834005798679493093, 158.8946464937287999, 1.432308184773210424 ) ) ;
#32072=CARTESIAN_POINT ( 'NONE',  ( 15.79478014299080435, 153.2725199748809928, -1.714666983805330558 ) ) ;
#32073=CARTESIAN_POINT ( 'NONE',  ( -0.5057995593169576365, 15.89392266832286182, -8.404578209849391968 ) ) ;
#32074=CARTESIAN_POINT ( 'NONE',  ( -18.58655447097580549, 128.6297099747515347, -1.738804191113343833 ) ) ;
#32075=CARTESIAN_POINT ( 'NONE',  ( 4.696390023408538283, 117.9631523383233969, -0.7094749930045800568 ) ) ;
#32077=CARTESIAN_POINT ( 'NONE',  ( 14.91134437184010864, 120.3281135999119158, 0.2979641475767020875 ) ) ;
#32078=CARTESIAN_POINT ( 'NONE',  ( -10.26263990951799165, 126.0184183664171655, -0.1119868329536247709 ) ) ;
#32079=CARTESIAN_POINT ( 'NONE',  ( -12.88625155327550331, 123.9867020804889961, -1.879256283450041032 ) ) ;
#32080=CARTESIAN_POINT ( 'NONE',  ( 2.577823224604873786, -15.72362945599133077, 5.534267358606157039 ) ) ;
#32082=DIRECTION ( 'NONE',  ( -0.9998004120163609398, 0.000000000000000000, -0.01997839162482749342 ) ) ;
#32086=CARTESIAN_POINT ( 'NONE',  ( -0.01111639999525440396, 119.1634951276629550, 0.5563101126475827884 ) ) ;
#32088=CIRCLE ( 'NONE', #1493, 4.826000000000001400 ) ;
#32090=CARTESIAN_POINT ( 'NONE',  ( -3.676218128927596140, 120.6652674781340551, 0.2791188998294429346 ) ) ;
#32091=CARTESIAN_POINT ( 'NONE',  ( -7.004517537292900720, 30.72436916340981838, -4.697416855195242213 ) ) ;
#32092=CARTESIAN_POINT ( 'NONE',  ( 3.627630705028838776, 120.8049117488720015, 0.4115075270184373468 ) ) ;
#32094=CARTESIAN_POINT ( 'NONE',  ( 21.87092457242483334, 136.8312970274703844, -0.6093905233339393934 ) ) ;
#32095=B_SPLINE_CURVE_WITH_KNOTS ( 'NONE', 3,
 ( #23914, #30309, #7955, #17940, #27745, #30942, #10924, #40344, #37134, #17319, #17726, #8367, #34155, #30729, #21127 ),
 .UNSPECIFIED., .F., .F.,
 ( 4, 2, 2, 2, 1, 2, 2, 4 ),
 ( 0.5000000000000000000, 0.5624999999999930056, 0.6249999999999928946, 0.7500000000000000000, 0.7812499999999951150, 0.8749999999999963363, 0.9374999999999982236, 1.000000000000000000 ),
 .UNSPECIFIED. ) ;
#32097=CIRCLE ( 'NONE', #10334, 0.5080000000000002292 ) ;
#32099=CIRCLE ( 'NONE', #14386, 0.5080000000000002292 ) ;
#32101=CARTESIAN_POINT ( 'NONE',  ( -0.0007535234283144901868, 116.4338605912342786, 0.03770939363766612207 ) ) ;
#32104=CARTESIAN_POINT ( 'NONE',  ( 4.491921773069756263, 119.5748936864404754, -0.7466653829840709244 ) ) ;
#32105=CARTESIAN_POINT ( 'NONE',  ( 4.840862041047174991, -14.92388815503642441, 4.310681236375266678 ) ) ;
#32106=CARTESIAN_POINT ( 'NONE',  ( -7.635798533888348061, 122.3449549946481056, -0.5106263504299666245 ) ) ;
#32107=DIRECTION ( 'NONE',  ( 0.9998004120163608288, 0.000000000000000000, 0.01997839162482749342 ) ) ;
#32108=CARTESIAN_POINT ( 'NONE',  ( 2.735903701988537051, 116.5290148844309357, 0.06805092059891054701 ) ) ;
#32110=CARTESIAN_POINT ( 'NONE',  ( 3.700881553190929374, 8.714383148187751615, -2.768892949411812854 ) ) ;
#32111=EDGE_CURVE ( 'NONE', #27588, #11942, #36283, .T. ) ;
#32114=CARTESIAN_POINT ( 'NONE',  ( 3.204964616970041646, 108.0380215227886680, 4.255332277598883550 ) ) ;
#32115=CARTESIAN_POINT ( 'NONE',  ( -7.016717161013801274, 121.3008223241220662, 0.6504084514987088506 ) ) ;
#32117=CARTESIAN_POINT ( 'NONE',  ( -1.246715508051662535, 10.49814879194060069, 4.449005273994115939 ) ) ;
#32118=CARTESIAN_POINT ( 'NONE',  ( 12.78669781772265956, 156.8686255264331635, 1.389142476906146895 ) ) ;
#32120=CARTESIAN_POINT ( 'NONE',  ( 3.116451998213339625, -14.00698646007624149, 1.619014592372306716 ) ) ;
#32121=CARTESIAN_POINT ( 'NONE',  ( 17.54996479678707288, 128.5781302034472162, -1.330722490425295446 ) ) ;
#32122=CARTESIAN_POINT ( 'NONE',  ( -3.984361711520921556, 7.699456178644025428, -2.362637291489932068 ) ) ;
#32123=CARTESIAN_POINT ( 'NONE',  ( -16.55455218413314356, 122.7279807066903032, -1.056987703419675739 ) ) ;
#32124=EDGE_CURVE ( 'NONE', #5098, #38197, #38226, .T. ) ;
#32126=CARTESIAN_POINT ( 'NONE',  ( -8.223969002016936258, 122.7966848691156514, 0.2142357769474922125 ) ) ;
#32127=CARTESIAN_POINT ( 'NONE',  ( 5.090702275550843758, -14.49510550894771121, 4.025111979839017806 ) ) ;
#32128=DIRECTION ( 'NONE',  ( -0.01997839162482737546, -1.040247600000939284E-18, 0.9998004120163610509 ) ) ;
#32130=CARTESIAN_POINT ( 'NONE',  ( -4.599484297918647435, 117.9522697134765963, -0.9462753457481243302 ) ) ;
#32131=CARTESIAN_POINT ( 'NONE',  ( 2.888995153171149077, 156.0927491134738716, 0.02440385714215731819 ) ) ;
#32133=CARTESIAN_POINT ( 'NONE',  ( 19.73710541150934006, 148.2167131080949787, 2.515028838702476399 ) ) ;
#32135=CARTESIAN_POINT ( 'NONE',  ( 0.03519895179119666290, 115.7029491485446613, -1.761499482103947800 ) ) ;
#32136=CARTESIAN_POINT ( 'NONE',  ( -16.34457059127857192, 122.7783120765077030, 0.5554794724330636146 ) ) ;
#32137=CARTESIAN_POINT ( 'NONE',  ( 5.008145846585815519, 117.3993852234726916, -0.7758522831737841852 ) ) ;
#32139=CARTESIAN_POINT ( 'NONE',  ( 22.51579307796273000, 137.1624432810789358, 0.01304004454942963957 ) ) ;
#32141=CARTESIAN_POINT ( 'NONE',  ( -5.166338518188872797, 115.7029491485453576, -1.236684454698984803 ) ) ;
#32144=CARTESIAN_POINT ( 'NONE',  ( -4.757346425016632629, 117.3993836136054227, -1.207075064339077963 ) ) ;
#32147=CARTESIAN_POINT ( 'NONE',  ( -4.590336119847570728, 118.0156493547208498, 0.6988070414943094999 ) ) ;
#32152=CARTESIAN_POINT ( 'NONE',  ( -3.332875914431231212, 118.5088515392226469, -0.9208157437338316820 ) ) ;
#32153=CARTESIAN_POINT ( 'NONE',  ( -7.253313547007707029, 123.0461458356614628, -0.2138788351844317370 ) ) ;
#32154=CARTESIAN_POINT ( 'NONE',  ( 4.641283449628422986, 117.8847305990883712, 1.004414769134842622 ) ) ;
#32155=CARTESIAN_POINT ( 'NONE',  ( 3.092642723064080279, -14.67800799544728285, 3.675123631970977911 ) ) ;
#32156=CARTESIAN_POINT ( 'NONE',  ( -6.495892026627714699, 121.2869106855140018, -0.7936256953933332747 ) ) ;
#32157=VECTOR ( 'NONE', #27908, 1000.000000000000227 ) ;
#32158=CARTESIAN_POINT ( 'NONE',  ( -3.600781874455683429, 115.7029491485453576, -1.622423596436841642 ) ) ;
#32161=CARTESIAN_POINT ( 'NONE',  ( 4.033305401784356370, 109.8300753404742096, -3.515372713824419737 ) ) ;
#32162=CARTESIAN_POINT ( 'NONE',  ( -13.52836484031764286, 128.5255724691869830, -1.838026323690954200 ) ) ;
#32163=CARTESIAN_POINT ( 'NONE',  ( -6.229205138088443228, 29.61971902930247325, 1.795445774805027428 ) ) ;
#32165=CARTESIAN_POINT ( 'NONE',  ( 3.315635589170361275, -10.27688868798473543, -3.234826238065520609 ) ) ;
#32166=CARTESIAN_POINT ( 'NONE',  ( 22.32005725002918339, 150.7328461917231550, 1.166919501784766666 ) ) ;
#32168=CARTESIAN_POINT ( 'NONE',  ( 3.161960256423347992, 104.6144662015368709, -4.310165282358256356 ) ) ;
#32169=CARTESIAN_POINT ( 'NONE',  ( 3.790367410748021637, -15.17722879538144198, -0.1767333597861489025 ) ) ;
#32170=CARTESIAN_POINT ( 'NONE',  ( -6.722174884994048583, 119.4737997143703012, 1.022258653430868192 ) ) ;
#32171=CARTESIAN_POINT ( 'NONE',  ( 0.3859925973045487679, 4.674766832570296238, -0.8944012262243137279 ) ) ;
#32174=CARTESIAN_POINT ( 'NONE',  ( 0.9436028068379492817, -1.428137797730904879, 0.2459283266283248115 ) ) ;
#32180=CARTESIAN_POINT ( 'NONE',  ( 2.027571083617039971, 109.8863472468248119, 3.714074494666526949 ) ) ;
#32182=CARTESIAN_POINT ( 'NONE',  ( -16.17714305270736830, 147.4171829256358137, 0.7878123557203799976 ) ) ;
#32184=CARTESIAN_POINT ( 'NONE',  ( 3.919216764667305064, -12.20455369412110080, 1.363517133079271026 ) ) ;
#32185=CARTESIAN_POINT ( 'NONE',  ( 11.30191013352078677, 123.2561760277034324, -1.170227508207775102 ) ) ;
#32186=CARTESIAN_POINT ( 'NONE',  ( 0.03212618750946916180, 158.2819368290249713, -1.607725792532325393 ) ) ;
#32188=CARTESIAN_POINT ( 'NONE',  ( 8.464818653216008570, 119.1964225064569263, 1.333813180544818344 ) ) ;
#32189=CARTESIAN_POINT ( 'NONE',  ( -4.138655142084676442, 33.37459457963606724, 1.694288919380972924 ) ) ;
#32190=CARTESIAN_POINT ( 'NONE',  ( 15.34424630368610032, 148.0267799683202554, -0.1426181633603110233 ) ) ;
#32194=CARTESIAN_POINT ( 'NONE',  ( -3.932819197772147390, 27.98301002373794333, 0.4898618918306563708 ) ) ;
#32197=CARTESIAN_POINT ( 'NONE',  ( 16.19371004148908710, 147.7868695473139553, 1.594401216537396637 ) ) ;
#32198=CARTESIAN_POINT ( 'NONE',  ( 4.756911902486301358, 117.3993836135862949, 1.207145067066230038 ) ) ;
#32199=CARTESIAN_POINT ( 'NONE',  ( 22.83585328881709131, 150.4073064562084880, 0.3794817294851796086 ) ) ;
#32200=CARTESIAN_POINT ( 'NONE',  ( -6.109903564962424483, 119.5248422734510427, 0.2725184514339176189 ) ) ;
#32202=CARTESIAN_POINT ( 'NONE',  ( -0.1363197777916403119, 115.6909491485452435, 1.761379840720195711 ) ) ;
#32204=CARTESIAN_POINT ( 'NONE',  ( -5.095652749712312080, 31.83908346630384756, 0.3959475160674750249 ) ) ;
#32205=CARTESIAN_POINT ( 'NONE',  ( 20.68324476251063615, 149.5879773183856685, 2.343194491808722191 ) ) ;
#32206=CARTESIAN_POINT ( 'NONE',  ( -4.384008014420753163, 17.61986127277741332, -1.463615122064717111 ) ) ;
#32207=CARTESIAN_POINT ( 'NONE',  ( 3.492884981554987611, 28.57741388400067706, -7.667201904029750992 ) ) ;
#32208=CARTESIAN_POINT ( 'NONE',  ( -2.161519886931281942, 116.7289984965020864, -0.4898792010161093780 ) ) ;
#32209=CARTESIAN_POINT ( 'NONE',  ( 0.08519874065837408639, 108.5751225745497948, -4.263693374914160117 ) ) ;
#32210=CARTESIAN_POINT ( 'NONE',  ( -23.11127252101368867, 149.9001116002701224, -0.4618182267416073850 ) ) ;
#32211=CARTESIAN_POINT ( 'NONE',  ( 3.691922595743098334, 109.5877055502880495, -3.633197977425771441 ) ) ;
#32212=CARTESIAN_POINT ( 'NONE',  ( 2.761911675679841860, 104.6144662015501012, 4.566626345672048615 ) ) ;
#32213=CARTESIAN_POINT ( 'NONE',  ( -3.130497002865707312, 23.39511390029671745, 3.426874451367011520 ) ) ;
#32216=CARTESIAN_POINT ( 'NONE',  ( 3.211984996733021624, -14.06435921420946755, 2.432701253525752172 ) ) ;
#32217=CARTESIAN_POINT ( 'NONE',  ( 0.3374525697214812436, 106.5118632461160217, -5.070939582669566903 ) ) ;
#32218=CARTESIAN_POINT ( 'NONE',  ( -14.33434017258165127, 120.4308286971427862, 0.3827902340739950393 ) ) ;
#32225=CARTESIAN_POINT ( 'NONE',  ( 4.774069126156925691, -15.45330506282495442, 3.807469687449487772 ) ) ;
#32226=CARTESIAN_POINT ( 'NONE',  ( -17.07772634048058791, 128.5677977248401476, 1.430458439683571115 ) ) ;
#32227=CARTESIAN_POINT ( 'NONE',  ( 11.01560508856915099, 119.3804150619309468, -0.7804404673305008755 ) ) ;
#32229=CARTESIAN_POINT ( 'NONE',  ( -1.576536484031922480, 10.66345178295009788, -4.350723848753511369 ) ) ;
#32231=ORIENTED_EDGE ( 'NONE', *, *, #30489, .F. ) ;
#32233=CARTESIAN_POINT ( 'NONE',  ( -0.009645608633146510874, 120.9711055683165597, 0.4827056984855356836 ) ) ;
#32234=CARTESIAN_POINT ( 'NONE',  ( -17.58003597271454765, 146.9817191466759141, 1.463309413676198378 ) ) ;
#32236=CARTESIAN_POINT ( 'NONE',  ( 3.344131534676130890, 119.2933411826354728, -0.7437009012386069928 ) ) ;
#32237=CARTESIAN_POINT ( 'NONE',  ( -11.72614449088027833, 156.4111399680655552, -2.003450915338490734 ) ) ;
#32241=CARTESIAN_POINT ( 'NONE',  ( 4.503783518555258603, 118.1168598955523663, -0.5561582125388926379 ) ) ;
#32242=CARTESIAN_POINT ( 'NONE',  ( 15.60301224545398036, 143.6313904367523833, -0.5515178422673748804 ) ) ;
#32243=ORIENTED_EDGE ( 'NONE', *, *, #29820, .T. ) ;
#32244=CARTESIAN_POINT ( 'NONE',  ( 0.02768739821002592222, 156.9833357668885014, -1.385590625008458643 ) ) ;
#32245=CARTESIAN_POINT ( 'NONE',  ( 3.347262984424072219, -14.85936863781750539, 0.1546827838429291613 ) ) ;
#32247=DIRECTION ( 'NONE',  ( 4.017660918040594346E-17, -1.000000000000000000, -2.376309959284834438E-19 ) ) ;
#32249=CARTESIAN_POINT ( 'NONE',  ( -4.833894161298425196, 117.7366906883232218, 0.8571493831372747341 ) ) ;
#32250=CARTESIAN_POINT ( 'NONE',  ( 2.540463897194693121, 119.9929590031203901, 0.6352340916430190276 ) ) ;
#32251=CARTESIAN_POINT ( 'NONE',  ( 2.711364258112229031, 37.31625399494021877, -1.095520810760639341 ) ) ;
#32253=CARTESIAN_POINT ( 'NONE',  ( -4.191205975170537279, 21.45845178295031630, -1.961646697876042511 ) ) ;
#32254=CARTESIAN_POINT ( 'NONE',  ( 9.348637138742738273, 124.2740283646700306, 0.4211050520620436832 ) ) ;
#32258=CARTESIAN_POINT ( 'NONE',  ( -0.8127763598983991367, 118.1588900138767997, 0.8680101205736402425 ) ) ;
#32261=FACE_OUTER_BOUND ( 'NONE', #36180, .T. ) ;
#32264=CARTESIAN_POINT ( 'NONE',  ( -1.415223785869884399, 159.6020224343070026, 0.1017758242917467665 ) ) ;
#32265=EDGE_LOOP ( 'NONE', ( #28256, #35812 ) ) ;
#32267=CARTESIAN_POINT ( 'NONE',  ( -7.822086219072885704, 122.4005678741224443, -0.6184629442691977896 ) ) ;
#32269=CARTESIAN_POINT ( 'NONE',  ( 2.054978793759712818, 115.7029326100966671, -1.635623593644852658 ) ) ;
#32270=CARTESIAN_POINT ( 'NONE',  ( -15.78746250177974808, 146.2429432508320417, -0.4439881280938304808 ) ) ;
#32271=CARTESIAN_POINT ( 'NONE',  ( 4.721559244837001401, -14.40436002768456802, 4.408607674763740825 ) ) ;
#32272=CARTESIAN_POINT ( 'NONE',  ( -10.67497907003079050, 119.8050749133877275, 0.9899969268117744248 ) ) ;
#32273=CARTESIAN_POINT ( 'NONE',  ( 3.174366308151880922, 104.6144662015457243, 0.06343139340882769650 ) ) ;
#32274=CARTESIAN_POINT ( 'NONE',  ( 3.280774808777962903, 159.4678586119998442, 0.2050961497903014685 ) ) ;
#32275=CARTESIAN_POINT ( 'NONE',  ( 9.092361046020325688, 153.9681463960921803, 0.2977057961392346463 ) ) ;
#32276=CARTESIAN_POINT ( 'NONE',  ( 5.205984836500144652, 115.6909491485453145, -1.025315722821639408 ) ) ;
#32277=CARTESIAN_POINT ( 'NONE',  ( -0.7871466699833823411, 12.39035052102135914, -0.5757299225971378442 ) ) ;
#32278=CARTESIAN_POINT ( 'NONE',  ( -18.76446887325688806, 125.2887878443791294, -0.4910110098351362362 ) ) ;
#32280=EDGE_CURVE ( 'NONE', #30579, #38903, #37850, .T. ) ;
#32283=CARTESIAN_POINT ( 'NONE',  ( -2.346178836033175230, 116.4819223308117984, 0.2686778099839046696 ) ) ;
#32286=CARTESIAN_POINT ( 'NONE',  ( -0.02399864187743109417, 159.1630378086529731, 1.200990174154242363 ) ) ;
#32287=CARTESIAN_POINT ( 'NONE',  ( 18.54838064703195499, 135.7714211226372640, -1.677382267734012666 ) ) ;
#32288=CARTESIAN_POINT ( 'NONE',  ( -8.422295717417405569, 8.547183656736235591, -0.3195422701574849311 ) ) ;
#32289=CARTESIAN_POINT ( 'NONE',  ( -12.43751437118963743, 120.3283006479967128, -1.391730434942824557 ) ) ;
#32290=CARTESIAN_POINT ( 'NONE',  ( 4.847166225461900346, 117.7641644975736739, -0.8119836883907423086 ) ) ;
#32291=CARTESIAN_POINT ( 'NONE',  ( 1.381059818124765526, 106.2379067940291293, 5.172899357470507553 ) ) ;
#32292=CARTESIAN_POINT ( 'NONE',  ( -9.076946558997759595, 124.0722828908287454, -0.1472919029216549491 ) ) ;
#32293=CARTESIAN_POINT ( 'NONE',  ( -18.92921826512576899, 147.2511928822236769, -2.484298966539742359 ) ) ;
#32294=CARTESIAN_POINT ( 'NONE',  ( 5.416639188517969217, -15.16156180871851333, 2.817365454923381307 ) ) ;
#32298=CARTESIAN_POINT ( 'NONE',  ( 16.28588378367221168, 151.0861551944122141, 2.361334407247334788 ) ) ;
#32301=CARTESIAN_POINT ( 'NONE',  ( -3.181806805318239562, 118.0279923103727242, 0.7725587567394768262 ) ) ;
#32302=CARTESIAN_POINT ( 'NONE',  ( -6.940074030747619638, 22.95585651114365788, 4.785772612677765991 ) ) ;
#32303=CARTESIAN_POINT ( 'NONE',  ( 6.262986112992323662, 155.3815620563194955, 0.9009107504210208672 ) ) ;
#32304=CARTESIAN_POINT ( 'NONE',  ( 22.69192130277340880, 142.3612397021088611, -0.6360799666370218208 ) ) ;
#32308=CARTESIAN_POINT ( 'NONE',  ( -5.757472737270721730, 159.1136035536173097, -0.1150480073142621795 ) ) ;
#32310=CARTESIAN_POINT ( 'NONE',  ( -8.104605239258354743, 120.9518455590310566, -1.347037562020136470 ) ) ;
#32311=CARTESIAN_POINT ( 'NONE',  ( -6.603988835907287056E-14, 91.53346620154573543, -3.493462572467304738E-18 ) ) ;
#32312=CARTESIAN_POINT ( 'NONE',  ( -15.91353055065151345, 146.3070982487133165, -0.9133378546330939152 ) ) ;
#32313=CARTESIAN_POINT ( 'NONE',  ( 2.381342306750187099, -14.83133394530772264, 5.477793184119461145 ) ) ;
#32315=CARTESIAN_POINT ( 'NONE',  ( 5.757472737270592944, 159.1136035536173097, 0.1150480073142623738 ) ) ;
#32316=EDGE_CURVE ( 'NONE', #31392, #15637, #34817, .T. ) ;
#32318=CARTESIAN_POINT ( 'NONE',  ( -4.492784857928645792, 12.16275517495587977, -1.104450737933446725 ) ) ;
#32319=CARTESIAN_POINT ( 'NONE',  ( -1.794468298957929475, 116.4672891243423578, -0.03585774721038168661 ) ) ;
#32323=CARTESIAN_POINT ( 'NONE',  ( -7.021952432075939221, 121.4379088036047563, 0.5782915293065207241 ) ) ;
#32324=CARTESIAN_POINT ( 'NONE',  ( 4.627658001546194555, 13.29687521248714610, 0.05192310334374634212 ) ) ;
#32325=CARTESIAN_POINT ( 'NONE',  ( 5.450899203173912966, 159.0107326448372191, 0.9576670044529983494 ) ) ;
#32326=CARTESIAN_POINT ( 'NONE',  ( 15.77133435453283461, 146.5691041611200660, 0.3151487940933137555 ) ) ;
#32328=CARTESIAN_POINT ( 'NONE',  ( 6.811759424595715373, 118.6475953829349379, -0.9158128249201541449 ) ) ;
#32329=CARTESIAN_POINT ( 'NONE',  ( 2.245307460665866728, 11.68515688572553479, 4.070821060848484940 ) ) ;
#32330=CARTESIAN_POINT ( 'NONE',  ( -22.49588706318651532, 149.6594668941642681, -1.627141970658571690 ) ) ;
#32333=CARTESIAN_POINT ( 'NONE',  ( -0.6320890182444199867, 120.8998192842950488, 0.1133706938477904158 ) ) ;
#32334=CARTESIAN_POINT ( 'NONE',  ( 5.507117158935161072, -13.70471586423162336, 3.054220594615255191 ) ) ;
#32335=CARTESIAN_POINT ( 'NONE',  ( -5.008697454415233175, 117.3984623471881292, 0.7756180019310896512 ) ) ;
#32337=ORIENTED_EDGE ( 'NONE', *, *, #8984, .T. ) ;
#32339=CARTESIAN_POINT ( 'NONE',  ( 5.838901281334536897, 119.0696708348911699, 1.193623469369259116 ) ) ;
#32340=FACE_OUTER_BOUND ( 'NONE', #36446, .T. ) ;
#32341=DIRECTION ( 'NONE',  ( -4.017660918040594346E-17, 1.000000000000000000, 2.376309959284834438E-19 ) ) ;
#32342=CARTESIAN_POINT ( 'NONE',  ( -15.42041356977108535, 121.5363848317736739, 0.5399810379570649799 ) ) ;
#32344=CARTESIAN_POINT ( 'NONE',  ( 0.002459394112954048622, 156.3065584682211124, -0.1230781383047672012 ) ) ;
#32345=CARTESIAN_POINT ( 'NONE',  ( 16.72896750809238853, 155.2649736186859570, -0.2017331744915135117 ) ) ;
#32349=CARTESIAN_POINT ( 'NONE',  ( -4.962828339513733589, 117.4036766243672076, -1.029743607666975036 ) ) ;
#32353=CYLINDRICAL_SURFACE ( 'NONE', #12505, 3.175000000000001155 ) ;
#32354=CARTESIAN_POINT ( 'NONE',  ( -4.554716542840457016, 118.0727055014217939, 0.6229934779673420575 ) ) ;
#32358=CARTESIAN_POINT ( 'NONE',  ( -0.7583562475726235430, 118.7629491485454025, -1.270948893816612690 ) ) ;
#32359=CARTESIAN_POINT ( 'NONE',  ( -8.356341240008237747, 119.7161836924744023, -1.429665635506445653 ) ) ;
#32360=CARTESIAN_POINT ( 'NONE',  ( -5.246142718657168302, 116.7267603939287426, -1.018146482794727525 ) ) ;
#32361=CARTESIAN_POINT ( 'NONE',  ( 4.716113435506099627, 117.7575315690381927, 1.081390950261145623 ) ) ;
#32362=CARTESIAN_POINT ( 'NONE',  ( 2.931439949929583122, -14.82325452411255640, 4.117531814738872420 ) ) ;
#32363=CARTESIAN_POINT ( 'NONE',  ( -10.11490785437018403, 123.9924233945428682, -1.115122180374877869 ) ) ;
#32364=CARTESIAN_POINT ( 'NONE',  ( -2.094230385292464192, 115.7021042694705955, -1.712899454762304430 ) ) ;
#32367=CARTESIAN_POINT ( 'NONE',  ( 6.897523911741961555, 121.8252198949890186, -0.01845719934638743662 ) ) ;
#32368=CARTESIAN_POINT ( 'NONE',  ( -16.94675455810626374, 147.0740084267719396, -1.925552282123431214 ) ) ;
#32369=CARTESIAN_POINT ( 'NONE',  ( -0.03245814172817904769, 157.7902383798253538, 1.624338139048501883 ) ) ;
#32372=CARTESIAN_POINT ( 'NONE',  ( 3.064284189169764971, -3.155149710853871525, 3.465721614369133174 ) ) ;
#32373=CARTESIAN_POINT ( 'NONE',  ( 15.17352684163996734, 120.8830733721255370, 0.9063557954379340975 ) ) ;
#32376=CARTESIAN_POINT ( 'NONE',  ( 3.819321967970790599, -15.20641387874817418, 0.06971680219106241028 ) ) ;
#32377=CARTESIAN_POINT ( 'NONE',  ( -15.17663987144310056, 128.5586215118215705, 1.546218023206676229 ) ) ;
#32378=CARTESIAN_POINT ( 'NONE',  ( 0.6656887758738300187, 13.74536131906779879, -0.7131539583378491143 ) ) ;
#32379=CARTESIAN_POINT ( 'NONE',  ( -2.795228999030447969, 116.6385632091030544, -0.2515850966972202896 ) ) ;
#32380=CARTESIAN_POINT ( 'NONE',  ( 0.8411255309083253140, 9.366862202269544468, -0.4933303560167117130 ) ) ;
#32381=ORIENTED_EDGE ( 'NONE', *, *, #7916, .T. ) ;
#32382=ORIENTED_EDGE ( 'NONE', *, *, #40219, .F. ) ;
#32384=CARTESIAN_POINT ( 'NONE',  ( 4.119305931990680847, 118.0988315448752530, 0.8046943418515852819 ) ) ;
#32386=CARTESIAN_POINT ( 'NONE',  ( -16.52109770691750867, 146.2355833862463328, 0.9494891650916720272 ) ) ;
#32387=CARTESIAN_POINT ( 'NONE',  ( 3.969679720280225421, -13.58737529183706627, 3.751183842293267290 ) ) ;
#32388=CARTESIAN_POINT ( 'NONE',  ( 17.67908073340989716, 148.3509993576462307, -1.576626744559513460 ) ) ;
#32389=CARTESIAN_POINT ( 'NONE',  ( -0.4459748878573762676, 118.5593716040226724, -0.6139719676240718016 ) ) ;
#32391=CARTESIAN_POINT ( 'NONE',  ( 2.102813808753936087, -15.18136450426021256, 5.202461169095355942 ) ) ;
#32392=CARTESIAN_POINT ( 'NONE',  ( -1.842030023794387406, 35.66238107416427994, 0.6533647080653418593 ) ) ;
#32393=CARTESIAN_POINT ( 'NONE',  ( 15.85793921209435098, 146.6055793175013093, -0.1365194753024329688 ) ) ;
#32396=CARTESIAN_POINT ( 'NONE',  ( -6.616924617768071466E-14, 97.37546620154573418, 7.965525879364083286E-30 ) ) ;
#32403=CARTESIAN_POINT ( 'NONE',  ( 15.89375338022607664, 121.0219768425927214, 0.2124277663179633124 ) ) ;
#32406=CARTESIAN_POINT ( 'NONE',  ( -7.694663930960380149, 124.9344662015457317, -0.1537576976229972081 ) ) ;
#32408=DIRECTION ( 'NONE',  ( -4.017660918040594346E-17, 1.000000000000000000, 2.376309959284834438E-19 ) ) ;
#32409=CARTESIAN_POINT ( 'NONE',  ( 4.636249899789679496, -11.37698174978397958, -0.2454043791197063895 ) ) ;
#32410=CARTESIAN_POINT ( 'NONE',  ( -3.786193870232612557, 33.00004608313867038, 1.177060218906804012 ) ) ;
#32411=CARTESIAN_POINT ( 'NONE',  ( 13.88956208308353801, 122.0315337860429423, 1.683705570428295495 ) ) ;
#32412=CARTESIAN_POINT ( 'NONE',  ( 0.3943543298815788134, 25.17882533764851871, -4.623353113333005915 ) ) ;
#32413=CARTESIAN_POINT ( 'NONE',  ( 5.686328549477039473, -14.11678386645415628, -6.209864621142330954 ) ) ;
#32414=CARTESIAN_POINT ( 'NONE',  ( 5.514681883891941361, 117.1567625688420691, -0.5563447151070903818 ) ) ;
#32415=CARTESIAN_POINT ( 'NONE',  ( -1.969999177844983684, 122.1523088006674840, -0.2733757396980688870 ) ) ;
#32417=CARTESIAN_POINT ( 'NONE',  ( 0.3678577911475685025, 105.9884271946378789, -5.283348413363662566 ) ) ;
#32418=CARTESIAN_POINT ( 'NONE',  ( 2.760961650891263552, 105.1243252582604129, 4.565018514838535602 ) ) ;
#32419=CARTESIAN_POINT ( 'NONE',  ( -0.1328416520900886078, 24.48205809745167372, 4.627450821846854190 ) ) ;
#32421=CARTESIAN_POINT ( 'NONE',  ( -1.969863483948048444, 117.3993837347434237, -1.449772854203450034 ) ) ;
#32422=CARTESIAN_POINT ( 'NONE',  ( 3.047801963512828394, -14.61332798263154054, 3.862229702996769376 ) ) ;
#32423=CARTESIAN_POINT ( 'NONE',  ( 2.437154581274076914, 119.8248006784163380, -0.4733635836876308178 ) ) ;
#32424=CARTESIAN_POINT ( 'NONE',  ( -11.41934419072027573, 118.9229013597968247, 0.3849275771520425105 ) ) ;
#32429=CARTESIAN_POINT ( 'NONE',  ( 6.125566448072323311, -14.60357603047697594, -0.1915981853098273624 ) ) ;
#32430=CARTESIAN_POINT ( 'NONE',  ( -7.829350110466720025, 119.0983413489662297, 1.000240898550800894 ) ) ;
#32431=CARTESIAN_POINT ( 'NONE',  ( 3.000642688540850145, 117.3922842568077698, -0.5420849065376539544 ) ) ;
#32432=CARTESIAN_POINT ( 'NONE',  ( -2.395914033174281865, 1.367755174955888275, -3.957843245732672877 ) ) ;
#32436=CIRCLE ( 'NONE', #5908, 5.334000000000001407 ) ;
#32438=CARTESIAN_POINT ( 'NONE',  ( -4.704233533693831681, 117.8349189730105309, 0.8529071958809373299 ) ) ;
#32439=CARTESIAN_POINT ( 'NONE',  ( -17.39219791206841137, 147.8988302317391117, 1.461875531624039493 ) ) ;
#32441=CARTESIAN_POINT ( 'NONE',  ( 13.69950719238972603, 125.8243951943327517, -1.418320022125399316 ) ) ;
#32442=CARTESIAN_POINT ( 'NONE',  ( -15.86975487622011016, 125.3951846505478329, -1.921535798876653711 ) ) ;
#32444=ORIENTED_EDGE ( 'NONE', *, *, #37802, .T. ) ;
#32445=CARTESIAN_POINT ( 'NONE',  ( 4.536962900200297355, 118.1142359939903486, -0.5195621094609307322 ) ) ;
#32446=CARTESIAN_POINT ( 'NONE',  ( 9.705341575047208735, 124.1466939447965814, -0.4180229424618548406 ) ) ;
#32448=CARTESIAN_POINT ( 'NONE',  ( -10.01853622893607643, 122.3915136462027817, -1.471741716425344570 ) ) ;
#32449=CARTESIAN_POINT ( 'NONE',  ( 2.845230715667840027, -15.32736664957809403, 4.381646938852296280 ) ) ;
#32450=CARTESIAN_POINT ( 'NONE',  ( 4.918680324695957395, 105.1215131357075450, -2.093362006766627648 ) ) ;
#32454=CARTESIAN_POINT ( 'NONE',  ( -4.833313786903620013, 117.6748972090164784, 0.9053765355249284719 ) ) ;
#32455=CARTESIAN_POINT ( 'NONE',  ( 16.32868586224174479, 149.3997711511537148, 2.122341471705227356 ) ) ;
#32456=CARTESIAN_POINT ( 'NONE',  ( -0.01822531903872333034, 118.1564764849152738, 0.9120692297075591037 ) ) ;
#32457=CIRCLE ( 'NONE', #8654, 3.683000000000001162 ) ;
#32459=CARTESIAN_POINT ( 'NONE',  ( -0.8080508600641240768, 24.25718022715097888, 4.550674767031389401 ) ) ;
#32460=CARTESIAN_POINT ( 'NONE',  ( 15.24801397198100972, 143.4548391324710224, 0.5370776308064710847 ) ) ;
#32462=VECTOR ( 'NONE', #9672, 1000.000000000000114 ) ;
#32464=CARTESIAN_POINT ( 'NONE',  ( -3.222356721042568317, 117.3993833695669906, 1.271110537006335139 ) ) ;
#32467=CARTESIAN_POINT ( 'NONE',  ( -8.795781703810718000, 117.6859433316420223, -0.2728653492683267845 ) ) ;
#32472=CARTESIAN_POINT ( 'NONE',  ( -22.95349865178522819, 150.1476136049543868, -0.1290964995630296541 ) ) ;
#32473=ORIENTED_EDGE ( 'NONE', *, *, #35802, .F. ) ;
#32475=CARTESIAN_POINT ( 'NONE',  ( -7.787039648717389184, 122.6067446965587067, -0.2565226439608999098 ) ) ;
#32478=CARTESIAN_POINT ( 'NONE',  ( -15.24801397198113762, 143.4548391324710224, -0.5370776308064708626 ) ) ;
#32479=CARTESIAN_POINT ( 'NONE',  ( 4.956269154958684808, -14.57630274377035029, 4.209183869072664841 ) ) ;
#32480=CARTESIAN_POINT ( 'NONE',  ( -12.10120965742751409, 156.5645100661158153, 1.400626166162074915 ) ) ;
#32482=CARTESIAN_POINT ( 'NONE',  ( 21.86057864824936559, 151.4416708234707301, 0.7622892283599554952 ) ) ;
#32483=COLOUR_RGB ( '', 0.72549020, 0.75294118, 0.79215686) ;
#32484=CARTESIAN_POINT ( 'NONE',  ( 14.12992900693046217, 138.8284504506842723, 0.4149782266466619518 ) ) ;
#32486=CARTESIAN_POINT ( 'NONE',  ( 0.6184700321857297123, 7.203955656377674543, 0.7581051976356608657 ) ) ;
#32487=CARTESIAN_POINT ( 'NONE',  ( -15.88955207386071677, 121.0219768425927214, -0.4226783167178084222 ) ) ;
#32491=CARTESIAN_POINT ( 'NONE',  ( 5.563236611437734069, 117.4964933332594939, 0.9016082036358555873 ) ) ;
#32492=ORIENTED_EDGE ( 'NONE', *, *, #24307, .F. ) ;
#32494=CARTESIAN_POINT ( 'NONE',  ( 1.092003032498458426, 117.6437429425539420, 0.5722403007656918783 ) ) ;
#32495=CARTESIAN_POINT ( 'NONE',  ( 0.01133701039331200082, 118.4098733054621277, -0.5673503590873753000 ) ) ;
#32496=CARTESIAN_POINT ( 'NONE',  ( -0.8194340683325834762, 6.824753112428224355, -0.5254904297167376503 ) ) ;
#32497=CARTESIAN_POINT ( 'NONE',  ( -6.293633234193186432, 17.08131519529194975, -5.670988759835773330 ) ) ;
#32498=CARTESIAN_POINT ( 'NONE',  ( -21.42793111275547346, 141.8478887571778273, -2.143904907781017943 ) ) ;
#32499=CARTESIAN_POINT ( 'NONE',  ( 4.744530630439001584, 117.8975126698502294, -0.7673925427075298789 ) ) ;
#32500=CARTESIAN_POINT ( 'NONE',  ( 5.244916502329305175, 116.2229785614576798, 1.177106425564501402 ) ) ;
#32501=CARTESIAN_POINT ( 'NONE',  ( 0.02156534543286487207, 156.6359106937186709, -1.079218069903262300 ) ) ;
#32503=CARTESIAN_POINT ( 'NONE',  ( -15.52759540040498543, 147.5317938866932366, -0.2591190040802685002 ) ) ;
#32505=CARTESIAN_POINT ( 'NONE',  ( -18.29412156995184446, 148.6295804641074483, -2.431306780064794282 ) ) ;
#32506=CARTESIAN_POINT ( 'NONE',  ( 4.894061823620152296, -15.42295773938226411, 3.608731902971048733 ) ) ;
#32510=CARTESIAN_POINT ( 'NONE',  ( 9.373281424700387277, 121.4347015428822374, 1.498606428831741111 ) ) ;
#32514=CARTESIAN_POINT ( 'NONE',  ( -2.298002300860151781, 118.5759350612125900, 0.7369678581462183464 ) ) ;
#32515=CARTESIAN_POINT ( 'NONE',  ( 3.492884981554987611, 28.57741388400067706, -7.667201904029750992 ) ) ;
#32516=CARTESIAN_POINT ( 'NONE',  ( 14.53200193279634433, 139.1552669279217298, 1.026914593849031165 ) ) ;
#32517=CARTESIAN_POINT ( 'NONE',  ( 14.83366055447111975, 120.8492938200443092, -0.4607208393402016933 ) ) ;
#32519=DIRECTION ( 'NONE',  ( -0.9998004120163608288, 0.000000000000000000, -0.01997839162482749342 ) ) ;
#32520=CARTESIAN_POINT ( 'NONE',  ( -5.775410652799862987, 116.9337168780244696, -0.1011920919882984826 ) ) ;
#32521=ORIENTED_EDGE ( 'NONE', *, *, #28132, .F. ) ;
#32522=CARTESIAN_POINT ( 'NONE',  ( -6.414862124821939737, 120.2136652291687113, -1.181229002280302254 ) ) ;
#32524=CARTESIAN_POINT ( 'NONE',  ( -9.165636745952109976, 123.6526633469202920, -0.6866826908162829701 ) ) ;
#32525=CARTESIAN_POINT ( 'NONE',  ( 4.292324012607982908, -12.68181061970326340, 2.304565294163185118 ) ) ;
#32526=DIRECTION ( 'NONE',  ( 0.9998004120163608288, 0.000000000000000000, 0.01997839162482749342 ) ) ;
#32527=CARTESIAN_POINT ( 'NONE',  ( 13.69515342115106904, 119.6466660129326272, 0.2899717296217781404 ) ) ;
#32528=VERTEX_POINT ( 'NONE', #25718 ) ;
#32529=CARTESIAN_POINT ( 'NONE',  ( -2.923568588381722844, 13.88697512809157786, 3.594856661414283394 ) ) ;
#32530=CARTESIAN_POINT ( 'NONE',  ( 5.182655383320532216, 105.1222097428776152, 1.273793769351906802 ) ) ;
#32533=CARTESIAN_POINT ( 'NONE',  ( 7.841223576139474183, 122.2967352183207339, 0.7262958897790078305 ) ) ;
#32534=CARTESIAN_POINT ( 'NONE',  ( -4.609865753310859127, 8.349128549105346409, -0.5081561704775721111 ) ) ;
#32535=CARTESIAN_POINT ( 'NONE',  ( 7.599585376671099901, 158.5456267226934131, 1.164890904197547261 ) ) ;
#32538=CARTESIAN_POINT ( 'NONE',  ( 21.06902287100046678, 145.7918284779248665, -1.526944944257475623 ) ) ;
#32539=CARTESIAN_POINT ( 'NONE',  ( 4.585212383536918956, 13.09695617864405470, 0.6580430208065696229 ) ) ;
#32540=CARTESIAN_POINT ( 'NONE',  ( -22.37507221999729623, 149.9331680011685251, -1.622875787667645620 ) ) ;
#32542=CARTESIAN_POINT ( 'NONE',  ( -4.346810452489807020, 155.8404949922767742, 0.3425513195823395307 ) ) ;
#32543=CARTESIAN_POINT ( 'NONE',  ( 5.566531978545880222, -14.14111126781847361, 3.212028819027522797 ) ) ;
#32544=CARTESIAN_POINT ( 'NONE',  ( -5.008842170714641107, 117.3975374489157133, 0.7756408261732131715 ) ) ;
#32545=ORIENTED_EDGE ( 'NONE', *, *, #13864, .F. ) ;
#32546=CARTESIAN_POINT ( 'NONE',  ( 0.4560022058367742548, 118.7114656741295988, 0.6168833707790647436 ) ) ;
#32547=CARTESIAN_POINT ( 'NONE',  ( 3.009276887026298031, 39.20946620154573736, -1.210121013456480599 ) ) ;
#32548=CARTESIAN_POINT ( 'NONE',  ( -6.550797450135577910E-14, 84.67546620154573134, 2.164564701558966795E-29 ) ) ;
#32549=VECTOR ( 'NONE', #9215, 1000.000000000000000 ) ;
#32550=CARTESIAN_POINT ( 'NONE',  ( -22.54293160324732526, 149.6594668941642681, 0.7271591872719226357 ) ) ;
#32551=ADVANCED_FACE ( 'NONE', ( #29340 ), #6838, .T. ) ;
#32552=EDGE_CURVE ( 'NONE', #27974, #40883, #38396, .T. ) ;
#32553=CARTESIAN_POINT ( 'NONE',  ( 23.16157447928863178, 142.6111785389246336, -0.1383437888640691449 ) ) ;
#32560=CARTESIAN_POINT ( 'NONE',  ( -4.541827306795418018, 118.0696916868041626, 0.6339922499592595129 ) ) ;
#32561=CARTESIAN_POINT ( 'NONE',  ( 3.682264917456193221, 72.48346620154573827, 0.07358041635424013294 ) ) ;
#32564=CARTESIAN_POINT ( 'NONE',  ( -4.401450347368204064, 115.6909491485452719, -1.538494961457526955 ) ) ;
#32566=CARTESIAN_POINT ( 'NONE',  ( 8.425593340951261112, 119.6232722969281355, -1.082523533391888115 ) ) ;
#32567=CARTESIAN_POINT ( 'NONE',  ( -5.263686092533428784, 116.7134249176580028, -1.019678336081760506 ) ) ;
#32568=CARTESIAN_POINT ( 'NONE',  ( 4.674394623628864487, 117.8377812495729273, 1.036795958576792076 ) ) ;
#32571=CARTESIAN_POINT ( 'NONE',  ( -5.862724111891735923, 121.1554468101848130, -0.6631653705238500507 ) ) ;
#32572=CARTESIAN_POINT ( 'NONE',  ( -3.385571042293893385, 115.7029692422994174, -1.641253599935611041 ) ) ;
#32575=CARTESIAN_POINT ( 'NONE',  ( 3.089687104934370598, 107.8271213589905386, -4.353618003723240371 ) ) ;
#32576=CARTESIAN_POINT ( 'NONE',  ( -1.432854634133492899, 120.0849730816093910, -0.5085234606245936373 ) ) ;
#32577=DIRECTION ( 'NONE',  ( -4.017660918040594346E-17, 1.000000000000000000, 2.376309959284834438E-19 ) ) ;
#32578=DIRECTION ( 'NONE',  ( -0.9998004120163608288, -5.205824365704082573E-17, -0.01997839162482760098 ) ) ;
#32580=CARTESIAN_POINT ( 'NONE',  ( -9.049360525155641710, 124.1535258118840517, -0.09135200362803799767 ) ) ;
#32581=CARTESIAN_POINT ( 'NONE',  ( -2.395914033174281865, 1.367755174955888275, -3.957843245732672877 ) ) ;
#32582=CARTESIAN_POINT ( 'NONE',  ( -0.004913308686096432183, 116.7872217978203224, 0.2458820580207659867 ) ) ;
#32583=VERTEX_POINT ( 'NONE', #39146 ) ;
#32584=LINE ( 'NONE', #19784, #9055 ) ;
#32585=CARTESIAN_POINT ( 'NONE',  ( 3.745939827176673731, -15.15858284179406823, -0.4807645327530354340 ) ) ;
#32586=CARTESIAN_POINT ( 'NONE',  ( -1.305241956589776819, 119.0230276286704054, 0.6306560096549496119 ) ) ;
#32587=CARTESIAN_POINT ( 'NONE',  ( -0.8250140797137134330, 8.550980984719981137, 0.5181985368706800710 ) ) ;
#32588=CARTESIAN_POINT ( 'NONE',  ( -20.48075987368149598, 152.5656283612522657, -1.113479615819600310 ) ) ;
#32589=CARTESIAN_POINT ( 'NONE',  ( 0.1867991717342751268, 10.66319190514178139, -0.9583599856553294272 ) ) ;
#32590=EDGE_CURVE ( 'NONE', #10724, #37473, #17707, .T. ) ;
#32594=CARTESIAN_POINT ( 'NONE',  ( 0.5964146925940678745, 106.0274289318137306, 5.278528196272315398 ) ) ;
#32596=CARTESIAN_POINT ( 'NONE',  ( -2.706440023329564681, 120.6505882111413683, 0.2907491850344329221 ) ) ;
#32597=CARTESIAN_POINT ( 'NONE',  ( 3.910559219094527528, -13.09373064504072737, 2.776858670901594994 ) ) ;
#32598=CARTESIAN_POINT ( 'NONE',  ( 17.79400844405170190, 146.5573550606970628, -1.533700293046251772 ) ) ;
#32599=CARTESIAN_POINT ( 'NONE',  ( -0.4560022058369030962, 118.7114656741295988, -0.6168833707790646326 ) ) ;
#32601=B_SPLINE_CURVE_WITH_KNOTS ( 'NONE', 3,
 ( #19431, #19850, #32648, #3910, #504, #6458 ),
 .UNSPECIFIED., .F., .F.,
 ( 4, 2, 4 ),
 ( 0.000000000000000000, 0.5000000000000000000, 1.000000000000000000 ),
 .UNSPECIFIED. ) ;
#32602=CARTESIAN_POINT ( 'NONE',  ( 2.827333099181600584, -13.37427733298611443, 0.6166582517569209054 ) ) ;
#32603=CARTESIAN_POINT ( 'NONE',  ( -0.1059412245877799363, 38.28537051638084421, -0.7326154344855524414 ) ) ;
#32604=CARTESIAN_POINT ( 'NONE',  ( 9.310784039460415329, 124.2035065715909496, -0.04725383350292533535 ) ) ;
#32607=CARTESIAN_POINT ( 'NONE',  ( 0.4669423002395221012, 105.9272292791236794, 5.319618862452587749 ) ) ;
#32608=VECTOR ( 'NONE', #8959, 1000.000000000000227 ) ;
#32614=CARTESIAN_POINT ( 'NONE',  ( 3.728135546147748336, 116.6403000632267464, -0.003128093132697572741 ) ) ;
#32615=CARTESIAN_POINT ( 'NONE',  ( -7.140971181236958287, 122.4194348751405101, -0.03314210641492758291 ) ) ;
#32616=CARTESIAN_POINT ( 'NONE',  ( -2.857476489931835673, 115.6909491485452577, 1.572699180235668903 ) ) ;
#32618=CARTESIAN_POINT ( 'NONE',  ( 0.5226899456406054467, 39.20946620154573026, -1.259808938293395908 ) ) ;
#32619=EDGE_CURVE ( 'NONE', #12162, #34968, #21087, .T. ) ;
#32620=CARTESIAN_POINT ( 'NONE',  ( 9.041969115052715722, 119.3941581119689204, 1.378656440977003461 ) ) ;
#32621=CARTESIAN_POINT ( 'NONE',  ( -2.131885088311801901, 26.04095958170969638, -4.099730575217565232 ) ) ;
#32622=CARTESIAN_POINT ( 'NONE',  ( 4.580344459542567748, 28.35322510196829171, -7.077419036913218164 ) ) ;
#32623=CARTESIAN_POINT ( 'NONE',  ( -5.477710374292670714, 117.3472291391384061, -0.8783748813296128333 ) ) ;
#32624=CARTESIAN_POINT ( 'NONE',  ( -1.846946891755202769, 121.3688471916803451, -0.3635544463458705300 ) ) ;
#32627=CARTESIAN_POINT ( 'NONE',  ( -2.044950736525416701, 104.6144662015456674, 4.372199481676336319 ) ) ;
#32628=CARTESIAN_POINT ( 'NONE',  ( 2.488009491785908800, 18.85968022696138391, -3.895047602898422223 ) ) ;
#32630=CARTESIAN_POINT ( 'NONE',  ( -22.76738278397264281, 137.3906169244638136, -0.4549464913834382340 ) ) ;
#32631=CARTESIAN_POINT ( 'NONE',  ( 3.219973314159829680, -14.13069947154231620, 2.606357176882864390 ) ) ;
#32632=CARTESIAN_POINT ( 'NONE',  ( 1.918777129854390084, 121.7602717223048501, -0.2400857948923554031 ) ) ;
#32633=CARTESIAN_POINT ( 'NONE',  ( -16.59152294496572111, 155.2525159475892167, 0.4418349252515508807 ) ) ;
#32638=ORIENTED_EDGE ( 'NONE', *, *, #34765, .F. ) ;
#32640=CARTESIAN_POINT ( 'NONE',  ( 5.890162669548780094, -14.87046963210582362, 1.285284309844398898 ) ) ;
#32641=CARTESIAN_POINT ( 'NONE',  ( -3.207104841129888584, 118.4902560533893592, 0.7629184910595989688 ) ) ;
#32642=CARTESIAN_POINT ( 'NONE',  ( 20.51279501983843545, 150.9797539340098069, -1.282250019969887855 ) ) ;
#32643=CARTESIAN_POINT ( 'NONE',  ( 4.440015753948663324, -2.305524871907271400, 1.325333094644747245 ) ) ;
#32645=ORIENTED_EDGE ( 'NONE', *, *, #21628, .F. ) ;
#32647=CARTESIAN_POINT ( 'NONE',  ( 0.1292312685652868276, 109.4728569552520554, 3.923176234211466440 ) ) ;
#32648=CARTESIAN_POINT ( 'NONE',  ( 4.934253595602364761, 117.4065730964002228, 1.087905710704323736 ) ) ;
#32649=CARTESIAN_POINT ( 'NONE',  ( -3.531217591821389501, 156.5024071230465097, 1.273243333543746303 ) ) ;
#32650=CARTESIAN_POINT ( 'NONE',  ( 5.152406760161801991, 116.8381519984425125, 0.1413306424610384082 ) ) ;
#32652=( BOUNDED_SURFACE ( )  B_SPLINE_SURFACE ( 3, 2, ( 
 ( #24072, #7901, #40077 ),
 ( #14267, #14684, #27691 ),
 ( #40699, #27278, #20236 ),
 ( #23426, #37084, #4720 ) ),
 .UNSPECIFIED., .F., .F., .F. ) 
 B_SPLINE_SURFACE_WITH_KNOTS ( ( 4, 4 ),
 ( 3, 3 ),
 ( -1.125575372986152065E-06, 0.0001887214708706781534 ),
 ( 0.000000000000000000, 0.2790336440021598530 ),
 .UNSPECIFIED. ) 
 GEOMETRIC_REPRESENTATION_ITEM ( )  RATIONAL_B_SPLINE_SURFACE ( (
 ( 1.000000000000000000, 0.9331452035001246426, 0.9035998819730153286),
 ( 1.000000000000000000, 0.9331452033132299206, 0.9035998817035257868),
 ( 1.000000000000000000, 0.9331453013021652199, 0.9036000229969769482),
 ( 1.000000000000000000, 0.9331453801652662694, 0.9036001367122621364) ) ) 
 REPRESENTATION_ITEM ( '' )  SURFACE ( )  );
#32653=CARTESIAN_POINT ( 'NONE',  ( 11.63135762381485883, 122.7176759045101022, -1.263630383496116005 ) ) ;
#32654=CARTESIAN_POINT ( 'NONE',  ( -12.77966252534845992, 121.3369795956499928, -1.646308105693409685 ) ) ;
#32657=ORIENTED_EDGE ( 'NONE', *, *, #18885, .F. ) ;
#32658=CARTESIAN_POINT ( 'NONE',  ( 4.601481835261479247, 118.0766341700411601, -0.5257344758955123654 ) ) ;
#32659=CARTESIAN_POINT ( 'NONE',  ( 10.29759560803357488, 124.8461398015159745, -0.5204633524205694028 ) ) ;
#32660=ORIENTED_EDGE ( 'NONE', *, *, #21163, .F. ) ;
#32661=CARTESIAN_POINT ( 'NONE',  ( -17.73735868213794475, 147.0764175921665640, -2.241444305069557164 ) ) ;
#32662=CARTESIAN_POINT ( 'NONE',  ( 3.116032494879745762, -15.28226460877120374, 3.911124699519683556 ) ) ;
#32663=CARTESIAN_POINT ( 'NONE',  ( -4.243821914726944478, 105.1218540727933686, -3.250214477582284989 ) ) ;
#32667=CARTESIAN_POINT ( 'NONE',  ( -4.881639387764474591, 117.7524908745723593, 0.7530060852826706563 ) ) ;
#32668=CARTESIAN_POINT ( 'NONE',  ( 16.41634355132952194, 139.9843038322558186, 2.146987391100668940 ) ) ;
#32669=CARTESIAN_POINT ( 'NONE',  ( -3.113414239748028223, 30.98679946927233431, 0.04088859964249486750 ) ) ;
#32670=CARTESIAN_POINT ( 'NONE',  ( -0.3239230800893593276, 29.42979164457532804, -4.628216972995994993 ) ) ;
#32671=CARTESIAN_POINT ( 'NONE',  ( 15.78659908162999947, 146.5797798787131399, 0.5456203974801299150 ) ) ;
#32675=CARTESIAN_POINT ( 'NONE',  ( -5.557118726059879776, 116.7202209307960459, -0.2768648844130547904 ) ) ;
#32676=CARTESIAN_POINT ( 'NONE',  ( -5.586884702347495235, 72.99146620154573384, -0.1116392523995361763 ) ) ;
#32678=PLANE ( 'NONE',  #5039 ) ;
#32680=DIRECTION ( 'NONE',  ( -4.017660918040594346E-17, 1.000000000000000000, 2.376309959284834438E-19 ) ) ;
#32685=CARTESIAN_POINT ( 'NONE',  ( -2.803048170062614641, 116.6385632091030544, 0.1397181956995451058 ) ) ;
#32687=ORIENTED_EDGE ( 'NONE', *, *, #38382, .F. ) ;
#32689=CARTESIAN_POINT ( 'NONE',  ( 6.978044078171404152, 121.9510782527418371, 0.05806353974079936364 ) ) ;
#32691=CARTESIAN_POINT ( 'NONE',  ( 3.960807457435879364, 115.7035851291592934, -1.436426024118471867 ) ) ;
#32692=CIRCLE ( 'NONE', #17712, 3.683000000000001162 ) ;
#32693=CARTESIAN_POINT ( 'NONE',  ( -5.939593986634166711, 121.5467800236367424, -0.1471147542197154823 ) ) ;
#32694=CARTESIAN_POINT ( 'NONE',  ( 5.943076596790061394, -13.74187730036333122, 2.284392803971454278 ) ) ;
#32695=CARTESIAN_POINT ( 'NONE',  ( -18.85079593648351803, 152.0234722879370111, 1.474728064877437239 ) ) ;
#32697=CARTESIAN_POINT ( 'NONE',  ( 5.710605682675650385, 159.1232349745254453, 0.3332304182141802573 ) ) ;
#32698=CARTESIAN_POINT ( 'NONE',  ( 2.062287441005058675, -15.63671396113243439, 5.843295106519123649 ) ) ;
#32699=CARTESIAN_POINT ( 'NONE',  ( 5.252108655715503005, 115.6909491485453145, -0.9240985664890069007 ) ) ;
#32700=CARTESIAN_POINT ( 'NONE',  ( -0.4650136207426652235, -7.476398416381191403, -0.8572754866018892361 ) ) ;
#32701=CARTESIAN_POINT ( 'NONE',  ( -22.69169950426951132, 137.3157656003441787, -0.5971823736698285146 ) ) ;
#32704=VERTEX_POINT ( 'NONE', #26033 ) ;
#32705=CARTESIAN_POINT ( 'NONE',  ( -5.560072573240018912, 117.2208093686857922, 0.5507231274924011544 ) ) ;
#32707=CARTESIAN_POINT ( 'NONE',  ( -17.87798177106725817, 144.5560955566678558, 1.636306359874434291 ) ) ;
#32709=CARTESIAN_POINT ( 'NONE',  ( 18.99721151120893126, 152.1029585079319020, 2.158688780372492566 ) ) ;
#32710=CARTESIAN_POINT ( 'NONE',  ( 19.78762832257843129, 149.1964539096042870, -1.700649111281397508 ) ) ;
#32711=CARTESIAN_POINT ( 'NONE',  ( 0.2491751845298053603, 0.8914985761586250446, 0.9476022430964140542 ) ) ;
#32712=CARTESIAN_POINT ( 'NONE',  ( -19.40029886644223467, 131.9512773411433670, -1.949052778313793866 ) ) ;
#32713=CARTESIAN_POINT ( 'NONE',  ( 4.865035472571053177, 117.7603446447191260, -0.7858820013116090131 ) ) ;
#32716=CARTESIAN_POINT ( 'NONE',  ( 5.771537640388776147, 118.4310156723767307, 0.6642225483502961492 ) ) ;
#32717=EDGE_CURVE ( 'NONE', #7084, #36618, #29448, .T. ) ;
#32718=CARTESIAN_POINT ( 'NONE',  ( 0.5800011805206757298, 120.2131932824006526, -0.3882866552237519420 ) ) ;
#32719=CARTESIAN_POINT ( 'NONE',  ( -10.21313493804737682, 125.9885856776569426, -0.1666469060040937644 ) ) ;
#32721=CARTESIAN_POINT ( 'NONE',  ( -0.9182646862280283706, 157.4778559999684830, -1.599919928990592988 ) ) ;
#32722=CARTESIAN_POINT ( 'NONE',  ( 4.515093156845158440, -15.50826969562475810, 4.181389551362865831 ) ) ;
#32728=CARTESIAN_POINT ( 'NONE',  ( 17.13831219182123888, 149.7102054596878702, 2.353104315458284468 ) ) ;
#32729=CARTESIAN_POINT ( 'NONE',  ( -6.585902005698190595E-14, 91.53346620154573543, 1.207165459464729879E-19 ) ) ;
#32730=AXIS2_PLACEMENT_3D ( 'NONE', #31085, #1924, #38329 ) ;
#32731=CARTESIAN_POINT ( 'NONE',  ( 0.8838529761740171464, 116.4325158421065680, 0.01766148591713753366 ) ) ;
#32732=CARTESIAN_POINT ( 'NONE',  ( -3.306315723242934990, 118.9685052735122355, 0.5531158949559313864 ) ) ;
#32733=CARTESIAN_POINT ( 'NONE',  ( -8.431077252155047219, 22.10977948022283357, 0.3997009428958171462 ) ) ;
#32734=CARTESIAN_POINT ( 'NONE',  ( 5.218277051435741498, 121.1607713875043117, 0.4468594773273021903 ) ) ;
#32735=CARTESIAN_POINT ( 'NONE',  ( 14.99285373232496532, 120.9606250904355704, -0.4613734978017340338 ) ) ;
#32737=DIRECTION ( 'NONE',  ( -4.017660918040594346E-17, 1.000000000000000000, 2.376309959284834438E-19 ) ) ;
#32738=CARTESIAN_POINT ( 'NONE',  ( -1.421877081889727945, 159.6054662015457666, -0.01472409299311845318 ) ) ;
#32739=ORIENTED_EDGE ( 'NONE', *, *, #1932, .F. ) ;
#32740=CARTESIAN_POINT ( 'NONE',  ( 5.171081541123786707, 120.2810485551120223, -0.6437068486157979663 ) ) ;
#32741=CARTESIAN_POINT ( 'NONE',  ( 2.467290606313818913, -15.47138089097717106, 5.855268220497546139 ) ) ;
#32742=CARTESIAN_POINT ( 'NONE',  ( -11.59282501421117750, 128.2970750771678752, -0.8590849294959498339 ) ) ;
#32743=CARTESIAN_POINT ( 'NONE',  ( 1.975269416564901404, -15.10067923695700109, 5.832845082603779652 ) ) ;
#32746=CARTESIAN_POINT ( 'NONE',  ( 21.64466742782788700, 132.7051459832101443, 0.4972030839502444288 ) ) ;
#32747=ORIENTED_EDGE ( 'NONE', *, *, #6581, .F. ) ;
#32748=CARTESIAN_POINT ( 'NONE',  ( -3.812863311134618183, 2.017465188139291765, -2.614655560905410958 ) ) ;
#32749=CARTESIAN_POINT ( 'NONE',  ( -13.70496720262328161, 119.6480011847128253, -0.2738578607176475055 ) ) ;
#32750=CARTESIAN_POINT ( 'NONE',  ( -6.606344270946872901E-14, 95.34346620154573770, 1.014423412895214384E-29 ) ) ;
#32751=CARTESIAN_POINT ( 'NONE',  ( 5.030795403078426098, 113.7219408396588562, 1.867219066840775987 ) ) ;
#32752=CARTESIAN_POINT ( 'NONE',  ( 6.087437787857826521, 121.3262240766859890, 0.5122669965167206962 ) ) ;
#32753=CARTESIAN_POINT ( 'NONE',  ( 0.7003524534433175353, 11.14785949628657669, 4.567531960304466843 ) ) ;
#32754=CARTESIAN_POINT ( 'NONE',  ( 22.43644356963070763, 149.3130771379323392, 1.752678757896036776 ) ) ;
#32755=CARTESIAN_POINT ( 'NONE',  ( 15.52687642492882070, 147.5330934759543879, 0.3102639428822866474 ) ) ;
#32757=CARTESIAN_POINT ( 'NONE',  ( 16.68922378205029489, 153.6190162071354735, -1.533137601955099294 ) ) ;
#32758=CIRCLE ( 'NONE', #23891, 0.5080000000000002292 ) ;
#32759=CARTESIAN_POINT ( 'NONE',  ( 1.368391094521330897, 11.37271669962338372, 4.434453701053673313 ) ) ;
#32760=CARTESIAN_POINT ( 'NONE',  ( -14.69808362324415363, 120.8948172685174001, -1.121060376578428386 ) ) ;
#32762=CARTESIAN_POINT ( 'NONE',  ( -14.35733687469677200, 139.0340687859245463, 0.1707862337897579352 ) ) ;
#32763=CARTESIAN_POINT ( 'NONE',  ( 3.397480601066255712, -15.04020002808364964, 5.521695076403254632 ) ) ;
#32764=CIRCLE ( 'NONE', #2859, 0.5080000000000002292 ) ;
#32765=CARTESIAN_POINT ( 'NONE',  ( -6.654617103318593247E-14, 104.6144662015457243, 1.534725424433578570E-31 ) ) ;
#32766=CARTESIAN_POINT ( 'NONE',  ( 4.999324130125957666, 117.3993846056547738, 0.8255830379890115589 ) ) ;
#32767=VERTEX_POINT ( 'NONE', #16226 ) ;
#32768=CARTESIAN_POINT ( 'NONE',  ( 15.19444909298863777, 153.0676604005411434, 2.356382943223728876 ) ) ;
#32769=DIRECTION ( 'NONE',  ( -4.017660918040594346E-17, 1.000000000000000000, 2.376309959284834438E-19 ) ) ;
#32770=DIRECTION ( 'NONE',  ( -0.9998004120163610509, -4.016384292689131511E-17, -0.01997839162482749689 ) ) ;
#32773=CARTESIAN_POINT ( 'NONE',  ( -21.45272375726306180, 151.3201912522522719, 0.6338752469853824456 ) ) ;
#32774=CARTESIAN_POINT ( 'NONE',  ( 3.006797519324799772, 15.24566924451032435, -7.865828698519952589 ) ) ;
#32776=CARTESIAN_POINT ( 'NONE',  ( 0.3220477894874517188, 116.6413645472259617, -0.1880332438949531837 ) ) ;
#32778=CARTESIAN_POINT ( 'NONE',  ( -5.036351857865265735, 117.3993844875897139, 0.5494637324817667201 ) ) ;
#32780=CARTESIAN_POINT ( 'NONE',  ( -4.937359598886440715, 117.4097706984612302, -1.081953738475849747 ) ) ;
#32783=CARTESIAN_POINT ( 'NONE',  ( -4.463408765292727232, 118.1258133513832860, 0.5547340330597864133 ) ) ;
#32785=ORIENTED_EDGE ( 'NONE', *, *, #12223, .T. ) ;
#32786=VERTEX_POINT ( 'NONE', #29233 ) ;
#32788=CARTESIAN_POINT ( 'NONE',  ( -6.069717446804125949, 119.4746383518879043, -1.260100842361058016 ) ) ;
#32789=CARTESIAN_POINT ( 'NONE',  ( -5.192700560041021873, 116.2637919873444190, -1.171650394069924772 ) ) ;
#32790=CARTESIAN_POINT ( 'NONE',  ( 4.556952415498273901, 118.0383946930539878, 0.8497061536611607568 ) ) ;
#32792=CARTESIAN_POINT ( 'NONE',  ( -16.47979853205677969, 146.5532241433796230, -1.607449420861547740 ) ) ;
#32793=CARTESIAN_POINT ( 'NONE',  ( -4.532044145959075010, 115.7029491485453718, -1.515528964257317757 ) ) ;
#32795=CARTESIAN_POINT ( 'NONE',  ( 4.812383263389150123, 112.7966860322829206, -2.369499567760593450 ) ) ;
#32796=CARTESIAN_POINT ( 'NONE',  ( -14.71707226966683812, 150.5114039713088516, -1.846696807168831000 ) ) ;
#32798=CARTESIAN_POINT ( 'NONE',  ( -6.431420355030265265E-14, 156.3034662015457172, 9.897580308537652682E-17 ) ) ;
#32799=CARTESIAN_POINT ( 'NONE',  ( 7.810699835753124098, 122.5400548747105915, -0.1271298699639721308 ) ) ;
#32800=CARTESIAN_POINT ( 'NONE',  ( -10.10118861072700192, 125.9371159002616309, -0.1041072054866566399 ) ) ;
#32801=CARTESIAN_POINT ( 'NONE',  ( -4.476207883417873568, -7.053342675672244155, -1.178223045331058705 ) ) ;
#32802=CARTESIAN_POINT ( 'NONE',  ( 19.79238143276385031, 128.7876384977266468, 1.131474956103616814 ) ) ;
#32804=CARTESIAN_POINT ( 'NONE',  ( 3.866492242221801767, -15.24987600803320831, 0.6064936129020901401 ) ) ;
#32805=CARTESIAN_POINT ( 'NONE',  ( -10.43940122747819466, 155.6679353847891321, 1.745147575944303364 ) ) ;
#32806=CARTESIAN_POINT ( 'NONE',  ( -0.8880852245287531588, 7.049514723814470862, -0.3999422104893632923 ) ) ;
#32807=CARTESIAN_POINT ( 'NONE',  ( -22.89058624538214204, 149.8162411397050278, -1.183733681586530917 ) ) ;
#32809=CARTESIAN_POINT ( 'NONE',  ( 0.7511875256325919459, -11.68598654017788974, 0.6195722450943603743 ) ) ;
#32813=CARTESIAN_POINT ( 'NONE',  ( 0.1274156416094324173, 105.9117620634264370, 5.326488824310051662 ) ) ;
#32815=CARTESIAN_POINT ( 'NONE',  ( -1.739825554503067861, 156.3676537730497387, 0.7044751146431476041 ) ) ;
#32816=CARTESIAN_POINT ( 'NONE',  ( 4.249299001760414640, -12.92553893317818847, 2.698699680779739207 ) ) ;
#32817=CARTESIAN_POINT ( 'NONE',  ( 15.43236126668700159, 134.8939017613128328, -1.443262610673740953 ) ) ;
#32818=CARTESIAN_POINT ( 'NONE',  ( -8.740007204533959850, 120.0394951565550343, -1.484413609726634942 ) ) ;
#32820=CARTESIAN_POINT ( 'NONE',  ( 3.026662605148213725, -13.87242449132548217, 1.205013440933411228 ) ) ;
#32821=CARTESIAN_POINT ( 'NONE',  ( -4.432242455686237648, 32.76553509196318004, 1.287969469385143784 ) ) ;
#32822=CARTESIAN_POINT ( 'NONE',  ( 0.6587526420362558310, 156.3106852680424765, -0.1744449402554845152 ) ) ;
#32824=EDGE_LOOP ( 'NONE', ( #9631, #17587 ) ) ;
#32825=CARTESIAN_POINT ( 'NONE',  ( -4.163217485963554232, 111.0900967538983650, 3.043985244824447101 ) ) ;
#32829=CARTESIAN_POINT ( 'NONE',  ( 20.42271720105680188, 129.0384130229076334, 0.2828206407990420113 ) ) ;
#32830=CARTESIAN_POINT ( 'NONE',  ( -6.920469006312010229, 121.8192184429722005, 0.01800753507563507619 ) ) ;
#32832=CARTESIAN_POINT ( 'NONE',  ( -1.648859552577025323, 115.6909491485452577, 1.667642768541721887 ) ) ;
#32834=CARTESIAN_POINT ( 'NONE',  ( 2.511959498749158470, 39.20946620154573026, -1.220058598423863661 ) ) ;
#32835=CARTESIAN_POINT ( 'NONE',  ( 18.59893286765435505, 151.9584835496716266, 2.273025404440325303 ) ) ;
#32836=CARTESIAN_POINT ( 'NONE',  ( 3.087053954869741101, 14.59627045569285286, -3.440871586639639990 ) ) ;
#32837=CARTESIAN_POINT ( 'NONE',  ( 0.01634572621781915994, 29.22912819268679030, -8.429653881604959764 ) ) ;
#32838=CARTESIAN_POINT ( 'NONE',  ( 2.187205382360373651, 116.7606846954971331, -0.4172344709117405959 ) ) ;
#32839=CARTESIAN_POINT ( 'NONE',  ( -3.156357112953910082, 123.6198120039584154, -0.1457842492014823077 ) ) ;
#32842=CARTESIAN_POINT ( 'NONE',  ( 3.196719817593447033, 104.6144662015522329, 4.273492549843798116 ) ) ;
#32843=CARTESIAN_POINT ( 'NONE',  ( -1.756104463947763206, 14.33678105357426702, 4.288642365192034234 ) ) ;
#32844=DIRECTION ( 'NONE',  ( -4.017660918040594346E-17, 1.000000000000000000, 2.376309959284832031E-19 ) ) ;
#32846=CARTESIAN_POINT ( 'NONE',  ( 2.715444768400132158, -14.72438443971033095, 4.720152092698882029 ) ) ;
#32847=CARTESIAN_POINT ( 'NONE',  ( 1.135428393696602312, 110.6314368487224300, -3.415474402745806159 ) ) ;
#32848=CARTESIAN_POINT ( 'NONE',  ( -22.82237111512532124, 142.4248215231809240, 0.5244786342524968559 ) ) ;
#32852=CARTESIAN_POINT ( 'NONE',  ( 5.035933200060415338, 117.3993844219003648, -0.5513780243448201945 ) ) ;
#32855=CARTESIAN_POINT ( 'NONE',  ( 5.215289103204772125, -15.32183344268082870, 2.967178555186370303 ) ) ;
#32856=CARTESIAN_POINT ( 'NONE',  ( -6.760483308329498620, 119.1290971219625021, 1.000752511853993054 ) ) ;
#32857=CARTESIAN_POINT ( 'NONE',  ( 13.46300103848306406, 120.9245410081625209, -0.9131080906212012405 ) ) ;
#32858=CARTESIAN_POINT ( 'NONE',  ( -2.424025297795170619, -5.104216246930970868, 3.935102955759355758 ) ) ;
#32861=VERTEX_POINT ( 'NONE', #6668 ) ;
#32863=CARTESIAN_POINT ( 'NONE',  ( 0.7402556297410838315, 119.5055576915191580, 0.7321893670752779304 ) ) ;
#32864=CARTESIAN_POINT ( 'NONE',  ( -4.737627528408766331, 117.7521883752312419, 0.9000133201668191196 ) ) ;
#32865=CARTESIAN_POINT ( 'NONE',  ( -0.5698427240851328124, 120.0661220204379305, 0.4260729765348977294 ) ) ;
#32866=CARTESIAN_POINT ( 'NONE',  ( -4.757346424997288103, 117.3993836135861386, -1.207075064218979810 ) ) ;
#32867=CARTESIAN_POINT ( 'NONE',  ( 16.81178602683893075, 135.2943057719725459, -1.678525023343173439 ) ) ;
#32868=CARTESIAN_POINT ( 'NONE',  ( -16.61465421735670844, 153.6190162071354735, -2.198628343207905900 ) ) ;
#32870=AXIS2_PLACEMENT_3D ( 'NONE', #36214, #20206, #6605 ) ;
#32872=CARTESIAN_POINT ( 'NONE',  ( 4.361691748181014461, 118.1815233605024957, -0.4501171095398698863 ) ) ;
#32873=EDGE_CURVE ( 'NONE', #5804, #28106, #30724, .T. ) ;
#32874=CARTESIAN_POINT ( 'NONE',  ( 9.326662024493369785, 153.8845013697122965, -0.4488502173044092158 ) ) ;
#32875=ORIENTED_EDGE ( 'NONE', *, *, #35448, .T. ) ;
#32876=CARTESIAN_POINT ( 'NONE',  ( -15.64494829320037894, 134.9797526104055123, -2.135645317121837472 ) ) ;
#32877=CARTESIAN_POINT ( 'NONE',  ( 2.816406720412386822, -15.24816796146632925, 4.372395393210481984 ) ) ;
#32878=CARTESIAN_POINT ( 'NONE',  ( -5.326136116496724249, 105.1224662015457341, -0.4468285755459980302 ) ) ;
#32879=VECTOR ( 'NONE', #26328, 1000.000000000000114 ) ;
#32880=CARTESIAN_POINT ( 'NONE',  ( 0.02983097946976470335, 117.3993836135854707, -1.492864285907033572 ) ) ;
#32881=CARTESIAN_POINT ( 'NONE',  ( -4.255528399684056495, 7.899375212487111497, -1.818898740287305138 ) ) ;
#32882=CARTESIAN_POINT ( 'NONE',  ( 13.40752216115192752, 152.3772590505219569, 2.011877943007317704 ) ) ;
#32883=CARTESIAN_POINT ( 'NONE',  ( -2.651076796310585237, 29.59993426230072089, 0.1800044463941182782 ) ) ;
#32884=CARTESIAN_POINT ( 'NONE',  ( 3.121479725567877228, 16.06095178295013071, 3.416230322513892137 ) ) ;
#32885=CARTESIAN_POINT ( 'NONE',  ( 7.046279781204515480, 122.0586610246435129, 0.2738582164285300879 ) ) ;
#32889=CARTESIAN_POINT ( 'NONE',  ( 2.182332163935870817, 116.1897970688993809, 0.04360819029724687795 ) ) ;
#32893=DIRECTION ( 'NONE',  ( 0.9998004120163608288, 0.000000000000000000, 0.01997839162482736852 ) ) ;
#32896=CARTESIAN_POINT ( 'NONE',  ( -4.074955089416341991, 118.2429491485453354, 0.1454234154749719787 ) ) ;
#32900=CARTESIAN_POINT ( 'NONE',  ( -11.66036501707591810, 118.7334002725740874, -0.02296568806519961800 ) ) ;
#32901=AXIS2_PLACEMENT_3D ( 'NONE', #38057, #40427, #1864 ) ;
#32904=CARTESIAN_POINT ( 'NONE',  ( -7.787433790559666669, 122.6039481253381922, -0.2654969604323166865 ) ) ;
#32905=ORIENTED_EDGE ( 'NONE', *, *, #18826, .F. ) ;
#32907=CARTESIAN_POINT ( 'NONE',  ( -10.21163942101063249, 125.9885856776569426, -0.2414886939513457842 ) ) ;
#32908=CARTESIAN_POINT ( 'NONE',  ( 5.879588643049518559, -13.10657381646278274, 1.873965859954596969 ) ) ;
#32909=CARTESIAN_POINT ( 'NONE',  ( -6.823161219633312236, 118.5360090424673274, 0.8871979454111539320 ) ) ;
#32910=CARTESIAN_POINT ( 'NONE',  ( 1.893578447776079754, 19.08455809737888487, -4.224370802633358402 ) ) ;
#32912=CARTESIAN_POINT ( 'NONE',  ( 0.9351853929027724721, 116.6346273530297850, 0.2267945756083742659 ) ) ;
#32913=CARTESIAN_POINT ( 'NONE',  ( 10.05542837570307668, 125.9185204131281210, 0.3475070621306587948 ) ) ;
#32915=CARTESIAN_POINT ( 'NONE',  ( -0.4068859638909740339, 2.017459551269393359, -0.8868740919469698669 ) ) ;
#32916=CARTESIAN_POINT ( 'NONE',  ( -2.764936593379252017, 116.5678055239024644, -0.1631480333911171920 ) ) ;
#32920=CARTESIAN_POINT ( 'NONE',  ( 5.552057423463700125, 116.7478124476613743, 0.3280336575071842176 ) ) ;
#32921=ORIENTED_EDGE ( 'NONE', *, *, #34488, .T. ) ;
#32922=CARTESIAN_POINT ( 'NONE',  ( -8.280704432558593453, 121.1361926620737393, 1.000371422393417697 ) ) ;
#32924=CARTESIAN_POINT ( 'NONE',  ( 14.04349332752973467, 121.9525460547650226, 1.645664411013196604 ) ) ;
#32925=CARTESIAN_POINT ( 'NONE',  ( 0.4802819474807752398, 118.7114656741295988, -0.5981741851633314289 ) ) ;
#32927=CARTESIAN_POINT ( 'NONE',  ( 0.05045227420522335748, 0.5774631391966889016, 0.9751023907654918776 ) ) ;
#32928=CARTESIAN_POINT ( 'NONE',  ( -7.956670401304606344, 118.4344479264803169, -1.111586840565143675 ) ) ;
#32929=CARTESIAN_POINT ( 'NONE',  ( 4.665372465336868224, 118.0265698473236711, -0.5749007169697829545 ) ) ;
#32930=CARTESIAN_POINT ( 'NONE',  ( 5.190622930436333604, 104.6144662015347535, 1.277265713775895151 ) ) ;
#32931=CARTESIAN_POINT ( 'NONE',  ( 11.98504388954655120, 126.0992317015783328, -1.027991910846089985 ) ) ;
#32932=CARTESIAN_POINT ( 'NONE',  ( -8.487687333566288572, 123.3253871723413368, -0.1696041924978711202 ) ) ;
#32934=CARTESIAN_POINT ( 'NONE',  ( -8.000928410381925815, 156.3870133935118076, -2.044342179695390893 ) ) ;
#32935=CARTESIAN_POINT ( 'NONE',  ( 4.689621780486535663, -15.62538141832135707, 3.172200491054990579 ) ) ;
#32938=CARTESIAN_POINT ( 'NONE',  ( -4.503792796599852544, 118.0666417019298109, -0.8213613892662697813 ) ) ;
#32940=EDGE_CURVE ( 'NONE', #3642, #21134, #6845, .T. ) ;
#32941=CARTESIAN_POINT ( 'NONE',  ( 4.147465018942456894, 118.2392518931096532, 0.3974363740737554274 ) ) ;
#32942=CARTESIAN_POINT ( 'NONE',  ( 11.77984014550159841, 123.3160021321619695, 1.727726820665321350 ) ) ;
#32945=CARTESIAN_POINT ( 'NONE',  ( 13.43845804798103316, 156.9141898299356512, 0.2685323735513602261 ) ) ;
#32947=CARTESIAN_POINT ( 'NONE',  ( -3.689824518792605978, 110.1236525333376619, 3.433021159709686909 ) ) ;
#32948=CARTESIAN_POINT ( 'NONE',  ( -4.443900581410109574, 30.07671411637534931, -7.177485988639727310 ) ) ;
#32949=CARTESIAN_POINT ( 'NONE',  ( 10.03827118703578059, 124.8772485319846055, 0.7459150106818386305 ) ) ;
#32950=CARTESIAN_POINT ( 'NONE',  ( 1.363555988950266862, 159.4956652290339605, -0.6451735917158236688 ) ) ;
#32953=AXIS2_PLACEMENT_3D ( 'NONE', #190, #13163, #9961 ) ;
#32956=CARTESIAN_POINT ( 'NONE',  ( -23.21412382727114121, 149.6303025714371131, -0.4381719528662391117 ) ) ;
#32958=CARTESIAN_POINT ( 'NONE',  ( 5.238238559199842825, 120.3605920493329222, -0.6250241856820153430 ) ) ;
#32961=CARTESIAN_POINT ( 'NONE',  ( 0.006534791579796636780, 156.3267223255430167, -0.3270276925529294054 ) ) ;
#32962=CARTESIAN_POINT ( 'NONE',  ( 4.270589230953349968, -11.85684205577233818, 0.9542379244983925091 ) ) ;
#32963=ADVANCED_FACE ( 'NONE', ( #4951 ), #1334, .T. ) ;
#32964=CARTESIAN_POINT ( 'NONE',  ( -14.55736095115768514, 121.4416029531759591, 0.8377414905974124304 ) ) ;
#32965=CARTESIAN_POINT ( 'NONE',  ( -10.39928917620371784, 153.1223395828141918, -0.2078025466733117443 ) ) ;
#32966=CARTESIAN_POINT ( 'NONE',  ( 23.35646125964490949, 148.8716009884483071, 0.5438655406665986458 ) ) ;
#32967=ORIENTED_EDGE ( 'NONE', *, *, #20898, .T. ) ;
#32968=CARTESIAN_POINT ( 'NONE',  ( 4.440015753948663324, -2.305524871907271400, 1.325333094644747245 ) ) ;
#32969=CARTESIAN_POINT ( 'NONE',  ( -5.772319165918015749, 116.9338547871927858, -0.1153446742911716505 ) ) ;
#32971=CARTESIAN_POINT ( 'NONE',  ( -8.228564651236517591, 120.5845947550810422, 1.087621554438485738 ) ) ;
#32972=CARTESIAN_POINT ( 'NONE',  ( 4.615940417482057967, 3.801270455692812966, -0.2501868467277520436 ) ) ;
#32973=CARTESIAN_POINT ( 'NONE',  ( 14.30926610799415144, 121.2650221238243944, 1.406141635412307300 ) ) ;
#32976=CARTESIAN_POINT ( 'NONE',  ( 13.79335258734181124, 122.1113760975138263, -1.168436778447113689 ) ) ;
#32977=CARTESIAN_POINT ( 'NONE',  ( 3.019445949670579665, 11.99742794009110014, 3.522755186455234000 ) ) ;
#32978=CARTESIAN_POINT ( 'NONE',  ( -16.30933243092150420, 122.7783120765077030, -1.207982166786797151 ) ) ;
#32980=LINE ( 'NONE', #13370, #40237 ) ;
#32981=ORIENTED_EDGE ( 'NONE', *, *, #2971, .T. ) ;
#32982=CARTESIAN_POINT ( 'NONE',  ( -9.203139800278419713, 153.8854248570426080, 0.2095608753156675830 ) ) ;
#32983=CARTESIAN_POINT ( 'NONE',  ( 4.517131889307780312, -14.80175198191645336, 4.712020298053779754 ) ) ;
#32984=DIRECTION ( 'NONE',  ( -0.9998004120163608288, 0.000000000000000000, -0.01997839162482747608 ) ) ;
#32985=CARTESIAN_POINT ( 'NONE',  ( 2.829627719599027369, -13.65247383265987757, 0.5238048331051645690 ) ) ;
#32987=CARTESIAN_POINT ( 'NONE',  ( 19.49537437117577454, 147.7952244890416296, 2.518105945687704406 ) ) ;
#32988=DIRECTION ( 'NONE',  ( -4.017660918040594346E-17, 1.000000000000000000, 2.376309959284834438E-19 ) ) ;
#32990=CARTESIAN_POINT ( 'NONE',  ( -22.21083362159536634, 150.4821223471089411, 0.6270836034604139186 ) ) ;
#32991=CARTESIAN_POINT ( 'NONE',  ( 4.770677904581660300, 21.51973835935561041, 6.970347630165958819 ) ) ;
#32992=CARTESIAN_POINT ( 'NONE',  ( 7.125042791937182152, 121.7184703992695773, 0.7630849752878294812 ) ) ;
#32993=CARTESIAN_POINT ( 'NONE',  ( 0.3287531253414590626, 116.7093555017326452, -0.2203909396130737663 ) ) ;
#32994=DIRECTION ( 'NONE',  ( -0.9998004120163609398, 0.000000000000000000, -0.01997839162482749689 ) ) ;
#32998=EDGE_CURVE ( 'NONE', #18074, #3139, #4671, .T. ) ;
#33001=CARTESIAN_POINT ( 'NONE',  ( -4.404930073839969928, 118.1622843756694010, 0.4910954181917899786 ) ) ;
#33003=ORIENTED_EDGE ( 'NONE', *, *, #15761, .F. ) ;
#33006=CARTESIAN_POINT ( 'NONE',  ( 8.346771193436987701, 120.0109853342942472, -1.116703882779259027 ) ) ;
#33007=CARTESIAN_POINT ( 'NONE',  ( -5.131660560486008826, 115.4810986995850755, -1.508144361588663829 ) ) ;
#33008=CARTESIAN_POINT ( 'NONE',  ( 4.553093912424611922, 118.0135662636855756, 0.8850293724966483699 ) ) ;
#33009=CARTESIAN_POINT ( 'NONE',  ( -14.07483374865171477, 150.3034377993741657, -1.364178037702375779 ) ) ;
#33011=CARTESIAN_POINT ( 'NONE',  ( 4.709982941061709560, 118.1651004037422865, -0.4215969789121262190 ) ) ;
#33012=CARTESIAN_POINT ( 'NONE',  ( 0.3655860903868409229, 105.8811906981200934, -5.329044222542315801 ) ) ;
#33013=CARTESIAN_POINT ( 'NONE',  ( -10.36176036692648594, 123.5464890276372785, -1.327270239784479333 ) ) ;
#33014=FACE_OUTER_BOUND ( 'NONE', #24505, .T. ) ;
#33015=CARTESIAN_POINT ( 'NONE',  ( -0.003550340867792285433, 156.3099534201614631, 0.1776735749810083032 ) ) ;
#33016=CARTESIAN_POINT ( 'NONE',  ( 8.044334902818746968, 121.4620208242424155, -0.8712540157607662206 ) ) ;
#33017=CARTESIAN_POINT ( 'NONE',  ( -8.915496673695567864, 123.9583917734820915, -0.08963474529912127120 ) ) ;
#33018=CARTESIAN_POINT ( 'NONE',  ( 0.7336086519982950582, 0.2932837538699786251, -4.563195415240439701 ) ) ;
#33019=CARTESIAN_POINT ( 'NONE',  ( 10.56633813141740497, 157.9214973357695158, 0.8874509626871487367 ) ) ;
#33021=CARTESIAN_POINT ( 'NONE',  ( 2.598075364112794716, -15.28479904474297513, 4.671545106743766773 ) ) ;
#33022=CARTESIAN_POINT ( 'NONE',  ( -18.78841748004283119, 148.4604323410545987, 1.722921296925317369 ) ) ;
#33023=CARTESIAN_POINT ( 'NONE',  ( 0.8462494346447723137, 11.68649857616015275, 0.4938625092760188795 ) ) ;
#33024=CARTESIAN_POINT ( 'NONE',  ( -5.654702199549804575, 159.1134716836843381, -0.5125381600378308145 ) ) ;
#33025=CARTESIAN_POINT ( 'NONE',  ( -0.8770832347484921465, 27.56386522087566249, 0.4220112102557041500 ) ) ;
#33028=CARTESIAN_POINT ( 'NONE',  ( 5.567295163420428850, 119.7830797108918688, 0.4963393297495872769 ) ) ;
#33031=CARTESIAN_POINT ( 'NONE',  ( -8.149220328376188149, 154.6259123219959690, 0.6607633090041664659 ) ) ;
#33032=CARTESIAN_POINT ( 'NONE',  ( 4.057314763829551474, -13.83595378911055285, 4.182047561617943110 ) ) ;
#33033=CARTESIAN_POINT ( 'NONE',  ( 5.120154531940189102, 120.2090573957402455, -0.7231840875875844565 ) ) ;
#33034=CARTESIAN_POINT ( 'NONE',  ( 0.03256023585714045571, 157.9544661776888290, -1.629447346748784220 ) ) ;
#33035=CARTESIAN_POINT ( 'NONE',  ( 4.761265771961571858, 104.6144662015457527, 0.8484901396519970440 ) ) ;
#33036=CARTESIAN_POINT ( 'NONE',  ( 3.162461164278121739, -14.57801340048104777, 3.369881103115548893 ) ) ;
#33037=CARTESIAN_POINT ( 'NONE',  ( -1.820350978615107751, 35.44831059284695129, 0.3018992756893350005 ) ) ;
#33038=CARTESIAN_POINT ( 'NONE',  ( 15.54908666625160940, 147.5346097818530211, 0.08167737433607563657 ) ) ;
#33039=ORIENTED_EDGE ( 'NONE', *, *, #1457, .F. ) ;
#33040=CARTESIAN_POINT ( 'NONE',  ( -2.469273130011678141, 107.0255785817588645, 4.723498045142633828 ) ) ;
#33042=CARTESIAN_POINT ( 'NONE',  ( 4.801338745261147345, 117.3993836135855275, -1.016148444996444189 ) ) ;
#33044=CARTESIAN_POINT ( 'NONE',  ( 2.769246990704956612, 116.5678055239024644, -0.05256187475617109944 ) ) ;
#33045=CARTESIAN_POINT ( 'NONE',  ( -6.719914377344099243, 121.2247800624193133, 0.07397671124164069412 ) ) ;
#33046=CARTESIAN_POINT ( 'NONE',  ( -2.812155987513873079, 118.7629491485454167, 1.088229539211323038 ) ) ;
#33048=CARTESIAN_POINT ( 'NONE',  ( -0.4217933310832886473, 35.81132274965050044, -0.2641305449634421820 ) ) ;
#33049=CARTESIAN_POINT ( 'NONE',  ( 11.58753624721085984, 156.3395478113760362, 2.047021040405475389 ) ) ;
#33051=CARTESIAN_POINT ( 'NONE',  ( 3.724956840101937505, 21.94285949141939440, 2.734508905299370518 ) ) ;
#33052=CARTESIAN_POINT ( 'NONE',  ( -7.980626778564171353, 22.53057930515566554, 2.691543149341120156 ) ) ;
#33053=CARTESIAN_POINT ( 'NONE',  ( -8.615205574347543305, 118.4878503906377460, -1.080356039600459894 ) ) ;
#33054=CARTESIAN_POINT ( 'NONE',  ( -1.788686868886097292, 120.9773948236336878, -0.4149341611056206469 ) ) ;
#33057=CARTESIAN_POINT ( 'NONE',  ( -3.166910920246462258, 104.6144662015195621, 4.306197946819769307 ) ) ;
#33058=CARTESIAN_POINT ( 'NONE',  ( -4.636761822055341042, 12.60011390031314349, 0.2095705037016724059 ) ) ;
#33061=CARTESIAN_POINT ( 'NONE',  ( 2.681353593581013328, -14.83682625404381028, 4.634604895792218571 ) ) ;
#33062=CARTESIAN_POINT ( 'NONE',  ( 1.397093717039300964, 113.6455945353133643, -2.337579097500038117 ) ) ;
#33063=CARTESIAN_POINT ( 'NONE',  ( -0.005915287708768494392, 116.9295063353193882, 0.2960251855814710065 ) ) ;
#33064=CARTESIAN_POINT ( 'NONE',  ( 4.901578213037685927, 117.4095775641370523, -0.9679565193343001583 ) ) ;
#33065=EDGE_LOOP ( 'NONE', ( #4491, #5752, #38856, #30380 ) ) ;
#33070=CARTESIAN_POINT ( 'NONE',  ( 3.437591410214265064, -15.71306207096091789, 4.322042152151218453 ) ) ;
#33071=CARTESIAN_POINT ( 'NONE',  ( -16.05265579080208482, 153.3736753708079732, 1.680156470693515036 ) ) ;
#33072=CARTESIAN_POINT ( 'NONE',  ( 13.91986491619282873, 121.5005676099359846, -1.010465608187345321 ) ) ;
#33073=CARTESIAN_POINT ( 'NONE',  ( -0.2409191691226134635, 30.52881386638012629, -0.9476172785465332149 ) ) ;
#33077=CARTESIAN_POINT ( 'NONE',  ( -0.1065646865916382441, 105.8844662015457203, 5.332932678536313809 ) ) ;
#33080=CARTESIAN_POINT ( 'NONE',  ( -12.96210878518750498, 128.4900567078429390, 1.108396809849303777 ) ) ;
#33082=CARTESIAN_POINT ( 'NONE',  ( 17.94049195465762736, 148.7876888829155746, -1.661648619591604481 ) ) ;
#33083=CARTESIAN_POINT ( 'NONE',  ( -4.065609891792139940, 118.4217611105734846, -0.9713962693593599651 ) ) ;
#33086=CARTESIAN_POINT ( 'NONE',  ( 4.555104234677612496, 118.1072174076028034, -0.4957042797719007909 ) ) ;
#33087=CARTESIAN_POINT ( 'NONE',  ( 15.56233417011314124, 148.0963874134046705, -0.5341686659567148610 ) ) ;
#33089=ORIENTED_EDGE ( 'NONE', *, *, #17483, .F. ) ;
#33090=CARTESIAN_POINT ( 'NONE',  ( 1.863517626568274910, -15.41251410767331720, 5.374852164437769808 ) ) ;
#33094=CARTESIAN_POINT ( 'NONE',  ( 0.3254831797250597458, 1.427361272777448509, 4.610396533461925905 ) ) ;
#33095=CARTESIAN_POINT ( 'NONE',  ( 17.50701641564904776, 146.6691408387931688, 2.165841098895501027 ) ) ;
#33096=CARTESIAN_POINT ( 'NONE',  ( 2.842584213824973283, 37.57586378862247045, -0.09837489246507950813 ) ) ;
#33097=EDGE_CURVE ( 'NONE', #30817, #7672, #13645, .T. ) ;
#33098=CARTESIAN_POINT ( 'NONE',  ( 3.548611814566905664, 16.26088872207684943, 2.983771105379771971 ) ) ;
#33099=CARTESIAN_POINT ( 'NONE',  ( 8.097005894254447611, 122.8525693413601800, 0.3074703907764579358 ) ) ;
#33102=CARTESIAN_POINT ( 'NONE',  ( -2.162143947430365643, 116.2986588195852420, -0.2515325357244250215 ) ) ;
#33107=CARTESIAN_POINT ( 'NONE',  ( 2.958531772299235918, 50.42904571186020490, 1.329372033065076453 ) ) ;
#33109=FACE_OUTER_BOUND ( 'NONE', #32026, .T. ) ;
#33113=CARTESIAN_POINT ( 'NONE',  ( -22.60023854264601439, 150.6256779753201158, -0.001684207673826830986 ) ) ;
#33114=AXIS2_PLACEMENT_3D ( 'NONE', #39336, #22482, #32519 ) ;
#33115=ORIENTED_EDGE ( 'NONE', *, *, #14406, .T. ) ;
#33117=CARTESIAN_POINT ( 'NONE',  ( -6.961417914879455715, 121.9448106840860504, -0.2443103574289700597 ) ) ;
#33120=CARTESIAN_POINT ( 'NONE',  ( -8.053145991180288732, 122.8529229587361442, -0.1924930237977967862 ) ) ;
#33121=CARTESIAN_POINT ( 'NONE',  ( 4.021138818454151220, -15.00176662281678475, 5.141887924562631440 ) ) ;
#33122=CARTESIAN_POINT ( 'NONE',  ( -20.90199038452910685, 141.6159226613069109, 1.473829418026497251 ) ) ;
#33123=CARTESIAN_POINT ( 'NONE',  ( 3.211436584971100849, 28.15539441671475274, -3.345526564039049688 ) ) ;
#33124=CARTESIAN_POINT ( 'NONE',  ( 5.807154922825556120, 117.0096406922080376, 0.3504623104576318204 ) ) ;
#33125=CARTESIAN_POINT ( 'NONE',  ( 11.71381910070873644, 130.2301003178167775, 0.4045216064884521456 ) ) ;
#33126=CARTESIAN_POINT ( 'NONE',  ( 4.622858883031034871, 26.85595184169372374, 0.2084198311932836112 ) ) ;
#33127=CARTESIAN_POINT ( 'NONE',  ( -0.1494942157332288524, 1.595350521021342782, -0.9636992805340545143 ) ) ;
#33128=CARTESIAN_POINT ( 'NONE',  ( -9.776364138556823846, 118.0142902678875885, -0.3953848830946984361 ) ) ;
#33132=CARTESIAN_POINT ( 'NONE',  ( 5.530216759611570332, 117.0052764743229261, 0.6302382510017663364 ) ) ;
#33133=CARTESIAN_POINT ( 'NONE',  ( -17.80491421350304648, 148.0643276405518804, 1.576192721057973145 ) ) ;
#33135=CARTESIAN_POINT ( 'NONE',  ( 13.68454576465603800, 121.6032371815301900, 1.618700059879337294 ) ) ;
#33136=CARTESIAN_POINT ( 'NONE',  ( 8.613587046216144572, 156.7723266660784986, -1.729508645372233033 ) ) ;
#33137=CARTESIAN_POINT ( 'NONE',  ( -0.6334066649623988354, -12.81304641701132851, -0.7396855475671405555 ) ) ;
#33138=CARTESIAN_POINT ( 'NONE',  ( -20.70408045738755831, 151.0745573368290593, -1.983427051661964535 ) ) ;
#33140=CARTESIAN_POINT ( 'NONE',  ( 4.664901767118291076, 118.0183831904404741, -0.6239428623521563466 ) ) ;
#33141=CARTESIAN_POINT ( 'NONE',  ( 4.696425917957757434, 104.6144662015457243, 1.156094417919997674 ) ) ;
#33142=ADVANCED_FACE ( 'NONE', ( #20893 ), #18119, .F. ) ;
#33143=B_SPLINE_CURVE_WITH_KNOTS ( 'NONE', 1,
 ( #41898, #12697 ),
 .UNSPECIFIED., .F., .F.,
 ( 2, 2 ),
 ( 0.000000000000000000, 1.000000000000000000 ),
 .UNSPECIFIED. ) ;
#33144=CARTESIAN_POINT ( 'NONE',  ( 9.968563030426308202, 123.7598584631124794, -0.7002966798862195752 ) ) ;
#33145=CARTESIAN_POINT ( 'NONE',  ( -5.945776936743828678, 121.5465042053001667, -0.1188107733588233406 ) ) ;
#33146=ORIENTED_EDGE ( 'NONE', *, *, #19781, .T. ) ;
#33147=CARTESIAN_POINT ( 'NONE',  ( -11.57159210561028928, 122.7176759045101022, -1.727280539041415874 ) ) ;
#33148=CARTESIAN_POINT ( 'NONE',  ( 3.970714270704740922, -15.74271870963887743, 3.976543152134710990 ) ) ;
#33149=AXIS2_PLACEMENT_3D ( 'NONE', #16131, #32769, #29134 ) ;
#33151=CARTESIAN_POINT ( 'NONE',  ( -4.642530418943314530, 118.0244946899635323, -0.7554534729805311155 ) ) ;
#33154=CARTESIAN_POINT ( 'NONE',  ( 4.065926199369043204, 118.2429491485453354, 0.3080910687088499467 ) ) ;
#33155=CARTESIAN_POINT ( 'NONE',  ( 2.153957835384796127, 157.2504501563031738, 1.632675037709188537 ) ) ;
#33157=CARTESIAN_POINT ( 'NONE',  ( 21.68875320759051917, 132.7412702629105468, 0.4333929054516008073 ) ) ;
#33158=CARTESIAN_POINT ( 'NONE',  ( 7.077328715112659374, 6.763356510963684620, 4.580356461215433939 ) ) ;
#33159=CARTESIAN_POINT ( 'NONE',  ( 9.577010982343992396, 124.1734284925964573, 0.7139017932201211503 ) ) ;
#33160=CARTESIAN_POINT ( 'NONE',  ( 15.10519797802274056, 121.1899582252741112, -0.5359826722732081716 ) ) ;
#33161=CARTESIAN_POINT ( 'NONE',  ( 5.322333424082418496, 105.1224784086732171, -0.3647577769771441769 ) ) ;
#33163=CARTESIAN_POINT ( 'NONE',  ( 0.9590485603908195378, 118.7629491485454025, 1.264668241433272833 ) ) ;
#33166=CARTESIAN_POINT ( 'NONE',  ( -21.60220573293495860, 132.6646020023713959, -0.2978857061057720856 ) ) ;
#33168=CARTESIAN_POINT ( 'NONE',  ( -6.826600680103125818, 121.4509929031113131, -0.7999390687483252105 ) ) ;
#33170=CARTESIAN_POINT ( 'NONE',  ( -9.239529650026234719, 153.8817031120973411, -0.7017441744976310458 ) ) ;
#33171=CARTESIAN_POINT ( 'NONE',  ( 3.936650548058306054, -12.34391569202568384, 1.586490187297609156 ) ) ;
#33172=CARTESIAN_POINT ( 'NONE',  ( -22.09732278473127565, 146.2042277794223537, 1.157738048209833170 ) ) ;
#33174=CARTESIAN_POINT ( 'NONE',  ( 1.421330246821746801, 159.6054662015457666, 0.04208995589191837083 ) ) ;
#33176=CARTESIAN_POINT ( 'NONE',  ( -3.594857975007920814, -7.703025367003809798, -2.923569511714296798 ) ) ;
#33177=CARTESIAN_POINT ( 'NONE',  ( 0.5136544389551274126, 105.1227275070236686, 5.319539499184048559 ) ) ;
#33181=CARTESIAN_POINT ( 'NONE',  ( -4.496095910029399789, 118.6657657825083305, 0.8773962309065390652 ) ) ;
#33182=EDGE_CURVE ( 'NONE', #33565, #25673, #1684, .T. ) ;
#33183=CARTESIAN_POINT ( 'NONE',  ( -3.339653329301207840, -2.245917679271888900, -3.199182135983138053 ) ) ;
#33184=CARTESIAN_POINT ( 'NONE',  ( 13.81631647976127120, 120.6843904051541898, 1.269697867868520014 ) ) ;
#33186=DIRECTION ( 'NONE',  ( 0.9998004120163608288, 0.000000000000000000, 0.01997839162482736852 ) ) ;
#33187=CARTESIAN_POINT ( 'NONE',  ( 20.86711222142698929, 145.7124547906547889, -1.576573076165909360 ) ) ;
#33188=CARTESIAN_POINT ( 'NONE',  ( 0.3254831797250597458, 1.427361272777448509, 4.610396533461925905 ) ) ;
#33189=CARTESIAN_POINT ( 'NONE',  ( -15.07172804838065261, 121.1899582252741112, -1.138989471373297535 ) ) ;
#33190=ORIENTED_EDGE ( 'NONE', *, *, #17108, .F. ) ;
#33191=CARTESIAN_POINT ( 'NONE',  ( -13.12764272666535526, 133.9996589410087324, 0.1750096343312400049 ) ) ;
#33193=CARTESIAN_POINT ( 'NONE',  ( 5.718287093813156474, -14.23487671053640113, 2.942044405997081391 ) ) ;
#33194=DIRECTION ( 'NONE',  ( 0.9998004120163609398, 0.000000000000000000, 0.01997839162482749689 ) ) ;
#33195=TOROIDAL_SURFACE ( 'NONE', #20910, 5.080000000000005400, 0.5080000000000000071 ) ;
#33197=CARTESIAN_POINT ( 'NONE',  ( -5.184089659939317585, 115.9100003722667083, -1.325920433419026434 ) ) ;
#33199=CARTESIAN_POINT ( 'NONE',  ( 17.10357040864152367, 151.3967157021085654, 2.430234537686704055 ) ) ;
#33202=CARTESIAN_POINT ( 'NONE',  ( -5.427513099616406045, 158.9671755112622122, 0.8485680044740095962 ) ) ;
#33203=CARTESIAN_POINT ( 'NONE',  ( 3.560122487986403517, 2.076091768892780909, 7.630420683349803390 ) ) ;
#33204=CARTESIAN_POINT ( 'NONE',  ( 16.46997841215771530, 146.2355833862463328, 1.608729380348347782 ) ) ;
#33206=CARTESIAN_POINT ( 'NONE',  ( 0.004913308685965686075, 116.7872217978203224, -0.2458820580207658757 ) ) ;
#33210=CARTESIAN_POINT ( 'NONE',  ( -4.713276526765134200, 118.1588900175951977, 0.4357070110130277785 ) ) ;
#33213=CARTESIAN_POINT ( 'NONE',  ( -4.555299138033702455, 118.1072373763005032, 0.4955848589101189972 ) ) ;
#33217=CARTESIAN_POINT ( 'NONE',  ( 6.090059827715747609, 119.4132085878391223, -1.021381826822683303 ) ) ;
#33218=CARTESIAN_POINT ( 'NONE',  ( -3.430439322123234991, 108.6576027043044377, -4.130303871225995849 ) ) ;
#33219=CARTESIAN_POINT ( 'NONE',  ( 4.531728878287003326, 118.1072486390968379, 0.6773096721064315595 ) ) ;
#33220=CARTESIAN_POINT ( 'NONE',  ( -12.31319552751079449, 152.0262389575480881, -1.296791798139146801 ) ) ;
#33223=CARTESIAN_POINT ( 'NONE',  ( 2.802571055147052626, 117.9496044482589951, -1.216643114892233868 ) ) ;
#33224=CARTESIAN_POINT ( 'NONE',  ( 3.100166793870271498, 107.8178375082508609, -4.356447870432107905 ) ) ;
#33226=CARTESIAN_POINT ( 'NONE',  ( 0.008308630153154609663, 120.0570981805881559, -0.4157978282972238371 ) ) ;
#33227=CARTESIAN_POINT ( 'NONE',  ( -5.329475387727676150, 116.0444662015457311, -0.2797177882896795809 ) ) ;
#33229=CARTESIAN_POINT ( 'NONE',  ( 8.561575482294122352, 118.9452303826420092, -0.9294693558782792797 ) ) ;
#33230=CARTESIAN_POINT ( 'NONE',  ( -10.39299036940601439, 153.1602481698635643, -0.02716054506326659457 ) ) ;
#33231=CARTESIAN_POINT ( 'NONE',  ( 4.928175349042589026, 117.6470996705704124, 0.8667669811659319823 ) ) ;
#33232=CARTESIAN_POINT ( 'NONE',  ( 11.39485104697103779, 118.9229013597968247, 0.8408094927682292496 ) ) ;
#33234=CARTESIAN_POINT ( 'NONE',  ( 1.853042888461218007, -15.33088210119805339, 5.380378780177352382 ) ) ;
#33235=CARTESIAN_POINT ( 'NONE',  ( -2.387896358646931283, 119.0637060312156024, 0.6953999086667947971 ) ) ;
#33236=CARTESIAN_POINT ( 'NONE',  ( 0.9553521702984651975, -6.993735180969975929, 0.1873809170862112405 ) ) ;
#33237=CARTESIAN_POINT ( 'NONE',  ( -18.29650779608106603, 125.1624627582897915, -0.9465853942869045801 ) ) ;
#33238=CARTESIAN_POINT ( 'NONE',  ( 0.7743132463278736832, -9.628960163071635492, -0.5975928149734356376 ) ) ;
#33241=CARTESIAN_POINT ( 'NONE',  ( 3.889650775106587854, 109.8300753404742096, 3.673692233826463482 ) ) ;
#33242=CARTESIAN_POINT ( 'NONE',  ( -16.17919469456376902, 146.7365623387580342, 0.6462428564100395345 ) ) ;
#33243=CARTESIAN_POINT ( 'NONE',  ( 4.475827780916731946, -13.19141740729908108, 3.156716699630707890 ) ) ;
#33244=CARTESIAN_POINT ( 'NONE',  ( 9.186197600956422349, 155.0058477609193801, -1.458900829815475975 ) ) ;
#33245=CARTESIAN_POINT ( 'NONE',  ( -5.836180790127460050, 119.4106843418347950, -1.193569107438471333 ) ) ;
#33246=CARTESIAN_POINT ( 'NONE',  ( -3.966471220580447987, 104.6144662015457811, 2.768186473522256108 ) ) ;
#33247=EDGE_CURVE ( 'NONE', #28135, #7084, #18327, .T. ) ;
#33248=CARTESIAN_POINT ( 'NONE',  ( 3.047801963512828394, -14.61332798263154054, 3.862229702996769376 ) ) ;
#33249=CARTESIAN_POINT ( 'NONE',  ( -4.773210155766332008, 117.5405312103193438, -1.172205701249354304 ) ) ;
#33250=CARTESIAN_POINT ( 'NONE',  ( 10.43234786055276686, 153.0845720789597522, 0.001036074960337154093 ) ) ;
#33251=EDGE_LOOP ( 'NONE', ( #33003, #31730, #10578, #27600 ) ) ;
#33253=CARTESIAN_POINT ( 'NONE',  ( -6.589702033682734540E-14, 87.97746620154572383, -4.338478393988997516E-18 ) ) ;
#33254=CARTESIAN_POINT ( 'NONE',  ( -6.654617103318593247E-14, 104.6144662015457243, 1.534725424433578570E-31 ) ) ;
#33256=CARTESIAN_POINT ( 'NONE',  ( 18.63219679753382962, 154.1293031355326946, 0.2996243416495531497 ) ) ;
#33258=CARTESIAN_POINT ( 'NONE',  ( -3.100166793870399840, 107.8178375082508609, 4.356447870432107905 ) ) ;
#33260=CARTESIAN_POINT ( 'NONE',  ( 2.060254573934078515, -15.43196230555739312, 5.989929398572627406 ) ) ;
#33261=CARTESIAN_POINT ( 'NONE',  ( -3.148524768479886937, 30.89467502894793327, -0.4672404312464801812 ) ) ;
#33262=CARTESIAN_POINT ( 'NONE',  ( -3.346823384277141766, 31.23146344785865480, -0.04602645998765462348 ) ) ;
#33263=CARTESIAN_POINT ( 'NONE',  ( 20.40332572169740288, 149.1468970683199586, 2.432323357318189050 ) ) ;
#33265=CARTESIAN_POINT ( 'NONE',  ( 4.103208822911150300, 18.85939590645278585, -7.354229849909827088 ) ) ;
#33266=CARTESIAN_POINT ( 'NONE',  ( -5.478737692705611728, 117.5010888497598103, -0.9448662039476222185 ) ) ;
#33267=CARTESIAN_POINT ( 'NONE',  ( -1.644890720626135172, 119.8612358676174949, -0.5912986496483324528 ) ) ;
#33271=CARTESIAN_POINT ( 'NONE',  ( 3.746277899330032302, -0.8937244826341392834, -2.755274729908455900 ) ) ;
#33273=CARTESIAN_POINT ( 'NONE',  ( -4.855449335888874174, 115.6909491485453003, 1.281272725539408297 ) ) ;
#33274=CARTESIAN_POINT ( 'NONE',  ( 2.976679874252225577, -13.20894259333504905, 0.9412263588231246647 ) ) ;
#33275=CARTESIAN_POINT ( 'NONE',  ( 3.568793996893895315, 120.2162445758188056, -0.3416935720284703937 ) ) ;
#33276=CARTESIAN_POINT ( 'NONE',  ( -0.01133159106151501033, 159.5297144918048673, 0.5670791535570577357 ) ) ;
#33279=( BOUNDED_SURFACE ( )  B_SPLINE_SURFACE ( 3, 2, ( 
 ( #30907, #1117, #18111 ),
 ( #37102, #17904, #14705 ),
 ( #8330, #4525, #17489 ),
 ( #40095, #21300, #4323 ),
 ( #7920, #17691, #20886 ),
 ( #27508, #7716, #14286 ),
 ( #34117, #8119, #33910 ),
 ( #17286, #4944, #11309 ),
 ( #1746, #20679, #10682 ),
 ( #30276, #4738, #31116 ),
 ( #30690, #27710, #30485 ),
 ( #1328, #40719, #5157 ),
 ( #11514, #34328, #24091 ),
 ( #1540, #36683, #40517 ),
 ( #27295, #33704, #40310 ),
 ( #1953, #26877, #7505 ),
 ( #11103, #37302, #20464 ),
 ( #12370, #25561, #15755 ),
 ( #15124, #41137, #37932 ),
 ( #24934, #28344, #12574 ),
 ( #41562, #5572, #19164 ),
 ( #28760, #18739, #24718 ),
 ( #15339, #2165, #34538 ),
 ( #38565, #38362, #6195 ),
 ( #25147, #28554, #2592 ),
 ( #2379, #8964, #22134 ),
 ( #21932, #41353, #5364 ),
 ( #25358, #31749, #5990 ),
 ( #40923, #18319, #31321 ),
 ( #15552, #28127, #21505 ),
 ( #18953, #32168, #18530 ),
 ( #34741, #9177, #35163 ),
 ( #34961, #11943, #31959 ),
 ( #8755, #9378, #37722 ),
 ( #12155, #2798, #14913 ),
 ( #41773, #21717, #38151 ),
 ( #11729, #31535, #22342 ),
 ( #35365, #5784, #27917 ),
 ( #8546, #22760, #12983 ),
 ( #654, #9792, #29607 ),
 ( #7247, #35793, #29815 ),
 ( #12776, #16166, #3417 ) ),
 .UNSPECIFIED., .F., .F., .T. ) 
 B_SPLINE_SURFACE_WITH_KNOTS ( ( 4, 2, 2, 2, 2, 2, 2, 2, 2, 2, 2, 2, 2, 2, 2, 2, 2, 2, 2, 2, 4 ),
 ( 3, 3 ),
 ( 0.000000000000000000, 0.0009429120494251018838, 0.001414368074137652880, 0.001885824098850203768, 0.002828736148275305760, 0.003771648197700407535, 0.004714560247125509744, 0.005186016271838060632, 0.005657472296550611519, 0.006600384345975713295, 0.007543296395400815070, 0.008486208444825917713, 0.009429120494251019488, 0.009900576518963571243, 0.01037203254367612126, 0.01131494459310122304, 0.01225785664252632481, 0.01272931266723887483, 0.01320076869195142659, 0.01414368074137652836, 0.01508659279080163014 ),
 ( 0.000000000000000000, 1.000000000000000000 ),
 .UNSPECIFIED. ) 
 GEOMETRIC_REPRESENTATION_ITEM ( )  RATIONAL_B_SPLINE_SURFACE ( (
 ( 1.000000000000000000, 0.7071103834195795468, 1.000000000000000000),
 ( 1.000000000000000000, 0.7071124051442869707, 1.000000000000000000),
 ( 1.000000000000000000, 0.7070849312894228467, 1.000000000000000000),
 ( 1.000000000000000000, 0.7071123019286037481, 1.000000000000000000),
 ( 1.000000000000000000, 0.7071614862087763909, 1.000000000000000000),
 ( 1.000000000000000000, 0.7073010037706329856, 1.000000000000000000),
 ( 1.000000000000000000, 0.7073901506915791781, 1.000000000000000000),
 ( 1.000000000000000000, 0.7076394263844208998, 1.000000000000000000),
 ( 1.000000000000000000, 0.7077756853797776415, 1.000000000000000000),
 ( 1.000000000000000000, 0.7077567304198957299, 1.000000000000000000),
 ( 1.000000000000000000, 0.7075957674067504533, 1.000000000000000000),
 ( 1.000000000000000000, 0.7070041386104982672, 1.000000000000000000),
 ( 1.000000000000000000, 0.7065667128226251759, 1.000000000000000000),
 ( 1.000000000000000000, 0.7061037264541912828, 1.000000000000000000),
 ( 1.000000000000000000, 0.7059795971604051479, 1.000000000000000000),
 ( 1.000000000000000000, 0.7058187053605305961, 1.000000000000000000),
 ( 1.000000000000000000, 0.7057806473396187608, 1.000000000000000000),
 ( 1.000000000000000000, 0.7057897566527251421, 1.000000000000000000),
 ( 1.000000000000000000, 0.7059679295365862695, 1.000000000000000000),
 ( 1.000000000000000000, 0.7064617003595946576, 1.000000000000000000),
 ( 1.000000000000000000, 0.7067673356939784268, 1.000000000000000000),
 ( 1.000000000000000000, 0.7071356715510913604, 1.000000000000000000),
 ( 1.000000000000000000, 0.7071413527495709062, 1.000000000000000000),
 ( 1.000000000000000000, 0.7067748178510451229, 1.000000000000000000),
 ( 1.000000000000000000, 0.7064655642066967056, 1.000000000000000000),
 ( 1.000000000000000000, 0.7060874411990923916, 1.000000000000000000),
 ( 1.000000000000000000, 0.7059745403824593257, 1.000000000000000000),
 ( 1.000000000000000000, 0.7058136453788583786, 1.000000000000000000),
 ( 1.000000000000000000, 0.7057652904070991218, 1.000000000000000000),
 ( 1.000000000000000000, 0.7057433926758498455, 1.000000000000000000),
 ( 1.000000000000000000, 0.7059038550872894779, 1.000000000000000000),
 ( 1.000000000000000000, 0.7065143984468699179, 1.000000000000000000),
 ( 1.000000000000000000, 0.7069574456150055086, 1.000000000000000000),
 ( 1.000000000000000000, 0.7074174870072401644, 1.000000000000000000),
 ( 1.000000000000000000, 0.7075394654349829171, 1.000000000000000000),
 ( 1.000000000000000000, 0.7077084337036048112, 1.000000000000000000),
 ( 1.000000000000000000, 0.7077551412959035559, 1.000000000000000000),
 ( 1.000000000000000000, 0.7077863613254063990, 1.000000000000000000),
 ( 1.000000000000000000, 0.7076589125939298786, 1.000000000000000000),
 ( 1.000000000000000000, 0.7073336049174636653, 1.000000000000000000),
 ( 1.000000000000000000, 0.7071402517120219944, 1.000000000000000000),
 ( 1.000000000000000000, 0.7071072175333811272, 1.000000000000000000) ) ) 
 REPRESENTATION_ITEM ( '' )  SURFACE ( )  );
#33281=CARTESIAN_POINT ( 'NONE',  ( -1.606566256928685599, 32.19982401495065716, 1.077694121983207021 ) ) ;
#33282=CARTESIAN_POINT ( 'NONE',  ( 5.240434970354078459, -15.39321860721029545, 1.015353449650246764 ) ) ;
#33283=CARTESIAN_POINT ( 'NONE',  ( -19.78169998575278044, 149.7343351798865285, 1.666391814173802999 ) ) ;
#33284=CARTESIAN_POINT ( 'NONE',  ( -2.983771112188844832, -5.329111280313512999, 3.548611825089460048 ) ) ;
#33288=CARTESIAN_POINT ( 'NONE',  ( 1.009032787325873537, 123.9312678891798640, 0.1103529103309999343 ) ) ;
#33290=CARTESIAN_POINT ( 'NONE',  ( -5.875224328284241793, 120.7327493588883840, 0.6546335550538251447 ) ) ;
#33291=CARTESIAN_POINT ( 'NONE',  ( 3.841735362705627210, 118.0214076499569700, 0.9713319504342076138 ) ) ;
#33293=CARTESIAN_POINT ( 'NONE',  ( 18.09865239071504206, 149.0664087073519681, -1.700023788287825299 ) ) ;
#33295=CARTESIAN_POINT ( 'NONE',  ( -12.86454329319610856, 121.9120276846612256, -1.753115191834736963 ) ) ;
#33298=CARTESIAN_POINT ( 'NONE',  ( 4.239670762977913121, 118.2238228529691213, -0.3214580067528489682 ) ) ;
#33299=CARTESIAN_POINT ( 'NONE',  ( 8.072651008563752839, 154.6119571123129788, -0.5584669891872421355 ) ) ;
#33301=CARTESIAN_POINT ( 'NONE',  ( 3.009962208777686499, -14.98531826913061771, 3.912431539232285704 ) ) ;
#33302=CARTESIAN_POINT ( 'NONE',  ( 4.023522443498899648, 105.1224988529233144, -3.517836912119111314 ) ) ;
#33303=CARTESIAN_POINT ( 'NONE',  ( -0.3558933743640902425, 1.202427940091101100, 4.626034787239965418 ) ) ;
#33304=CARTESIAN_POINT ( 'NONE',  ( 9.709460118793433736, 122.6450757329969434, 1.337221984871323821 ) ) ;
#33305=CARTESIAN_POINT ( 'NONE',  ( 2.944445591501515747, 38.71711244820894393, 0.2891746879855487395 ) ) ;
#33306=CARTESIAN_POINT ( 'NONE',  ( 4.573446973487649281, 17.56025517495590904, -0.6989348988664985107 ) ) ;
#33307=CARTESIAN_POINT ( 'NONE',  ( 15.39298062464833450, 147.8297367799732456, 0.5361660792469027381 ) ) ;
#33308=CARTESIAN_POINT ( 'NONE',  ( -2.872265077263356226, 44.28946620154572855, -5.646510212151727437 ) ) ;
#33311=CARTESIAN_POINT ( 'NONE',  ( 8.797613110180989793, 117.6982703817063367, 0.05471292246626040245 ) ) ;
#33312=CARTESIAN_POINT ( 'NONE',  ( 1.421603664355671315, 159.6054662015457666, 0.02840702444251847966 ) ) ;
#33314=CARTESIAN_POINT ( 'NONE',  ( -6.451606698686837575E-14, 65.62546620154573418, 4.217636114931141265E-29 ) ) ;
#33318=FACE_OUTER_BOUND ( 'NONE', #38680, .T. ) ;
#33320=CARTESIAN_POINT ( 'NONE',  ( 0.01180776361637191768, 120.3637084677655764, -0.5909087754570011564 ) ) ;
#33321=CARTESIAN_POINT ( 'NONE',  ( -5.699072711719833428, 159.1209727096294273, 0.1881040421785058481 ) ) ;
#33324=CARTESIAN_POINT ( 'NONE',  ( 7.792635189458867906, 122.6008994260911891, 0.03648374067325547282 ) ) ;
#33326=CARTESIAN_POINT ( 'NONE',  ( -8.798071503382049130, 117.6842349159514640, -0.1758064068840608507 ) ) ;
#33327=CARTESIAN_POINT ( 'NONE',  ( 0.001367086239699496575, 156.3041635968983485, -0.06841458569046195148 ) ) ;
#33328=CARTESIAN_POINT ( 'NONE',  ( 2.293780832555937010, -15.47183500671027367, 5.912194120686782739 ) ) ;
#33329=CARTESIAN_POINT ( 'NONE',  ( -21.18042260023744205, 148.1333099715771766, 1.515480231459294336 ) ) ;
#33330=CARTESIAN_POINT ( 'NONE',  ( 1.580769961479467911, 28.79261460129497863, -4.363931058323818668 ) ) ;
#33331=CARTESIAN_POINT ( 'NONE',  ( 4.764559463231916148, 116.8420656028321218, 0.3170442335454677907 ) ) ;
#33332=CARTESIAN_POINT ( 'NONE',  ( 2.224323458635174777, -15.45660113867128338, 5.869303334135124395 ) ) ;
#33333=CARTESIAN_POINT ( 'NONE',  ( 2.332027132427558769, 25.33165720878049498, 3.998286310156994983 ) ) ;
#33334=CARTESIAN_POINT ( 'NONE',  ( -0.3677562164248854293, -4.027846162062824753, 0.9036657059391408620 ) ) ;
#33335=CARTESIAN_POINT ( 'NONE',  ( -0.9228193675735004708, 116.5712332538976455, -0.1866785551396778486 ) ) ;
#33337=CARTESIAN_POINT ( 'NONE',  ( 4.937305977349591757, 117.4065427751604460, 1.082467720437599645 ) ) ;
#33338=ORIENTED_EDGE ( 'NONE', *, *, #12282, .F. ) ;
#33339=CARTESIAN_POINT ( 'NONE',  ( -2.194728688019693674, 116.2160623166575277, 0.009134385426443037206 ) ) ;
#33340=CARTESIAN_POINT ( 'NONE',  ( -16.80660261901795849, 149.5530097695598215, 1.582604632240843801 ) ) ;
#33342=CARTESIAN_POINT ( 'NONE',  ( 4.922209265113101750, 118.1424809852657773, 0.9875327093606014461 ) ) ;
#33343=CARTESIAN_POINT ( 'NONE',  ( 3.262238196373776766, 118.8118204130220903, -0.7766580032327176086 ) ) ;
#33344=CARTESIAN_POINT ( 'NONE',  ( -0.7500621227288748472, -10.43934603300536956, 0.6214162388253807734 ) ) ;
#33345=CARTESIAN_POINT ( 'NONE',  ( -7.877908914988320355, 118.7344292658239340, -1.218006232967851377 ) ) ;
#33347=CARTESIAN_POINT ( 'NONE',  ( 4.970465051853945937, 104.6144662015435642, 1.943362965483819593 ) ) ;
#33349=CARTESIAN_POINT ( 'NONE',  ( 16.53085885483072559, 146.5532241433796230, -0.9478179252731553373 ) ) ;
#33350=CARTESIAN_POINT ( 'NONE',  ( -15.64207015331068185, 147.2204672151589193, -0.3125657877211906466 ) ) ;
#33352=CARTESIAN_POINT ( 'NONE',  ( -18.59210649535975435, 147.7499600834086948, -2.443498639627971869 ) ) ;
#33353=CARTESIAN_POINT ( 'NONE',  ( 5.113606203424133412, -15.47995924129362599, 1.801594979316981204 ) ) ;
#33355=CARTESIAN_POINT ( 'NONE',  ( -4.659430783399328035, 117.9638225107766800, -0.9016972064179303858 ) ) ;
#33358=CARTESIAN_POINT ( 'NONE',  ( 7.396903380747357204, 120.6159063994810055, 1.271367681336521782 ) ) ;
#33359=CARTESIAN_POINT ( 'NONE',  ( -3.328555392133318858, 33.88165127674241717, 1.160568618710268618 ) ) ;
#33360=CARTESIAN_POINT ( 'NONE',  ( 16.17587344042694397, 121.2571949256804089, 0.3060957306870976113 ) ) ;
#33361=CARTESIAN_POINT ( 'NONE',  ( -4.329333532990936817, 10.85900946394830413, -7.254296797256971630 ) ) ;
#33362=CARTESIAN_POINT ( 'NONE',  ( 8.259016884198906894, 122.7564308547279666, 0.6276379194545153029 ) ) ;
#33363=CARTESIAN_POINT ( 'NONE',  ( 22.10675755583028490, 150.4421090420883900, -0.7299123522449002532 ) ) ;
#33365=AXIS2_PLACEMENT_3D ( 'NONE', #12228, #25633, #38643 ) ;
#33366=CARTESIAN_POINT ( 'NONE',  ( 3.682264917456191888, 104.6144662015457243, 0.07358041635424013294 ) ) ;
#33367=CARTESIAN_POINT ( 'NONE',  ( -9.815320032040085962, 117.9943556427423488, -0.1502691370658184589 ) ) ;
#33369=CARTESIAN_POINT ( 'NONE',  ( 5.671770810419905828, 120.9487722882625604, -0.4210702782392469201 ) ) ;
#33373=CARTESIAN_POINT ( 'NONE',  ( -11.34253674425788994, 128.2076764602477681, -0.6137764907266787251 ) ) ;
#33374=CARTESIAN_POINT ( 'NONE',  ( 3.029556690758328674, -14.73736909467317169, 5.484434072839230012 ) ) ;
#33375=CARTESIAN_POINT ( 'NONE',  ( -22.40052491088804842, 148.4347612714453248, 0.9998933253014316014 ) ) ;
#33377=CARTESIAN_POINT ( 'NONE',  ( 0.2977815589728530221, 116.4565202671238069, 0.07303518451646379139 ) ) ;
#33379=CARTESIAN_POINT ( 'NONE',  ( -0.8472427164685307766, -8.777537934218566207, -4.544909406875613733 ) ) ;
#33380=CARTESIAN_POINT ( 'NONE',  ( -3.706843470526901996, 116.6237204831772232, -0.08772160974583163850 ) ) ;
#33383=B_SPLINE_CURVE_WITH_KNOTS ( 'NONE', 3,
 ( #7480, #20229, #33466, #40286, #4085, #30044, #11078, #11283 ),
 .UNSPECIFIED., .F., .F.,
 ( 4, 2, 2, 4 ),
 ( -6.000000000046590246E-08, 0.002398650364449638004, 0.003598005546674457045, 0.004797360728899276519 ),
 .UNSPECIFIED. ) ;
#33385=CARTESIAN_POINT ( 'NONE',  ( -8.274446143174570167, 120.3630673002886056, 1.110374729364685065 ) ) ;
#33386=CARTESIAN_POINT ( 'NONE',  ( -1.146732334619779969, -3.095543821355960734, -4.488006035213349953 ) ) ;
#33387=CARTESIAN_POINT ( 'NONE',  ( 5.309498559578469390, 158.9031408473208273, 1.190161311236993313 ) ) ;
#33390=CARTESIAN_POINT ( 'NONE',  ( 20.99182874412617039, 148.0559997909317644, -1.564581863923973470 ) ) ;
#33391=CARTESIAN_POINT ( 'NONE',  ( -4.449009123739010363, -11.09185097514761331, -1.246716907482375847 ) ) ;
#33392=CARTESIAN_POINT ( 'NONE',  ( -5.838122194618600602, 117.4684171610355747, -0.7518181979692856176 ) ) ;
#33393=TOROIDAL_SURFACE ( 'NONE', #12303, 5.080000000000005400, 0.5080000000000000071 ) ;
#33394=ADVANCED_FACE ( 'NONE', ( #25366 ), #25585, .T. ) ;
#33395=ORIENTED_EDGE ( 'NONE', *, *, #23484, .F. ) ;
#33396=CARTESIAN_POINT ( 'NONE',  ( -0.6587526420363846169, 156.3106852680424765, 0.1744449402554847373 ) ) ;
#33397=CARTESIAN_POINT ( 'NONE',  ( 5.379112111825198106, -14.48849916137785776, 3.594839802689186570 ) ) ;
#33400=B_SPLINE_CURVE_WITH_KNOTS ( 'NONE', 3,
 ( #11512, #39298, #13520, #10732, #8328, #753, #36732, #963, #36324, #30123, #20099, #7555, #17902, #33330, #39729, #7142, #33123, #13728, #3741, #36111, #3952, #26508, #26721, #10528, #36525, #17123, #21298, #29704, #4375, #18109, #16914, #4160, #23498, #23714, #34326, #39513, #7344, #26290, #13932, #26927, #5155, #40717, #19895, #10106, #20304, #39940, #20515, #33543, #30905, #16699, #1744, #14703, #27708, #24498, #37502, #337, #32910, #13303, #6925, #545, #10319, #23287, #18527, #25355, #9174, #18316, #5781, #34535, #37719, #34738, #22131, #6192, #5569, #35160, #9375, #2162, #5987, #25558, #28341, #31532, #12152, #40921, #15121, #38562, #11727, #28124, #2376, #28551, #35362, #15752, #12367, #41350, #31114, #8543, #41134, #11940, #41559, #41770, #31956, #21502, #31318, #24931, #22339, #21714, #1951, #21929, #2795, #8752, #27915, #38359, #18736, #18950, #28757, #34958, #24715, #37929, #15336, #25144, #5361, #38148, #31746, #14911, #8961, #2589, #15549, #12571, #13410, #12773, #3847, #22757, #20000, #25763, #3414, #35790, #38770, #32581, #26399, #9581, #16811, #6602, #33018, #16381, #19366, #9997, #14, #35999, #19782, #22550, #23177, #23394, #22969, #15960, #3000, #652, #29386, #32372, #3201, #19573, #226, #13201, #6812, #7033, #26185, #41974, #39618, #39404, #29813, #39189, #10207, #13620, #16163, #35580, #32801, #26611, #29168, #6396, #10424, #12980, #28958, #3632, #16596, #29605, #440, #25973, #36212, #36426, #19161, #32165, #38981, #9789, #1487, #30226, #17851, #4059, #20411 ),
 .UNSPECIFIED., .F., .F.,
 ( 4, 1, 1, 1, 1, 1, 1, 1, 1, 1, 1, 1, 1, 1, 1, 1, 1, 1, 1, 1, 1, 1, 1, 1, 1, 1, 1, 1, 1, 1, 1, 1, 1, 1, 1, 1, 1, 1, 1, 1, 1, 1, 1, 1, 1, 1, 1, 1, 1, 1, 1, 1, 1, 1, 1, 1, 1, 1, 1, 1, 1, 1, 1, 1, 1, 1, 1, 1, 1, 1, 1, 1, 1, 1, 1, 1, 1, 1, 1, 1, 1, 1, 1, 1, 1, 1, 1, 1, 1, 1, 1, 1, 1, 1, 1, 1, 1, 1, 1, 1, 1, 1, 1, 1, 1, 1, 1, 1, 1, 1, 1, 1, 1, 1, 1, 1, 1, 1, 1, 1, 1, 1, 1, 1, 1, 1, 1, 1, 1, 1, 1, 1, 1, 1, 1, 1, 1, 1, 1, 1, 1, 1, 1, 1, 1, 1, 1, 1, 1, 1, 1, 1, 1, 1, 1, 1, 1, 1, 1, 1, 1, 1, 1, 1, 1, 1, 1, 1, 1, 1, 1, 1, 1, 1, 1, 1, 1, 1, 1, 1, 1, 1, 1, 1, 1, 1, 1, 1, 1, 1, 1, 1, 4 ),
 ( 0.000000000000000000, 0.007812500000000423273, 0.01388888888888889506, 0.01562500000000000000, 0.02343749999999998959, 0.02777777777777778317, 0.03125000000000092981, 0.03906249999999999306, 0.04166666666666667823, 0.04687500000000000000, 0.05468749999999999306, 0.05555555555555556635, 0.06249999999999997918, 0.06944444444444446141, 0.07031250000000000000, 0.07812500000000000000, 0.08333333333333334259, 0.08593749999999998612, 0.09374999999999603095, 0.09722222222222223764, 0.1015625000000000139, 0.1093750000000000000, 0.1111111111111111188, 0.1171875000000000000, 0.1250000000000000000, 0.1328125000000000000, 0.1388888888888889228, 0.1406250000000000000, 0.1484375000000000000, 0.1527777777777778179, 0.1562500000000039690, 0.1640625000000000000, 0.1666666666666666852, 0.1718750000000000000, 0.1796875000000000000, 0.1805555555555555802, 0.1875000000000000000, 0.1944444444444444753, 0.1953125000000000000, 0.2031250000000000000, 0.2083333333333333703, 0.2109375000000000000, 0.2187499999999960310, 0.2222222222222222376, 0.2265625000000000000, 0.2343750000000000000, 0.2361111111111111327, 0.2421875000000000000, 0.2500000000000000000, 0.2578125000000000000, 0.2638888888888888951, 0.2656250000000000000, 0.2734375000000000000, 0.2777777777777777346, 0.2812500000000039968, 0.2890625000000000000, 0.2916666666666665741, 0.2968750000000000000, 0.3046875000000000000, 0.3055555555555554692, 0.3125000000000000000, 0.3194444444444443088, 0.3203125000000000000, 0.3281250000000000000, 0.3333333333333332038, 0.3359375000000000000, 0.3437499999999960587, 0.3472222222222220434, 0.3515625000000000000, 0.3593750000000000000, 0.3611111111111109384, 0.3671875000000000000, 0.3750000000000000000, 0.3828125000000000000, 0.3888888888888886175, 0.3906250000000000000, 0.3984375000000000000, 0.4027777777777775126, 0.4062500000000039968, 0.4140625000000000000, 0.4166666666666663521, 0.4218750000000000000, 0.4296875000000000000, 0.4305555555555552472, 0.4375000000000000000, 0.4444444444444440867, 0.4453125000000000000, 0.4531250000000000000, 0.4583333333333329818, 0.4609375000000000000, 0.4687499999999960587, 0.4722222222222218768, 0.4765625000000000000, 0.4843750000000000000, 0.4861111111111107719, 0.4921875000000000000, 0.5000000000000000000, 0.5078125000000000000, 0.5138888888888886175, 0.5156250000000000000, 0.5234375000000000000, 0.5277777777777775681, 0.5312500000000039968, 0.5390625000000000000, 0.5416666666666664076, 0.5468750000000000000, 0.5546875000000000000, 0.5555555555555553582, 0.5625000000000000000, 0.5694444444444443088, 0.5703125000000000000, 0.5781250000000000000, 0.5833333333333331483, 0.5859375000000000000, 0.5937499999999960032, 0.5972222222222220989, 0.6015625000000000000, 0.6093750000000000000, 0.6111111111111110494, 0.6171875000000000000, 0.6250000000000000000, 0.6328125000000000000, 0.6388888888888888395, 0.6406250000000000000, 0.6484375000000000000, 0.6527777777777777901, 0.6562500000000039968, 0.6640625000000000000, 0.6666666666666666297, 0.6718750000000000000, 0.6796875000000000000, 0.6805555555555555802, 0.6875000000000000000, 0.6944444444444445308, 0.6953125000000000000, 0.7031250000000000000, 0.7083333333333333703, 0.7109375000000000000, 0.7187499999999960032, 0.7222222222222223209, 0.7265625000000000000, 0.7343750000000000000, 0.7361111111111111605, 0.7421875000000000000, 0.7500000000000000000, 0.7578125000000000000, 0.7638888888888889506, 0.7656250000000000000, 0.7734375000000000000, 0.7777777777777779011, 0.7812500000000039968, 0.7890625000000000000, 0.7916666666666668517, 0.7968750000000000000, 0.8046875000000000000, 0.8055555555555556912, 0.8125000000000000000, 0.8194444444444446418, 0.8203125000000000000, 0.8281250000000000000, 0.8333333333333335924, 0.8359375000000000000, 0.8437499999999960032, 0.8472222222222224319, 0.8515625000000000000, 0.8593750000000000000, 0.8611111111111113825, 0.8671875000000000000, 0.8750000000000000000, 0.8828125000000000000, 0.8888888888888891726, 0.8906250000000000000, 0.8984375000000000000, 0.9027777777777781232, 0.9062500000000039968, 0.9140625000000000000, 0.9166666666666670737, 0.9218750000000000000, 0.9296875000000000000, 0.9305555555555559133, 0.9375000000000000000, 0.9444444444444447528, 0.9453125000000000000, 0.9531250000000000000, 0.9583333333333335924, 0.9609375000000000000, 0.9687499999999991118, 0.9722222222222224319, 0.9765625000000000000, 0.9843750000000000000, 0.9861111111111111605, 0.9921874999999995559, 1.000000000000000000 ),
 .UNSPECIFIED. ) ;
#33401=CARTESIAN_POINT ( 'NONE',  ( 0.02983097946977083040, 117.3993836135855133, -1.492864285907016697 ) ) ;
#33403=ORIENTED_EDGE ( 'NONE', *, *, #14947, .T. ) ;
#33404=CARTESIAN_POINT ( 'NONE',  ( 3.228607480374420913, 118.8118204130220903, 0.9063605472083391401 ) ) ;
#33405=CARTESIAN_POINT ( 'NONE',  ( 4.973152232786927307, 117.3993868326352015, 0.9753084504214339923 ) ) ;
#33407=CARTESIAN_POINT ( 'NONE',  ( -0.006942562093356200587, 117.0978366787122127, 0.3474341964894884782 ) ) ;
#33408=CARTESIAN_POINT ( 'NONE',  ( -1.555401355773622374, 10.72473834230686762, 8.302158768936594768 ) ) ;
#33409=CARTESIAN_POINT ( 'NONE',  ( 7.153290765949940955, 121.6016026263613838, 0.8513816870021355676 ) ) ;
#33411=CARTESIAN_POINT ( 'NONE',  ( 15.85309526068949104, 121.4040080620525117, -0.2080479070310632672 ) ) ;
#33415=CARTESIAN_POINT ( 'NONE',  ( -2.811131974896623031, 117.3993815978873414, 1.303371054368798410 ) ) ;
#33419=EDGE_CURVE ( 'NONE', #29613, #21134, #26691, .T. ) ;
#33420=CARTESIAN_POINT ( 'NONE',  ( -4.378391549104950542, 118.1844058569687519, 0.4336172515691945617 ) ) ;
#33421=CARTESIAN_POINT ( 'NONE',  ( 3.441724091444921196, 108.4907294080017692, -4.067959973020410125 ) ) ;
#33426=CARTESIAN_POINT ( 'NONE',  ( -6.088634770323529288, 119.5152126290041679, -1.257500645984790166 ) ) ;
#33427=CARTESIAN_POINT ( 'NONE',  ( -7.694725746745366912, 124.7202454748262710, -0.1536377669325635076 ) ) ;
#33429=CARTESIAN_POINT ( 'NONE',  ( 4.541907748926803379, 118.0342732306360176, 0.8605405987047681782 ) ) ;
#33430=CARTESIAN_POINT ( 'NONE',  ( -9.448695200928863613, 153.9068681542131856, -1.043141309954137341 ) ) ;
#33431=CARTESIAN_POINT ( 'NONE',  ( -0.5787063603190276684, 115.7029630171035848, -1.760568961526914000 ) ) ;
#33433=CARTESIAN_POINT ( 'NONE',  ( 0.5514881128753655881, 117.3993826274773795, -1.472903135207439762 ) ) ;
#33434=CARTESIAN_POINT ( 'NONE',  ( 6.540839804427455384, 120.6338824379019172, -0.1347920106280765806 ) ) ;
#33435=CARTESIAN_POINT ( 'NONE',  ( -16.27782172975869557, 148.1602266505728380, -1.760797687140677192 ) ) ;
#33438=CARTESIAN_POINT ( 'NONE',  ( 8.625062891301235268, 118.6226016915421582, -0.7970602507506778789 ) ) ;
#33439=CARTESIAN_POINT ( 'NONE',  ( -0.002141537396551156710, 156.3034662015459446, 0.1071712884387201609 ) ) ;
#33441=CARTESIAN_POINT ( 'NONE',  ( 20.83375562662813962, 132.2939277659177151, 1.304325680028331824 ) ) ;
#33442=DIRECTION ( 'NONE',  ( 5.206863593109713661E-17, -1.000000000000000000, 1.077750396879097183E-30 ) ) ;
#33443=CARTESIAN_POINT ( 'NONE',  ( 3.373996639098103323, -14.83046237366941789, 1.396824179944331723 ) ) ;
#33444=CARTESIAN_POINT ( 'NONE',  ( -9.549337214234009608, 121.2752502669211339, 1.156350410895870429 ) ) ;
#33445=CARTESIAN_POINT ( 'NONE',  ( -0.7500621227288748472, -10.43934603300536956, 0.6214162388253807734 ) ) ;
#33446=CARTESIAN_POINT ( 'NONE',  ( -22.69296959717488704, 150.3666470947781022, -1.044501570340798269 ) ) ;
#33447=CARTESIAN_POINT ( 'NONE',  ( 0.3060232888392590556, -2.951246395405549450, 0.9280917289473271659 ) ) ;
#33450=CARTESIAN_POINT ( 'NONE',  ( 2.643983731439564444, 108.0685014782224442, 4.389169220726125253 ) ) ;
#33452=CARTESIAN_POINT ( 'NONE',  ( -3.641174103387575745, 120.8049117488720015, 0.2662595081522519669 ) ) ;
#33453=CARTESIAN_POINT ( 'NONE',  ( 3.361239686659836856, -14.56070858809799162, 5.257229516148527182 ) ) ;
#33454=CARTESIAN_POINT ( 'NONE',  ( 17.58003597271441620, 146.9817191466759141, -1.463309413676198156 ) ) ;
#33456=CARTESIAN_POINT ( 'NONE',  ( -2.329084838959003534, 118.9063233352275972, -0.7992829875212341673 ) ) ;
#33457=CARTESIAN_POINT ( 'NONE',  ( 0.7256241136792617175, 104.6144662015456817, 4.780927069918088357 ) ) ;
#33459=CARTESIAN_POINT ( 'NONE',  ( 2.666490510518176649, -13.49855353256042889, 0.05227394649444832425 ) ) ;
#33460=CARTESIAN_POINT ( 'NONE',  ( -4.831581646441107658, 117.6432783874694366, -1.087973816982874320 ) ) ;
#33461=CARTESIAN_POINT ( 'NONE',  ( 5.999396524113651097, 155.3621521873626534, -0.05839828084409114106 ) ) ;
#33463=CARTESIAN_POINT ( 'NONE',  ( 3.009276887026298031, 39.20946620154573736, -1.210121013456480599 ) ) ;
#33464=CARTESIAN_POINT ( 'NONE',  ( 2.163405660033729028, 107.1115117626483055, 4.788046284768042504 ) ) ;
#33466=CARTESIAN_POINT ( 'NONE',  ( 3.168525235803220763, 117.3993833749843532, 1.398852401101993159 ) ) ;
#33468=ADVANCED_FACE ( 'NONE', ( #31329, #22349 ), #41571, .F. ) ;
#33469=CARTESIAN_POINT ( 'NONE',  ( 22.82234304556241256, 150.4043717142618277, 0.2269822898261401878 ) ) ;
#33471=CARTESIAN_POINT ( 'NONE',  ( 1.941303917661279632, -15.39441291017290503, 6.018986302445838099 ) ) ;
#33473=CARTESIAN_POINT ( 'NONE',  ( -0.1605347423948317587, 34.07300127660931111, 0.3172648596225849382 ) ) ;
#33474=CARTESIAN_POINT ( 'NONE',  ( 18.19503446209933983, 151.8090458617612057, 2.356823057848428160 ) ) ;
#33476=CARTESIAN_POINT ( 'NONE',  ( 1.359589829139859152, 24.67768052395325284, 8.332721669750835503 ) ) ;
#33477=CARTESIAN_POINT ( 'NONE',  ( 2.336946977945878690, 117.1813995298343656, -0.5665797218883661390 ) ) ;
#33478=CARTESIAN_POINT ( 'NONE',  ( -3.231430644863531931, 118.6786177306206014, -0.7432888438146499910 ) ) ;
#33480=CARTESIAN_POINT ( 'NONE',  ( -4.800085724567980883, 115.7029491485352537, -1.472342921364584889 ) ) ;
#33481=CARTESIAN_POINT ( 'NONE',  ( -0.0006472084743510491366, 124.6436471961814476, 0.03238895860161190854 ) ) ;
#33483=CARTESIAN_POINT ( 'NONE',  ( -0.2084201458593382406, 5.265951782950084592, 4.622859108429906883 ) ) ;
#33485=CARTESIAN_POINT ( 'NONE',  ( -5.208855653336853742, 31.38455280743060527, -0.6720767434146609487 ) ) ;
#33486=CARTESIAN_POINT ( 'NONE',  ( -4.765768241072703582, 118.5264896598256854, 0.8412120300991379196 ) ) ;
#33487=CARTESIAN_POINT ( 'NONE',  ( 2.739926266261139887, -12.91893237176182296, 0.2921503600690461555 ) ) ;
#33488=CARTESIAN_POINT ( 'NONE',  ( 0.4402454045156525830, 106.4201689084969047, -5.104646014783341457 ) ) ;
#33489=CARTESIAN_POINT ( 'NONE',  ( -11.36388202081354137, 118.9804978796424706, 0.4533785775503093585 ) ) ;
#33490=CARTESIAN_POINT ( 'NONE',  ( -1.149787651882492989, 32.77214111141197606, 3.982284714218304433 ) ) ;
#33493=CARTESIAN_POINT ( 'NONE',  ( 5.332935392244917416, 115.7029491189645825, 0.1065647408284378928 ) ) ;
#33494=CARTESIAN_POINT ( 'NONE',  ( 3.313323393711395948, -15.78004832563367721, 4.785553473879357256 ) ) ;
#33495=CARTESIAN_POINT ( 'NONE',  ( -14.40310572532117384, 154.4775811199918110, 1.681202589455180307 ) ) ;
#33496=CARTESIAN_POINT ( 'NONE',  ( 1.360477052538118681, -3.804838552850991817, 4.419457122809256511 ) ) ;
#33499=CARTESIAN_POINT ( 'NONE',  ( 0.7466139261199012944, 119.9044272045951374, 0.6467483038796006944 ) ) ;
#33500=CARTESIAN_POINT ( 'NONE',  ( -0.02156534543299366835, 156.6359106937186709, 1.079218069903262744 ) ) ;
#33503=CARTESIAN_POINT ( 'NONE',  ( 11.50356673920478201, 154.6851215890897038, -1.708948620147628716 ) ) ;
#33504=CARTESIAN_POINT ( 'NONE',  ( -2.184917017309302878, 118.1205262787358663, -0.7523320384000312666 ) ) ;
#33505=FACE_OUTER_BOUND ( 'NONE', #32824, .T. ) ;
#33506=CARTESIAN_POINT ( 'NONE',  ( 4.241009399425758275, 118.2240432067376759, -0.3200593562746568144 ) ) ;
#33507=CARTESIAN_POINT ( 'NONE',  ( 9.384706802269484172, 123.8909350679826815, -0.3250447036211729368 ) ) ;
#33509=CARTESIAN_POINT ( 'NONE',  ( 3.216867006742271329, -14.81339725456490264, 3.133484537391586944 ) ) ;
#33513=CARTESIAN_POINT ( 'NONE',  ( -1.889208318266999198, 10.27326514537015534, 4.227218769941996968 ) ) ;
#33514=CARTESIAN_POINT ( 'NONE',  ( 8.921947645406950400, 154.9128698100208794, 1.713759150786742458 ) ) ;
#33515=CARTESIAN_POINT ( 'NONE',  ( 2.940994655134018032, 38.68039677755331951, -0.1346318768538148081 ) ) ;
#33516=CARTESIAN_POINT ( 'NONE',  ( 4.617411384770501392, 7.639850289152962048, 0.2838591255797697777 ) ) ;
#33517=CARTESIAN_POINT ( 'NONE',  ( 13.59043555108493884, 150.2357272821285221, 0.3212980696657039004 ) ) ;
#33518=CARTESIAN_POINT ( 'NONE',  ( 5.078986093043053707, 92.04146620154574521, 0.1014902294541244060 ) ) ;
#33523=CARTESIAN_POINT ( 'NONE',  ( -8.789536962982657187, 117.7096669775960862, -0.3419224959890725390 ) ) ;
#33524=CARTESIAN_POINT ( 'NONE',  ( -6.629500982736845120E-14, 97.88346620154572975, -1.984505748321436882E-18 ) ) ;
#33528=CARTESIAN_POINT ( 'NONE',  ( 4.034796628256747120, -3.593727855734754950, 7.433834689985365785 ) ) ;
#33530=CARTESIAN_POINT ( 'NONE',  ( -6.373576640880495633E-14, 50.63946620154572997, 5.832708929232124832E-29 ) ) ;
#33531=DIRECTION ( 'NONE',  ( 0.01997839162482749689, 1.040247600000945640E-18, -0.9998004120163610509 ) ) ;
#33533=CARTESIAN_POINT ( 'NONE',  ( 0.01111760956202519947, 120.5507043431653784, -0.5563706444133252882 ) ) ;
#33534=CARTESIAN_POINT ( 'NONE',  ( -20.08431799972946052, 128.8637844977697569, 0.1093955315764417319 ) ) ;
#33537=CARTESIAN_POINT ( 'NONE',  ( -7.784760752776371362, 122.6240640030675877, -0.1928348868300470975 ) ) ;
#33540=CARTESIAN_POINT ( 'NONE',  ( -0.6448247514297434924, 156.3042436901572216, -0.08557349692115849560 ) ) ;
#33541=CARTESIAN_POINT ( 'NONE',  ( 5.498302128480847983, -14.40662979408034694, 3.384674516772870234 ) ) ;
#33542=CARTESIAN_POINT ( 'NONE',  ( -15.16136233027302183, 154.7927800759015042, 1.480671785937533569 ) ) ;
#33543=CARTESIAN_POINT ( 'NONE',  ( -3.854280124997887746, 21.23357344512866973, -2.551540157904111261 ) ) ;
#33545=CARTESIAN_POINT ( 'NONE',  ( 2.795228999030319628, 116.6385632091030544, 0.2515850966972204561 ) ) ;
#33546=CARTESIAN_POINT ( 'NONE',  ( 2.204990229119355050, -15.43588533350201430, 5.895893715474639585 ) ) ;
#33549=CARTESIAN_POINT ( 'NONE',  ( 0.9102147817015755482, -10.07290960004636737, -0.3509275504499672627 ) ) ;
#33550=CARTESIAN_POINT ( 'NONE',  ( -3.748677658115184386, 116.6824454826851820, -0.2320358872840702358 ) ) ;
#33551=CARTESIAN_POINT ( 'NONE',  ( -4.823516985575233562, 117.8389059115630744, 0.7421444254238848126 ) ) ;
#33553=CARTESIAN_POINT ( 'NONE',  ( 8.748582098294324538, 117.8797259988493096, 0.6463030221440396739 ) ) ;
#33554=CARTESIAN_POINT ( 'NONE',  ( -9.240212912644894416, 121.6705353891887995, 1.055487293716822039 ) ) ;
#33556=CARTESIAN_POINT ( 'NONE',  ( 13.87194369518284809, 121.7708260186165177, 1.632391212143506021 ) ) ;
#33557=CARTESIAN_POINT ( 'NONE',  ( 19.34566907036573014, 149.3473233412102275, -1.724881794388704703 ) ) ;
#33558=CARTESIAN_POINT ( 'NONE',  ( -0.6538259107469485132, -10.21753563294075384, 0.7251761174241220242 ) ) ;
#33559=CARTESIAN_POINT ( 'NONE',  ( -5.844526503020657238, 118.0670013439590491, -1.005764768584936686 ) ) ;
#33562=CARTESIAN_POINT ( 'NONE',  ( 5.190856860529054373, 105.1222051271263780, 1.277391616506039274 ) ) ;
#33563=CARTESIAN_POINT ( 'NONE',  ( 8.590326429123150476, 154.7538831414287870, -1.096848044820071921 ) ) ;
#33564=CARTESIAN_POINT ( 'NONE',  ( -11.82813386268903955, 130.3161362890850512, -0.2363542639706541493 ) ) ;
#33565=VERTEX_POINT ( 'NONE', #2805 ) ;
#33566=CARTESIAN_POINT ( 'NONE',  ( -12.38071862475251450, 124.1810962131942517, -1.797420231217670139 ) ) ;
#33567=CARTESIAN_POINT ( 'NONE',  ( 2.573200380748495331, -15.70867456196409151, 5.149826986703908815 ) ) ;
#33568=DIRECTION ( 'NONE',  ( 0.9998004120163608288, 0.000000000000000000, 0.01997839162482736852 ) ) ;
#33569=CARTESIAN_POINT ( 'NONE',  ( -4.441329932981612494, 118.1268108493847109, -0.7296998205460351050 ) ) ;
#33571=CARTESIAN_POINT ( 'NONE',  ( -6.527452395418614125E-14, 72.48346620154573827, -8.020333044904917549E-18 ) ) ;
#33572=CARTESIAN_POINT ( 'NONE',  ( 6.586386431196439517, 120.2999964176511014, 1.183541128842728885 ) ) ;
#33573=DIRECTION ( 'NONE',  ( 4.017660918040594346E-17, -1.000000000000000000, -2.376309959284834438E-19 ) ) ;
#33574=CARTESIAN_POINT ( 'NONE',  ( 16.31694223957253698, 121.4173703750124531, 0.3260513381110076714 ) ) ;
#33575=CARTESIAN_POINT ( 'NONE',  ( 7.667154907385915763, 6.987472373264454362, 3.492918021822637442 ) ) ;
#33576=CARTESIAN_POINT ( 'NONE',  ( 10.60367000503885748, 126.1357510980948575, 0.6849044484263044907 ) ) ;
#33578=CARTESIAN_POINT ( 'NONE',  ( 17.61824099940326604, 125.1652531886817172, -0.6886689253619217022 ) ) ;
#33583=CARTESIAN_POINT ( 'NONE',  ( -0.8998519745136789316, 116.4604358222411236, 0.05108568132534212214 ) ) ;
#33586=CARTESIAN_POINT ( 'NONE',  ( -5.679082498912885413, 121.0114208266025599, -0.6118695118735946181 ) ) ;
#33589=CARTESIAN_POINT ( 'NONE',  ( -2.769557799161974199, 120.9068798055765370, -0.2367794989410799689 ) ) ;
#33590=CARTESIAN_POINT ( 'NONE',  ( 4.077043646397369159, -14.32506836492906999, 4.807529146363894057 ) ) ;
#33591=CARTESIAN_POINT ( 'NONE',  ( -22.28974849274172598, 149.2301036976659816, 0.9981255638314735501 ) ) ;
#33593=CARTESIAN_POINT ( 'NONE',  ( 22.73177750447365497, 137.3553536570635742, 0.5243227317837022561 ) ) ;
#33595=CARTESIAN_POINT ( 'NONE',  ( 4.219463811995017188, -1.205994944679912306, -1.932895124392335573 ) ) ;
#33596=CARTESIAN_POINT ( 'NONE',  ( -11.73662545640882904, 118.7267541726749869, -0.2503127652027325456 ) ) ;
#33597=CARTESIAN_POINT ( 'NONE',  ( 5.078986093043053707, 81.62746620154572952, 0.1014902294541237954 ) ) ;
#33600=CARTESIAN_POINT ( 'NONE',  ( -5.506994448060305025, 119.6850719548569941, 0.8864364066137871978 ) ) ;
#33601=CARTESIAN_POINT ( 'NONE',  ( 4.168288449772385995, -6.568960759998498489, 2.029292378399509378 ) ) ;
#33602=CARTESIAN_POINT ( 'NONE',  ( -0.008308726997799834729, 117.3658353995175503, 0.4158026747930030353 ) ) ;
#33604=CARTESIAN_POINT ( 'NONE',  ( 4.850700283611232067, 158.3075559295907055, -1.526604748539100775 ) ) ;
#33606=CARTESIAN_POINT ( 'NONE',  ( 1.463615122064738427, -3.970138727222522590, -4.384008014421088895 ) ) ;
#33607=CARTESIAN_POINT ( 'NONE',  ( 0.01443894962456205439, 159.4760848062415732, -0.7225840825867285711 ) ) ;
#33609=CARTESIAN_POINT ( 'NONE',  ( -8.625872078176357149, 123.3364012560002578, 0.04702935286775016682 ) ) ;
#33611=CARTESIAN_POINT ( 'NONE',  ( 4.984919470525341012, -14.71752327621497791, 4.178560682339194976 ) ) ;
#33614=CARTESIAN_POINT ( 'NONE',  ( -4.943847941134515089, 113.9634239269208393, -2.116083417004583467 ) ) ;
#33615=ORIENTED_EDGE ( 'NONE', *, *, #11287, .T. ) ;
#33616=CARTESIAN_POINT ( 'NONE',  ( 12.03045567952066364, 122.8144071692085504, 1.784322758991244040 ) ) ;
#33619=AXIS2_PLACEMENT_3D ( 'NONE', #32765, #5953, #22304 ) ;
#33621=CARTESIAN_POINT ( 'NONE',  ( -21.83270838041260120, 150.5404744109896171, 0.8586010584139895929 ) ) ;
#33622=CARTESIAN_POINT ( 'NONE',  ( -3.310625167495538257, 6.824969433126684137, -7.744297517547710896 ) ) ;
#33623=CARTESIAN_POINT ( 'NONE',  ( 3.199116795994500606, 156.2293907256693331, 0.9954876105832139999 ) ) ;
#33624=DIRECTION ( 'NONE',  ( -5.206863593109713661E-17, 1.000000000000000000, -1.077750396879097183E-30 ) ) ;
#33626=CARTESIAN_POINT ( 'NONE',  ( 18.31971715989119076, 125.1624627582897915, -0.2149060778942796235 ) ) ;
#33628=CIRCLE ( 'NONE', #26805, 5.588000000000006295 ) ;
#33634=CARTESIAN_POINT ( 'NONE',  ( -4.394434931943050238, 118.1841795841535827, 0.4163878308331336875 ) ) ;
#33635=CARTESIAN_POINT ( 'NONE',  ( 1.392235599252770184, 106.3000011757766003, -5.100451643702543336 ) ) ;
#33636=ORIENTED_EDGE ( 'NONE', *, *, #10346, .F. ) ;
#33638=CARTESIAN_POINT ( 'NONE',  ( -6.112386360759682447, 119.5658119500284755, -1.253701994526288832 ) ) ;
#33639=CARTESIAN_POINT ( 'NONE',  ( -7.669310211018488310, 124.7206709383052043, -0.1531702926821040256 ) ) ;
#33640=CARTESIAN_POINT ( 'NONE',  ( 4.459538917479417997, 118.1136197194245625, 0.7514127147595077716 ) ) ;
#33641=CARTESIAN_POINT ( 'NONE',  ( -1.517991627498799900, 120.5919059741422217, -0.3392643659851172222 ) ) ;
#33642=CARTESIAN_POINT ( 'NONE',  ( -0.7773321051407233728, 115.7028436671041192, -1.754947197622949817 ) ) ;
#33643=CARTESIAN_POINT ( 'NONE',  ( 0.4423781608754945860, 117.9496046456311120, -1.391511169922456270 ) ) ;
#33644=CARTESIAN_POINT ( 'NONE',  ( -4.349660437102230048, 31.17966527223318707, -1.615541842050199461 ) ) ;
#33645=CARTESIAN_POINT ( 'NONE',  ( -3.288791919378307504, 156.3062290909284116, -1.149731754608032563 ) ) ;
#33646=EDGE_CURVE ( 'NONE', #38078, #36646, #24207, .T. ) ;
#33648=CARTESIAN_POINT ( 'NONE',  ( -3.743815577281075058, 31.31851751214970037, -0.6207396561878217867 ) ) ;
#33649=CARTESIAN_POINT ( 'NONE',  ( 7.878666962137408802, 122.2304107671078981, -0.4668939115120620542 ) ) ;
#33650=CARTESIAN_POINT ( 'NONE',  ( -9.093386426035655390, 153.9805809586646888, -0.007641094020508640110 ) ) ;
#33651=CARTESIAN_POINT ( 'NONE',  ( 5.078986093043052819, 101.1854662015457365, 0.1014902294541237954 ) ) ;
#33652=CARTESIAN_POINT ( 'NONE',  ( 4.821777392514684735, 117.1414559920645644, 0.5894805283384126904 ) ) ;
#33654=CARTESIAN_POINT ( 'NONE',  ( 3.411744169395244164, -14.91921274028452871, 2.011823270444000666 ) ) ;
#33655=CARTESIAN_POINT ( 'NONE',  ( -10.61219202125007399, 121.9340018749941663, 1.210411277014657561 ) ) ;
#33656=CARTESIAN_POINT ( 'NONE',  ( 0.6771123631923940955, -5.471153235863896569, -0.7014129483058207937 ) ) ;
#33657=CARTESIAN_POINT ( 'NONE',  ( -13.14908049612679974, 156.9583929045107595, -0.9825115876436353313 ) ) ;
#33658=CARTESIAN_POINT ( 'NONE',  ( -0.3362158861861603287, -7.698726726604804504, -0.9163890413163552351 ) ) ;
#33661=CARTESIAN_POINT ( 'NONE',  ( 5.229314312453159808, 116.0897965414613964, 1.239798673375258842 ) ) ;
#33663=CARTESIAN_POINT ( 'NONE',  ( -0.009747742627877935620, 156.3581291470199233, 0.4878169013068173743 ) ) ;
#33665=CARTESIAN_POINT ( 'NONE',  ( 2.771648496353774860, -15.01054376081380148, 5.729243832102374867 ) ) ;
#33666=CARTESIAN_POINT ( 'NONE',  ( 10.73673663838188475, 123.5542795626547417, -1.004701191943994765 ) ) ;
#33668=CARTESIAN_POINT ( 'NONE',  ( -8.358437701610750281, 156.6436466068687423, -2.074018175080057702 ) ) ;
#33669=CARTESIAN_POINT ( 'NONE',  ( 3.489354382163187385, 115.7029491485452866, 1.632628334074333720 ) ) ;
#33670=CARTESIAN_POINT ( 'NONE',  ( 2.946624452826990925, -14.63926610985447141, 4.195571020465345136 ) ) ;
#33673=CARTESIAN_POINT ( 'NONE',  ( 1.597555633484664339, 120.9451058151398399, -0.06333991727891964685 ) ) ;
#33675=CARTESIAN_POINT ( 'NONE',  ( 3.174067013697414730, 118.4902560533893592, 0.8904294910640483396 ) ) ;
#33676=CARTESIAN_POINT ( 'NONE',  ( 3.402909602042748283, 108.3861600575998949, 4.100009543453226435 ) ) ;
#33680=CARTESIAN_POINT ( 'NONE',  ( 22.52215935351586751, 150.7865899205276321, 0.2217371156544979960 ) ) ;
#33682=CARTESIAN_POINT ( 'NONE',  ( 2.054492031761760984, -15.24248389176698026, 5.952799576744645549 ) ) ;
#33684=FACE_OUTER_BOUND ( 'NONE', #33065, .T. ) ;
#33685=CARTESIAN_POINT ( 'NONE',  ( -0.02969037535081452128, 158.7301711276701894, 1.485827791648137275 ) ) ;
#33687=CARTESIAN_POINT ( 'NONE',  ( 1.932697321913770416, 19.28018055242734619, -8.218723488459904303 ) ) ;
#33688=CARTESIAN_POINT ( 'NONE',  ( 5.539598496142141393, 117.7704119632382032, -0.8150624102158662287 ) ) ;
#33689=CARTESIAN_POINT ( 'NONE',  ( -3.894863181655659368, 121.5791280715047122, -0.3237234463424496500 ) ) ;
#33692=CARTESIAN_POINT ( 'NONE',  ( -3.966471221021101723, 104.6144662015457243, 2.768186473823242011 ) ) ;
#33693=CARTESIAN_POINT ( 'NONE',  ( -4.319812470756069445, 11.96289413176387129, -1.686699837767231536 ) ) ;
#33696=CARTESIAN_POINT ( 'NONE',  ( 3.191397606779386109, -14.26579101578730224, 3.890870127686782087 ) ) ;
#33697=CARTESIAN_POINT ( 'NONE',  ( 4.548929788228058158, 119.7344140837147819, -0.3435137807816314726 ) ) ;
#33698=CARTESIAN_POINT ( 'NONE',  ( -9.616121018674380849, 118.2964180356302961, 0.4479623223841152635 ) ) ;
#33700=CARTESIAN_POINT ( 'NONE',  ( -4.062624110921462695, 30.12807731062649452, 3.861355649616186270 ) ) ;
#33704=CARTESIAN_POINT ( 'NONE',  ( -3.055407127328060746, 104.6144662015402247, -4.375668876421388909 ) ) ;
#33705=CARTESIAN_POINT ( 'NONE',  ( 4.901850132730561249, -15.30225767492697564, -0.5056678198325348372 ) ) ;
#33706=CARTESIAN_POINT ( 'NONE',  ( -12.49437611722099994, 122.1796674805547980, 1.295212323302053159 ) ) ;
#33707=CARTESIAN_POINT ( 'NONE',  ( -3.594857975007920814, -7.703025367003809798, -2.923569511714296798 ) ) ;
#33708=ORIENTED_EDGE ( 'NONE', *, *, #37510, .F. ) ;
#33712=CARTESIAN_POINT ( 'NONE',  ( 2.364009027793788853, 119.4803856251332945, 0.6315868319338826531 ) ) ;
#33714=CARTESIAN_POINT ( 'NONE',  ( -16.69554899298730177, 147.2809512400332608, 1.108146210772844809 ) ) ;
#33716=CARTESIAN_POINT ( 'NONE',  ( 0.01023306027083611264, 119.5380416804913324, -0.5121041807152043601 ) ) ;
#33717=CARTESIAN_POINT ( 'NONE',  ( -10.23541510771069696, 120.3038588096988803, -1.551695437301547020 ) ) ;
#33719=CARTESIAN_POINT ( 'NONE',  ( 4.269777116393453475, 118.2237272103456007, -0.2881531109393317136 ) ) ;
#33720=CARTESIAN_POINT ( 'NONE',  ( 5.897637645108018134, 121.3687970875902806, -0.2476274089428440461 ) ) ;
#33722=CARTESIAN_POINT ( 'NONE',  ( 3.283982329611080608, -15.09957111342241731, 3.272784416514652239 ) ) ;
#33724=CARTESIAN_POINT ( 'NONE',  ( -4.815275531776046947, 117.4047736241515736, 1.012442419610674271 ) ) ;
#33727=AXIS2_PLACEMENT_3D ( 'NONE', #8065, #37666, #2319 ) ;
#33728=CARTESIAN_POINT ( 'NONE',  ( 4.623297697159335584, 3.588818502778304609, 0.3943307014320480697 ) ) ;
#33729=CARTESIAN_POINT ( 'NONE',  ( 16.06787389343314132, 149.3012944676311804, 2.013231008103361308 ) ) ;
#33730=CARTESIAN_POINT ( 'NONE',  ( -2.475166694215277907, 30.06136823196653296, 2.243632805404280450 ) ) ;
#33731=CARTESIAN_POINT ( 'NONE',  ( -3.106711772599575649, 110.6400929099055332, 3.287732168264224430 ) ) ;
#33732=CARTESIAN_POINT ( 'NONE',  ( -4.012847786888796620, 11.73797844546971270, -2.294585225469591983 ) ) ;
#33733=CARTESIAN_POINT ( 'NONE',  ( 15.21722582537762847, 143.4245298570049840, 0.3558394363636830926 ) ) ;
#33736=CARTESIAN_POINT ( 'NONE',  ( -2.166455499162651233, 116.2749100498806172, -0.2279745749322064641 ) ) ;
#33739=CARTESIAN_POINT ( 'NONE',  ( -1.814775304374550924, 106.5834530906598445, 4.954023504585296500 ) ) ;
#33741=CARTESIAN_POINT ( 'NONE',  ( 6.696816702757251605, -2.959147833993511778, 5.158690622954519078 ) ) ;
#33746=CARTESIAN_POINT ( 'NONE',  ( -13.35275951139071005, 156.9675713949798421, 0.1105600748258541571 ) ) ;
#33747=ORIENTED_EDGE ( 'NONE', *, *, #24850, .T. ) ;
#33749=CARTESIAN_POINT ( 'NONE',  ( -6.992180608686842547, 121.9518168112129644, -0.1549296657180008197 ) ) ;
#33750=ORIENTED_EDGE ( 'NONE', *, *, #3337, .T. ) ;
#33752=CARTESIAN_POINT ( 'NONE',  ( -9.083767709417969627, 124.1603612693012053, -0.1367774190269939183 ) ) ;
#33753=CARTESIAN_POINT ( 'NONE',  ( 4.983883817524661808, -15.00518790705197780, 4.081033524500047527 ) ) ;
#33754=CARTESIAN_POINT ( 'NONE',  ( -9.293546136053135953, 157.2521837264336853, 1.575842917768122797 ) ) ;
#33755=CARTESIAN_POINT ( 'NONE',  ( 10.68516669180060319, 157.9381250348597234, 0.6779181152352151685 ) ) ;
#33756=CARTESIAN_POINT ( 'NONE',  ( 22.27457866854806667, 149.8733841865972920, -0.8555749715664360266 ) ) ;
#33757=CARTESIAN_POINT ( 'NONE',  ( -3.290491044589036740, 30.52917213649525507, -3.264312889705288878 ) ) ;
#33758=CARTESIAN_POINT ( 'NONE',  ( -22.49140923449514418, 150.7830971219523519, -0.7772193431698345423 ) ) ;
#33760=CARTESIAN_POINT ( 'NONE',  ( 4.812098290572522252, 117.4080384897477813, 1.196841167122759897 ) ) ;
#33763=CARTESIAN_POINT ( 'NONE',  ( -8.771991783980059409, 117.8544350838303103, 0.2656743787463436979 ) ) ;
#33764=CARTESIAN_POINT ( 'NONE',  ( -12.98417868877910131, 125.9520529675768898, 1.303718779035868192 ) ) ;
#33766=CARTESIAN_POINT ( 'NONE',  ( 19.87863739466932600, 147.4002846799066333, -1.728157425434577288 ) ) ;
#33767=CARTESIAN_POINT ( 'NONE',  ( -0.2718671964776636085, -13.46374167387040366, -0.9358251418597670623 ) ) ;
#33768=CARTESIAN_POINT ( 'NONE',  ( -16.99346516877630719, 153.7580772870718988, -2.083520914717074124 ) ) ;
#33771=CARTESIAN_POINT ( 'NONE',  ( 0.01887828017110892292, 156.5412816204240301, -0.9447463363288812754 ) ) ;
#33774=CARTESIAN_POINT ( 'NONE',  ( -10.38552121992541366, 122.0805278159965610, -1.592441429402149833 ) ) ;
#33775=CARTESIAN_POINT ( 'NONE',  ( 4.747814429275453385, -15.55672444834840817, 1.946379828023123482 ) ) ;
#33777=CARTESIAN_POINT ( 'NONE',  ( -4.535012393063357017, 118.1058069998952362, -0.6732513337841837808 ) ) ;
#33781=CARTESIAN_POINT ( 'NONE',  ( 18.11471409803301214, 146.9188445454784357, 2.346026295494533453 ) ) ;
#33782=LINE ( 'NONE', #10133, #10015 ) ;
#33783=CARTESIAN_POINT ( 'NONE',  ( 16.86202032626302483, 155.2029898760372646, 0.3369432954968345495 ) ) ;
#33784=CARTESIAN_POINT ( 'NONE',  ( -8.412017540776835389, 12.59877214424737524, 0.8828606482577823211 ) ) ;
#33785=CARTESIAN_POINT ( 'NONE',  ( -0.006534791579925431325, 156.3267223255430167, 0.3270276925529296275 ) ) ;
#33787=CARTESIAN_POINT ( 'NONE',  ( 15.42041356977095745, 121.5363848317736739, -0.5399810379570647578 ) ) ;
#33791=CARTESIAN_POINT ( 'NONE',  ( -1.817820247522510924, 116.4909138135563040, 0.03564457049243165837 ) ) ;
#33794=CARTESIAN_POINT ( 'NONE',  ( 5.842028984958227866, 121.2385196568167203, -0.2395641771394423913 ) ) ;
#33797=CARTESIAN_POINT ( 'NONE',  ( 0.1233530899022908384, 118.7629491485454025, -1.274984814944074785 ) ) ;
#33798=CARTESIAN_POINT ( 'NONE',  ( -15.59067940631276272, 147.5518517437054982, -0.7624272054715743874 ) ) ;
#33799=CARTESIAN_POINT ( 'NONE',  ( 2.939725130288969979, -14.94165859211278580, 5.651657094137466864 ) ) ;
#33800=CARTESIAN_POINT ( 'NONE',  ( -21.76596270643833364, 150.3096123636779566, 1.000581967439477360 ) ) ;
#33802=CARTESIAN_POINT ( 'NONE',  ( 6.901437262003186746, 117.1762911274595496, 0.2238905109288660267 ) ) ;
#33804=CARTESIAN_POINT ( 'NONE',  ( 3.102408547967445696, -0.5812848888516047863, -3.453265078539196509 ) ) ;
#33805=CARTESIAN_POINT ( 'NONE',  ( -14.89944180985308364, 120.3262451489332818, -0.3144022614128132997 ) ) ;
#33809=CARTESIAN_POINT ( 'NONE',  ( 5.474781159379864093, 119.6919804704018588, 1.105622938617728090 ) ) ;
#33810=CARTESIAN_POINT ( 'NONE',  ( 4.064497669612420871, 2.951628549105334454, 2.233594334442648766 ) ) ;
#33811=CARTESIAN_POINT ( 'NONE',  ( 9.366440581936233301, 118.7255599110314961, 1.127239873969282824 ) ) ;
#33814=CARTESIAN_POINT ( 'NONE',  ( 20.18437654629502020, 141.3454246894093274, -1.633934361538418090 ) ) ;
#33815=CARTESIAN_POINT ( 'NONE',  ( -4.567530434605131084, -10.44214056487004250, 0.7003524306260878740 ) ) ;
#33816=CARTESIAN_POINT ( 'NONE',  ( -15.23381565553120254, 121.5932973536894934, -1.241876992062232121 ) ) ;
#33819=CARTESIAN_POINT ( 'NONE',  ( -5.280870373041201660, 121.3253820001177417, 0.01155303659100765171 ) ) ;
#33820=CARTESIAN_POINT ( 'NONE',  ( 3.039728791924208195, -15.34324946256290723, 5.681930179901951483 ) ) ;
#33822=CARTESIAN_POINT ( 'NONE',  ( -5.084954045839870318, 114.9389534559779946, -1.737685838023535601 ) ) ;
#33824=CARTESIAN_POINT ( 'NONE',  ( 12.25516334840909138, 122.6846661264431191, 1.808440497450061413 ) ) ;
#33829=CARTESIAN_POINT ( 'NONE',  ( -3.136615966272743083, 159.3365417412370562, 0.7296721229192901781 ) ) ;
#33830=CARTESIAN_POINT ( 'NONE',  ( 8.344183819546742598, 4.025392264050483782, -1.191670311180863528 ) ) ;
#33831=CARTESIAN_POINT ( 'NONE',  ( 5.192366003377009598, 121.0352659167314755, 0.5503205103620257832 ) ) ;
#33833=CARTESIAN_POINT ( 'NONE',  ( 18.44051311885884914, 154.1649927243852858, -0.3121108635588941138 ) ) ;
#33836=FACE_OUTER_BOUND ( 'NONE', #24000, .T. ) ;
#33839=CARTESIAN_POINT ( 'NONE',  ( -4.242438329162251165, 118.2242328442825681, 0.3186281974751150048 ) ) ;
#33840=CARTESIAN_POINT ( 'NONE',  ( 4.163769306296988937, 111.0901538136045161, -3.043919495886841631 ) ) ;
#33842=VERTEX_POINT ( 'NONE', #8001 ) ;
#33844=CARTESIAN_POINT ( 'NONE',  ( 4.224406003510333463, 119.3195559688346066, -0.7598301222401262489 ) ) ;
#33845=CARTESIAN_POINT ( 'NONE',  ( -5.246745461248100817, 116.0761519159950552, -1.241752167516083194 ) ) ;
#33846=CARTESIAN_POINT ( 'NONE',  ( 4.397138658150465673, 118.1792182539645353, 0.5669217176520113810 ) ) ;
#33847=CARTESIAN_POINT ( 'NONE',  ( -8.969937932052687302, 123.1852847016406685, -0.8267063328025512359 ) ) ;
#33849=CARTESIAN_POINT ( 'NONE',  ( 4.410581516669115132, 117.9496053154420423, -1.006313971990577372 ) ) ;
#33851=CARTESIAN_POINT ( 'NONE',  ( 3.580579253266004347, 108.6681208952157078, -3.986884027299105071 ) ) ;
#33852=CARTESIAN_POINT ( 'NONE',  ( -0.5759676376930302766, 120.3589971203204669, -0.3694376532493067189 ) ) ;
#33853=CARTESIAN_POINT ( 'NONE',  ( 4.141126571459865069, 104.6144662015457243, 4.161112031276615220 ) ) ;
#33854=CARTESIAN_POINT ( 'NONE',  ( -3.321756749363752537, 31.07797388775926350, -0.5319413560150946241 ) ) ;
#33856=CARTESIAN_POINT ( 'NONE',  ( -13.59405114508080992, 150.2694781165900793, -0.07689127809379422973 ) ) ;
#33857=CARTESIAN_POINT ( 'NONE',  ( 4.980754117605273201, 117.5239965563486919, 0.8160915654990145152 ) ) ;
#33858=CARTESIAN_POINT ( 'NONE',  ( 22.92073667220923738, 148.8788797244430384, 1.430292205038965037 ) ) ;
#33860=CARTESIAN_POINT ( 'NONE',  ( 3.178195937486941958, -14.44740043277138675, 1.484392166672811930 ) ) ;
#33861=CARTESIAN_POINT ( 'NONE',  ( 21.51828093163809896, 145.9698620541949765, -1.394984360948490210 ) ) ;
#33862=CARTESIAN_POINT ( 'NONE',  ( -0.5200570697821880195, 119.3183582894065893, 0.5597423419424876201 ) ) ;
#33863=CARTESIAN_POINT ( 'NONE',  ( -0.4659799999662124215, -3.540968264561009882, -0.8578381542037093466 ) ) ;
#33864=CARTESIAN_POINT ( 'NONE',  ( -23.01936977803475770, 148.9204423966469335, -1.315221278248082548 ) ) ;
#33866=CARTESIAN_POINT ( 'NONE',  ( -0.2236011429256814231, 15.24623788552754888, -0.9474642044971398613 ) ) ;
#33867=EDGE_LOOP ( 'NONE', ( #17810, #10445, #9815, #21361 ) ) ;
#33870=CARTESIAN_POINT ( 'NONE',  ( -7.092669859378217367, 121.9239394581621809, 0.2697480494961537190 ) ) ;
#33871=CARTESIAN_POINT ( 'NONE',  ( 4.995837928452414367, -12.01622098921958859, 1.211524600846092481 ) ) ;
#33872=CARTESIAN_POINT ( 'NONE',  ( 4.353257824593153025, 120.2039194668847699, -0.6262808803686855663 ) ) ;
#33874=CARTESIAN_POINT ( 'NONE',  ( 3.605593953823826414, 115.7029500407100926, 1.621980936835669018 ) ) ;
#33877=CARTESIAN_POINT ( 'NONE',  ( 3.370512099616890467, -13.86485436517860492, 3.147780574041331825 ) ) ;
#33878=FACE_OUTER_BOUND ( 'NONE', #37284, .T. ) ;
#33879=EDGE_CURVE ( 'NONE', #34211, #17903, #34847, .T. ) ;
#33880=CARTESIAN_POINT ( 'NONE',  ( 15.26897697690599109, 148.0131224598485744, 0.1773810520481279573 ) ) ;
#33882=CARTESIAN_POINT ( 'NONE',  ( 12.93098116229895211, 122.2940260782629451, 1.802317002068888785 ) ) ;
#33883=CARTESIAN_POINT ( 'NONE',  ( 3.410149960233146427, 109.2372012348956645, 3.913055101880209552 ) ) ;
#33885=CARTESIAN_POINT ( 'NONE',  ( 0.01289612358321986542, 159.5048567107479585, -0.6453747585945881493 ) ) ;
#33886=CARTESIAN_POINT ( 'NONE',  ( 22.65693159617090657, 137.2763855621842026, 0.2353725067100886914 ) ) ;
#33887=CARTESIAN_POINT ( 'NONE',  ( -3.174366308152011040, 69.94346620154573202, -0.06343139340882729404 ) ) ;
#33888=CARTESIAN_POINT ( 'NONE',  ( 1.727570783967031787, -15.53207390529406950, 5.484086197889097569 ) ) ;
#33890=CARTESIAN_POINT ( 'NONE',  ( -3.113414239748029111, 30.98679946927233431, 0.04088859964249514506 ) ) ;
#33891=CARTESIAN_POINT ( 'NONE',  ( 9.223174309219125178, 157.2521837264336853, 1.945851059610182565 ) ) ;
#33892=ORIENTED_EDGE ( 'NONE', *, *, #24021, .T. ) ;
#33893=CARTESIAN_POINT ( 'NONE',  ( -6.605212570472872358, 13.46189590645272460, 5.224192399652773489 ) ) ;
#33894=CARTESIAN_POINT ( 'NONE',  ( -8.578767457482950221, 118.6581505231196161, -1.156225727184389207 ) ) ;
#33895=CARTESIAN_POINT ( 'NONE',  ( -2.027571083617168313, 109.8863472468248119, -3.714074494666526505 ) ) ;
#33897=FACE_OUTER_BOUND ( 'NONE', #39321, .T. ) ;
#33898=CARTESIAN_POINT ( 'NONE',  ( -0.003708075273252911530, 123.1683257372384901, 0.1855672496570451302 ) ) ;
#33899=B_SPLINE_CURVE_WITH_KNOTS ( 'NONE', 3,
 ( #9835, #693, #35626, #39234, #10252, #36466, #29431, #25807, #16211, #35838, #32630, #36257, #13665, #16006 ),
 .UNSPECIFIED., .F., .F.,
 ( 4, 1, 1, 1, 2, 1, 1, 1, 1, 1, 4 ),
 ( 0.2031000000004874739, 0.2063375000004613602, 0.2095750000004352187, 0.2128125000004091050, 0.2160500000003829635, 0.2667374999999738705, 0.3174249999995648608, 0.3681124999991557400, 0.4187999999987466193, 0.5201749999979284889, 0.6215499999971102474 ),
 .UNSPECIFIED. ) ;
#33900=CIRCLE ( 'NONE', #15515, 3.175000000000001155 ) ;
#33901=CARTESIAN_POINT ( 'NONE',  ( 0.7007450612751181529, 9.901275517365906609, -4.597291952374415125 ) ) ;
#33903=CARTESIAN_POINT ( 'NONE',  ( -5.206518307116178690, 115.6909491485453003, 1.025009323720317500 ) ) ;
#33904=CARTESIAN_POINT ( 'NONE',  ( 3.119424175201863214, -14.34824051949108714, 4.229366443754182470 ) ) ;
#33906=CARTESIAN_POINT ( 'NONE',  ( 4.368052411777142652, 123.4689364668338385, 0.008193521294100057292 ) ) ;
#33907=CARTESIAN_POINT ( 'NONE',  ( -3.958300029084214522, 28.23836431654050472, 1.224951011016432778 ) ) ;
#33908=CARTESIAN_POINT ( 'NONE',  ( -2.027701166914974706, 115.7029486569566785, 1.637676004427128351 ) ) ;
#33910=CARTESIAN_POINT ( 'NONE',  ( -4.648735762212839795, 104.6144662015457527, -1.307085752955095437 ) ) ;
#33911=CARTESIAN_POINT ( 'NONE',  ( 3.970714270704740922, -15.74271870963887743, 3.976543152134710990 ) ) ;
#33912=CARTESIAN_POINT ( 'NONE',  ( -17.13393749618838413, 131.5760549582342094, 1.627836260134054802 ) ) ;
#33913=CARTESIAN_POINT ( 'NONE',  ( -0.9745549951769645336, 13.24125360461694001, -0.07243667530571006041 ) ) ;
#33917=CARTESIAN_POINT ( 'NONE',  ( 2.302803873444530858, 118.9955205646042344, 0.7292456921539738346 ) ) ;
#33918=CARTESIAN_POINT ( 'NONE',  ( -5.165015969722906775, 120.6777149489875569, 0.5489573293230839424 ) ) ;
#33920=CARTESIAN_POINT ( 'NONE',  ( 4.619030643355426236, 118.0409184362119532, -0.6363634065985189769 ) ) ;
#33921=CARTESIAN_POINT ( 'NONE',  ( 17.20821608673143999, 140.2562023718666353, -1.644530994948828706 ) ) ;
#33922=CARTESIAN_POINT ( 'NONE',  ( -19.97852701226068461, 149.8444905389382882, -2.417717604095676265 ) ) ;
#33926=CARTESIAN_POINT ( 'NONE',  ( 4.157985977180885584, 118.2391351103022430, -0.2336046903670694896 ) ) ;
#33927=CARTESIAN_POINT ( 'NONE',  ( 9.286476516977916873, 123.9149913687586064, -0.2326040378870055936 ) ) ;
#33929=CARTESIAN_POINT ( 'NONE',  ( 3.092086460852839114, -14.79905751219236265, 3.633802299706017980 ) ) ;
#33934=EDGE_CURVE ( 'NONE', #40008, #2172, #13452, .T. ) ;
#33935=CARTESIAN_POINT ( 'NONE',  ( 0.5082173563136543892, -13.24086043563247728, -4.610200172643777350 ) ) ;
#33936=CARTESIAN_POINT ( 'NONE',  ( 10.62607977745477505, 123.8807653058400575, 1.354828998092944659 ) ) ;
#33937=CARTESIAN_POINT ( 'NONE',  ( -3.222454021317843864, 28.56592918162606054, 1.039686905332308342 ) ) ;
#33938=CARTESIAN_POINT ( 'NONE',  ( -0.6941271473899978117, 106.1608668108878817, 5.200699783222979988 ) ) ;
#33939=CARTESIAN_POINT ( 'NONE',  ( -4.478778176974228309, 3.316883148187759645, 1.141857468124592101 ) ) ;
#33940=CARTESIAN_POINT ( 'NONE',  ( 2.896036792256140302, 156.0891579660883508, 0.1428477814196380258 ) ) ;
#33943=CARTESIAN_POINT ( 'NONE',  ( 2.180768841371605316, 116.2301253052036145, -0.09025952647190275957 ) ) ;
#33946=CARTESIAN_POINT ( 'NONE',  ( -1.205614202975156202, 106.0882118856389980, 5.200918596848653763 ) ) ;
#33948=CARTESIAN_POINT ( 'NONE',  ( 7.077328715112659374, 6.763356510963684620, 4.580356461215433939 ) ) ;
#33953=CARTESIAN_POINT ( 'NONE',  ( 0.008700780990288231598, 121.2597428844645293, -0.4354226598342533783 ) ) ;
#33954=CARTESIAN_POINT ( 'NONE',  ( -9.739177221546430729, 118.0756159837034716, 0.1634508798788867900 ) ) ;
#33958=TOROIDAL_SURFACE ( 'NONE', #16252, 3.683000000000000718, 0.5080000000000000071 ) ;
#33961=CARTESIAN_POINT ( 'NONE',  ( -8.487687333566288572, 123.3253871723413368, -0.1696041924978711757 ) ) ;
#33962=CARTESIAN_POINT ( 'NONE',  ( 2.853125897180512460, -15.37704012655945185, 5.752692477956393269 ) ) ;
#33963=CARTESIAN_POINT ( 'NONE',  ( -13.44735859403588840, 121.7711344121973411, 1.154596522737721953 ) ) ;
#33965=CARTESIAN_POINT ( 'NONE',  ( 18.94714202558204619, 128.6554162386474047, -0.8647899522199679057 ) ) ;
#33967=CARTESIAN_POINT ( 'NONE',  ( -15.13553065988589275, 156.1345691653134509, -0.5893329488795887583 ) ) ;
#33971=CARTESIAN_POINT ( 'NONE',  ( -10.63443090528977031, 122.8495954190337898, 1.101905667251144472 ) ) ;
#33973=CARTESIAN_POINT ( 'NONE',  ( 7.611130975157075262, 119.9600249249614592, -1.076879093209133442 ) ) ;
#33974=CARTESIAN_POINT ( 'NONE',  ( -12.03559625110899312, 156.5645100661158153, -1.882936990620205586 ) ) ;
#33976=CARTESIAN_POINT ( 'NONE',  ( 0.7813136802278927151, 156.5584078035761593, -0.9574549430346843693 ) ) ;
#33977=CARTESIAN_POINT ( 'NONE',  ( -15.77133435453296606, 146.5691041611200660, -0.3151487940933135334 ) ) ;
#33979=CARTESIAN_POINT ( 'NONE',  ( -5.554730375463081238, 156.7050554705274408, -1.852363956736410522 ) ) ;
#33980=CARTESIAN_POINT ( 'NONE',  ( 4.466571682983457414, -15.50692525667736454, 1.643437993322231838 ) ) ;
#33982=CARTESIAN_POINT ( 'NONE',  ( -4.342952997683876326, 118.1822044573729471, -0.6217259542595968691 ) ) ;
#33984=CARTESIAN_POINT ( 'NONE',  ( -4.979023873620669782, 117.5329379046127656, 0.7799942829153793111 ) ) ;
#33985=CARTESIAN_POINT ( 'NONE',  ( 5.064401052258119762, 119.9665122172617231, 0.9903757029826919522 ) ) ;
#33989=CARTESIAN_POINT ( 'NONE',  ( 23.45022726768229404, 146.8469795362756258, 0.4427096500589556838 ) ) ;
#33990=CARTESIAN_POINT ( 'NONE',  ( -0.4304388160753707671, 14.75877898171113145, 8.412599170943037663 ) ) ;
#33991=CARTESIAN_POINT ( 'NONE',  ( -0.003052472355949370757, 120.8426702770480148, 0.1527581987772198835 ) ) ;
#33995=CARTESIAN_POINT ( 'NONE',  ( 4.799946221453406103, 115.6909491485452435, 1.474290515418332115 ) ) ;
#33997=CARTESIAN_POINT ( 'NONE',  ( -23.44551923343654209, 146.8400249081559537, -0.3912800906488113073 ) ) ;
#34000=CARTESIAN_POINT ( 'NONE',  ( 5.827611813826044873, 121.2139407771506541, -0.2588721111321020674 ) ) ;
#34001=CARTESIAN_POINT ( 'NONE',  ( -3.174366308152012817, 88.99346620154574339, -0.06343139340882730792 ) ) ;
#34003=CARTESIAN_POINT ( 'NONE',  ( 0.6166252005165503425, 115.7029855507786209, -1.738059646771149547 ) ) ;
#34004=CARTESIAN_POINT ( 'NONE',  ( -0.6320571215040977631, 120.9405031987692212, -0.1040377489725131110 ) ) ;
#34005=CARTESIAN_POINT ( 'NONE',  ( 4.964329757808820354, -12.46733462535230785, 1.954119038396571417 ) ) ;
#34006=CARTESIAN_POINT ( 'NONE',  ( -6.863242444369421769, 118.1252062928739832, 0.7545491157480666011 ) ) ;
#34008=CARTESIAN_POINT ( 'NONE',  ( 4.741236776273888509, 116.7839080817633430, 0.2126559219428779679 ) ) ;
#34010=CARTESIAN_POINT ( 'NONE',  ( 5.959810334499592521, 155.3892724211786742, 0.1190911940436167188 ) ) ;
#34012=CARTESIAN_POINT ( 'NONE',  ( 0.5005776846888100318, 19.73258526448893591, -0.8400667230076528380 ) ) ;
#34013=B_SPLINE_CURVE_WITH_KNOTS ( 'NONE', 3,
 ( #18678, #24440, #18465, #11665 ),
 .UNSPECIFIED., .F., .F.,
 ( 4, 4 ),
 ( 0.000000000000000000, 0.0004246169644143726364 ),
 .UNSPECIFIED. ) ;
#34014=CARTESIAN_POINT ( 'NONE',  ( -18.63389541082843337, 154.1203422869290023, -0.3962720605433150967 ) ) ;
#34018=CARTESIAN_POINT ( 'NONE',  ( -6.503981220335420706E-14, 66.64146620154573952, -9.408573323119121831E-18 ) ) ;
#34021=CARTESIAN_POINT ( 'NONE',  ( -3.222226742346633088, 117.5522224569482574, 0.6736568086485349438 ) ) ;
#34022=CARTESIAN_POINT ( 'NONE',  ( 4.406646451516359697, -6.344046434980911364, 1.391598188203984288 ) ) ;
#34023=CARTESIAN_POINT ( 'NONE',  ( 21.97492997893991884, 149.1257232373000647, 2.026018130409337648 ) ) ;
#34025=CARTESIAN_POINT ( 'NONE',  ( 11.63724909022833387, 121.0393782313542346, -1.189926691809806814 ) ) ;
#34026=CARTESIAN_POINT ( 'NONE',  ( -2.092221094934305192, 20.21789226318614041, 8.165053130886693822 ) ) ;
#34027=CARTESIAN_POINT ( 'NONE',  ( -13.98195098595651942, 120.5923583732999873, -1.177051350580812894 ) ) ;
#34028=CARTESIAN_POINT ( 'NONE',  ( 4.814618516084593125, 117.6401595242498530, -0.9373198651747913779 ) ) ;
#34029=EDGE_LOOP ( 'NONE', ( #13259, #8609, #24846, #17458 ) ) ;
#34030=CARTESIAN_POINT ( 'NONE',  ( -9.357997026032906618, 124.2740283646700306, 0.04730198213477326136 ) ) ;
#34031=CARTESIAN_POINT ( 'NONE',  ( 2.292478802652971659, -15.50831694688660534, 5.896745190559482985 ) ) ;
#34033=CARTESIAN_POINT ( 'NONE',  ( -0.1782324565444364795, 117.3993841991624834, -1.495935750720309265 ) ) ;
#34034=ORIENTED_EDGE ( 'NONE', *, *, #23484, .T. ) ;
#34035=CARTESIAN_POINT ( 'NONE',  ( 19.20654067994509262, 147.6776069388173767, 2.506343067704081218 ) ) ;
#34037=DIRECTION ( 'NONE',  ( -4.017660918040594346E-17, 1.000000000000000000, 2.376309959284834438E-19 ) ) ;
#34038=CARTESIAN_POINT ( 'NONE',  ( -1.604275531929196363, 118.9836165220538504, 0.7112099450351576646 ) ) ;
#34039=CARTESIAN_POINT ( 'NONE',  ( 7.658903097349539557, 3.149683656735901671, 3.518291596705641400 ) ) ;
#34040=CARTESIAN_POINT ( 'NONE',  ( 15.86545709684687111, 148.0001117310855250, 1.424070646214982139 ) ) ;
#34042=CARTESIAN_POINT ( 'NONE',  ( 1.391432384042537551, 159.5643428290674990, -0.4004207282219805486 ) ) ;
#34043=DIRECTION ( 'NONE',  ( -0.9998004120163608288, 0.000000000000000000, -0.01997839162482749342 ) ) ;
#34048=CARTESIAN_POINT ( 'NONE',  ( 1.831848720338790093, -15.17974794010013539, 5.463771816453675712 ) ) ;
#34049=CARTESIAN_POINT ( 'NONE',  ( -4.123206031880720879, 118.2429491485453354, 0.1807802907187911756 ) ) ;
#34050=CARTESIAN_POINT ( 'NONE',  ( 1.454130924128286484, 106.2090255614461398, -5.133973488550625852 ) ) ;
#34054=CARTESIAN_POINT ( 'NONE',  ( 8.327809159883996060, 120.1035990385444592, -1.118180374562136148 ) ) ;
#34055=CARTESIAN_POINT ( 'NONE',  ( -5.590287297675261335, 117.9270669303711117, -0.7481252288361712743 ) ) ;
#34056=CARTESIAN_POINT ( 'NONE',  ( 4.264584009495184347, 118.2128444281766946, 0.5331355191356830225 ) ) ;
#34057=CARTESIAN_POINT ( 'NONE',  ( -4.469395743915104191, 155.8822484669112214, -0.8121950557409370886 ) ) ;
#34060=CARTESIAN_POINT ( 'NONE',  ( 0.2172131096560099284, 118.1651004646295888, -0.8870994772933850081 ) ) ;
#34063=CARTESIAN_POINT ( 'NONE',  ( 3.874746376330849618, 18.20996518813934628, -2.522041008920607563 ) ) ;
#34064=CARTESIAN_POINT ( 'NONE',  ( -12.60153737394488438, 128.4643691153342218, -1.495224527512394985 ) ) ;
#34067=CARTESIAN_POINT ( 'NONE',  ( -6.507153519498132566E-14, 76.29346620154572634, 3.067795752821199360E-29 ) ) ;
#34068=CARTESIAN_POINT ( 'NONE',  ( -5.946351765289578317, 155.4082313378804088, -0.01440516234414714047 ) ) ;
#34069=CARTESIAN_POINT ( 'NONE',  ( 4.982727044776202874, 117.5252055169183762, -0.7682891009986807518 ) ) ;
#34070=CARTESIAN_POINT ( 'NONE',  ( 15.07172804838052471, 121.1899582252741112, 1.138989471373297535 ) ) ;
#34071=CARTESIAN_POINT ( 'NONE',  ( -3.682264917456323339, 76.29346620154572634, -0.07358041635423923088 ) ) ;
#34072=CARTESIAN_POINT ( 'NONE',  ( 2.102813808753936087, -15.18136450426021256, 5.202461169095355942 ) ) ;
#34073=CARTESIAN_POINT ( 'NONE',  ( 17.30645727728350280, 153.8449085212272678, -1.293747054194649415 ) ) ;
#34075=CARTESIAN_POINT ( 'NONE',  ( -11.99432760026360434, 123.0912118827050108, 1.285395851362399977 ) ) ;
#34076=CARTESIAN_POINT ( 'NONE',  ( -0.9748693424575083366, -1.807339741155509660, 0.05984739681150109264 ) ) ;
#34077=CARTESIAN_POINT ( 'NONE',  ( -15.01050271945743653, 120.7699597703182945, -0.9001124940000717611 ) ) ;
#34078=CARTESIAN_POINT ( 'NONE',  ( 0.7251766580790658390, 11.37246313919491314, 0.6538263676454795226 ) ) ;
#34081=CARTESIAN_POINT ( 'NONE',  ( -9.519849589794810996, 124.0643708016488063, 0.3285928725474107082 ) ) ;
#34082=CARTESIAN_POINT ( 'NONE',  ( 2.009495809369673314, -15.14277677434763802, 5.899592854099822148 ) ) ;
#34083=CARTESIAN_POINT ( 'NONE',  ( 8.931878350220390672, 122.0520977060996586, -0.9029078837920735401 ) ) ;
#34084=ORIENTED_EDGE ( 'NONE', *, *, #27427, .T. ) ;
#34085=CARTESIAN_POINT ( 'NONE',  ( 2.528150074622308452, 115.7031097523288139, 1.694672199128987256 ) ) ;
#34086=CARTESIAN_POINT ( 'NONE',  ( 2.604768916882071128, -14.79682312136586297, 4.847387382002324330 ) ) ;
#34087=CARTESIAN_POINT ( 'NONE',  ( -4.970811386520536779, 117.4009602783328461, -0.9886943268754924130 ) ) ;
#34088=CARTESIAN_POINT ( 'NONE',  ( 10.26263990951786198, 126.0184183664171655, 0.1119868329536249096 ) ) ;
#34090=CARTESIAN_POINT ( 'NONE',  ( 5.841774105247304227, 118.7305451321402501, 1.158284778981343743 ) ) ;
#34091=CARTESIAN_POINT ( 'NONE',  ( 5.242938621905797625, 115.7725906505842488, 0.9935740274284472484 ) ) ;
#34094=CARTESIAN_POINT ( 'NONE',  ( 0.02768739821002592222, 156.9833357668885014, -1.385590625008458643 ) ) ;
#34095=CARTESIAN_POINT ( 'NONE',  ( 0.002459401150238499107, 159.6023738651833810, -0.1230784904792618234 ) ) ;
#34098=CARTESIAN_POINT ( 'NONE',  ( 1.786952995998799532, -15.53348570852046429, 5.439464539514906605 ) ) ;
#34100=CYLINDRICAL_SURFACE ( 'NONE', #13743, 5.588000000000006295 ) ;
#34101=CARTESIAN_POINT ( 'NONE',  ( -4.726345281775343743, 117.8966967845652505, 0.7850290684345025971 ) ) ;
#34103=CARTESIAN_POINT ( 'NONE',  ( -0.1233619748781853986, 118.7629491485454025, 1.274984637400677245 ) ) ;
#34104=CARTESIAN_POINT ( 'NONE',  ( -3.290814539092682622, 118.4664756651339701, -0.9164823782932540741 ) ) ;
#34105=CARTESIAN_POINT ( 'NONE',  ( -4.585195778441760517, 124.9344662015457459, -0.09162312381275013184 ) ) ;
#34106=CARTESIAN_POINT ( 'NONE',  ( 4.755188516126013454, 117.4716628415562525, 1.195539700728312393 ) ) ;
#34108=CARTESIAN_POINT ( 'NONE',  ( -0.04081796246458029020, 114.7739974199301969, 2.042697753608868627 ) ) ;
#34109=CARTESIAN_POINT ( 'NONE',  ( -3.158589313471108273, 4.191505055319898254, 3.400481138232230194 ) ) ;
#34112=CARTESIAN_POINT ( 'NONE',  ( 3.930318996895993955, -12.97851325427171254, 2.595110522791146401 ) ) ;
#34113=CARTESIAN_POINT ( 'NONE',  ( 4.039333660417788074, 117.0582680968029905, -0.9406562914258044250 ) ) ;
#34114=CARTESIAN_POINT ( 'NONE',  ( 0.9692622191906820062, 39.20946620154573026, 1.289621693195544205 ) ) ;
#34115=CARTESIAN_POINT ( 'NONE',  ( -1.844538656955264866, 115.7029491485453292, 1.651265962246492913 ) ) ;
#34117=CARTESIAN_POINT ( 'NONE',  ( -5.138143029425324748, 105.1220589700577079, -1.444278753282428385 ) ) ;
#34118=CARTESIAN_POINT ( 'NONE',  ( 4.161657294200716173, -15.28457189793756754, -0.5145498944859950852 ) ) ;
#34119=CARTESIAN_POINT ( 'NONE',  ( -19.22223103763165497, 149.5120288530235655, 1.725574580128898861 ) ) ;
#34121=CARTESIAN_POINT ( 'NONE',  ( 0.6140693529284619867, 19.51110927180549481, -0.7576854961706591673 ) ) ;
#34122=ORIENTED_EDGE ( 'NONE', *, *, #30040, .T. ) ;
#34125=CARTESIAN_POINT ( 'NONE',  ( 4.467639297142982358, 123.9529229959338608, 0.1358511699341446444 ) ) ;
#34126=CARTESIAN_POINT ( 'NONE',  ( -16.21676096112159371, 148.3349945484709451, 1.109893536416839188 ) ) ;
#34128=CARTESIAN_POINT ( 'NONE',  ( 4.523391899494686896, 118.0850475785753559, -0.6138312095713829297 ) ) ;
#34129=CARTESIAN_POINT ( 'NONE',  ( 11.45258232062217907, 123.1738952066917534, -1.204891439250160401 ) ) ;
#34130=CIRCLE ( 'NONE', #21837, 0.5080000000000002292 ) ;
#34131=CARTESIAN_POINT ( 'NONE',  ( -8.818906024077520556, 119.8693228481767932, -1.468947216590822169 ) ) ;
#34133=ORIENTED_EDGE ( 'NONE', *, *, #38673, .F. ) ;
#34134=CARTESIAN_POINT ( 'NONE',  ( 4.253933811591600112, 118.2250371594836906, -0.3060402623648788567 ) ) ;
#34135=CARTESIAN_POINT ( 'NONE',  ( 4.346810452489679122, 155.8404949922767742, -0.3425513195823393087 ) ) ;
#34137=CARTESIAN_POINT ( 'NONE',  ( 3.213008622916347701, -14.43860267280072662, 2.307402664594705222 ) ) ;
#34138=CIRCLE ( 'NONE', #26641, 0.5080000000000002292 ) ;
#34141=CARTESIAN_POINT ( 'NONE',  ( -0.4757704999385121702, -3.320450887815510121, -4.596079559024887295 ) ) ;
#34142=CARTESIAN_POINT ( 'NONE',  ( 11.12341512264660892, 124.6236798342360856, 1.410428355923976751 ) ) ;
#34143=CARTESIAN_POINT ( 'NONE',  ( 0.08255133343488754716, 33.15144596319247938, 2.721925856402449551 ) ) ;
#34144=CARTESIAN_POINT ( 'NONE',  ( -5.416028590487236727, 119.2618716387835747, 0.3471801096392534425 ) ) ;
#34146=VECTOR ( 'NONE', #24129, 1000.000000000000000 ) ;
#34147=CARTESIAN_POINT ( 'NONE',  ( 3.746277899330032302, -0.8937244826341392834, -2.755274729908455900 ) ) ;
#34148=CARTESIAN_POINT ( 'NONE',  ( 14.17736129766400310, 138.8817910697950140, 0.3341079978015795149 ) ) ;
#34149=FACE_OUTER_BOUND ( 'NONE', #11860, .T. ) ;
#34152=CARTESIAN_POINT ( 'NONE',  ( -5.529636975226489781, 116.8416598262861896, -0.5092621927480067701 ) ) ;
#34155=CARTESIAN_POINT ( 'NONE',  ( 1.824651611884651636, -15.33505462125984131, 5.392305443003409415 ) ) ;
#34157=CARTESIAN_POINT ( 'NONE',  ( -8.364652471777612064, 2.666895906452835252, -0.9765287277423425616 ) ) ;
#34159=CARTESIAN_POINT ( 'NONE',  ( -6.376221727585796537E-14, 51.14746620154573264, 5.777789833161707559E-29 ) ) ;
#34161=EDGE_CURVE ( 'NONE', #15637, #38156, #11966, .T. ) ;
#34163=CARTESIAN_POINT ( 'NONE',  ( -1.900581966506003084, 116.7132768022172797, 0.2320997050762017011 ) ) ;
#34166=ORIENTED_EDGE ( 'NONE', *, *, #31332, .T. ) ;
#34168=CARTESIAN_POINT ( 'NONE',  ( -0.0006557933561996413981, 120.9974662015457767, 0.03281858119439454852 ) ) ;
#34169=CARTESIAN_POINT ( 'NONE',  ( 6.347728850385006005, -14.18411723689298753, 0.2678442101147658905 ) ) ;
#34170=CARTESIAN_POINT ( 'NONE',  ( -4.967439785005512753, 118.2512723699127832, 0.8146033317824223907 ) ) ;
#34171=CARTESIAN_POINT ( 'NONE',  ( 22.55594873278722545, 149.0203452686010337, -0.8552431815872718612 ) ) ;
#34172=CARTESIAN_POINT ( 'NONE',  ( -1.471791394198959102, 24.03230288535706549, 4.399545648925609065 ) ) ;
#34173=CARTESIAN_POINT ( 'NONE',  ( -18.54318072098663706, 125.2038358216989735, -0.7288164436403700153 ) ) ;
#34179=CARTESIAN_POINT ( 'NONE',  ( -0.02874415600673332558, 157.0795416643300939, 1.438475106415294302 ) ) ;
#34180=DIRECTION ( 'NONE',  ( -0.01997839162482761832, -1.040247600000950455E-18, 0.9998004120163610509 ) ) ;
#34181=CARTESIAN_POINT ( 'NONE',  ( 0.03256023585714045571, 157.9544661776888290, -1.629447346748784220 ) ) ;
#34182=CARTESIAN_POINT ( 'NONE',  ( -21.52870603658947957, 148.1022500232506616, -2.247031159961963898 ) ) ;
#34185=CARTESIAN_POINT ( 'NONE',  ( 1.514956540612153235, 120.4980338609919386, -0.3173598453907556793 ) ) ;
#34188=CARTESIAN_POINT ( 'NONE',  ( -11.01240597710811997, 122.5598569164413334, -1.651065454484658801 ) ) ;
#34189=CARTESIAN_POINT ( 'NONE',  ( 4.008975597637738808, -15.55340266690961926, 2.658432704422428738 ) ) ;
#34190=CARTESIAN_POINT ( 'NONE',  ( -4.357656026889322298, 118.1846519306246250, -0.6081638617269276015 ) ) ;
#34194=CARTESIAN_POINT ( 'NONE',  ( -4.880246989775093525, 117.5475785438034961, 0.9414120544623780784 ) ) ;
#34195=CARTESIAN_POINT ( 'NONE',  ( 9.561780282765681704, 155.2307989660268959, 2.006535919638082532 ) ) ;
#34198=CARTESIAN_POINT ( 'NONE',  ( 13.43647848967384029, 156.9186530619738562, 0.2471310363275584510 ) ) ;
#34199=CARTESIAN_POINT ( 'NONE',  ( -0.3997009428961929567, 0.5197794802236572753, -8.431077252154732804 ) ) ;
#34200=CARTESIAN_POINT ( 'NONE',  ( 9.229671467331764134, 123.9961275534082148, 0.5040434471971629860 ) ) ;
#34201=CARTESIAN_POINT ( 'NONE',  ( 0.01793833495430298061, 118.1627382089642566, -0.8977079103094813828 ) ) ;
#34203=CARTESIAN_POINT ( 'NONE',  ( -2.755218082995318341, 118.1588897907562625, 0.7196486339555533407 ) ) ;
#34206=CARTESIAN_POINT ( 'NONE',  ( -8.060084350832312339, 158.6724238832827609, -0.05135189671889796303 ) ) ;
#34209=CARTESIAN_POINT ( 'NONE',  ( 7.896700704331069076, 122.1485567550560205, -0.5293793203400826153 ) ) ;
#34210=CARTESIAN_POINT ( 'NONE',  ( -8.321979263998686704, 120.1320355853848554, 1.118248183737064583 ) ) ;
#34211=VERTEX_POINT ( 'NONE', #16251 ) ;
#34212=CARTESIAN_POINT ( 'NONE',  ( -4.757346424997288103, 117.3993836135861386, -1.207075064218979810 ) ) ;
#34213=CARTESIAN_POINT ( 'NONE',  ( -14.70702164887893559, 148.8393470518043955, -0.6194100056173926783 ) ) ;
#34214=CARTESIAN_POINT ( 'NONE',  ( 4.982342844640083257, -12.32172870019713962, 1.713706004506841740 ) ) ;
#34215=CARTESIAN_POINT ( 'NONE',  ( -2.946692055775997687, 159.0164033662945258, 1.213088979206726314 ) ) ;
#34217=CARTESIAN_POINT ( 'NONE',  ( 16.05840932322194803, 121.2308719818149712, 0.4813400273897942006 ) ) ;
#34218=CARTESIAN_POINT ( 'NONE',  ( 4.209818400188686027, 155.8650778562950450, 0.1319121167718819154 ) ) ;
#34219=CARTESIAN_POINT ( 'NONE',  ( 0.6140693529284619867, 19.51110927180549481, -0.7576854961706591673 ) ) ;
#34220=CARTESIAN_POINT ( 'NONE',  ( -22.53527615164633602, 150.7831677823008363, -0.4503084484864735004 ) ) ;
#34226=CARTESIAN_POINT ( 'NONE',  ( -4.211597740687054170, 118.4194010483798536, 0.8451905551736870192 ) ) ;
#34228=CARTESIAN_POINT ( 'NONE',  ( 21.36223069762250049, 149.8571540977637255, 2.130384393597193782 ) ) ;
#34230=CARTESIAN_POINT ( 'NONE',  ( 13.10063739191614118, 155.4510764517707742, -1.634185922311342409 ) ) ;
#34231=CARTESIAN_POINT ( 'NONE',  ( 6.371402057089752269, 24.08812572624405135, -5.527521448792488634 ) ) ;
#34232=CARTESIAN_POINT ( 'NONE',  ( -22.43644356963083908, 149.3130771379323392, -1.752678757896036332 ) ) ;
#34233=CARTESIAN_POINT ( 'NONE',  ( 4.978618612593685988, 117.5329194034797382, -0.7802320411340670780 ) ) ;
#34234=EDGE_LOOP ( 'NONE', ( #24030, #19213, #7437, #20772 ) ) ;
#34235=CARTESIAN_POINT ( 'NONE',  ( -7.582677863711315247, 122.4179301937671767, -0.01237541680613125222 ) ) ;
#34236=CARTESIAN_POINT ( 'NONE',  ( 6.238852630440780977, -14.32403127715267743, 0.8647906437036265714 ) ) ;
#34242=CARTESIAN_POINT ( 'NONE',  ( 4.177977944338209682, 119.2415290214368042, 0.9917981586689075257 ) ) ;
#34247=CARTESIAN_POINT ( 'NONE',  ( -3.292372560053943520, 124.4927030837263118, -0.04348745598417495112 ) ) ;
#34249=CARTESIAN_POINT ( 'NONE',  ( -1.603550922812138735, -3.093932695209369754, -8.287855504117967342 ) ) ;
#34250=CARTESIAN_POINT ( 'NONE',  ( 0.5945828676174961247, 120.5739061664170606, 0.2962085107056581790 ) ) ;
#34251=CARTESIAN_POINT ( 'NONE',  ( -4.787919979293251416, 115.6909491485453003, -1.476228160204360096 ) ) ;
#34252=CARTESIAN_POINT ( 'NONE',  ( 22.47867321467002810, 150.2745577238280816, -0.5153050491938899746 ) ) ;
#34258=CARTESIAN_POINT ( 'NONE',  ( 1.930977371672658816, -15.05712096081326123, 5.742647184725755416 ) ) ;
#34259=CARTESIAN_POINT ( 'NONE',  ( -4.298763888250202392, 118.2143499254979133, 0.3450211622763035280 ) ) ;
#34260=CARTESIAN_POINT ( 'NONE',  ( 2.560925085873138052, 106.9236017804954599, -4.673771261702133195 ) ) ;
#34263=CARTESIAN_POINT ( 'NONE',  ( -6.212440689485183576, 119.7770897763353446, -1.234393554324211939 ) ) ;
#34264=CARTESIAN_POINT ( 'NONE',  ( 5.243110457265114377, 104.6144662015457527, 1.505012106405181127 ) ) ;
#34266=CARTESIAN_POINT ( 'NONE',  ( 4.381688799442883031, 118.1622743267563607, 0.6667146239118652007 ) ) ;
#34267=CARTESIAN_POINT ( 'NONE',  ( -5.875838086862464671, 121.3091694753028520, -0.5415667612380997697 ) ) ;
#34269=CARTESIAN_POINT ( 'NONE',  ( 13.70496720262315193, 119.6480011847128253, 0.2738578607176476165 ) ) ;
#34271=CARTESIAN_POINT ( 'NONE',  ( 2.163044864548389956, 28.58015952483584954, -4.087059112497700042 ) ) ;
#34272=CARTESIAN_POINT ( 'NONE',  ( 0.007600002268316488618, 120.2037396364829505, -0.3803351912374555721 ) ) ;
#34275=CARTESIAN_POINT ( 'NONE',  ( 5.586884702347364673, 94.32746620154571815, 0.1116392523995368424 ) ) ;
#34276=CARTESIAN_POINT ( 'NONE',  ( 6.990440677580159523, 121.9275277802277344, 0.3101014599809851502 ) ) ;
#34277=CARTESIAN_POINT ( 'NONE',  ( -4.488006035213030209, 18.49445617864287073, 1.146732334616328286 ) ) ;
#34278=CARTESIAN_POINT ( 'NONE',  ( 15.50015290592184591, 121.4967652112180048, 1.085784428920436584 ) ) ;
#34280=CARTESIAN_POINT ( 'NONE',  ( 3.162130362391316840, -14.71481139081727640, 3.323541290955854599 ) ) ;
#34281=CARTESIAN_POINT ( 'NONE',  ( 10.67497907003066260, 119.8050749133877275, -0.9899969268117742027 ) ) ;
#34282=CARTESIAN_POINT ( 'NONE',  ( -12.69690185265283056, 124.0847267554996591, 1.337322108705696566 ) ) ;
#34283=CARTESIAN_POINT ( 'NONE',  ( -2.131885088311801901, 26.04095958170969638, -4.099730575217565232 ) ) ;
#34284=CARTESIAN_POINT ( 'NONE',  ( -18.41332411163130800, 154.1649927243852858, -1.048538238682171775 ) ) ;
#34286=CARTESIAN_POINT ( 'NONE',  ( -0.8578381542044509755, 18.04903173543935679, 0.4659799999690844019 ) ) ;
#34289=CARTESIAN_POINT ( 'NONE',  ( -9.705341575047336633, 124.1466939447965814, 0.4180229424618550627 ) ) ;
#34290=CARTESIAN_POINT ( 'NONE',  ( 4.326150682005948767, -14.13415638199089130, 4.511655897031580764 ) ) ;
#34291=CARTESIAN_POINT ( 'NONE',  ( 5.149255372874153913, 120.5246234221128248, -0.6142761105479899175 ) ) ;
#34292=VECTOR ( 'NONE', #4292, 1000.000000000000000 ) ;
#34294=CARTESIAN_POINT ( 'NONE',  ( 1.791698859000329769, 115.7029403034601103, 1.723151393639055229 ) ) ;
#34295=CARTESIAN_POINT ( 'NONE',  ( 1.878022632408997250, -15.11918648689831990, 5.509382895440600336 ) ) ;
#34296=CARTESIAN_POINT ( 'NONE',  ( -4.697896922046175483, 117.7521787132836408, -1.088562244697523385 ) ) ;
#34297=CARTESIAN_POINT ( 'NONE',  ( 5.301853325284109353, 121.3529869156830046, 0.07809170188345493369 ) ) ;
#34299=CARTESIAN_POINT ( 'NONE',  ( 20.36154792711260697, 148.1475078817917961, 2.480623434655590209 ) ) ;
#34300=CARTESIAN_POINT ( 'NONE',  ( -6.580517660824093636E-14, 85.69146620154573668, -4.881702850681514412E-18 ) ) ;
#34301=AXIS2_PLACEMENT_3D ( 'NONE', #3238, #16196, #29201 ) ;
#34302=DIRECTION ( 'NONE',  ( -4.017660918040594346E-17, 1.000000000000000000, 2.376309959284832031E-19 ) ) ;
#34304=CARTESIAN_POINT ( 'NONE',  ( 0.01443894962456205439, 159.4760848062415732, -0.7225840825867285711 ) ) ;
#34305=CARTESIAN_POINT ( 'NONE',  ( 13.61761151811281501, 119.6358206793323404, 0.1207630679856301764 ) ) ;
#34306=FACE_OUTER_BOUND ( 'NONE', #8545, .T. ) ;
#34307=CIRCLE ( 'NONE', #3028, 3.175000000000001155 ) ;
#34308=CARTESIAN_POINT ( 'NONE',  ( 1.661411379530861154, -15.34330027928626450, 5.771677961256235001 ) ) ;
#34309=CARTESIAN_POINT ( 'NONE',  ( 4.962080476404062246, 117.4056796065936368, 1.029808796348710143 ) ) ;
#34311=CARTESIAN_POINT ( 'NONE',  ( -4.712400925315380462, 117.8378367728824117, 0.8491269253323575628 ) ) ;
#34313=PLANE ( 'NONE',  #28878 ) ;
#34314=CARTESIAN_POINT ( 'NONE',  ( -3.010539197181554272, 118.1721198718190635, -0.8802744401777266026 ) ) ;
#34315=CARTESIAN_POINT ( 'NONE',  ( -3.281580062219434435, 118.9685052735122355, -0.6847577310700789788 ) ) ;
#34316=CARTESIAN_POINT ( 'NONE',  ( 4.932381249567058035, 117.4753000372011229, 1.061590090608461212 ) ) ;
#34317=CARTESIAN_POINT ( 'NONE',  ( -4.697896922046175483, 117.7521787132836408, -1.088562244697523385 ) ) ;
#34318=CARTESIAN_POINT ( 'NONE',  ( -0.09934209769005267199, 106.7790779034713324, 4.971484795507161714 ) ) ;
#34319=CARTESIAN_POINT ( 'NONE',  ( 4.636249899789679496, -11.37698174978397958, -0.2454043791197063895 ) ) ;
#34320=CARTESIAN_POINT ( 'NONE',  ( 5.007034960109912447, 117.4001718673160468, -0.7827158424842978190 ) ) ;
#34321=DIRECTION ( 'NONE',  ( -0.9998004120163608288, 0.000000000000000000, -0.01997839162482747608 ) ) ;
#34322=CARTESIAN_POINT ( 'NONE',  ( 1.889397806843069905, -15.09730794468430659, 5.542604807410119072 ) ) ;
#34323=CARTESIAN_POINT ( 'NONE',  ( 6.279970060868345527, 120.0898888515776264, -0.2014705954985338276 ) ) ;
#34324=CARTESIAN_POINT ( 'NONE',  ( 2.928799644063047936, 38.81416391459460158, 1.351591292951386247 ) ) ;
#34325=CARTESIAN_POINT ( 'NONE',  ( -0.3836348520032437648, 115.7029491485453008, 1.750602596047696524 ) ) ;
#34326=CARTESIAN_POINT ( 'NONE',  ( -1.471791394198959324, 24.03230288535706549, 4.399545648925609065 ) ) ;
#34327=ORIENTED_EDGE ( 'NONE', *, *, #15761, .T. ) ;
#34328=CARTESIAN_POINT ( 'NONE',  ( -3.608777164148366801, 104.6144662015523465, -3.943486902631163638 ) ) ;
#34330=CARTESIAN_POINT ( 'NONE',  ( 4.057567908148627112, -15.53776324113162488, 2.457816012360223290 ) ) ;
#34331=CARTESIAN_POINT ( 'NONE',  ( -12.64706598677953764, 155.2353133052689032, 1.715565181845534637 ) ) ;
#34332=CARTESIAN_POINT ( 'NONE',  ( 0.5691593726700751033, 20.64373787749807576, 0.7897743370290384313 ) ) ;
#34333=CARTESIAN_POINT ( 'NONE',  ( -0.2901879621234837447, 21.01165217803846730, -0.9340445150429393939 ) ) ;
#34334=VERTEX_POINT ( 'NONE', #27113 ) ;
#34337=CARTESIAN_POINT ( 'NONE',  ( 3.231038154352767311, 124.0549386377059307, 0.1153833196696142788 ) ) ;
#34338=CARTESIAN_POINT ( 'NONE',  ( -7.181592176188232202, 121.6016026263613838, 0.5649366106928357389 ) ) ;
#34339=CARTESIAN_POINT ( 'NONE',  ( -6.453647670433203483E-14, 66.13346620154574396, 1.207165459738467839E-19 ) ) ;
#34340=CARTESIAN_POINT ( 'NONE',  ( 4.728982595459171101, 117.9669356887236376, -0.6198681105378882616 ) ) ;
#34341=CARTESIAN_POINT ( 'NONE',  ( 15.17272240541826989, 131.2890697635526465, -1.517944203131903036 ) ) ;
#34342=CARTESIAN_POINT ( 'NONE',  ( -20.08651816730963802, 147.5185649274072830, -2.508444087122727595 ) ) ;
#34344=CARTESIAN_POINT ( 'NONE',  ( -1.535725013305945685, 36.30113686556708785, 2.247037283891923476 ) ) ;
#34345=CARTESIAN_POINT ( 'NONE',  ( 15.93731397951207107, 146.3070982487133165, -0.2768821801232402291 ) ) ;
#34347=CARTESIAN_POINT ( 'NONE',  ( 3.141231902390079878, -14.40076222614043644, 1.273921468989656969 ) ) ;
#34350=CARTESIAN_POINT ( 'NONE',  ( -4.434453077421578904, -10.21728329253013179, 1.368390957472948921 ) ) ;
#34351=CARTESIAN_POINT ( 'NONE',  ( 1.805426509874223262, 156.5029897098349636, 1.055579731365336338 ) ) ;
#34352=CARTESIAN_POINT ( 'NONE',  ( -3.938977128594349342, 28.07268674286775223, 0.7495841607770360460 ) ) ;
#34353=CARTESIAN_POINT ( 'NONE',  ( -6.650203214911595495, 123.1390089711370166, -0.06171709628626032701 ) ) ;
#34354=CARTESIAN_POINT ( 'NONE',  ( 1.719524320724281852, 5.915668354077112667, 4.300554535892874064 ) ) ;
#34355=CARTESIAN_POINT ( 'NONE',  ( 8.959768907663312021, 123.9105667600146177, 0.2128205007565313611 ) ) ;
#34356=CARTESIAN_POINT ( 'NONE',  ( 1.876134371277577761, -7.842104223405461205, 8.241158351834352302 ) ) ;
#34358=CARTESIAN_POINT ( 'NONE',  ( -8.748764066053464461, 117.8789303818463452, -0.6453613471464660911 ) ) ;
#34361=CARTESIAN_POINT ( 'NONE',  ( -2.169500164636429140, 35.42160933236649356, 3.123960633263313635 ) ) ;
#34362=CARTESIAN_POINT ( 'NONE',  ( -8.161197318747062113, 2.438352165997351495, -2.203247879407881804 ) ) ;
#34363=CARTESIAN_POINT ( 'NONE',  ( 0.08161408160584908422, 118.1588881536456199, 0.9086033322154761782 ) ) ;
#34364=DIRECTION ( 'NONE',  ( 0.9998004120163609398, 4.016384292689130894E-17, 0.01997839162482749689 ) ) ;
#34365=CARTESIAN_POINT ( 'NONE',  ( 0.3885115210725473278, 119.2343925067223722, -0.8110907263698885483 ) ) ;
#34366=CARTESIAN_POINT ( 'NONE',  ( -22.41683308396160967, 150.7562895891929031, 0.1409227600426841420 ) ) ;
#34371=CARTESIAN_POINT ( 'NONE',  ( -15.72385166996626715, 146.8976323831864477, -0.3141999770531619940 ) ) ;
#34372=CARTESIAN_POINT ( 'NONE',  ( 5.095505811086057157, -15.28584205578724386, 3.479711806413861908 ) ) ;
#34373=CARTESIAN_POINT ( 'NONE',  ( -5.883034912960858343, 118.4234969239897453, 0.8666102449821463383 ) ) ;
#34374=CARTESIAN_POINT ( 'NONE',  ( 21.51828904745222815, 136.6907720476960435, -0.8331038389761593610 ) ) ;
#34375=CARTESIAN_POINT ( 'NONE',  ( 1.325333094648095011, 19.28447512809159292, -4.440015753949128730 ) ) ;
#34376=CARTESIAN_POINT ( 'NONE',  ( -15.91552649980327772, 121.2232988859741027, -0.6415868299260653052 ) ) ;
#34379=CARTESIAN_POINT ( 'NONE',  ( -5.563746608210566436, 116.6985881138792962, -0.07299084064307925779 ) ) ;
#34381=CARTESIAN_POINT ( 'NONE',  ( -17.77977776825587597, 147.3864036964934598, 1.530147356706996753 ) ) ;
#34383=CARTESIAN_POINT ( 'NONE',  ( 12.16919611748917518, 122.5392882283422864, -1.309229788656694815 ) ) ;
#34384=CARTESIAN_POINT ( 'NONE',  ( -18.77683424009551771, 152.0234722879370111, -2.226617664588433243 ) ) ;
#34386=CARTESIAN_POINT ( 'NONE',  ( 1.530333064024422374, 120.5919059741422217, -0.2783515840389083063 ) ) ;
#34389=CARTESIAN_POINT ( 'NONE',  ( -7.383155613640980164, 155.9567503867590972, -1.861932028473975986 ) ) ;
#34390=CARTESIAN_POINT ( 'NONE',  ( 4.538337246427208704, -15.41107556132688394, 0.6303774773485874006 ) ) ;
#34391=CARTESIAN_POINT ( 'NONE',  ( -4.459763086995446990, 118.1136472263767558, -0.7513301278392107152 ) ) ;
#34394=CARTESIAN_POINT ( 'NONE',  ( -4.992877067835030935, 117.4692132720523432, 0.8000675072955271139 ) ) ;
#34395=CARTESIAN_POINT ( 'NONE',  ( 9.425008295912057577, 155.1592096034013366, 1.957465225861826807 ) ) ;
#34397=CARTESIAN_POINT ( 'NONE',  ( -8.412600736458745843, -6.831223903669816799, -0.4304377746521336201 ) ) ;
#34398=CARTESIAN_POINT ( 'NONE',  ( 13.11017186724473405, 133.9996589410087324, 0.6993036124459158787 ) ) ;
#34402=CARTESIAN_POINT ( 'NONE',  ( -1.585929963085191741, 118.1588900223178058, 0.8129015274758119025 ) ) ;
#34403=CARTESIAN_POINT ( 'NONE',  ( 1.967271012213831938, 118.7629491485454025, 1.232500030677896374 ) ) ;
#34406=CARTESIAN_POINT ( 'NONE',  ( -23.41759249777153684, 146.8136392739129974, -0.2357739188755807458 ) ) ;
#34410=CARTESIAN_POINT ( 'NONE',  ( 6.912737236431420129, 121.7988612569186984, -0.2654354181093423470 ) ) ;
#34411=CARTESIAN_POINT ( 'NONE',  ( -8.036149603168206923, 121.5005262100067256, 0.8572904197357047451 ) ) ;
#34414=CARTESIAN_POINT ( 'NONE',  ( -15.80537369954035753, 146.5893318786020814, -0.6464893008334197111 ) ) ;
#34415=CARTESIAN_POINT ( 'NONE',  ( 4.916912942907655903, -13.49232782388964935, 3.465564004687308408 ) ) ;
#34416=CARTESIAN_POINT ( 'NONE',  ( -20.76678851138498416, 151.0745573368290593, 1.154740394482948407 ) ) ;
#34417=B_SPLINE_CURVE_WITH_KNOTS ( 'NONE', 3,
 ( #36484, #30081, #7305, #39895, #26886, #10487, #23457, #33291, #30285, #1127 ),
 .UNSPECIFIED., .F., .F.,
 ( 4, 2, 2, 2, 4 ),
 ( 0.000000000000000000, 0.001159180624616241214, 0.002318361249232482428, 0.003477541873848724509, 0.004636722498464966591 ),
 .UNSPECIFIED. ) ;
#34419=CARTESIAN_POINT ( 'NONE',  ( 22.64824804725698826, 137.2763855621842026, 0.6699328029008020380 ) ) ;
#34420=CARTESIAN_POINT ( 'NONE',  ( -0.0006556493172109406848, 120.9974662015457767, 0.03281137289327806100 ) ) ;
#34422=CARTESIAN_POINT ( 'NONE',  ( -0.7472855871240335901, 21.88424109716052612, -0.6269268744489370215 ) ) ;
#34424=CARTESIAN_POINT ( 'NONE',  ( -1.804784692667670054, 116.4728921782852922, -0.07541441754812425180 ) ) ;
#34428=CARTESIAN_POINT ( 'NONE',  ( 3.896950258392768873, 118.1803102188741121, 0.9604330818198881792 ) ) ;
#34430=CARTESIAN_POINT ( 'NONE',  ( 12.43751437118950953, 120.3283006479967128, 1.391730434942824779 ) ) ;
#34432=CARTESIAN_POINT ( 'NONE',  ( 19.84954981513660499, 141.2215177107240436, -1.686013488323441001 ) ) ;
#34433=CARTESIAN_POINT ( 'NONE',  ( 4.135298993362768627, -14.76517611359900961, -2.065434832541708676 ) ) ;
#34434=CARTESIAN_POINT ( 'NONE',  ( -13.81631647976139909, 120.6843904051541898, -1.269697867868519792 ) ) ;
#34435=CARTESIAN_POINT ( 'NONE',  ( 4.784420482501478666, 117.7320086554665721, -0.8971979045722391355 ) ) ;
#34436=CARTESIAN_POINT ( 'NONE',  ( 1.980401745280924830, 106.6864334246082961, 4.967395836420048560 ) ) ;
#34437=ORIENTED_EDGE ( 'NONE', *, *, #38483, .T. ) ;
#34438=B_SPLINE_CURVE_WITH_KNOTS ( 'NONE', 3,
 ( #27213, #1252, #16985, #24003 ),
 .UNSPECIFIED., .F., .F.,
 ( 4, 4 ),
 ( 0.000000000000000000, 1.000000000000000000 ),
 .UNSPECIFIED. ) ;
#34439=CARTESIAN_POINT ( 'NONE',  ( -11.90298433346896090, 130.3805625696445816, -0.1299774887382022792 ) ) ;
#34440=CARTESIAN_POINT ( 'NONE',  ( -19.37512658372783747, 148.3988719805327037, -2.511650730565585299 ) ) ;
#34441=CARTESIAN_POINT ( 'NONE',  ( 6.104261451579751530, -14.47397795074312299, 1.449478640324443290 ) ) ;
#34442=FACE_OUTER_BOUND ( 'NONE', #23240, .T. ) ;
#34444=CARTESIAN_POINT ( 'NONE',  ( -1.086168526012032842, 117.3993836040899623, -1.476592527281789691 ) ) ;
#34447=CARTESIAN_POINT ( 'NONE',  ( 18.98749958112889757, 148.5750135429820205, 2.495758040776019371 ) ) ;
#34448=TOROIDAL_SURFACE ( 'NONE', #1137, 5.080000000000005400, 0.5080000000000000071 ) ;
#34450=CARTESIAN_POINT ( 'NONE',  ( -4.842657161150313527, 118.7629491485453599, -0.3779612899170270435 ) ) ;
#34451=CARTESIAN_POINT ( 'NONE',  ( -0.5876368209473940007, 111.1955024190080223, 3.248215591009249170 ) ) ;
#34452=CARTESIAN_POINT ( 'NONE',  ( 5.926391002875100789, -6.993723907645660098, 5.986726992520772228 ) ) ;
#34453=CARTESIAN_POINT ( 'NONE',  ( 10.86813797462336950, 153.1125297277760069, 1.236783938685797501 ) ) ;
#34454=CARTESIAN_POINT ( 'NONE',  ( -4.911716961673469939, 115.6909491485453003, -1.456282297173534301 ) ) ;
#34456=CARTESIAN_POINT ( 'NONE',  ( 5.603706277412528358, 159.0849926622337023, -0.4754325247485730599 ) ) ;
#34459=FILL_AREA_STYLE_COLOUR ( '', #36437 ) ;
#34460=CARTESIAN_POINT ( 'NONE',  ( 22.46755768833288158, 150.8526571111528654, 0.4489552724284878171 ) ) ;
#34461=CARTESIAN_POINT ( 'NONE',  ( -4.267945882554810666, 118.2240384700266418, 0.2902935525537765904 ) ) ;
#34462=CARTESIAN_POINT ( 'NONE',  ( -17.31377588638430964, 122.7721875394316555, -0.3459704467065359834 ) ) ;
#34466=CARTESIAN_POINT ( 'NONE',  ( 8.297356343339515661, 120.2518627151980013, -1.115698539510747489 ) ) ;
#34467=FACE_OUTER_BOUND ( 'NONE', #9117, .T. ) ;
#34468=CARTESIAN_POINT ( 'NONE',  ( 4.254265354952431188, 118.2238472574425998, 0.4591671670676380490 ) ) ;
#34469=CARTESIAN_POINT ( 'NONE',  ( -9.255566420661768490, 123.6186430441458981, -0.7743267827205286835 ) ) ;
#34471=CARTESIAN_POINT ( 'NONE',  ( 1.794468298957800689, 116.4672891243423578, 0.03585774721038179763 ) ) ;
#34472=ORIENTED_EDGE ( 'NONE', *, *, #15989, .T. ) ;
#34473=CARTESIAN_POINT ( 'NONE',  ( -4.460028654926622593, 22.53297844546955631, 1.214995109042491528 ) ) ;
#34478=CARTESIAN_POINT ( 'NONE',  ( -6.995060180358994906, 121.8891585157791866, 0.1212626282798120736 ) ) ;
#34479=EDGE_CURVE ( 'NONE', #30442, #7672, #4546, .T. ) ;
#34480=CARTESIAN_POINT ( 'NONE',  ( -2.714482067202859561, 26.26591195808746448, -3.750338772627290762 ) ) ;
#34481=CARTESIAN_POINT ( 'NONE',  ( 14.73023064483735922, 156.1040168620350244, 1.249499669456201723 ) ) ;
#34482=CARTESIAN_POINT ( 'NONE',  ( -0.7257356453791840023, 104.6144662015456390, -4.780984660456490509 ) ) ;
#34483=CARTESIAN_POINT ( 'NONE',  ( 3.092086460852839114, -14.79905751219236265, 3.633802299706017980 ) ) ;
#34484=CARTESIAN_POINT ( 'NONE',  ( 7.037849409249268717, 158.0922581832940921, -1.451942896407524275 ) ) ;
#34485=CARTESIAN_POINT ( 'NONE',  ( -0.9532528233480704882, 157.3234082283764792, 1.521469375400507529 ) ) ;
#34486=CARTESIAN_POINT ( 'NONE',  ( 4.626035402534343532, 22.79242798913371360, 0.3558936578225105341 ) ) ;
#34487=CARTESIAN_POINT ( 'NONE',  ( -23.03149411880800912, 148.7220611141358404, -1.316198435982438575 ) ) ;
#34488=EDGE_CURVE ( 'NONE', #22232, #4990, #8352, .T. ) ;
#34489=CARTESIAN_POINT ( 'NONE',  ( 0.7093541224826089842, 23.24201423063343697, -0.6674325600367136957 ) ) ;
#34490=ORIENTED_EDGE ( 'NONE', *, *, #25321, .F. ) ;
#34492=CARTESIAN_POINT ( 'NONE',  ( -10.70072142757971889, 153.0728289088170300, 0.5595718250706017693 ) ) ;
#34493=CARTESIAN_POINT ( 'NONE',  ( 5.386302285778954868, -11.84411807400357475, 0.7125209553660817319 ) ) ;
#34494=CARTESIAN_POINT ( 'NONE',  ( 12.26974321764554965, 126.0625018263836807, -1.123002009909297438 ) ) ;
#34497=CARTESIAN_POINT ( 'NONE',  ( 0.7571409010366814130, 115.7028914826202595, 1.755555203384807861 ) ) ;
#34499=CARTESIAN_POINT ( 'NONE',  ( 2.253193219399967973, -14.99063959920543532, 5.175666457621841410 ) ) ;
#34500=CARTESIAN_POINT ( 'NONE',  ( -4.656554223671448334, 117.8898311454812244, -0.9968106679264355785 ) ) ;
#34501=CARTESIAN_POINT ( 'NONE',  ( 12.88210196283048248, 133.7932622986943159, 0.2101989309002757766 ) ) ;
#34504=CARTESIAN_POINT ( 'NONE',  ( 11.40914533023166832, 121.1873859956591843, 1.678693868224012009 ) ) ;
#34505=DIRECTION ( 'NONE',  ( -0.9998004120163609398, -4.016384292689130894E-17, -0.01997839162482749689 ) ) ;
#34508=CARTESIAN_POINT ( 'NONE',  ( 0.02874415600660452930, 157.0795416643300939, -1.438475106415293858 ) ) ;
#34509=AXIS2_PLACEMENT_3D ( 'NONE', #28850, #6280, #22846 ) ;
#34510=CARTESIAN_POINT ( 'NONE',  ( 9.765169485063754706, 118.0373187826741486, -0.07890504670268475018 ) ) ;
#34512=CARTESIAN_POINT ( 'NONE',  ( 1.680419162510425002, -15.45927319065069838, 5.515672785773912068 ) ) ;
#34515=ADVANCED_FACE ( 'NONE', ( #39916 ), #23690, .F. ) ;
#34516=CARTESIAN_POINT ( 'NONE',  ( -4.617919775738188015, 117.9735533346422187, 0.7423233486650107071 ) ) ;
#34521=CARTESIAN_POINT ( 'NONE',  ( -2.668721918458945019, 117.7585162296088583, -0.8088457382527453055 ) ) ;
#34522=CARTESIAN_POINT ( 'NONE',  ( -6.983090746392761616, 124.7321584522365896, -0.1405484879196982895 ) ) ;
#34523=CARTESIAN_POINT ( 'NONE',  ( 4.741947938571901666, 117.6342773529492547, 1.141888482007099137 ) ) ;
#34525=CARTESIAN_POINT ( 'NONE',  ( -1.012635771704909038, 123.9312678891798640, 0.06995516121779321583 ) ) ;
#34527=CARTESIAN_POINT ( 'NONE',  ( -3.832284926465886254, -5.753926550059754064, 2.584458424559757272 ) ) ;
#34528=CARTESIAN_POINT ( 'NONE',  ( 4.866147868668515564, 117.4089627612368076, -0.9906677743061890196 ) ) ;
#34530=CARTESIAN_POINT ( 'NONE',  ( 2.131140412894510838, -15.01828590152304344, 5.319755587316977952 ) ) ;
#34531=CARTESIAN_POINT ( 'NONE',  ( 5.235361408262197536, 116.2637919873444190, -0.9632728985350239581 ) ) ;
#34532=CARTESIAN_POINT ( 'NONE',  ( 7.787533423162888546, 122.6196153997145473, 0.09973116958504993357 ) ) ;
#34533=CARTESIAN_POINT ( 'NONE',  ( -6.346781410994640993, 30.04503731349425166, 1.591420273447384348 ) ) ;
#34534=CARTESIAN_POINT ( 'NONE',  ( -0.6270198638313982942, 115.7029626491897716, 1.737414609200174542 ) ) ;
#34535=CARTESIAN_POINT ( 'NONE',  ( 4.256838582791900194, 16.71066835407712858, 1.825063967593055558 ) ) ;
#34536=CARTESIAN_POINT ( 'NONE',  ( 22.84108495963309693, 150.1122123445777277, 1.048654020290956446 ) ) ;
#34538=CARTESIAN_POINT ( 'NONE',  ( 0.2171711340010081537, 104.6144662015456674, -4.831476934653068156 ) ) ;
#34539=CARTESIAN_POINT ( 'NONE',  ( 2.152540537132713538, -15.51301927577993034, 5.194954439406326507 ) ) ;
#34540=CARTESIAN_POINT ( 'NONE',  ( -15.79478014299093580, 153.2725199748809928, 1.714666983805330780 ) ) ;
#34541=CARTESIAN_POINT ( 'NONE',  ( -0.7801697309092696653, 18.27050645547500451, 0.5824522774875325881 ) ) ;
#34543=CARTESIAN_POINT ( 'NONE',  ( 0.9475510003767251277, 17.78785052102138664, 0.2306771022979090535 ) ) ;
#34548=CARTESIAN_POINT ( 'NONE',  ( 2.044121638888182435, 114.8832439220486350, 1.972317757894941570 ) ) ;
#34549=CARTESIAN_POINT ( 'NONE',  ( -1.473868052710668675, 120.2326517397585377, 0.4086940711265545922 ) ) ;
#34551=CARTESIAN_POINT ( 'NONE',  ( 3.494528270914563528, -13.06595970051097133, 2.012497701936279082 ) ) ;
#34552=CARTESIAN_POINT ( 'NONE',  ( 10.29797255167324010, 122.2012759285571946, -1.140151759267314047 ) ) ;
#34553=CARTESIAN_POINT ( 'NONE',  ( -13.17434061382168231, 122.5785676075921060, -1.825321299320728397 ) ) ;
#34556=CARTESIAN_POINT ( 'NONE',  ( 4.520495148372919658, 121.0527503406816123, -0.1761357111252131458 ) ) ;
#34557=ORIENTED_EDGE ( 'NONE', *, *, #6569, .F. ) ;
#34558=CARTESIAN_POINT ( 'NONE',  ( 2.993548201347409510, -14.88003303992029025, 3.932447912750371977 ) ) ;
#34559=CARTESIAN_POINT ( 'NONE',  ( 0.03201377673046579275, 33.52827609515317420, 3.383309648808628278 ) ) ;
#34562=CARTESIAN_POINT ( 'NONE',  ( -4.070821798575407158, -9.904843093959119216, 2.245307785351264407 ) ) ;
#34563=CARTESIAN_POINT ( 'NONE',  ( 9.825947633753759902, 123.3250567171901082, 1.189973159844531114 ) ) ;
#34564=CARTESIAN_POINT ( 'NONE',  ( -3.032836294544972056, 29.78154503720477919, 3.248403939658073281 ) ) ;
#34565=CARTESIAN_POINT ( 'NONE',  ( -5.480007210012731278, 117.5214873295501405, 0.6081561229113362499 ) ) ;
#34566=CARTESIAN_POINT ( 'NONE',  ( 0.6989348986720191892, -4.029744825116962303, 4.573446973323917142 ) ) ;
#34567=CARTESIAN_POINT ( 'NONE',  ( 9.538359384048550993, 124.8019839352694476, 0.1905991205270211042 ) ) ;
#34568=CARTESIAN_POINT ( 'NONE',  ( 7.363685156731384573, -6.572911479292511849, 4.144591825403105112 ) ) ;
#34570=CARTESIAN_POINT ( 'NONE',  ( 2.157000451504500482, 116.4221920678469928, -0.2562403356321266146 ) ) ;
#34571=CARTESIAN_POINT ( 'NONE',  ( 0.09221630143964076876, 107.6766875080336376, -4.614880812453268533 ) ) ;
#34574=CARTESIAN_POINT ( 'NONE',  ( -6.690270197923770645, -5.753818539685515709, 5.116497609988504891 ) ) ;
#34575=CARTESIAN_POINT ( 'NONE',  ( 1.551977928113887462, 118.1588881584012825, 0.8756194964229589983 ) ) ;
#34577=CARTESIAN_POINT ( 'NONE',  ( -6.564189886853176475E-14, 81.62746620154572952, -5.847435218134868453E-18 ) ) ;
#34578=CARTESIAN_POINT ( 'NONE',  ( 0.9632506926927688617, 123.2612876230388395, -0.1349244037310162458 ) ) ;
#34579=CARTESIAN_POINT ( 'NONE',  ( -22.86474403352236706, 150.1122123445777277, 0.1353427831800517178 ) ) ;
#34582=ORIENTED_EDGE ( 'NONE', *, *, #36900, .F. ) ;
#34583=CARTESIAN_POINT ( 'NONE',  ( -3.770027696949578289, 121.0935558011302930, -0.04039886233734658882 ) ) ;
#34584=CARTESIAN_POINT ( 'NONE',  ( 5.672040739448011237, -14.80640238898532601, 2.735881018706089129 ) ) ;
#34585=CARTESIAN_POINT ( 'NONE',  ( -18.67489051167937930, 151.9584835496716266, 1.528205706551668541 ) ) ;
#34586=CARTESIAN_POINT ( 'NONE',  ( 22.59612908711461188, 148.7221180073953235, -0.8559155618276410582 ) ) ;
#34587=CARTESIAN_POINT ( 'NONE',  ( -3.453265078539333288, 21.00871511114837276, -3.102408547967784092 ) ) ;
#34588=CARTESIAN_POINT ( 'NONE',  ( -22.45364888651512913, 150.7739627601066275, -0.8979154079963819202 ) ) ;
#34591=CARTESIAN_POINT ( 'NONE',  ( -5.563323361884090268, 116.7152635471598359, 0.01911022379953509695 ) ) ;
#34593=CARTESIAN_POINT ( 'NONE',  ( -16.76421760064445365, 140.0893442862094673, 1.556517483701108207 ) ) ;
#34595=CARTESIAN_POINT ( 'NONE',  ( 5.043395383124224196, 119.2220797256985350, -0.8992592568097312888 ) ) ;
#34596=CARTESIAN_POINT ( 'NONE',  ( -14.14688762606146177, 122.0820592118662091, -1.654226634644705651 ) ) ;
#34598=CARTESIAN_POINT ( 'NONE',  ( 0.6059414056332816934, 120.5739061664170606, -0.2722191786371236377 ) ) ;
#34600=CARTESIAN_POINT ( 'NONE',  ( -11.24613893767488548, 123.2561760277034324, -1.620791190024704953 ) ) ;
#34601=CARTESIAN_POINT ( 'NONE',  ( 3.662106647173574370, -15.69883703644059381, 4.006612474821164227 ) ) ;
#34603=CARTESIAN_POINT ( 'NONE',  ( -4.154103066237196273, 118.2394448457162497, -0.3903888767277005067 ) ) ;
#34606=CARTESIAN_POINT ( 'NONE',  ( 4.277613954752398584, 119.9149831030956932, 0.8793409099722719890 ) ) ;
#34609=CARTESIAN_POINT ( 'NONE',  ( -2.337594367139880003, 4.813278044257511823, 8.129740476481943645 ) ) ;
#34610=CARTESIAN_POINT ( 'NONE',  ( 1.586003330670501699, 156.2604006213118453, 0.2328413704193784128 ) ) ;
#34614=EDGE_LOOP ( 'NONE', ( #22645, #25055, #34827, #37861 ) ) ;
#34617=CARTESIAN_POINT ( 'NONE',  ( -7.846889724220757145, 122.2670687553216879, -0.7512547164983297554 ) ) ;
#34620=CARTESIAN_POINT ( 'NONE',  ( -0.001640166039862459230, 159.6041700698465036, 0.08208061555506504514 ) ) ;
#34623=CARTESIAN_POINT ( 'NONE',  ( -5.815556676244801437, 121.2350703429551686, -0.4688114442016741434 ) ) ;
#34624=CARTESIAN_POINT ( 'NONE',  ( -7.810699836270218910, 122.5400548736092645, 0.1271298722260623126 ) ) ;
#34625=VERTEX_POINT ( 'NONE', #23909 ) ;
#34626=CARTESIAN_POINT ( 'NONE',  ( 1.110063233458014054, 118.7629491485454025, -1.217940297164741059 ) ) ;
#34627=CARTESIAN_POINT ( 'NONE',  ( -15.55764736111898827, 147.5402044622178153, -0.6398501105574219139 ) ) ;
#34628=CARTESIAN_POINT ( 'NONE',  ( 5.898638393742167807, -12.20234047945549527, 0.6047796074133310329 ) ) ;
#34629=CARTESIAN_POINT ( 'NONE',  ( -21.49647223597101942, 141.8478887571778273, 1.286173174470951475 ) ) ;
#34631=CARTESIAN_POINT ( 'NONE',  ( 15.17534484293427610, 156.1124880001465556, 0.4370721430752774750 ) ) ;
#34632=CARTESIAN_POINT ( 'NONE',  ( 14.14780984094775995, 138.8477333867038226, 0.3490212194013133651 ) ) ;
#34633=FACE_OUTER_BOUND ( 'NONE', #16694, .T. ) ;
#34634=CARTESIAN_POINT ( 'NONE',  ( 0.8139239711521952803, 26.85569158835278003, 0.5393279072465841928 ) ) ;
#34635=CARTESIAN_POINT ( 'NONE',  ( -0.8904708500337824573, 116.4394364983335493, -0.05634004476769395586 ) ) ;
#34639=CARTESIAN_POINT ( 'NONE',  ( -8.528025516331789291, 119.1134116098120046, 0.9763900485721217493 ) ) ;
#34640=CARTESIAN_POINT ( 'NONE',  ( 0.5082173563136543892, -13.24086043563247728, -4.610200172643778238 ) ) ;
#34641=CARTESIAN_POINT ( 'NONE',  ( 10.85289063249347485, 119.5270080912504653, 1.298249717235596901 ) ) ;
#34642=CARTESIAN_POINT ( 'NONE',  ( 16.76200238010684984, 128.5636217276695561, -1.481418206722939335 ) ) ;
#34643=CARTESIAN_POINT ( 'NONE',  ( -7.510622214715407807, 18.91685342841953954, 3.806420843228597306 ) ) ;
#34644=CARTESIAN_POINT ( 'NONE',  ( -10.11685142855846564, 157.7687470436769388, -1.412159022929360574 ) ) ;
#34645=CARTESIAN_POINT ( 'NONE',  ( 4.824598637124480227, 117.6415664293784999, -0.9314390197744758515 ) ) ;
#34646=CARTESIAN_POINT ( 'NONE',  ( 6.508649675961964753, 120.6419738463991536, 0.3953840990482028750 ) ) ;
#34647=ORIENTED_EDGE ( 'NONE', *, *, #16675, .F. ) ;
#34648=CARTESIAN_POINT ( 'NONE',  ( -2.818990841020207139, 121.0122979933374978, 0.009253692138209404852 ) ) ;
#34649=CARTESIAN_POINT ( 'NONE',  ( -18.69815986816982800, 149.1225091032880528, -2.485088035475524038 ) ) ;
#34651=CARTESIAN_POINT ( 'NONE',  ( 2.074264724554232053, -15.58053249244904848, 5.900626476732238501 ) ) ;
#34653=DIRECTION ( 'NONE',  ( 4.017660918040594346E-17, -1.000000000000000000, -2.376309959284834438E-19 ) ) ;
#34656=CARTESIAN_POINT ( 'NONE',  ( 14.41820472940914932, 152.7616507467334372, 2.289036833064873822 ) ) ;
#34659=CARTESIAN_POINT ( 'NONE',  ( -2.040875107092424479, 122.5452913651401587, 0.1521094801190008561 ) ) ;
#34660=CARTESIAN_POINT ( 'NONE',  ( -6.568537450833661140, -2.023721358670699466, -5.272568914532883788 ) ) ;
#34661=CARTESIAN_POINT ( 'NONE',  ( 15.61785206596066899, 148.1291547725267037, 1.273309296088947828 ) ) ;
#34662=CARTESIAN_POINT ( 'NONE',  ( -5.167980139463525191, 115.6909491485453003, -1.237717243154890845 ) ) ;
#34663=CARTESIAN_POINT ( 'NONE',  ( 9.649066847268002789, 118.2334930433176652, -0.3843608719459136180 ) ) ;
#34668=VECTOR ( 'NONE', #4604, 1000.000000000000000 ) ;
#34669=CARTESIAN_POINT ( 'NONE',  ( -4.318590049495329097, 118.2119091611040886, 0.3227723479053775102 ) ) ;
#34670=CARTESIAN_POINT ( 'NONE',  ( -8.216926545874587262, 117.5004104479096583, -0.1641937475849288286 ) ) ;
#34673=VECTOR ( 'NONE', #31057, 1000.000000000000000 ) ;
#34674=CARTESIAN_POINT ( 'NONE',  ( 4.042069430835217858, 119.1497344468857875, -0.7634344030164779138 ) ) ;
#34675=CARTESIAN_POINT ( 'NONE',  ( -2.498958912387992282, 107.2142675576569530, -4.733253560342793875 ) ) ;
#34676=CARTESIAN_POINT ( 'NONE',  ( -9.680894551640223611, 124.1466939447965814, -0.8054060769509037154 ) ) ;
#34677=CARTESIAN_POINT ( 'NONE',  ( -6.474089935681887051E-14, 69.94346620154573202, 3.752704589293910110E-29 ) ) ;
#34681=CARTESIAN_POINT ( 'NONE',  ( 3.979181138743986601, 26.09377549647152961, 2.406711837290479661 ) ) ;
#34685=CARTESIAN_POINT ( 'NONE',  ( 7.784012320830338005, 122.6313477005580665, 0.1555430910899518460 ) ) ;
#34686=CARTESIAN_POINT ( 'NONE',  ( 6.999941501148388312, 121.9564690986170916, 0.1592458515995052726 ) ) ;
#34687=CARTESIAN_POINT ( 'NONE',  ( -2.673854242087471356, 19.56896771519852862, 3.769861741755948348 ) ) ;
#34688=CARTESIAN_POINT ( 'NONE',  ( 22.33788829447780344, 150.2360280492587776, 1.519312068210846300 ) ) ;
#34689=CARTESIAN_POINT ( 'NONE',  ( 3.957988466488265633, 104.6144662015457669, -2.766880044203430256 ) ) ;
#34690=CARTESIAN_POINT ( 'NONE',  ( 2.233078627056604759, -15.14192004606506536, 5.083345892419886880 ) ) ;
#34691=CARTESIAN_POINT ( 'NONE',  ( 5.881556420379451033, 118.2031694463412634, -0.8113220510518367456 ) ) ;
#34692=CARTESIAN_POINT ( 'NONE',  ( -2.217461812776308161, 157.2504501563031738, 1.545323669738358774 ) ) ;
#34693=CARTESIAN_POINT ( 'NONE',  ( 0.5230511744754561265, -14.76557578359995837, -0.8217837604668620788 ) ) ;
#34694=CARTESIAN_POINT ( 'NONE',  ( -9.590549175011975791, 118.2964180356302961, -0.8317573021886299767 ) ) ;
#34695=CARTESIAN_POINT ( 'NONE',  ( 0.7990752137124343957, 23.01725015362593396, -0.5559626729366093922 ) ) ;
#34696=ORIENTED_EDGE ( 'NONE', *, *, #30316, .T. ) ;
#34699=CARTESIAN_POINT ( 'NONE',  ( -8.758948435532792232, 123.3024417045633498, 0.2233049321804339571 ) ) ;
#34700=CARTESIAN_POINT ( 'NONE',  ( 5.009217890960311337, -13.99182267686448178, 3.873128360714999552 ) ) ;
#34701=CARTESIAN_POINT ( 'NONE',  ( 13.78713281179550876, 131.0408573235120571, -1.173264656791310534 ) ) ;
#34702=ORIENTED_EDGE ( 'NONE', *, *, #38026, .T. ) ;
#34703=CARTESIAN_POINT ( 'NONE',  ( 0.6180999634803059362, 115.7031371519886562, 1.759524179880340267 ) ) ;
#34704=CARTESIAN_POINT ( 'NONE',  ( -4.871873180668504943, 117.6697712886699350, -1.013429949543328989 ) ) ;
#34705=CARTESIAN_POINT ( 'NONE',  ( 8.507314851146803747, 123.3280575159016905, 0.1373787248657621640 ) ) ;
#34707=CARTESIAN_POINT ( 'NONE',  ( 15.05911097818674094, 125.5446871707752763, 2.024973821723874856 ) ) ;
#34711=CARTESIAN_POINT ( 'NONE',  ( 0.01887828017110892292, 156.5412816204240301, -0.9447463363288812754 ) ) ;
#34712=CARTESIAN_POINT ( 'NONE',  ( 13.52003375314293265, 119.6474162840860771, -0.03304800104807574523 ) ) ;
#34713=ADVANCED_FACE ( 'NONE', ( #34149 ), #30350, .F. ) ;
#34716=AXIS2_PLACEMENT_3D ( 'NONE', #11676, #24663, #12102 ) ;
#34717=CARTESIAN_POINT ( 'NONE',  ( 1.882827824557420815, -15.10077973259936535, 5.845967129181769195 ) ) ;
#34720=CARTESIAN_POINT ( 'NONE',  ( -4.833760488234558395, 117.8347844218319125, 0.7195636590734230120 ) ) ;
#34723=CARTESIAN_POINT ( 'NONE',  ( -3.249327724917783211, 118.4242012496010688, -0.9118293563264334711 ) ) ;
#34724=CARTESIAN_POINT ( 'NONE',  ( -4.774443427420668407, 116.8297769931967309, -1.047991251433075366 ) ) ;
#34726=CARTESIAN_POINT ( 'NONE',  ( 4.760793893673167076, 117.5395337211100326, 1.175852012856988926 ) ) ;
#34727=CARTESIAN_POINT ( 'NONE',  ( -4.748912967724773004, 117.5371765964522126, -1.178473615865876400 ) ) ;
#34728=CARTESIAN_POINT ( 'NONE',  ( -0.3798947725662609742, 120.3637084677653633, 0.5835535210198283806 ) ) ;
#34729=CARTESIAN_POINT ( 'NONE',  ( -3.974385726840726107, -7.478117039488521023, -2.359557994316856533 ) ) ;
#34732=CARTESIAN_POINT ( 'NONE',  ( 3.513860297840244673, -13.27766151250851756, 2.382095677556017588 ) ) ;
#34733=CARTESIAN_POINT ( 'NONE',  ( 5.907561988889377780, 118.9932487913337411, -0.3492918592308484338 ) ) ;
#34734=CARTESIAN_POINT ( 'NONE',  ( -5.838061318223103591, 120.4133487461328826, -1.005638731867922742 ) ) ;
#34735=CARTESIAN_POINT ( 'NONE',  ( 6.079477277396037493, 121.4435701191419952, 0.1217998136931948000 ) ) ;
#34736=CARTESIAN_POINT ( 'NONE',  ( -6.442297258278467886, 29.65178619621697464, 0.8020365093557799696 ) ) ;
#34737=CARTESIAN_POINT ( 'NONE',  ( -0.7270430668245355665, 115.7031259515097474, 1.730794492507717441 ) ) ;
#34738=CARTESIAN_POINT ( 'NONE',  ( 3.548611814566905664, 16.26088872207684943, 2.983771105379771971 ) ) ;
#34739=CARTESIAN_POINT ( 'NONE',  ( 0.9473015597125142850, 116.7004868406603322, 0.2634242240387512646 ) ) ;
#34741=CARTESIAN_POINT ( 'NONE',  ( 3.700359840729924521, 105.1233170995033959, -3.856631435510931905 ) ) ;
#34742=CARTESIAN_POINT ( 'NONE',  ( 4.296659151754357531, -15.58794764271442901, 2.529927869898711545 ) ) ;
#34743=CARTESIAN_POINT ( 'NONE',  ( -10.95471005835515577, 121.6366708983051836, 1.250572042008267548 ) ) ;
#34744=CARTESIAN_POINT ( 'NONE',  ( -0.9409916986186561694, 26.46864381685040257, -0.2619748070941995688 ) ) ;
#34746=CARTESIAN_POINT ( 'NONE',  ( -0.7871466699833823411, 12.39035052102135914, -0.5757299225971378442 ) ) ;
#34748=EDGE_LOOP ( 'NONE', ( #4586, #36533, #37, #10664 ) ) ;
#34750=CARTESIAN_POINT ( 'NONE',  ( 1.876195077988473292, 107.8038693663528278, 4.521701016168464093 ) ) ;
#34751=CARTESIAN_POINT ( 'NONE',  ( -12.88338908221817114, 130.8243885708800747, 0.7627239795610335493 ) ) ;
#34753=CARTESIAN_POINT ( 'NONE',  ( 3.416089938271958726, -12.71546774565127080, 1.400931973480754822 ) ) ;
#34754=CARTESIAN_POINT ( 'NONE',  ( 16.76421760064431865, 140.0893442862094673, -1.556517483701107984 ) ) ;
#34755=CARTESIAN_POINT ( 'NONE',  ( -14.32444608545413089, 154.4775811199918110, -2.255247442408088165 ) ) ;
#34758=CARTESIAN_POINT ( 'NONE',  ( -15.52687642492895037, 147.5330934759543879, -0.3102639428822864254 ) ) ;
#34759=CARTESIAN_POINT ( 'NONE',  ( -5.495523183683928004, 31.57050297546189199, 3.325088329614593885 ) ) ;
#34760=CARTESIAN_POINT ( 'NONE',  ( 11.98620439842957097, 151.9649008058812569, -0.3157042427443430554 ) ) ;
#34763=CARTESIAN_POINT ( 'NONE',  ( 3.096790694169950342, -14.35231825047024401, 1.054797312298405121 ) ) ;
#34765=EDGE_CURVE ( 'NONE', #38342, #10310, #18978, .T. ) ;
#34767=DIRECTION ( 'NONE',  ( 4.017660918040594346E-17, -1.000000000000000000, -2.376309959284834438E-19 ) ) ;
#34769=CARTESIAN_POINT ( 'NONE',  ( -4.449009123739010363, -11.09185097514761331, -1.246716907482375847 ) ) ;
#34770=CARTESIAN_POINT ( 'NONE',  ( 16.54853992722322786, 147.5857818452174115, 1.770514083359864266 ) ) ;
#34771=CARTESIAN_POINT ( 'NONE',  ( 3.682264917456193665, 63.33946620154573282, 0.07358041635423968885 ) ) ;
#34772=CARTESIAN_POINT ( 'NONE',  ( -6.497658445673645033, 120.6500652548963899, 0.1353193420278800130 ) ) ;
#34773=EDGE_CURVE ( 'NONE', #35331, #14379, #32436, .T. ) ;
#34774=CARTESIAN_POINT ( 'NONE',  ( -4.595132424582489605, -6.828429371805166959, -0.5093739664528403877 ) ) ;
#34775=CARTESIAN_POINT ( 'NONE',  ( 12.85860202769631755, 133.7716054015561156, 0.2569454702854388484 ) ) ;
#34776=CARTESIAN_POINT ( 'NONE',  ( 7.114778624005384522, 4.676967889965610858, -4.534447634950107719 ) ) ;
#34778=CARTESIAN_POINT ( 'NONE',  ( -8.740223524600960303, 117.9165407173578899, -0.6868026839525182003 ) ) ;
#34779=CARTESIAN_POINT ( 'NONE',  ( 0.01331772328987725074, 119.9741034315943864, -0.6664733318051296873 ) ) ;
#34781=DIRECTION ( 'NONE',  ( -4.017660918040594346E-17, 1.000000000000000000, 2.376309959284834438E-19 ) ) ;
#34783=CARTESIAN_POINT ( 'NONE',  ( -3.982871878373832164, -5.105173558950587775, 7.419718595111914894 ) ) ;
#34786=CARTESIAN_POINT ( 'NONE',  ( 0.9126123168628460514, 122.5862318000603182, -0.2067773319678722355 ) ) ;
#34787=CARTESIAN_POINT ( 'NONE',  ( -0.3287531253415878485, 116.7093555017326452, 0.2203909396130739051 ) ) ;
#34793=CARTESIAN_POINT ( 'NONE',  ( -8.871044653442362815, 123.8953218705242421, -0.08906294657775859491 ) ) ;
#34794=CARTESIAN_POINT ( 'NONE',  ( 2.825551972395176303, -15.60239892947398666, 5.624417742107700846 ) ) ;
#34795=CARTESIAN_POINT ( 'NONE',  ( -2.242939865367220342, 118.2767885243204944, 0.6835633642702236834 ) ) ;
#34796=CARTESIAN_POINT ( 'NONE',  ( 1.091392056212987960, 117.4935207075373569, -0.4954137919519207012 ) ) ;
#34797=CARTESIAN_POINT ( 'NONE',  ( 0.1710433496020407063, 14.98650505531991506, 4.637963194678765610 ) ) ;
#34798=CARTESIAN_POINT ( 'NONE',  ( -14.58714721168234796, 120.3300541288867862, -0.7025926276034525353 ) ) ;
#34801=CARTESIAN_POINT ( 'NONE',  ( 8.797014378848668770, 117.6856624139819445, 0.2140604904457499569 ) ) ;
#34803=CARTESIAN_POINT ( 'NONE',  ( -3.432158483474483379, 119.7942873563901713, 0.6544105580379842024 ) ) ;
#34804=CARTESIAN_POINT ( 'NONE',  ( -6.519774838065697039E-14, 78.83346620154574680, 1.207165459601591275E-19 ) ) ;
#34805=CARTESIAN_POINT ( 'NONE',  ( 1.037157837436363916, 157.7941190989783991, -1.604419329240821979 ) ) ;
#34807=CARTESIAN_POINT ( 'NONE',  ( -20.93418857319378645, 149.0309112320384486, -2.352213276463849034 ) ) ;
#34809=CARTESIAN_POINT ( 'NONE',  ( 3.624202338748673036, 120.7384399880717467, -0.3073100964232672316 ) ) ;
#34811=CARTESIAN_POINT ( 'NONE',  ( -12.41677917861200164, 153.6617311634574037, -2.127417120026096953 ) ) ;
#34812=CARTESIAN_POINT ( 'NONE',  ( 4.057567908148627112, -15.53776324113162488, 2.457816012360223290 ) ) ;
#34814=CARTESIAN_POINT ( 'NONE',  ( -4.250359704263266813, 118.2244096797001731, -0.4633146300828262509 ) ) ;
#34815=TOROIDAL_SURFACE ( 'NONE', #3549, 5.080000000000005400, 0.5080000000000000071 ) ;
#34817=CIRCLE ( 'NONE', #34716, 3.683000000000001162 ) ;
#34818=CARTESIAN_POINT ( 'NONE',  ( -4.825875739449531743, 117.4745444320467129, 0.9994230495043341378 ) ) ;
#34819=CARTESIAN_POINT ( 'NONE',  ( 10.01853622893594853, 122.3915136462027817, 1.471741716425344570 ) ) ;
#34820=FACE_BOUND ( 'NONE', #38275, .T. ) ;
#34822=EDGE_CURVE ( 'NONE', #6660, #1790, #20167, .T. ) ;
#34823=CARTESIAN_POINT ( 'NONE',  ( 4.223004820120735303, -0.3563183945215069870, -7.287282906663286930 ) ) ;
#34824=CARTESIAN_POINT ( 'NONE',  ( 15.55764736111886037, 147.5402044622178153, 0.6398501105574221359 ) ) ;
#34827=ORIENTED_EDGE ( 'NONE', *, *, #17569, .T. ) ;
#34828=CARTESIAN_POINT ( 'NONE',  ( -1.043075768918328983, 117.9394518566729033, 1.353628448391521077 ) ) ;
#34830=CARTESIAN_POINT ( 'NONE',  ( -7.962997644397243668, 121.6654936142849692, -1.110444070604056366 ) ) ;
#34833=CARTESIAN_POINT ( 'NONE',  ( -23.10641284836741960, 149.8968678342272653, -0.3080169626343541300 ) ) ;
#34836=CARTESIAN_POINT ( 'NONE',  ( 6.959716963148959046, 121.9406942131701754, -0.009715431953628055062 ) ) ;
#34839=CARTESIAN_POINT ( 'NONE',  ( 0.9195240100825864404, 115.7029491485453434, -1.717302178571716409 ) ) ;
#34840=CARTESIAN_POINT ( 'NONE',  ( -8.097005894254575509, 122.8525693413601800, -0.3074703907764577693 ) ) ;
#34841=CARTESIAN_POINT ( 'NONE',  ( 3.183750377336629356, -15.03749083096926675, 5.611903928707999256 ) ) ;
#34842=CARTESIAN_POINT ( 'NONE',  ( -10.77577921906396163, 119.6772744462923157, 0.9367561965627281273 ) ) ;
#34844=CIRCLE ( 'NONE', #40301, 3.683000000000001162 ) ;
#34845=CARTESIAN_POINT ( 'NONE',  ( 23.30140632484780383, 142.7201128741078833, 0.7978754358820902004 ) ) ;
#34846=CARTESIAN_POINT ( 'NONE',  ( 2.884051542275651414, 156.0957788938021054, 0.05763021347587640730 ) ) ;
#34847=B_SPLINE_CURVE_WITH_KNOTS ( 'NONE', 3,
 ( #18187, #8198, #24801, #4820 ),
 .UNSPECIFIED., .F., .F.,
 ( 4, 4 ),
 ( 0.000000000000000000, 1.000000000000000000 ),
 .UNSPECIFIED. ) ;
#34849=CARTESIAN_POINT ( 'NONE',  ( 0.1724166890850278577, 29.87817833284422875, -0.9617850639438362270 ) ) ;
#34850=CARTESIAN_POINT ( 'NONE',  ( -1.814945173922756227, 116.4909138135563040, -0.1082358691141156737 ) ) ;
#34854=CARTESIAN_POINT ( 'NONE',  ( -6.156441858550770085, 118.9979555525181496, 0.9955410089892811065 ) ) ;
#34855=CARTESIAN_POINT ( 'NONE',  ( 4.581716828367337513, -15.30239761468843973, -0.5121115983836379559 ) ) ;
#34856=CARTESIAN_POINT ( 'NONE',  ( 21.62407820142100690, 149.9601031839316079, 2.013249247985050783 ) ) ;
#34857=CARTESIAN_POINT ( 'NONE',  ( 12.92430874792252560, 121.9120276846612256, -1.237792553996327261 ) ) ;
#34858=CARTESIAN_POINT ( 'NONE',  ( 4.500746820419270655, 24.54286538861932598, -7.153999163526271410 ) ) ;
#34859=CARTESIAN_POINT ( 'NONE',  ( -7.493104803958972049, 158.4854300789945398, -1.293057490532128151 ) ) ;
#34860=CARTESIAN_POINT ( 'NONE',  ( 4.766322966312536380, 117.7281155096933674, -0.9072089781911022444 ) ) ;
#34861=CARTESIAN_POINT ( 'NONE',  ( 5.210105874137030746, 116.2501875120488393, 1.173469071234783723 ) ) ;
#34863=CARTESIAN_POINT ( 'NONE',  ( -5.999396524113779883, 155.3621521873626534, 0.05839828084409132841 ) ) ;
#34864=CARTESIAN_POINT ( 'NONE',  ( -18.57576200519322640, 149.2887123452801745, -2.480868434872863126 ) ) ;
#34865=CARTESIAN_POINT ( 'NONE',  ( 2.105506875138051459, -15.57594099408041188, 5.887502213194136580 ) ) ;
#34866=DIRECTION ( 'NONE',  ( -4.017660918040594346E-17, 1.000000000000000000, 2.376309959284834438E-19 ) ) ;
#34868=ORIENTED_EDGE ( 'NONE', *, *, #31919, .F. ) ;
#34869=CARTESIAN_POINT ( 'NONE',  ( 11.21148455117555898, 122.4230570912197038, 1.693600966768365357 ) ) ;
#34873=CARTESIAN_POINT ( 'NONE',  ( -3.079316153087905850, 123.1875568577169560, 0.05586128712921783340 ) ) ;
#34874=CARTESIAN_POINT ( 'NONE',  ( 2.619848522501802446, -13.46771402114085703, -8.002427727062926266 ) ) ;
#34875=CARTESIAN_POINT ( 'NONE',  ( 15.73537819279951755, 147.9505201145231865, 1.277015258756127869 ) ) ;
#34876=CARTESIAN_POINT ( 'NONE',  ( -4.727273527973792078, 118.5930653697794384, -1.020421541027422219 ) ) ;
#34878=CARTESIAN_POINT ( 'NONE',  ( 22.93637923037181992, 149.5023856264156450, -0.3943874666890923586 ) ) ;
#34884=AXIS2_PLACEMENT_3D ( 'NONE', #8194, #2027, #5020 ) ;
#34889=CARTESIAN_POINT ( 'NONE',  ( -8.215589217028934854, 120.4019796500743809, -1.435742804604346556 ) ) ;
#34890=CARTESIAN_POINT ( 'NONE',  ( -1.987587706212319727, 106.6795586461009009, -4.969950645211479667 ) ) ;
#34891=CARTESIAN_POINT ( 'NONE',  ( -8.259016884199036568, 122.7564308547279666, -0.6276379194545151918 ) ) ;
#34893=FACE_OUTER_BOUND ( 'NONE', #8924, .T. ) ;
#34895=CARTESIAN_POINT ( 'NONE',  ( 4.636458409304901274, 17.36039413176390411, -0.09481320587925551324 ) ) ;
#34900=CARTESIAN_POINT ( 'NONE',  ( -6.995832315028981618, 121.9523011290228283, -0.1203680031076684170 ) ) ;
#34902=CARTESIAN_POINT ( 'NONE',  ( 15.18175346423885230, 121.1469641333237917, 1.070035192906481303 ) ) ;
#34905=CARTESIAN_POINT ( 'NONE',  ( 21.50873886539572410, 148.9071063441643048, -1.383230070950766777 ) ) ;
#34906=CARTESIAN_POINT ( 'NONE',  ( -11.76378629788681174, 123.2143981803894093, 1.250304744737055440 ) ) ;
#34907=CARTESIAN_POINT ( 'NONE',  ( 0.4006815055314144058, 20.64345356492705719, 4.603752038498275745 ) ) ;
#34908=CARTESIAN_POINT ( 'NONE',  ( -2.883180212088917393, 116.9538966677400254, -0.4754005367760562040 ) ) ;
#34910=CARTESIAN_POINT ( 'NONE',  ( -0.06925455797148694081, -4.192134993018743927, -0.9746272421430232091 ) ) ;
#34911=B_SPLINE_CURVE_WITH_KNOTS ( 'NONE', 3,
 ( #40404, #1012, #594, #20150, #26771, #20352, #10995, #30588, #32965, #16959, #11198, #39781, #6974 ),
 .UNSPECIFIED., .F., .F.,
 ( 4, 1, 1, 1, 1, 1, 1, 1, 1, 1, 4 ),
 ( 0.000000000000000000, 0.1249999999999999167, 0.1767086109055020227, 0.2499999999999998335, 0.3750000000000003886, 0.5000000000000003331, 0.5890287030183404271, 0.6249999999999998890, 0.7499999999999995559, 0.8749999999999997780, 1.000000000000000000 ),
 .UNSPECIFIED. ) ;
#34914=CARTESIAN_POINT ( 'NONE',  ( -16.01386893308431780, 146.3393691146323761, 0.4087692286948390596 ) ) ;
#34916=CARTESIAN_POINT ( 'NONE',  ( 5.365742231761132963, -12.30384844886438245, 1.459887348375163096 ) ) ;
#34917=CARTESIAN_POINT ( 'NONE',  ( 12.98740932513240764, 152.2092440956282076, -1.257387005612584652 ) ) ;
#34919=CARTESIAN_POINT ( 'NONE',  ( 1.183385436418662007, 115.7029491485453008, 1.742418698461533522 ) ) ;
#34922=CARTESIAN_POINT ( 'NONE',  ( -4.825672693197581964, 117.7347280262817293, -1.017632466350065990 ) ) ;
#34924=CARTESIAN_POINT ( 'NONE',  ( 6.503408402854558013, 121.7799126398724354, 0.1299535771408518448 ) ) ;
#34926=CARTESIAN_POINT ( 'NONE',  ( 19.79373099999700258, 147.4002846799066333, 2.520905760949471386 ) ) ;
#34927=DIRECTION ( 'NONE',  ( 0.01997839162482749689, 1.040247600000945640E-18, -0.9998004120163610509 ) ) ;
#34928=CARTESIAN_POINT ( 'NONE',  ( 15.70103477329399766, 145.5797129992483292, 0.3137440411564567100 ) ) ;
#34930=CARTESIAN_POINT ( 'NONE',  ( 4.799155079147907621, 117.4716649492776241, -1.004620440989309138 ) ) ;
#34931=CARTESIAN_POINT ( 'NONE',  ( 20.20614143541403962, 128.9119615565081176, 0.01722291150864752388 ) ) ;
#34936=CARTESIAN_POINT ( 'NONE',  ( 1.753189578010867056, -15.12811351701386009, 5.597763803460143350 ) ) ;
#34938=CARTESIAN_POINT ( 'NONE',  ( -6.552964542248172189E-14, 78.83346620154574680, -6.511376220759049693E-18 ) ) ;
#34941=CARTESIAN_POINT ( 'NONE',  ( -4.751290763676331963, 117.9442343397520290, 0.6305581417652982301 ) ) ;
#34942=ORIENTED_EDGE ( 'NONE', *, *, #8676, .T. ) ;
#34944=CARTESIAN_POINT ( 'NONE',  ( -8.466947760633088294, 119.1862599057703846, -1.332611659245268365 ) ) ;
#34945=CARTESIAN_POINT ( 'NONE',  ( -3.094730188726814823, 108.9521120498200730, -4.030551393973050622 ) ) ;
#34946=CARTESIAN_POINT ( 'NONE',  ( 4.590341383356626892, 117.9757822827139222, 0.9229197263701504061 ) ) ;
#34947=CARTESIAN_POINT ( 'NONE',  ( 3.150244473240279675, -14.07033042043420146, 1.813758411523331393 ) ) ;
#34948=CARTESIAN_POINT ( 'NONE',  ( -0.4165637647021588341, 124.3520329708341023, 0.05485040398408839307 ) ) ;
#34953=CARTESIAN_POINT ( 'NONE',  ( 2.055333930833562750, 107.8038693663528278, -4.443139710053165103 ) ) ;
#34954=CARTESIAN_POINT ( 'NONE',  ( -0.5409540667465209118, 119.9180165495073283, -0.4819738915938376889 ) ) ;
#34955=CARTESIAN_POINT ( 'NONE',  ( 5.064182118629766194, 117.2683359310143913, -0.4803582174348582923 ) ) ;
#34956=CARTESIAN_POINT ( 'NONE',  ( -5.682669411112049040, 29.64564914382334138, 2.717066260770635289 ) ) ;
#34958=CARTESIAN_POINT ( 'NONE',  ( 2.829288187452689396, 6.340478445469713620, 3.655570690059357197 ) ) ;
#34959=CARTESIAN_POINT ( 'NONE',  ( 21.76232006938114694, 151.4242408681541008, 1.019401482499525891 ) ) ;
#34960=ORIENTED_EDGE ( 'NONE', *, *, #3230, .T. ) ;
#34961=CARTESIAN_POINT ( 'NONE',  ( 3.944319131782805243, 105.1226808459336866, -3.607269903450494919 ) ) ;
#34962=CARTESIAN_POINT ( 'NONE',  ( 4.174810697594108611, -15.62279056926031728, 2.935701831792822514 ) ) ;
#34963=CARTESIAN_POINT ( 'NONE',  ( -13.20509474233035263, 123.8872625266795211, 1.378179767694161395 ) ) ;
#34964=CARTESIAN_POINT ( 'NONE',  ( -0.07513956969218944792, 19.57165678886816096, 0.9711860325417217554 ) ) ;
#34965=CARTESIAN_POINT ( 'NONE',  ( -0.3507176028818052571, 11.51684809748499028, -0.9106068057588879716 ) ) ;
#34966=EDGE_CURVE ( 'NONE', #7672, #30817, #37874, .T. ) ;
#34967=EDGE_LOOP ( 'NONE', ( #38108, #38546, #20907, #8207 ) ) ;
#34968=VERTEX_POINT ( 'NONE', #26124 ) ;
#34970=CARTESIAN_POINT ( 'NONE',  ( 3.448667622495753982, 119.7720183225874138, 0.5479595714127597494 ) ) ;
#34971=CARTESIAN_POINT ( 'NONE',  ( -15.38818086081976766, 149.0334586719817764, 0.9521378535654884123 ) ) ;
#34973=CARTESIAN_POINT ( 'NONE',  ( 3.154356104639033820, -12.65568165217861818, 0.8785170097314246584 ) ) ;
#34974=CARTESIAN_POINT ( 'NONE',  ( 11.03120429849336226, 123.2082810311540300, -1.124825114493487321 ) ) ;
#34976=CARTESIAN_POINT ( 'NONE',  ( -19.08488522674174703, 150.4642993720107143, -2.434974558521497912 ) ) ;
#34979=CARTESIAN_POINT ( 'NONE',  ( 8.567507150466024513, 118.7110241784669427, 1.177141029754138479 ) ) ;
#34980=CARTESIAN_POINT ( 'NONE',  ( -5.871471797037544071, 31.01275966357848901, 2.875548327037550589 ) ) ;
#34981=CARTESIAN_POINT ( 'NONE',  ( 9.115521395012498473, 123.9337093609977529, -0.04715588286475763669 ) ) ;
#34983=ORIENTED_EDGE ( 'NONE', *, *, #16719, .F. ) ;
#34989=CARTESIAN_POINT ( 'NONE',  ( 5.629075615873821548, 21.71503808657377022, 6.277010319805454763 ) ) ;
#34990=CARTESIAN_POINT ( 'NONE',  ( 2.605661685743386968, 120.2926465633240127, 0.5460719465365780900 ) ) ;
#34991=DIRECTION ( 'NONE',  ( -4.017660918040594346E-17, 1.000000000000000000, 2.376309959284834438E-19 ) ) ;
#34992=CARTESIAN_POINT ( 'NONE',  ( 21.64725176087509340, 132.7051459832101443, 0.3678724904816470520 ) ) ;
#34993=CARTESIAN_POINT ( 'NONE',  ( -5.398477100378502591, 117.1940586887245388, 0.6826447346010612316 ) ) ;
#34995=CARTESIAN_POINT ( 'NONE',  ( 3.745621265272091716, -10.50169880513956322, -2.708184146228840294 ) ) ;
#34996=CARTESIAN_POINT ( 'NONE',  ( 15.76285804746341235, 145.9067145067653541, 0.3149794173055769919 ) ) ;
#34997=EDGE_CURVE ( 'NONE', #36577, #12023, #10376, .T. ) ;
#34998=CARTESIAN_POINT ( 'NONE',  ( -8.417729735924666556, -0.9468307554896212563, 0.2322036382352700989 ) ) ;
#34999=CARTESIAN_POINT ( 'NONE',  ( -2.143513273935226948, 116.5966001900618494, -0.4290450327811727860 ) ) ;
#35000=CARTESIAN_POINT ( 'NONE',  ( 0.09934209769091897901, 106.7790779034713324, -4.971484795507141285 ) ) ;
#35002=DIRECTION ( 'NONE',  ( 4.017660918040594346E-17, -1.000000000000000000, -2.376309959284834438E-19 ) ) ;
#35004=CARTESIAN_POINT ( 'NONE',  ( -6.147169039531121371, -7.901875862888119606, -5.777837204501876656 ) ) ;
#35005=CARTESIAN_POINT ( 'NONE',  ( 3.361427982427648065, 117.3993835122936247, 1.373626019692422817 ) ) ;
#35007=FACE_OUTER_BOUND ( 'NONE', #29011, .T. ) ;
#35008=CARTESIAN_POINT ( 'NONE',  ( 0.1698098321966529933, 106.7790779034713324, -4.970076682467829521 ) ) ;
#35009=CARTESIAN_POINT ( 'NONE',  ( -3.228502273017121560, 159.4348965051207756, 0.3922148187338913572 ) ) ;
#35015=CARTESIAN_POINT ( 'NONE',  ( -15.78555315239537116, 146.2345694261926496, -0.1810740433878625377 ) ) ;
#35016=CARTESIAN_POINT ( 'NONE',  ( 6.400388595320081642, -14.10124341269280990, -0.01754875274584842895 ) ) ;
#35017=CARTESIAN_POINT ( 'NONE',  ( -4.766456943369862920, 158.1906701298835856, 1.576320697809042937 ) ) ;
#35018=CARTESIAN_POINT ( 'NONE',  ( 0.008308726997667138792, 117.3658353995175503, -0.4158026747930029243 ) ) ;
#35019=CARTESIAN_POINT ( 'NONE',  ( 2.267534764145236803, 6.115564135048844108, 4.037922524061999141 ) ) ;
#35020=CARTESIAN_POINT ( 'NONE',  ( -0.9351853929029012580, 116.6346273530297850, -0.2267945756083741271 ) ) ;
#35022=ORIENTED_EDGE ( 'NONE', *, *, #14689, .F. ) ;
#35023=CARTESIAN_POINT ( 'NONE',  ( 0.3633380039124867733, 121.5961256765096152, 0.3912981906941394028 ) ) ;
#35025=CARTESIAN_POINT ( 'NONE',  ( -7.187319939301759497, 155.7895407640516510, 1.441898956427383416 ) ) ;
#35027=ADVANCED_FACE ( 'NONE', ( #3350 ), #25619, .F. ) ;
#35028=CARTESIAN_POINT ( 'NONE',  ( 18.37903003504434807, 149.1773161885088825, -1.724610598947830198 ) ) ;
#35029=CARTESIAN_POINT ( 'NONE',  ( -20.82642717637633822, 141.6159226613069109, -2.307662509007912366 ) ) ;
#35032=CARTESIAN_POINT ( 'NONE',  ( 15.71237885704634607, 143.6801599334541208, -0.6671153439278898478 ) ) ;
#35034=CARTESIAN_POINT ( 'NONE',  ( 0.01023306027084651924, 119.5380416804913324, -0.5121041807152041381 ) ) ;
#35035=CARTESIAN_POINT ( 'NONE',  ( 2.255636784185061749, -15.37476536804864580, 5.049411959999403621 ) ) ;
#35036=CARTESIAN_POINT ( 'NONE',  ( -4.109772556805769028, 118.2429491485453070, -0.3484531805798580795 ) ) ;
#35038=CARTESIAN_POINT ( 'NONE',  ( -4.810414185812548205, 117.7356259150898126, 0.8787797982406257979 ) ) ;
#35039=CARTESIAN_POINT ( 'NONE',  ( 17.71853448156623756, 146.5573550606970628, 2.243325415855148108 ) ) ;
#35040=CARTESIAN_POINT ( 'NONE',  ( 1.957912617769093311, 35.96399040732271857, -0.5992445403938203574 ) ) ;
#35041=CARTESIAN_POINT ( 'NONE',  ( 8.428375251627102216, -1.854023157342211903, -0.5381045032988257537 ) ) ;
#35042=CARTESIAN_POINT ( 'NONE',  ( 9.187421481788707212, 153.8854248570426080, 0.5770480568347668981 ) ) ;
#35045=CARTESIAN_POINT ( 'NONE',  ( -0.7553559341985174314, 117.3993842960191785, 1.459876094933623802 ) ) ;
#35048=CARTESIAN_POINT ( 'NONE',  ( -7.967423902850907957, 121.6429398603349057, -1.120207190759914484 ) ) ;
#35052=CARTESIAN_POINT ( 'NONE',  ( -23.20816695139205166, 149.6253602407241488, -0.3098579641399930029 ) ) ;
#35055=CARTESIAN_POINT ( 'NONE',  ( 6.952013292454969573, 121.9314134082488437, -0.04296861412470696223 ) ) ;
#35056=CARTESIAN_POINT ( 'NONE',  ( -7.903630729594187443, 122.1168884809555237, 0.5501188935067273800 ) ) ;
#35057=VERTEX_POINT ( 'NONE', #14168 ) ;
#35058=CARTESIAN_POINT ( 'NONE',  ( 1.574585577260951386, 115.7027553830524482, -1.670870382018978528 ) ) ;
#35059=CARTESIAN_POINT ( 'NONE',  ( -15.77366026095721274, 146.5725700477668170, -0.4436318658883099397 ) ) ;
#35060=CARTESIAN_POINT ( 'NONE',  ( 5.114911232981273592, -13.88689734646693452, 3.682185042294812582 ) ) ;
#35061=CARTESIAN_POINT ( 'NONE',  ( -2.147481372520724463, 117.7847241295267651, 0.6070331404035438361 ) ) ;
#35062=CARTESIAN_POINT ( 'NONE',  ( -6.617255152258657249E-14, 94.83546620154572793, -2.708805023911452991E-18 ) ) ;
#35063=CARTESIAN_POINT ( 'NONE',  ( 23.24214586660302118, 149.3282167461061931, 0.7955682979737043192 ) ) ;
#35064=CARTESIAN_POINT ( 'NONE',  ( 7.768456763902117146, 154.6794480478109222, 0.2667523075916575781 ) ) ;
#35066=CARTESIAN_POINT ( 'NONE',  ( 0.9616503885695291132, 8.288457568681202758, 0.1719041247055087540 ) ) ;
#35067=CARTESIAN_POINT ( 'NONE',  ( -16.27462974253343830, 121.4070763266325628, -0.3766275504196340829 ) ) ;
#35072=CARTESIAN_POINT ( 'NONE',  ( 2.308497710762058563, 116.4336050630576267, 0.3288393404144274168 ) ) ;
#35073=CARTESIAN_POINT ( 'NONE',  ( -0.09930934064637705894, -13.04092083763876175, -4.623607705436294957 ) ) ;
#35074=CARTESIAN_POINT ( 'NONE',  ( 13.86838617718231603, 121.5005676099359846, 1.565740997395133949 ) ) ;
#35075=CARTESIAN_POINT ( 'NONE',  ( 19.50252919055201062, 149.6234262069624492, -1.702160239338572412 ) ) ;
#35076=CARTESIAN_POINT ( 'NONE',  ( -8.331803066987694351, 8.350395779143005015, -1.420432620954584113 ) ) ;
#35077=CARTESIAN_POINT ( 'NONE',  ( -5.842876937034696461, 117.7475948868982698, -0.8887855332765350891 ) ) ;
#35078=CARTESIAN_POINT ( 'NONE',  ( 4.881271996281774328, 117.7524462357942099, -0.7532070458226111098 ) ) ;
#35079=EDGE_CURVE ( 'NONE', #32861, #31901, #41957, .T. ) ;
#35080=CARTESIAN_POINT ( 'NONE',  ( 6.487065698694983062, 120.6500652548963899, 0.3947850323583861898 ) ) ;
#35081=CARTESIAN_POINT ( 'NONE',  ( -10.41298992473528351, 153.0987333575537548, -0.09138415589099052605 ) ) ;
#35082=CARTESIAN_POINT ( 'NONE',  ( -18.91839881582121663, 147.5601278813269914, -2.482394308196493871 ) ) ;
#35083=CARTESIAN_POINT ( 'NONE',  ( 5.457633994894312224, -14.92472868577397804, 3.194711634204877804 ) ) ;
#35084=CARTESIAN_POINT ( 'NONE',  ( 4.726645377701876427, 118.5931160184169073, 1.020514608935862544 ) ) ;
#35085=CARTESIAN_POINT ( 'NONE',  ( -3.969859667707119844, 117.3993838098210745, -1.318277526388289989 ) ) ;
#35086=EDGE_LOOP ( 'NONE', ( #2684, #6200 ) ) ;
#35087=CARTESIAN_POINT ( 'NONE',  ( 4.201129436297820874, 119.4047208153655646, 0.9741049750989215772 ) ) ;
#35090=CARTESIAN_POINT ( 'NONE',  ( -0.7414234751012540592, 107.0594419416054848, 4.828671665556864667 ) ) ;
#35091=CARTESIAN_POINT ( 'NONE',  ( 3.771486885279011325, -13.69470344665998773, -7.544622693077620568 ) ) ;
#35092=CARTESIAN_POINT ( 'NONE',  ( 2.711066548582543145, 120.7183352303693340, 0.3631387678457471124 ) ) ;
#35094=CARTESIAN_POINT ( 'NONE',  ( 14.85158921512553931, 156.1223461918646933, -0.5575614454322267433 ) ) ;
#35097=CARTESIAN_POINT ( 'NONE',  ( -8.796272724451718261, 117.6874569103046184, -0.2327601223367594674 ) ) ;
#35099=CARTESIAN_POINT ( 'NONE',  ( -23.21373371908098449, 149.6306211361744829, -0.4638656453230912136 ) ) ;
#35101=CARTESIAN_POINT ( 'NONE',  ( -4.581230805175637855, 119.7013507852435907, -0.9162263165478330418 ) ) ;
#35102=CARTESIAN_POINT ( 'NONE',  ( 4.678875543802746506, 116.0444662015457737, -3.608683038041131663 ) ) ;
#35103=CARTESIAN_POINT ( 'NONE',  ( -9.301285777573651714, 153.8845013697122965, -0.8210809464416256587 ) ) ;
#35105=CARTESIAN_POINT ( 'NONE',  ( 20.69846590548368681, 152.5542719854981044, 0.4384689201006755077 ) ) ;
#35106=ORIENTED_EDGE ( 'NONE', *, *, #8389, .F. ) ;
#35107=CARTESIAN_POINT ( 'NONE',  ( 1.616848224653315569, 9.589005055319924864, -4.350374724214612243 ) ) ;
#35108=CARTESIAN_POINT ( 'NONE',  ( -5.224344491509385513, 105.1221337964526015, 1.129052726857179945 ) ) ;
#35109=CARTESIAN_POINT ( 'NONE',  ( -4.829025010785088057, 117.4037175691626800, 1.009844946545902733 ) ) ;
#35111=DIRECTION ( 'NONE',  ( -0.9998004120163608288, 0.000000000000000000, -0.01997839162482749342 ) ) ;
#35112=CARTESIAN_POINT ( 'NONE',  ( 6.069967830169430201, 121.4313382071030958, 0.2855943879085542370 ) ) ;
#35113=CARTESIAN_POINT ( 'NONE',  ( -4.282102574861781363, 27.11529131024228434, -1.748715980913516876 ) ) ;
#35114=CARTESIAN_POINT ( 'NONE',  ( 5.389281185859638335, 158.9671755112622122, 1.064713296837521916 ) ) ;
#35115=CARTESIAN_POINT ( 'NONE',  ( -1.034730806123546287, 104.6144662015457243, -4.723492537174234229 ) ) ;
#35117=CARTESIAN_POINT ( 'NONE',  ( 21.60128648486314518, 148.1022500232506616, -1.385191265705788100 ) ) ;
#35118=CARTESIAN_POINT ( 'NONE',  ( -2.469877670440149942, 119.5064228623769225, 0.6390414609872484553 ) ) ;
#35119=CARTESIAN_POINT ( 'NONE',  ( -4.621355134897683570, 27.56591289442953041, -0.4301045952606497025 ) ) ;
#35120=CARTESIAN_POINT ( 'NONE',  ( -17.89857548597121095, 125.1504969321615164, -1.218861057454596830 ) ) ;
#35124=CARTESIAN_POINT ( 'NONE',  ( -9.945677869405052718, 124.8826105625126530, 0.2455395418728892332 ) ) ;
#35125=CARTESIAN_POINT ( 'NONE',  ( 5.381753124113789255, -12.14417964010665330, 1.193960664996519094 ) ) ;
#35126=CARTESIAN_POINT ( 'NONE',  ( 1.906664127224543481, 156.5995568990359175, -1.114948187579593020 ) ) ;
#35128=CARTESIAN_POINT ( 'NONE',  ( -4.783699877145565438, 117.7666882364519836, -1.035143524469993359 ) ) ;
#35129=CARTESIAN_POINT ( 'NONE',  ( 11.03183784343224616, 128.0124916018596650, 0.2204423744267035301 ) ) ;
#35131=CARTESIAN_POINT ( 'NONE',  ( 20.09316625820287427, 147.7236477000422497, 2.507557202006583719 ) ) ;
#35132=CARTESIAN_POINT ( 'NONE',  ( 15.19943428492308080, 148.1072807477730748, 0.3037208696559882681 ) ) ;
#35134=CARTESIAN_POINT ( 'NONE',  ( 4.997288873896878592, 117.4043910709748104, -0.8233982764724142589 ) ) ;
#35135=CARTESIAN_POINT ( 'NONE',  ( 23.34493312772026030, 146.7646281656787437, 0.007662864037405868467 ) ) ;
#35136=( BOUNDED_CURVE ( )  B_SPLINE_CURVE ( 3, ( #17258, #30249, #36873, #24062 ),
 .UNSPECIFIED., .F., .T. ) 
 B_SPLINE_CURVE_WITH_KNOTS ( ( 4, 4 ),
 ( 0.1539179638657816873, 0.4253411113690419576 ),
 .UNSPECIFIED. ) 
 CURVE ( )  GEOMETRIC_REPRESENTATION_ITEM ( )  RATIONAL_B_SPLINE_CURVE ( ( 0.5738540613416667213, 0.4347666551225499165, 0.4921339822382616580, 0.7459560426888020013 ) ) 
 REPRESENTATION_ITEM ( '' )  );
#35138=CARTESIAN_POINT ( 'NONE',  ( 4.812253369269448022, 118.7629491485453030, 0.6571626099536693744 ) ) ;
#35140=CARTESIAN_POINT ( 'NONE',  ( 1.740236503711715343, -15.12629859915687369, 5.675635612196994195 ) ) ;
#35143=CARTESIAN_POINT ( 'NONE',  ( -4.592121672059828796, 118.0813459264795284, 0.5392318162658802372 ) ) ;
#35146=ORIENTED_EDGE ( 'NONE', *, *, #13693, .F. ) ;
#35148=CARTESIAN_POINT ( 'NONE',  ( 3.610368082249861388, 118.7437733682415058, -0.7930644133314173061 ) ) ;
#35149=CARTESIAN_POINT ( 'NONE',  ( -6.110436517261230271, 121.4157903421748301, -0.3281350463252857286 ) ) ;
#35150=CARTESIAN_POINT ( 'NONE',  ( 4.682529446909616588, 117.8402053342184530, 1.032763938081705524 ) ) ;
#35151=CARTESIAN_POINT ( 'NONE',  ( 2.994295736468014280, -14.77441112906794984, 3.968895097548184037 ) ) ;
#35152=CARTESIAN_POINT ( 'NONE',  ( -0.5861964566937933885, 120.4790399057546182, -0.3305540093316994277 ) ) ;
#35153=CARTESIAN_POINT ( 'NONE',  ( 3.501419995798253915, -2.955197114699519734, 3.043391175950921568 ) ) ;
#35156=CARTESIAN_POINT ( 'NONE',  ( 4.753511127315582563, 115.8251506319059843, -1.256829922054841786 ) ) ;
#35157=CARTESIAN_POINT ( 'NONE',  ( -11.37357585002895810, 124.5424752485109963, -1.510439678823544352 ) ) ;
#35159=CARTESIAN_POINT ( 'NONE',  ( -2.876480734726157173, 115.7032361094657631, 1.566537190358891163 ) ) ;
#35160=CARTESIAN_POINT ( 'NONE',  ( 1.111903444298625754, 15.29877551736591812, 4.515507465039587665 ) ) ;
#35161=CARTESIAN_POINT ( 'NONE',  ( 1.889792677999337700, 116.7132768022172797, 0.3078404110637331659 ) ) ;
#35163=CARTESIAN_POINT ( 'NONE',  ( 3.348477637022819309, 104.6144662015456959, -3.488726040212962953 ) ) ;
#35164=CARTESIAN_POINT ( 'NONE',  ( 3.716361853963529249, -15.42594482578084403, 2.788391211141477921 ) ) ;
#35165=CARTESIAN_POINT ( 'NONE',  ( -17.18700207657779089, 151.3967157021085654, 1.745027292404997654 ) ) ;
#35166=CARTESIAN_POINT ( 'NONE',  ( 0.3309596775784566236, 20.21946177965197222, 0.9160044982600296093 ) ) ;
#35168=CARTESIAN_POINT ( 'NONE',  ( -0.5393284202071846334, 5.265691905141185458, 0.8139242273222374591 ) ) ;
#35171=VERTEX_POINT ( 'NONE', #7802 ) ;
#35173=CARTESIAN_POINT ( 'NONE',  ( 3.099458292114882774, 117.0475107411037641, 1.222660999933594672 ) ) ;
#35174=CARTESIAN_POINT ( 'NONE',  ( -12.34427413551901509, 128.4316967252784991, 0.8534409008407578545 ) ) ;
#35175=CARTESIAN_POINT ( 'NONE',  ( -12.85860202769644545, 133.7716054015561156, -0.2569454702854386263 ) ) ;
#35176=CARTESIAN_POINT ( 'NONE',  ( 2.509002420848308823, -14.82469439542799527, 5.007744185041904217 ) ) ;
#35177=CARTESIAN_POINT ( 'NONE',  ( 17.67426794430086900, 144.4767212251450417, -1.594784396078125166 ) ) ;
#35179=CARTESIAN_POINT ( 'NONE',  ( -13.83536887852640440, 154.2684476645699760, -2.291766773079779274 ) ) ;
#35181=CARTESIAN_POINT ( 'NONE',  ( 7.948490438896031129, 121.7395506310447217, 1.077254804507452812 ) ) ;
#35182=CARTESIAN_POINT ( 'NONE',  ( -2.330492536650612845, 35.40100364009314404, 2.787243435389755941 ) ) ;
#35183=CARTESIAN_POINT ( 'NONE',  ( 5.918555687551686262, 121.5031286879076902, -0.05579296748036344233 ) ) ;
#35186=CARTESIAN_POINT ( 'NONE',  ( -1.615419284005069400, 106.5834530906608819, -5.022566955870309435 ) ) ;
#35188=DIRECTION ( 'NONE',  ( -0.9998004120163608288, 0.000000000000000000, -0.01997839162482749342 ) ) ;
#35190=CARTESIAN_POINT ( 'NONE',  ( -8.047487967707532164, 27.33737370333709649, -2.486188741727015206 ) ) ;
#35191=CARTESIAN_POINT ( 'NONE',  ( 14.71707226966671023, 150.5114039713088516, 1.846696807168831223 ) ) ;
#35192=DIRECTION ( 'NONE',  ( -5.206863593109713661E-17, 1.000000000000000000, -1.077750396879097183E-30 ) ) ;
#35193=CARTESIAN_POINT ( 'NONE',  ( 23.29076518286600361, 149.3500807853454546, 0.3882996703880465250 ) ) ;
#35194=CARTESIAN_POINT ( 'NONE',  ( -2.658992269297188127, 107.2388417251876547, 4.621886736208384860 ) ) ;
#35197=CARTESIAN_POINT ( 'NONE',  ( 4.599243292695290641, 121.2024757821991159, 0.09190382657876450256 ) ) ;
#35199=CARTESIAN_POINT ( 'NONE',  ( 13.73566407960799296, 122.1113760975138263, 1.718532046871276808 ) ) ;
#35200=CARTESIAN_POINT ( 'NONE',  ( -8.389224625646681588, -1.175411479303250628, -1.011143247504549869 ) ) ;
#35201=CARTESIAN_POINT ( 'NONE',  ( -5.484251324081573564, 117.2052654494406454, -0.8040846112588506678 ) ) ;
#35202=CARTESIAN_POINT ( 'NONE',  ( -0.3796903751653987746, 122.8649044353670803, -0.2268226101886973156 ) ) ;
#35204=CARTESIAN_POINT ( 'NONE',  ( 3.524443185806435341, 109.1382852134488104, -3.813950880701249879 ) ) ;
#35205=CARTESIAN_POINT ( 'NONE',  ( -4.050807963365556930, 30.95410787014092335, -2.229501126309402448 ) ) ;
#35206=CARTESIAN_POINT ( 'NONE',  ( 1.086073555308449290, 117.3993836040883423, 1.476595440916665058 ) ) ;
#35208=CARTESIAN_POINT ( 'NONE',  ( 1.979956398862833922, -15.17398463081316784, 5.317940750273952411 ) ) ;
#35209=CARTESIAN_POINT ( 'NONE',  ( 0.7907195946116533092, 120.5370721568272216, -0.4966358104988963240 ) ) ;
#35210=CARTESIAN_POINT ( 'NONE',  ( -22.56840570087990017, 150.3096427868838987, 0.3971349512683052252 ) ) ;
#35211=CIRCLE ( 'NONE', #1231, 0.5080000000000002292 ) ;
#35212=ORIENTED_EDGE ( 'NONE', *, *, #31584, .T. ) ;
#35214=ORIENTED_EDGE ( 'NONE', *, *, #29131, .T. ) ;
#35216=CARTESIAN_POINT ( 'NONE',  ( 4.496247062743834455, -15.66418688627994804, 3.575535799018406014 ) ) ;
#35217=CARTESIAN_POINT ( 'NONE',  ( -9.147047865982875336, 157.1510513929294177, 1.627767162235162601 ) ) ;
#35218=CARTESIAN_POINT ( 'NONE',  ( 21.39260515875391633, 150.3702682424204511, -1.149856210633945608 ) ) ;
#35219=CARTESIAN_POINT ( 'NONE',  ( -4.399545650080316506, 2.442302885307133131, -1.471791394725967095 ) ) ;
#35220=ADVANCED_FACE ( 'NONE', ( #1001 ), #26281, .T. ) ;
#35222=EDGE_LOOP ( 'NONE', ( #11923, #20470 ) ) ;
#35224=CARTESIAN_POINT ( 'NONE',  ( -0.1065646865916383690, 105.8844662015456919, 5.332932678536313809 ) ) ;
#35225=CARTESIAN_POINT ( 'NONE',  ( -5.946078212987909062, 28.42590610009757413, 0.3016625663984517924 ) ) ;
#35226=CARTESIAN_POINT ( 'NONE',  ( -10.84039127762421195, 123.6843197456346672, 1.011594478071749847 ) ) ;
#35228=CARTESIAN_POINT ( 'NONE',  ( 16.64003893621117314, 151.1890201267100906, -1.733044620493700672 ) ) ;
#35229=CARTESIAN_POINT ( 'NONE',  ( -20.86684145051977879, 149.6610172957225586, -2.296701127946504606 ) ) ;
#35231=CIRCLE ( 'NONE', #2580, 0.5080000000000002292 ) ;
#35233=CARTESIAN_POINT ( 'NONE',  ( 9.814938192569819364, 124.1138826855306831, -0.4990610963926596644 ) ) ;
#35234=VERTEX_POINT ( 'NONE', #33366 ) ;
#35235=CARTESIAN_POINT ( 'NONE',  ( -17.88897823598650305, 147.4621342421176848, -2.293131556269223381 ) ) ;
#35236=CARTESIAN_POINT ( 'NONE',  ( 3.520778385322295811, -15.02221911624387829, 1.583774285062736986 ) ) ;
#35237=CARTESIAN_POINT ( 'NONE',  ( -4.223640366674269231, 118.2238299684479301, -0.4905063076566205105 ) ) ;
#35239=CARTESIAN_POINT ( 'NONE',  ( -4.981834297919686350, 117.5302800348309518, 0.7676192988303492948 ) ) ;
#35240=CARTESIAN_POINT ( 'NONE',  ( 13.61432229890752943, 152.4534842159446271, 2.088615715084950697 ) ) ;
#35243=CARTESIAN_POINT ( 'NONE',  ( 2.163044864548389956, 28.58015952483584954, -4.087059112497700042 ) ) ;
#35244=CARTESIAN_POINT ( 'NONE',  ( 10.47888833811890130, 153.0637448873655728, 0.6176438153593470926 ) ) ;
#35255=CARTESIAN_POINT ( 'NONE',  ( -23.32076472591260341, 148.8446908248229477, -0.1342014517686427599 ) ) ;
#35256=ORIENTED_EDGE ( 'NONE', *, *, #26310, .F. ) ;
#35258=CARTESIAN_POINT ( 'NONE',  ( 7.835216397241184794, 122.4239432713123961, -0.2785063474257676863 ) ) ;
#35259=CARTESIAN_POINT ( 'NONE',  ( 4.901676919075300454, 117.4083593258483660, -0.9680037761291583331 ) ) ;
#35261=CARTESIAN_POINT ( 'NONE',  ( 2.452571136908805016, 115.7029491485453718, -1.604305510785485556 ) ) ;
#35262=CARTESIAN_POINT ( 'NONE',  ( -7.564868681920799531, 122.4257779438054285, -0.2276018551017723324 ) ) ;
#35263=CARTESIAN_POINT ( 'NONE',  ( 2.291753010757021869, -15.38865404460348962, 5.937071240476925027 ) ) ;
#35264=CARTESIAN_POINT ( 'NONE',  ( -21.59954917983698408, 148.3057046726078170, 1.384394358321686669 ) ) ;
#35266=CARTESIAN_POINT ( 'NONE',  ( 16.80483327138715310, 155.2524275687165982, 0.6336504121414452406 ) ) ;
#35267=CARTESIAN_POINT ( 'NONE',  ( 4.201361461317214996, 155.8715872134815754, 0.1795330533319696442 ) ) ;
#35269=CARTESIAN_POINT ( 'NONE',  ( -0.4793318477812648082, 11.74037758575859058, -0.8492235504747065455 ) ) ;
#35270=CARTESIAN_POINT ( 'NONE',  ( -4.732570698819529298, 116.7698466342620378, -0.1749797587976939517 ) ) ;
#35274=CARTESIAN_POINT ( 'NONE',  ( -8.638482609000943668, 118.5544449468999915, 0.7679241716596895140 ) ) ;
#35277=CARTESIAN_POINT ( 'NONE',  ( 7.226289359486251840, 158.3006260280594404, 1.552328403643545185 ) ) ;
#35278=CARTESIAN_POINT ( 'NONE',  ( 20.02944843481977699, 148.6304843473828043, -1.700276915703843983 ) ) ;
#35279=CARTESIAN_POINT ( 'NONE',  ( -7.798946185677827714, 9.198776092563324625, 3.184250115244839030 ) ) ;
#35280=CARTESIAN_POINT ( 'NONE',  ( -5.309498559578598176, 158.9031408473208273, -1.190161311236993091 ) ) ;
#35281=CARTESIAN_POINT ( 'NONE',  ( 4.797843704864214409, 117.8843084929736733, -0.6937365112328826022 ) ) ;
#35282=DIRECTION ( 'NONE',  ( 0.9998004120163609398, 0.000000000000000000, 0.01997839162482749689 ) ) ;
#35283=CARTESIAN_POINT ( 'NONE',  ( -3.740144479511176900, 121.0798372856833538, -0.007817740762067527244 ) ) ;
#35284=CARTESIAN_POINT ( 'NONE',  ( -11.41083474541188814, 122.2847249198043471, -1.726555165334429764 ) ) ;
#35285=CARTESIAN_POINT ( 'NONE',  ( 5.792286216032899837, -14.99041835605292938, 0.9165201714659111376 ) ) ;
#35288=ADVANCED_FACE ( 'NONE', ( #10771 ), #3127, .F. ) ;
#35290=CARTESIAN_POINT ( 'NONE',  ( 11.57159210561016138, 122.7176759045101022, 1.727280539041415874 ) ) ;
#35294=CARTESIAN_POINT ( 'NONE',  ( -0.1065646865916159980, 105.8844662015457061, 5.332932678536314697 ) ) ;
#35295=CARTESIAN_POINT ( 'NONE',  ( 8.391146056172745560, -15.30543149186461527, -0.4349570568239987667 ) ) ;
#35296=CARTESIAN_POINT ( 'NONE',  ( 15.91132205781015863, 147.3275361421020193, 1.167720536598261027 ) ) ;
#35297=CARTESIAN_POINT ( 'NONE',  ( 3.862028650946859543, 117.0275016673472663, -0.3788463918649357387 ) ) ;
#35301=CARTESIAN_POINT ( 'NONE',  ( -15.97340373827834270, 121.0409387471171101, -0.3191866212789524204 ) ) ;
#35304=CARTESIAN_POINT ( 'NONE',  ( 8.266801410408760376, 120.3999688492377942, -1.106489660158431754 ) ) ;
#35305=LINE ( 'NONE', #39342, #27166 ) ;
#35306=CARTESIAN_POINT ( 'NONE',  ( -9.627236290563509158, 124.2480737032941533, -0.7173579674491835645 ) ) ;
#35308=CARTESIAN_POINT ( 'NONE',  ( 18.63389541082830192, 154.1203422869290023, 0.3962720605433153187 ) ) ;
#35309=ORIENTED_EDGE ( 'NONE', *, *, #39114, .T. ) ;
#35310=CARTESIAN_POINT ( 'NONE',  ( -3.789191232057584902, 13.46218022696137773, 2.646434746401360893 ) ) ;
#35312=CARTESIAN_POINT ( 'NONE',  ( -4.854821967544332928, 117.4083635672741366, 0.9981540133063625531 ) ) ;
#35313=CARTESIAN_POINT ( 'NONE',  ( -6.654617103318593247E-14, 104.6144662015457243, 1.534725424433578570E-31 ) ) ;
#35314=CARTESIAN_POINT ( 'NONE',  ( -4.468667403750213651, 27.88063884994054220, 0.5133561255362272258 ) ) ;
#35315=CARTESIAN_POINT ( 'NONE',  ( 7.950778463150458997, 121.7274446046149450, 1.085857570170044140 ) ) ;
#35317=CARTESIAN_POINT ( 'NONE',  ( 4.453423564604278795, 13.74662854910535792, -1.294644163995742225 ) ) ;
#35318=CARTESIAN_POINT ( 'NONE',  ( 3.066799924081360817, 159.2904672602661549, 0.9578552656232323104 ) ) ;
#35320=CARTESIAN_POINT ( 'NONE',  ( 2.768561164044480272, -13.57843041371762460, 0.3119852368007841603 ) ) ;
#35321=CARTESIAN_POINT ( 'NONE',  ( 4.917623111643079525, 158.3981005702974016, -1.478962986009813463 ) ) ;
#35322=CARTESIAN_POINT ( 'NONE',  ( -15.17272240541839778, 131.2890697635526465, 1.517944203131903258 ) ) ;
#35323=CARTESIAN_POINT ( 'NONE',  ( 3.087053954869741101, 14.59627045569285286, -3.440871586639639990 ) ) ;
#35324=CARTESIAN_POINT ( 'NONE',  ( -9.626009506019258311, 118.2334930433176652, -0.7695227696168690512 ) ) ;
#35325=EDGE_LOOP ( 'NONE', ( #19623, #14220, #6040, #12963 ) ) ;
#35326=CARTESIAN_POINT ( 'NONE',  ( -14.81827458270682918, 148.8567844064068026, 0.2884810962875102858 ) ) ;
#35327=CARTESIAN_POINT ( 'NONE',  ( 5.879588643049518559, -13.10657381646278274, 1.873965859954596969 ) ) ;
#35329=CARTESIAN_POINT ( 'NONE',  ( -4.574660132527480272, 118.0200319299317329, -0.8704685883761965615 ) ) ;
#35330=CARTESIAN_POINT ( 'NONE',  ( 15.26332761227456913, 148.0152273645666980, 0.2540164781927349846 ) ) ;
#35331=VERTEX_POINT ( 'NONE', #40594 ) ;
#35332=CARTESIAN_POINT ( 'NONE',  ( 19.80203545474858018, 147.6055923437354238, 2.520003004638577515 ) ) ;
#35335=CARTESIAN_POINT ( 'NONE',  ( -22.38075128446561379, 150.2360280492587776, 0.6257272249761320904 ) ) ;
#35336=CARTESIAN_POINT ( 'NONE',  ( 0.001367086239699496575, 156.3041635968983485, -0.06841458569046195148 ) ) ;
#35337=CARTESIAN_POINT ( 'NONE',  ( 0.003550357975883500824, 159.5989787797044812, -0.1776744311461873616 ) ) ;
#35339=VECTOR ( 'NONE', #32578, 1000.000000000000227 ) ;
#35343=CARTESIAN_POINT ( 'NONE',  ( 2.143789057001533660, -15.08792135351709440, 5.678686283222974751 ) ) ;
#35346=CARTESIAN_POINT ( 'NONE',  ( -6.111026219684664010E-14, 94.83546620154572793, 9.844778328339670704E-17 ) ) ;
#35347=CARTESIAN_POINT ( 'NONE',  ( -4.569938957122442247, 118.0881010721686692, 0.5676615755902681970 ) ) ;
#35350=CARTESIAN_POINT ( 'NONE',  ( -8.367821637836184934, 119.6608375418318673, -1.423109165391701847 ) ) ;
#35351=CARTESIAN_POINT ( 'NONE',  ( -0.1497278248017035740, 105.8844662015457629, -5.338012126719978490 ) ) ;
#35352=CARTESIAN_POINT ( 'NONE',  ( 4.680159262726512281, 117.9616872321280994, 0.8793832278182402984 ) ) ;
#35354=CARTESIAN_POINT ( 'NONE',  ( -2.668671847104423289, 120.5579296053302727, -0.4429723278990744251 ) ) ;
#35355=CARTESIAN_POINT ( 'NONE',  ( -4.337156242749934165, 111.8943083658765119, 2.742175979689941645 ) ) ;
#35357=CARTESIAN_POINT ( 'NONE',  ( 6.321818188556049378, 120.0717973201777511, -0.2011600071967685199 ) ) ;
#35358=CARTESIAN_POINT ( 'NONE',  ( -9.120583164541152144, 155.0058477609193801, -1.824713877226967762 ) ) ;
#35359=LINE ( 'NONE', #22128, #19404 ) ;
#35361=CARTESIAN_POINT ( 'NONE',  ( -2.370637312493784954, 115.7028718339712867, 1.611039750900896017 ) ) ;
#35362=CARTESIAN_POINT ( 'NONE',  ( -4.319812470756069445, 11.96289413176386951, -1.686699837767231536 ) ) ;
#35363=CARTESIAN_POINT ( 'NONE',  ( 20.48075987368136452, 152.5656283612522657, 1.113479615819600532 ) ) ;
#35365=CARTESIAN_POINT ( 'NONE',  ( 4.895972490868764737, 105.1214892841856994, -2.148021949592362478 ) ) ;
#35366=CARTESIAN_POINT ( 'NONE',  ( 3.518836906362542205, -15.09289160254213868, 2.194652486238897193 ) ) ;
#35367=CARTESIAN_POINT ( 'NONE',  ( -19.53500017296066815, 148.0998626603252148, 1.736236475658778255 ) ) ;
#35368=CARTESIAN_POINT ( 'NONE',  ( 0.9269407327955943021, 12.00036500698010578, 0.3089908296573128932 ) ) ;
#35369=CARTESIAN_POINT ( 'NONE',  ( -0.2812775050834619428, 1.806455656379289287, -0.9370761103187740249 ) ) ;
#35372=ORIENTED_EDGE ( 'NONE', *, *, #11028, .T. ) ;
#35374=CARTESIAN_POINT ( 'NONE',  ( 6.983605877934210504, 124.9344662015457175, 0.1395490654994195612 ) ) ;
#35376=CARTESIAN_POINT ( 'NONE',  ( -16.33963436279749715, 146.4745453488731357, 0.7896242330311489255 ) ) ;
#35377=CARTESIAN_POINT ( 'NONE',  ( -7.784012322544769269, 122.6313477034873074, -0.1555430911242075831 ) ) ;
#35378=CARTESIAN_POINT ( 'NONE',  ( 2.626143189074743756, -14.75305764222682647, 4.894789397842846945 ) ) ;
#35379=CARTESIAN_POINT ( 'NONE',  ( 11.26369337785505742, 123.4744472594011739, -1.139971239082960830 ) ) ;
#35380=CARTESIAN_POINT ( 'NONE',  ( -19.55492868859755617, 148.8045834396381508, -2.507096624874099344 ) ) ;
#35382=CARTESIAN_POINT ( 'NONE',  ( 7.889029732257585081, 122.0453901860990982, 0.9157283810244409850 ) ) ;
#35383=CARTESIAN_POINT ( 'NONE',  ( -6.004997167832389238, 30.93677315496120173, -0.5383843454024033193 ) ) ;
#35384=CARTESIAN_POINT ( 'NONE',  ( 15.72482880707709541, 147.2451778420852406, -0.1375710997406973113 ) ) ;
#35385=ORIENTED_EDGE ( 'NONE', *, *, #15894, .F. ) ;
#35389=CARTESIAN_POINT ( 'NONE',  ( 5.007985129730328389, 117.3993836135851438, -0.7769739375564292949 ) ) ;
#35390=CARTESIAN_POINT ( 'NONE',  ( -3.263082884110522386, 19.99377609092593389, 7.766292582686701529 ) ) ;
#35391=CARTESIAN_POINT ( 'NONE',  ( 9.075659781537913418, 123.1184971541203055, 0.9241268708344096972 ) ) ;
#35393=CARTESIAN_POINT ( 'NONE',  ( 1.421877081889598937, 159.6054662015457666, 0.01472409299311864921 ) ) ;
#35394=CARTESIAN_POINT ( 'NONE',  ( -5.252825482164497295, 116.2501875120488393, 0.9643948023431454519 ) ) ;
#35397=CARTESIAN_POINT ( 'NONE',  ( 1.104432469574216480, -9.427232690354344413, -4.492858291722996888 ) ) ;
#35398=CARTESIAN_POINT ( 'NONE',  ( 0.3395595041295305649, 35.30132035414327873, -0.2191788681752833978 ) ) ;
#35400=CARTESIAN_POINT ( 'NONE',  ( 20.91256836843372469, 148.0559997909317644, 2.401931445155506939 ) ) ;
#35401=CARTESIAN_POINT ( 'NONE',  ( -5.887876509958990923, -9.367530720701759961, 6.022233148990229878 ) ) ;
#35402=CARTESIAN_POINT ( 'NONE',  ( 2.179975478414604595, 116.7279437644658344, -0.4024351897304699333 ) ) ;
#35403=CARTESIAN_POINT ( 'NONE',  ( -0.3920235582992755985, 123.4679809879532542, -0.1617017839830490744 ) ) ;
#35406=CARTESIAN_POINT ( 'NONE',  ( -3.571940676414631533, 104.6144662015457243, 3.260099874920956431 ) ) ;
#35407=CARTESIAN_POINT ( 'NONE',  ( -2.923568588381722844, 13.88697512809157786, 3.594856661414283394 ) ) ;
#35409=DIRECTION ( 'NONE',  ( 0.01997839162482760444, 1.040247600000950455E-18, -0.9998004120163609398 ) ) ;
#35410=CARTESIAN_POINT ( 'NONE',  ( 2.932272473696061255, -14.72556872895393276, 4.151486945341092749 ) ) ;
#35411=CARTESIAN_POINT ( 'NONE',  ( 2.738288815228959727, 121.4869043954268903, -0.2316524989510642119 ) ) ;
#35412=CARTESIAN_POINT ( 'NONE',  ( -18.36446446646858632, 154.1536317137893661, 0.4323159980074339215 ) ) ;
#35418=CARTESIAN_POINT ( 'NONE',  ( 2.988498945533646367, -15.63929389023541106, 5.494461050752756925 ) ) ;
#35419=CARTESIAN_POINT ( 'NONE',  ( -20.18403667007074986, 149.6821479856479300, 1.616815787834456231 ) ) ;
#35421=CARTESIAN_POINT ( 'NONE',  ( 6.877630800715452963, 117.9658002137636856, -0.6876290806823442958 ) ) ;
#35422=CARTESIAN_POINT ( 'NONE',  ( -4.274281473441157608, 3.541781053574249327, 1.790774723582081451 ) ) ;
#35426=CARTESIAN_POINT ( 'NONE',  ( -0.04081796247070307998, 114.7739974199301969, 2.042697753608746059 ) ) ;
#35427=( NAMED_UNIT ( * ) SI_UNIT ( $, .STERADIAN. ) SOLID_ANGLE_UNIT ( ) );
#35429=CARTESIAN_POINT ( 'NONE',  ( -17.27635908418611166, 147.1820577694790018, 1.364000445115660876 ) ) ;
#35431=CARTESIAN_POINT ( 'NONE',  ( 1.325863631979435686, 119.1766673560425858, -0.6173222594915835915 ) ) ;
#35433=CARTESIAN_POINT ( 'NONE',  ( -4.854614700615708323, 158.3981005702974016, -1.674235554132198489 ) ) ;
#35436=CARTESIAN_POINT ( 'NONE',  ( 4.558037855495248536, 118.1057855763819049, -0.4916461251602846638 ) ) ;
#35437=CARTESIAN_POINT ( 'NONE',  ( 0.6112472438485718751, 120.6441756478195089, -0.2446543754660636949 ) ) ;
#35439=CARTESIAN_POINT ( 'NONE',  ( 0.02874415600660452930, 157.0795416643300939, -1.438475106415293858 ) ) ;
#35440=CARTESIAN_POINT ( 'NONE',  ( 3.487342509456591522, -15.13654059619573644, 2.575171134517089566 ) ) ;
#35441=CARTESIAN_POINT ( 'NONE',  ( -4.105768389763392534, 118.2429491485453070, -0.3526141341681313102 ) ) ;
#35444=CARTESIAN_POINT ( 'NONE',  ( -4.920305038941537923, 117.6396262227241749, 0.8278391774136714121 ) ) ;
#35445=CARTESIAN_POINT ( 'NONE',  ( 17.41367791652938735, 147.5992144370567871, 2.159268082968858415 ) ) ;
#35448=EDGE_CURVE ( 'NONE', #39680, #31017, #25149, .T. ) ;
#35449=CARTESIAN_POINT ( 'NONE',  ( 7.253464168720983096, -10.72948646729439659, -4.330533999219945862 ) ) ;
#35450=CARTESIAN_POINT ( 'NONE',  ( 4.547323659248075245, 121.1438296405421937, 0.2486498796252668564 ) ) ;
#35454=CARTESIAN_POINT ( 'NONE',  ( -0.6048974376704769895, 117.3993834314756128, 1.469641059425755403 ) ) ;
#35458=CARTESIAN_POINT ( 'NONE',  ( -8.362805289807246467, 119.6845456798349829, -1.431079265360458486 ) ) ;
#35462=CARTESIAN_POINT ( 'NONE',  ( -0.003073183581813956986, 116.5806198863164838, 0.1537946732117061455 ) ) ;
#35465=CARTESIAN_POINT ( 'NONE',  ( 6.919917455521427563, 121.8373941398667313, -0.2187690460202940113 ) ) ;
#35467=CARTESIAN_POINT ( 'NONE',  ( 0.7849178055945060795, 115.7029491485453718, -1.726834944265495553 ) ) ;
#35468=CARTESIAN_POINT ( 'NONE',  ( -5.289698609640079319, 121.3432423864224177, -0.1753557357117458970 ) ) ;
#35469=CARTESIAN_POINT ( 'NONE',  ( 3.228727248129140026, -15.23899909574484646, 5.612614099740361517 ) ) ;
#35470=CARTESIAN_POINT ( 'NONE',  ( -21.16640241758172181, 149.7512365312068709, 1.384406599442889352 ) ) ;
#35471=LINE ( 'NONE', #32273, #2312 ) ;
#35472=CARTESIAN_POINT ( 'NONE',  ( 10.77008264951268046, 157.9328640892066460, 0.4716003899658740006 ) ) ;
#35473=CARTESIAN_POINT ( 'NONE',  ( 8.009213594383991719, 122.8488802212246611, 0.2424541544307477758 ) ) ;
#35475=CARTESIAN_POINT ( 'NONE',  ( 0.8487236205744517203, 17.35912690172634143, 0.4866769997786373203 ) ) ;
#35476=CARTESIAN_POINT ( 'NONE',  ( -15.17534484293440578, 156.1124880001465556, -0.4370721430752772529 ) ) ;
#35479=EDGE_LOOP ( 'NONE', ( #62, #17164, #13899, #37912, #29566, #32921, #28324, #5448 ) ) ;
#35480=CARTESIAN_POINT ( 'NONE',  ( 2.603427674266608260, 116.9065387239081701, 0.5777963497691434025 ) ) ;
#35481=ORIENTED_EDGE ( 'NONE', *, *, #30451, .F. ) ;
#35482=ADVANCED_FACE ( 'NONE', ( #32261 ), #22216, .T. ) ;
#35484=CARTESIAN_POINT ( 'NONE',  ( 1.224709079186512728, 159.1407128229522527, 1.247756218451904431 ) ) ;
#35485=CARTESIAN_POINT ( 'NONE',  ( 13.23674331388971304, 122.5785676075921060, -1.297564987558605498 ) ) ;
#35486=CARTESIAN_POINT ( 'NONE',  ( -1.555401355773622374, 10.72473834230686762, 8.302158768936594768 ) ) ;
#35487=CARTESIAN_POINT ( 'NONE',  ( -9.950292893259929272, 157.6892375622926181, -1.550998551202242393 ) ) ;
#35488=CARTESIAN_POINT ( 'NONE',  ( 4.633276512935547764, 117.9522311679255893, -0.7618818254156639602 ) ) ;
#35492=CARTESIAN_POINT ( 'NONE',  ( -11.06366964751665982, 128.0319838675845290, -0.1805508315534839758 ) ) ;
#35493=CARTESIAN_POINT ( 'NONE',  ( -19.16322371038640071, 147.9830121424878939, -2.503561316673066361 ) ) ;
#35494=CARTESIAN_POINT ( 'NONE',  ( 5.898825546834660649, -14.84738759216856785, 0.02597052417917125600 ) ) ;
#35501=CARTESIAN_POINT ( 'NONE',  ( 11.66906004923067641, 122.8035986606355152, 1.736571914056905142 ) ) ;
#35502=CARTESIAN_POINT ( 'NONE',  ( -15.70103477329412911, 145.5797129992483292, -0.3137440411564564879 ) ) ;
#35504=CARTESIAN_POINT ( 'NONE',  ( -6.631541954483209765E-14, 98.39146620154573952, -1.863789202389766375E-18 ) ) ;
#35505=CARTESIAN_POINT ( 'NONE',  ( -4.585195778441760517, 124.9344662015457459, -0.09162312381275070083 ) ) ;
#35506=CARTESIAN_POINT ( 'NONE',  ( 1.249529592346430240, 29.00528243095578063, -8.330927077797271707 ) ) ;
#35507=CARTESIAN_POINT ( 'NONE',  ( 9.600854460372817201, 124.0356975489027036, 0.7994020406953790125 ) ) ;
#35508=CARTESIAN_POINT ( 'NONE',  ( 14.24059674577810597, 120.4756499382577886, -0.4587616384891653465 ) ) ;
#35509=CARTESIAN_POINT ( 'NONE',  ( 5.274109024393328404, 115.7029491485453150, -0.8140283081321303404 ) ) ;
#35512=CARTESIAN_POINT ( 'NONE',  ( -2.736438259132304207, 116.5290148844309357, -0.04129949523434437580 ) ) ;
#35514=CARTESIAN_POINT ( 'NONE',  ( -6.482835885433019030, 120.3696088574302507, -1.155002112961008631 ) ) ;
#35515=CARTESIAN_POINT ( 'NONE',  ( 2.851877909000272382, -15.42561672255453331, 5.733748130541576060 ) ) ;
#35516=CARTESIAN_POINT ( 'NONE',  ( -10.72508252498929515, 126.1521286088116369, -0.7954780730053832016 ) ) ;
#35517=CARTESIAN_POINT ( 'NONE',  ( 3.658150719587269784, -13.97641594243527408, 4.344832359604154703 ) ) ;
#35519=CARTESIAN_POINT ( 'NONE',  ( 5.774842806153344554, 116.9337168780244696, 0.1296094601971085336 ) ) ;
#35521=CARTESIAN_POINT ( 'NONE',  ( -4.319812470756069445, 11.96289413176387129, -1.686699837767231536 ) ) ;
#35522=CARTESIAN_POINT ( 'NONE',  ( -15.97340373827834270, 121.0409387471171101, -0.3191866212789525314 ) ) ;
#35523=CARTESIAN_POINT ( 'NONE',  ( -4.829078608027735697, 117.4024328994306501, 1.010041111858091423 ) ) ;
#35527=CARTESIAN_POINT ( 'NONE',  ( -6.121275585599194713, 121.0364858238823729, 0.5305944776602569135 ) ) ;
#35528=VECTOR ( 'NONE', #28169, 1000.000000000000227 ) ;
#35529=CARTESIAN_POINT ( 'NONE',  ( 4.428293322310913993, 12.87204911218450398, 1.319288874004734158 ) ) ;
#35530=EDGE_CURVE ( 'NONE', #12906, #1598, #3296, .T. ) ;
#35531=CARTESIAN_POINT ( 'NONE',  ( 16.28621419528960601, 155.1963085991477271, 1.407434501154738671 ) ) ;
#35532=CARTESIAN_POINT ( 'NONE',  ( -0.1058213901579529159, 105.9761915687834914, 5.295735085524055030 ) ) ;
#35534=CARTESIAN_POINT ( 'NONE',  ( 4.057542840006381546, 118.1249481555716301, -0.7600096289331683685 ) ) ;
#35535=CARTESIAN_POINT ( 'NONE',  ( 4.453423564604278795, 13.74662854910535792, -1.294644163995742225 ) ) ;
#35536=CARTESIAN_POINT ( 'NONE',  ( -20.83375562662827107, 132.2939277659177151, -1.304325680028331602 ) ) ;
#35538=CARTESIAN_POINT ( 'NONE',  ( -10.55375732331629557, 153.0603347025997323, 0.3251829154788382636 ) ) ;
#35539=EDGE_CURVE ( 'NONE', #40413, #1790, #37904, .T. ) ;
#35540=CARTESIAN_POINT ( 'NONE',  ( 4.290763117780162617, -14.65756668531598095, 4.875966813445055337 ) ) ;
#35541=FACE_OUTER_BOUND ( 'NONE', #37601, .T. ) ;
#35542=CIRCLE ( 'NONE', #19863, 0.5080000000000002292 ) ;
#35544=CARTESIAN_POINT ( 'NONE',  ( -4.521871022792333328, 118.0719105266109636, -0.8080184913735506402 ) ) ;
#35545=CARTESIAN_POINT ( 'NONE',  ( 15.78598348091615122, 146.2390805666957192, 0.2639793761055732602 ) ) ;
#35546=ORIENTED_EDGE ( 'NONE', *, *, #24127, .T. ) ;
#35547=CARTESIAN_POINT ( 'NONE',  ( 20.07331991451302500, 148.0303212619860744, 2.505472171123445779 ) ) ;
#35550=CARTESIAN_POINT ( 'NONE',  ( -16.32943869337488962, 155.1963085991477271, 0.7556961354993018132 ) ) ;
#35551=CARTESIAN_POINT ( 'NONE',  ( 0.008148072696521003327, 156.3406798448389168, -0.4077628766201953359 ) ) ;
#35552=CIRCLE ( 'NONE', #22598, 0.5080000000000002292 ) ;
#35553=CARTESIAN_POINT ( 'NONE',  ( 15.95511372484715729, 121.3860667298135070, -0.1093881341078833114 ) ) ;
#35555=CARTESIAN_POINT ( 'NONE',  ( -4.883848590450072358, 117.7607009110569862, 0.7127853619805604168 ) ) ;
#35557=CARTESIAN_POINT ( 'NONE',  ( -4.973714125165286326, 117.3984623533981022, -0.9750903916985453890 ) ) ;
#35560=CARTESIAN_POINT ( 'NONE',  ( 2.676630639921374399, -14.70069741876437242, -0.3491543817257181659 ) ) ;
#35561=CARTESIAN_POINT ( 'NONE',  ( -4.550470251402174426, 118.0718861047856336, 0.6267538730547278503 ) ) ;
#35564=CARTESIAN_POINT ( 'NONE',  ( -0.1669248393526201191, 115.6909491485452435, -1.766429783486955341 ) ) ;
#35565=CARTESIAN_POINT ( 'NONE',  ( 3.588165399132631883, 118.7223001924098895, -0.7939635985234113624 ) ) ;
#35566=CARTESIAN_POINT ( 'NONE',  ( 0.1065646865915095692, 105.8844662015456919, -5.332932678536313809 ) ) ;
#35567=CARTESIAN_POINT ( 'NONE',  ( 4.698333873473698574, 117.8441154341451238, 1.023705869601185814 ) ) ;
#35568=CARTESIAN_POINT ( 'NONE',  ( 2.829627719599027369, -13.65247383265987757, 0.5238048331051645690 ) ) ;
#35569=CARTESIAN_POINT ( 'NONE',  ( -7.827001302695666851, 121.9903164032602518, -0.9115841697347603079 ) ) ;
#35571=CARTESIAN_POINT ( 'NONE',  ( -1.900728597266289288, 115.7024225971088214, -1.719626108874834580 ) ) ;
#35572=CARTESIAN_POINT ( 'NONE',  ( -1.769971949791458332, 106.5487674150453046, 4.971549122525432907 ) ) ;
#35573=CARTESIAN_POINT ( 'NONE',  ( -4.664314973664742681, 117.9253040426969790, -0.9621209789661747669 ) ) ;
#35574=CARTESIAN_POINT ( 'NONE',  ( 4.828659834973804799, 112.7831754354443348, -2.372633244901563021 ) ) ;
#35575=CARTESIAN_POINT ( 'NONE',  ( -10.50156301541560211, 123.3532649940754027, -1.413946074136436470 ) ) ;
#35580=CARTESIAN_POINT ( 'NONE',  ( -4.595132424582489605, -6.828429371805166959, -0.5093739664528403877 ) ) ;
#35581=CARTESIAN_POINT ( 'NONE',  ( 6.899218498548927769, 117.3903047926647787, 0.5887349169472964050 ) ) ;
#35582=ORIENTED_EDGE ( 'NONE', *, *, #27318, .F. ) ;
#35584=CARTESIAN_POINT ( 'NONE',  ( 2.617865251411226613, -15.35234423845867369, 4.678879665404411803 ) ) ;
#35585=CARTESIAN_POINT ( 'NONE',  ( -18.75354316333454818, 144.8948545501563103, 1.742436930347202262 ) ) ;
#35586=CARTESIAN_POINT ( 'NONE',  ( 0.5056692551311988693, 10.92592451650425112, 0.8332994872028685052 ) ) ;
#35587=CIRCLE ( 'NONE', #13800, 0.5079999999999997851 ) ;
#35588=CARTESIAN_POINT ( 'NONE',  ( -0.6378939814135665687, 2.446253604616882349, -0.7403349100440516084 ) ) ;
#35592=CARTESIAN_POINT ( 'NONE',  ( 0.05023876518783839534, 106.0087397856094356, 5.285590276201098447 ) ) ;
#35593=CARTESIAN_POINT ( 'NONE',  ( -16.45208226155739695, 147.1833543704171348, 0.9460114105336800971 ) ) ;
#35594=CARTESIAN_POINT ( 'NONE',  ( 4.270589230953349968, -11.85684205577233818, 0.9542379244983925091 ) ) ;
#35595=CARTESIAN_POINT ( 'NONE',  ( 16.80660261901782704, 149.5530097695598215, -1.582604632240843578 ) ) ;
#35596=CARTESIAN_POINT ( 'NONE',  ( -3.228607480374549255, 118.8118204130220903, -0.9063605472083390291 ) ) ;
#35599=CARTESIAN_POINT ( 'NONE',  ( 8.255953115981643720, 120.2039708552018880, 1.447841472369825189 ) ) ;
#35600=CARTESIAN_POINT ( 'NONE',  ( -6.009810541787921068, 31.01725040276547674, -0.2975034299463961696 ) ) ;
#35601=CARTESIAN_POINT ( 'NONE',  ( 9.238523569213899833, 124.0999252189730697, -0.04720364951821272304 ) ) ;
#35603=FACE_OUTER_BOUND ( 'NONE', #27916, .T. ) ;
#35605=FACE_OUTER_BOUND ( 'NONE', #29061, .T. ) ;
#35607=CARTESIAN_POINT ( 'NONE',  ( 2.639528505629576305, 120.4390018212493914, 0.4929570044210890845 ) ) ;
#35608=DIRECTION ( 'NONE',  ( -4.017660918040594346E-17, 1.000000000000000000, 2.376309959284834438E-19 ) ) ;
#35609=CARTESIAN_POINT ( 'NONE',  ( 10.81400209053368755, 157.9177219752764358, 0.09677702710655973484 ) ) ;
#35610=B_SPLINE_CURVE_WITH_KNOTS ( 'NONE', 3,
 ( #21586, #31192, #27791, #14579, #3826, #23374, #29996, #10609, #14788, #7224, #13810, #40800, #27999, #27584, #4035, #16996, #4247, #17209 ),
 .UNSPECIFIED., .F., .F.,
 ( 4, 2, 2, 2, 2, 2, 2, 2, 4 ),
 ( 0.000000000000000000, 0.0008271074710775116285, 0.001654214942155023257, 0.003308429884310066463, 0.004135537355387588175, 0.004962644826465109453, 0.006616859768620188438, 0.009925289652930347276, 0.01323371953724050698 ),
 .UNSPECIFIED. ) ;
#35611=CARTESIAN_POINT ( 'NONE',  ( -0.1065646865916160396, 105.8844662015456777, 5.332932678536313809 ) ) ;
#35613=CYLINDRICAL_SURFACE ( 'NONE', #34301, 5.588000000000006295 ) ;
#35615=CARTESIAN_POINT ( 'NONE',  ( -2.045891073389006554, 34.07700515036425770, 0.6666589014435788663 ) ) ;
#35616=CARTESIAN_POINT ( 'NONE',  ( 2.160664645061408873, 117.9909145081919917, 0.7315704174731482157 ) ) ;
#35617=CARTESIAN_POINT ( 'NONE',  ( -3.990024091077861268, 18.91925256873344807, 2.329872802929966902 ) ) ;
#35618=CARTESIAN_POINT ( 'NONE',  ( -2.878135459294852705, -8.718908198948343014, 7.912908975683875745 ) ) ;
#35619=CARTESIAN_POINT ( 'NONE',  ( -5.482592266946507031, 117.2336767834907363, -0.8194921820605090002 ) ) ;
#35620=CARTESIAN_POINT ( 'NONE',  ( -1.907654281882167568, 121.7602717223048501, -0.3165470008995034945 ) ) ;
#35621=CARTESIAN_POINT ( 'NONE',  ( -22.83540780336928577, 150.4058779721138421, -0.4563057931615319140 ) ) ;
#35622=CARTESIAN_POINT ( 'NONE',  ( 0.7529411215435434235, 106.0533076082122790, -5.240246454641519946 ) ) ;
#35623=CARTESIAN_POINT ( 'NONE',  ( 0.09871621327668905765, 104.6144662015456959, 4.835249534459434173 ) ) ;
#35624=CARTESIAN_POINT ( 'NONE',  ( -4.492784857928645792, 12.16275517495587977, -1.104450737933446725 ) ) ;
#35625=CARTESIAN_POINT ( 'NONE',  ( -6.019568728095220427E-14, 78.83346620154574680, 1.000738015618740492E-16 ) ) ;
#35626=CARTESIAN_POINT ( 'NONE',  ( -15.73471677570942262, 120.8416612192442159, -0.3144170877234248596 ) ) ;
#35627=CARTESIAN_POINT ( 'NONE',  ( 3.205191379615736746, -14.47393913169138102, 3.051678166811226500 ) ) ;
#35628=CARTESIAN_POINT ( 'NONE',  ( 2.908797093394981381, 122.3314979878274045, -0.1372540494999658078 ) ) ;
#35629=CARTESIAN_POINT ( 'NONE',  ( -15.62635203013939034, 121.2802728028965475, 0.2997488694636322171 ) ) ;
#35634=AXIS2_PLACEMENT_3D ( 'NONE', #30373, #36375, #23338 ) ;
#35635=CARTESIAN_POINT ( 'NONE',  ( 4.376329468599289285, -15.53264713215277126, 4.356271056886698467 ) ) ;
#35636=CARTESIAN_POINT ( 'NONE',  ( -4.101170551582197454, 118.4217611105734846, 0.8082045602434786424 ) ) ;
#35637=CARTESIAN_POINT ( 'NONE',  ( 22.13784291382268066, 148.5290936231802448, -1.147597636374165342 ) ) ;
#35638=CARTESIAN_POINT ( 'NONE',  ( 2.522041008973656240, -3.380034811851383214, 3.874746376371965617 ) ) ;
#35643=FILL_AREA_STYLE_COLOUR ( '', #32483 ) ;
#35644=CARTESIAN_POINT ( 'NONE',  ( -16.48900842742864015, 139.9843038322558186, 1.489460148179643895 ) ) ;
#35645=CARTESIAN_POINT ( 'NONE',  ( 5.124055468070814356, 116.9398885036888487, 0.3846614261691105874 ) ) ;
#35647=CARTESIAN_POINT ( 'NONE',  ( 16.12483552447390167, 131.4332636412663931, -1.626400019052950396 ) ) ;
#35648=CARTESIAN_POINT ( 'NONE',  ( -20.63667788919588730, 149.2407879669073054, -2.389545083207230913 ) ) ;
#35650=AXIS2_PLACEMENT_3D ( 'NONE', #10659, #14474, #40289 ) ;
#35651=VERTEX_POINT ( 'NONE', #13917 ) ;
#35652=CARTESIAN_POINT ( 'NONE',  ( 4.482242274157552053, 118.1125264040518061, -0.5758228734123297388 ) ) ;
#35653=CARTESIAN_POINT ( 'NONE',  ( 9.482824821899882295, 153.9068681542131856, -0.6648444853843684665 ) ) ;
#35655=CARTESIAN_POINT ( 'NONE',  ( 0.009931517865179408100, 119.6374844068871397, -0.4970137656763582990 ) ) ;
#35656=CARTESIAN_POINT ( 'NONE',  ( 3.340243159461592448, -15.49156354636899202, 3.813188716183662397 ) ) ;
#35659=CARTESIAN_POINT ( 'NONE',  ( 4.615704859843055452, 105.1215186159430885, -2.696439918938831948 ) ) ;
#35661=CARTESIAN_POINT ( 'NONE',  ( -4.933822780877020087, 117.6566500539053379, 0.7550610955488965548 ) ) ;
#35662=CARTESIAN_POINT ( 'NONE',  ( 11.01900745353688293, 123.5714170083676748, 1.527874194239944305 ) ) ;
#35665=CARTESIAN_POINT ( 'NONE',  ( 4.377640660406503237, 26.40621510375495973, 1.544744264128281364 ) ) ;
#35666=CARTESIAN_POINT ( 'NONE',  ( 11.96249418807702547, 130.4318746828361100, 0.4433914376541254199 ) ) ;
#35669=VERTEX_POINT ( 'NONE', #20716 ) ;
#35673=CARTESIAN_POINT ( 'NONE',  ( -8.798071503382049130, 117.6842349159514640, -0.1758064068840608507 ) ) ;
#35678=CARTESIAN_POINT ( 'NONE',  ( -13.52003375314306055, 119.6474162840860771, 0.03304800104807582156 ) ) ;
#35681=CARTESIAN_POINT ( 'NONE',  ( -6.945483162495717622, 121.9345112681876060, -0.2969950648847965446 ) ) ;
#35682=VERTEX_POINT ( 'NONE', #1363 ) ;
#35683=CARTESIAN_POINT ( 'NONE',  ( 3.248299790614018967, 115.7029686237793271, -1.528078099553393798 ) ) ;
#35684=CARTESIAN_POINT ( 'NONE',  ( -15.74517894787283012, 145.7063497038720925, -0.5455200375299574800 ) ) ;
#35685=CARTESIAN_POINT ( 'NONE',  ( 4.290763117780162617, -14.65756668531598095, 4.875966813445055337 ) ) ;
#35686=CARTESIAN_POINT ( 'NONE',  ( -6.834340443517129771, 118.4250403807481575, 0.8562881416378698152 ) ) ;
#35688=CARTESIAN_POINT ( 'NONE',  ( 15.55067499035023815, 120.8127473925414108, 0.5415919938617849150 ) ) ;
#35689=CARTESIAN_POINT ( 'NONE',  ( -0.001311298634349677191, 120.9974662015458193, 0.06562274578655612201 ) ) ;
#35690=CARTESIAN_POINT ( 'NONE',  ( 4.831562716854217676, 118.5266822147775940, -0.7494263288004241463 ) ) ;
#35691=CARTESIAN_POINT ( 'NONE',  ( -0.6941440390767986690, 12.16465383894776409, -0.6855803344193639459 ) ) ;
#35692=CARTESIAN_POINT ( 'NONE',  ( -14.79880180360901498, 120.3086691715681695, -0.4511713404943135108 ) ) ;
#35696=CARTESIAN_POINT ( 'NONE',  ( -8.703195117136894865, 118.2213682157332499, 0.5883247612393129877 ) ) ;
#35697=EDGE_LOOP ( 'NONE', ( #32013, #23072, #41844, #21551, #6151 ) ) ;
#35699=CARTESIAN_POINT ( 'NONE',  ( 20.80232463633019080, 150.1670661137953289, 2.219268881695795059 ) ) ;
#35700=CARTESIAN_POINT ( 'NONE',  ( 0.01147819631899514407, 118.5605975114896609, -0.5744158801423953076 ) ) ;
#35701=CARTESIAN_POINT ( 'NONE',  ( 0.1324238259082184954, -4.506001423838159603, -0.9708255322318050107 ) ) ;
#35702=CARTESIAN_POINT ( 'NONE',  ( 0.7792876995799051798, 11.14506788600763443, 8.385000233822015758 ) ) ;
#35703=CARTESIAN_POINT ( 'NONE',  ( -10.85289063249360275, 119.5270080912504653, -1.298249717235596679 ) ) ;
#35704=CARTESIAN_POINT ( 'NONE',  ( 4.680411924161218096, 117.9630966871662707, -0.7259034715361608603 ) ) ;
#35706=CARTESIAN_POINT ( 'NONE',  ( 2.498958912387863940, 107.2142675576569530, 4.733253560342793875 ) ) ;
#35707=EDGE_CURVE ( 'NONE', #6038, #21896, #27684, .T. ) ;
#35708=CARTESIAN_POINT ( 'NONE',  ( -3.758730197597831779, 121.0943292417197199, -0.07510837462871998438 ) ) ;
#35710=CARTESIAN_POINT ( 'NONE',  ( -11.66906004923080609, 122.8035986606355152, -1.736571914056904919 ) ) ;
#35711=CARTESIAN_POINT ( 'NONE',  ( 6.120062074970366695, -14.59381343598747982, -0.2446369611249375742 ) ) ;
#35713=B_SPLINE_CURVE_WITH_KNOTS ( 'NONE', 3,
 ( #5943, #28502, #9332, #2950, #39147, #28914, #18902, #9951, #12524, #31699, #29123, #9534, #25927, #6555, #38726, #15502, #31912, #41929, #22089, #12316 ),
 .UNSPECIFIED., .F., .F.,
 ( 4, 2, 2, 2, 2, 2, 2, 2, 2, 4 ),
 ( -5.999999999773951516E-08, 0.0007881763970578359617, 0.001576412794115669615, 0.002364649191173503161, 0.003152885588231336706, 0.003941121985289170251, 0.004729358382347004230, 0.006305831176462709485, 0.009458776764694155556, 0.01261172235292560423 ),
 .UNSPECIFIED. ) ;
#35715=EDGE_LOOP ( 'NONE', ( #36396, #209, #3554, #5668 ) ) ;
#35716=CARTESIAN_POINT ( 'NONE',  ( 18.24092514812179289, 147.9371514012413229, 2.391122828403475342 ) ) ;
#35717=CARTESIAN_POINT ( 'NONE',  ( 2.656309428775586845, -12.29155461912079339, 0.4553234995023021647 ) ) ;
#35719=CARTESIAN_POINT ( 'NONE',  ( -4.141015252736775842, 122.5143120247930142, 0.07252455213604060147 ) ) ;
#35720=CARTESIAN_POINT ( 'NONE',  ( 8.390987441844862005, -15.30508105673078667, -0.4368898320763015541 ) ) ;
#35721=CARTESIAN_POINT ( 'NONE',  ( 9.322631400391582446, 123.9819092696984910, 0.6064563484049506625 ) ) ;
#35722=CARTESIAN_POINT ( 'NONE',  ( 5.526300601521314526, 159.0395019988757781, -0.6540312330581287137 ) ) ;
#35724=CARTESIAN_POINT ( 'NONE',  ( 4.581721556995678846, -15.30239758790170157, -0.5121114949450596976 ) ) ;
#35726=CARTESIAN_POINT ( 'NONE',  ( -20.50175740331293284, 129.0975500345852822, -0.3894088793431773610 ) ) ;
#35728=CARTESIAN_POINT ( 'NONE',  ( 8.182757305131426406, 120.8045583724933039, -1.052530632093990670 ) ) ;
#35729=CARTESIAN_POINT ( 'NONE',  ( 2.293129817604454335, -15.49007597679844395, 5.904469655623132418 ) ) ;
#35730=CARTESIAN_POINT ( 'NONE',  ( -9.269771126213486312, 123.9149913687586064, -0.6034020272129926310 ) ) ;
#35731=CARTESIAN_POINT ( 'NONE',  ( 3.564576864782785570, -14.06793500455072454, 4.479818044377421593 ) ) ;
#35732=CARTESIAN_POINT ( 'NONE',  ( -5.091661282192257332, 117.1433449680017276, 0.3971322054743541274 ) ) ;
#35733=CARTESIAN_POINT ( 'NONE',  ( -6.439805278602227377E-14, 159.6054662015457382, 1.008550168686281963E-16 ) ) ;
#35734=VERTEX_POINT ( 'NONE', #26706 ) ;
#35735=CARTESIAN_POINT ( 'NONE',  ( 2.829288187452689396, 6.340478445469713620, 3.655570690059357197 ) ) ;
#35736=CARTESIAN_POINT ( 'NONE',  ( -0.4952506866058259405, 105.1225159476502711, 5.321743445971568676 ) ) ;
#35737=CARTESIAN_POINT ( 'NONE',  ( -4.828903201324592942, 117.4062739125616162, 1.009435533365967697 ) ) ;
#35738=CARTESIAN_POINT ( 'NONE',  ( 3.332917225768783798, 108.2589911827716520, 4.156415063234818241 ) ) ;
#35739=CARTESIAN_POINT ( 'NONE',  ( -7.010790661031958138, 121.7392789538311462, 0.3431444702839729910 ) ) ;
#35740=CARTESIAN_POINT ( 'NONE',  ( -0.5832499861179958334, 10.72304255322087307, 4.598074068532726599 ) ) ;
#35741=CARTESIAN_POINT ( 'NONE',  ( 22.31420326625516637, 142.2114994846844240, 1.760598597564681622 ) ) ;
#35742=CARTESIAN_POINT ( 'NONE',  ( 15.72385166996613570, 146.8976323831864477, 0.3141999770531622160 ) ) ;
#35744=CARTESIAN_POINT ( 'NONE',  ( 1.147165779964274046, 117.8708904510121016, -0.5694250185432008227 ) ) ;
#35745=CARTESIAN_POINT ( 'NONE',  ( -3.586339569854333664, 7.474549112184490696, -2.913498476264247294 ) ) ;
#35746=CARTESIAN_POINT ( 'NONE',  ( -9.554367121731717205, 118.3624989119526418, -0.8896461348445368067 ) ) ;
#35749=CARTESIAN_POINT ( 'NONE',  ( -5.910930898603252714, 121.4708175001875077, 0.1161132702817544021 ) ) ;
#35750=CARTESIAN_POINT ( 'NONE',  ( 6.030629465787032295, -12.69248357272054228, 1.053518048143269548 ) ) ;
#35751=DIRECTION ( 'NONE',  ( 0.9998004120163608288, 0.000000000000000000, 0.01997839162482736852 ) ) ;
#35752=EDGE_CURVE ( 'NONE', #27898, #34334, #29047, .T. ) ;
#35755=CARTESIAN_POINT ( 'NONE',  ( 19.45004534592201040, 148.0998626603252148, 2.515250464377977391 ) ) ;
#35758=CARTESIAN_POINT ( 'NONE',  ( -22.75813664408071446, 148.5871737753741115, 0.7284712318767733175 ) ) ;
#35759=CARTESIAN_POINT ( 'NONE',  ( 0.004910662370358530836, 159.5928157220454295, -0.2457496255665020946 ) ) ;
#35764=CARTESIAN_POINT ( 'NONE',  ( -4.812557187411091064, 117.4080492109849416, -1.196763905027394159 ) ) ;
#35767=CARTESIAN_POINT ( 'NONE',  ( -4.678425872278161535, 118.0125782974996582, 0.6042734876502935393 ) ) ;
#35770=ORIENTED_EDGE ( 'NONE', *, *, #24850, .F. ) ;
#35772=CARTESIAN_POINT ( 'NONE',  ( -3.195518864091055455, 115.6909491485452719, -1.660603084447102917 ) ) ;
#35774=CARTESIAN_POINT ( 'NONE',  ( 3.370951604764516496, 118.5093630253226280, -0.7873060099658909516 ) ) ;
#35775=CARTESIAN_POINT ( 'NONE',  ( -5.210481185491613765, 116.4925209815607730, -1.089480302653437871 ) ) ;
#35776=CARTESIAN_POINT ( 'NONE',  ( 4.611851918533471206, 117.9566237460099103, 0.9391389632551998545 ) ) ;
#35777=CARTESIAN_POINT ( 'NONE',  ( 2.460727335429193197, -15.06314154744310585, 4.845259171755021299 ) ) ;
#35778=CARTESIAN_POINT ( 'NONE',  ( -9.075659781538043092, 123.1184971541203055, -0.9241268708344094751 ) ) ;
#35781=CARTESIAN_POINT ( 'NONE',  ( -4.129065684684445792, 110.9559963654141228, 3.095242660527065759 ) ) ;
#35783=CARTESIAN_POINT ( 'NONE',  ( 7.450817465826167663, 123.6645382909113664, 0.1143006167400528322 ) ) ;
#35784=CARTESIAN_POINT ( 'NONE',  ( -15.02674521555436371, 134.7883251604851580, -1.951091898071898978 ) ) ;
#35786=CARTESIAN_POINT ( 'NONE',  ( -0.006534887713674904404, 159.5822087645323393, 0.3270325034788581497 ) ) ;
#35788=CARTESIAN_POINT ( 'NONE',  ( -2.277020932126007757, 115.7026820661928497, 1.618586367388850533 ) ) ;
#35789=CARTESIAN_POINT ( 'NONE',  ( -0.001311586712342687876, 120.9974662015458193, 0.06563716238878879172 ) ) ;
#35790=CARTESIAN_POINT ( 'NONE',  ( -3.426874451426485724, 1.805113900313119357, -3.130497002818263930 ) ) ;
#35791=CARTESIAN_POINT ( 'NONE',  ( 4.801439827634202295, 117.0090399748681875, 0.4924919612534520152 ) ) ;
#35793=CARTESIAN_POINT ( 'NONE',  ( 5.284192421469999346, 104.6144662015304050, -0.8069602218790292714 ) ) ;
#35794=CARTESIAN_POINT ( 'NONE',  ( 3.866904830252686054, -15.34763638737450542, 1.784481441967298743 ) ) ;
#35795=CARTESIAN_POINT ( 'NONE',  ( -0.01133701094407592140, 119.0130636887059410, 0.5673503866435173348 ) ) ;
#35796=CARTESIAN_POINT ( 'NONE',  ( 0.9260135661551653907, 3.379156789086214197, -0.3022368940483516897 ) ) ;
#35797=CARTESIAN_POINT ( 'NONE',  ( -0.9473015597126430709, 116.7004868406603322, -0.2634242240387510980 ) ) ;
#35798=CARTESIAN_POINT ( 'NONE',  ( -0.1566604602083998543, 5.914057227930348049, 0.9647682902456425902 ) ) ;
#35799=VERTEX_POINT ( 'NONE', #21334 ) ;
#35802=EDGE_CURVE ( 'NONE', #36618, #20434, #10878, .T. ) ;
#35803=CARTESIAN_POINT ( 'NONE',  ( 4.774443427420539621, 116.8297769931967309, 1.047991251433075366 ) ) ;
#35804=CARTESIAN_POINT ( 'NONE',  ( -15.77383231466701297, 147.9505201145231865, 0.6473862450635484711 ) ) ;
#35805=CARTESIAN_POINT ( 'NONE',  ( 2.629318991877339418, -14.82094413389492615, 5.549789958447211013 ) ) ;
#35806=CARTESIAN_POINT ( 'NONE',  ( 7.333780486663145304, 155.8804291298944236, -1.515250586328038773 ) ) ;
#35807=CARTESIAN_POINT ( 'NONE',  ( -19.78444808418236178, 147.9128418260961837, -2.517891032746078839 ) ) ;
#35809=CARTESIAN_POINT ( 'NONE',  ( 2.931439949929583122, -14.82325452411255640, 4.117531814738872420 ) ) ;
#35810=CARTESIAN_POINT ( 'NONE',  ( -5.164545546852735036, 32.23602039546388909, 1.233576701498339201 ) ) ;
#35811=CARTESIAN_POINT ( 'NONE',  ( 1.609565093910530154, 156.2658572007470639, -0.2453390865415086830 ) ) ;
#35812=ORIENTED_EDGE ( 'NONE', *, *, #10812, .T. ) ;
#35813=CARTESIAN_POINT ( 'NONE',  ( -0.01009854879487165520, 117.2429491485453070, 0.5053730761602109878 ) ) ;
#35816=EDGE_CURVE ( 'NONE', #18326, #41007, #40858, .T. ) ;
#35821=CARTESIAN_POINT ( 'NONE',  ( 21.60220573293482715, 132.6646020023713959, 0.2978857061057722522 ) ) ;
#35823=CARTESIAN_POINT ( 'NONE',  ( -7.694720906311372843, 124.7202454748262710, -0.1538800020430350635 ) ) ;
#35825=CARTESIAN_POINT ( 'NONE',  ( -2.646443841375008432, -8.127818987380491578, -3.789199236247322133 ) ) ;
#35826=CARTESIAN_POINT ( 'NONE',  ( -4.834802360910630981, 32.27718159487177729, 0.9856153350916389000 ) ) ;
#35827=CARTESIAN_POINT ( 'NONE',  ( 4.930931983215351977, 118.2512723699127832, 1.012396356527061725 ) ) ;
#35828=CARTESIAN_POINT ( 'NONE',  ( -3.618988008572157522, 19.14412854911201123, 2.900346660497036044 ) ) ;
#35829=CARTESIAN_POINT ( 'NONE',  ( 1.420544585151703343, -13.23898594424576203, -8.332176651214544094 ) ) ;
#35830=CARTESIAN_POINT ( 'NONE',  ( 8.756088789680248397, 117.9414872320107435, -0.3631643394575467809 ) ) ;
#35831=CARTESIAN_POINT ( 'NONE',  ( -1.302594956492468370, 113.6455945353133643, -2.391525302099168027 ) ) ;
#35832=CARTESIAN_POINT ( 'NONE',  ( -23.36555825341177339, 148.7788340588663800, -0.4668994608413308267 ) ) ;
#35833=CARTESIAN_POINT ( 'NONE',  ( 4.129667044122415476, 110.9560305189546767, -3.095181893054258282 ) ) ;
#35834=CARTESIAN_POINT ( 'NONE',  ( -2.260567382777518119, 105.1242543621358436, 4.832464655412169741 ) ) ;
#35835=CARTESIAN_POINT ( 'NONE',  ( -0.8080508600641240768, 24.25718022715097888, 4.550674767031389401 ) ) ;
#35838=CARTESIAN_POINT ( 'NONE',  ( -21.68875320759065062, 132.7412702629105468, -0.4333929054516006962 ) ) ;
#35839=CARTESIAN_POINT ( 'NONE',  ( 2.770737963896511946, -14.84290363635286347, 4.452025088638788652 ) ) ;
#35840=CARTESIAN_POINT ( 'NONE',  ( 2.292460607442518672, 118.3648483361698851, -0.7949187631362102380 ) ) ;
#35841=CARTESIAN_POINT ( 'NONE',  ( -15.03447867299186669, 120.7699597703182945, 0.2997422626971647519 ) ) ;
#35848=CARTESIAN_POINT ( 'NONE',  ( 4.231574481101612051, -15.55479495760878095, 4.522910428756792278 ) ) ;
#35849=CARTESIAN_POINT ( 'NONE',  ( -19.16692462419661425, 150.4642993720107143, 1.670612363451736249 ) ) ;
#35850=CARTESIAN_POINT ( 'NONE',  ( 16.54768821719722993, 125.2933801378020888, -1.124873388181685030 ) ) ;
#35851=CARTESIAN_POINT ( 'NONE',  ( 1.398650104629075797, 0.06838872207683838189, -4.420329592304430122 ) ) ;
#35856=CARTESIAN_POINT ( 'NONE',  ( 0.3796903751652699888, 122.8649044353670803, 0.2268226101886974821 ) ) ;
#35857=CARTESIAN_POINT ( 'NONE',  ( -4.678029067978729749, 117.8847919582286465, 0.8180832583663835145 ) ) ;
#35858=CARTESIAN_POINT ( 'NONE',  ( -2.030192889891393460, 156.8313070664539168, 1.335154060002984311 ) ) ;
#35860=CARTESIAN_POINT ( 'NONE',  ( 15.17663987144297266, 128.5586215118215705, -1.546218023206676229 ) ) ;
#35861=CARTESIAN_POINT ( 'NONE',  ( -18.42009423903802556, 151.8926627062091086, -2.314360763190140169 ) ) ;
#35863=ORIENTED_EDGE ( 'NONE', *, *, #20652, .F. ) ;
#35864=CARTESIAN_POINT ( 'NONE',  ( 4.580295709240714608, 118.0857834188402791, -0.5549505832812218209 ) ) ;
#35865=CARTESIAN_POINT ( 'NONE',  ( 16.03056103447425684, 147.0154580547469152, -0.5309802628845385897 ) ) ;
#35867=CARTESIAN_POINT ( 'NONE',  ( -13.61432229890765733, 152.4534842159446271, -2.088615715084950253 ) ) ;
#35868=CARTESIAN_POINT ( 'NONE',  ( 3.614876661864775187, -15.45153451277975165, 3.150551394879585132 ) ) ;
#35869=CARTESIAN_POINT ( 'NONE',  ( 0.5023112062301228198, 105.1225718423296343, -5.320799118487369306 ) ) ;
#35870=TOROIDAL_SURFACE ( 'NONE', #29720, 3.683000000000000718, 0.5080000000000000071 ) ;
#35873=CARTESIAN_POINT ( 'NONE',  ( -4.896827542163006974, 117.7233055579753938, 0.7633307427583084781 ) ) ;
#35874=CARTESIAN_POINT ( 'NONE',  ( 10.91091678335008552, 123.4376579628654014, 1.516229561143084714 ) ) ;
#35877=CARTESIAN_POINT ( 'NONE',  ( -0.9950013725589796909, 29.65466048987409309, -4.513790593961638287 ) ) ;
#35878=CARTESIAN_POINT ( 'NONE',  ( 2.908234975202448780, 156.0868537499222839, 0.2102064236019249022 ) ) ;
#35879=DIRECTION ( 'NONE',  ( -0.01997839162482761832, -1.040247600000950455E-18, 0.9998004120163610509 ) ) ;
#35882=CARTESIAN_POINT ( 'NONE',  ( -2.183929936140839523, 116.1876165027943273, -0.08882796894186900660 ) ) ;
#35883=CARTESIAN_POINT ( 'NONE',  ( -5.078986093043186045, 78.83346620154574680, -0.1014902294541237815 ) ) ;
#35886=DIRECTION ( 'NONE',  ( -0.01997839162482761832, -1.040247600000950455E-18, 0.9998004120163610509 ) ) ;
#35888=CARTESIAN_POINT ( 'NONE',  ( -4.074955089416341991, 118.2429491485453354, 0.1454234154749719787 ) ) ;
#35889=DIRECTION ( 'NONE',  ( -4.017660918040594346E-17, 1.000000000000000000, 2.376309959284834438E-19 ) ) ;
#35892=CARTESIAN_POINT ( 'NONE',  ( -21.48671512862192756, 132.5742979909900328, -0.1330572995313747120 ) ) ;
#35893=ORIENTED_EDGE ( 'NONE', *, *, #19283, .T. ) ;
#35895=CARTESIAN_POINT ( 'NONE',  ( -6.964740248879998319, 121.9459328161491385, -0.2343094465020360562 ) ) ;
#35897=CYLINDRICAL_SURFACE ( 'NONE', #28748, 0.5080000000000002292 ) ;
#35898=CARTESIAN_POINT ( 'NONE',  ( -9.115475939616176859, 153.9201329141909866, -0.2944159349489392508 ) ) ;
#35899=CARTESIAN_POINT ( 'NONE',  ( 4.815776949948430641, -14.65450223259012752, 4.385166865640996114 ) ) ;
#35900=CARTESIAN_POINT ( 'NONE',  ( -21.17963693554089488, 147.9292434580435724, 1.516351520135284847 ) ) ;
#35901=DIRECTION ( 'NONE',  ( -5.206863593109713661E-17, 1.000000000000000000, -1.077750396879097183E-30 ) ) ;
#35902=CARTESIAN_POINT ( 'NONE',  ( 6.905604733424301145, 117.2797055272990292, 0.4577529590079177368 ) ) ;
#35904=CARTESIAN_POINT ( 'NONE',  ( 12.79726118125660150, 133.7150753560844976, 0.3789659047097265199 ) ) ;
#35906=CARTESIAN_POINT ( 'NONE',  ( -0.2932310942476468174, 5.691741097161698626, 0.9303163870417268111 ) ) ;
#35907=CARTESIAN_POINT ( 'NONE',  ( -22.96225337745244488, 150.1545470440437953, -0.6883021358963677949 ) ) ;
#35911=CARTESIAN_POINT ( 'NONE',  ( -8.625020111792197852, 118.6230397979781799, 0.7981352872006625132 ) ) ;
#35914=CARTESIAN_POINT ( 'NONE',  ( -0.009513433763583356226, 117.6614778598761291, 0.4760911276077179899 ) ) ;
#35915=CARTESIAN_POINT ( 'NONE',  ( 17.73303733098136448, 151.6044147853587845, -1.711203799303050666 ) ) ;
#35916=CARTESIAN_POINT ( 'NONE',  ( 0.9260135661551653907, 3.379156789086214197, -0.3022368940483516897 ) ) ;
#35917=CARTESIAN_POINT ( 'NONE',  ( -2.144872632962109726, 6.596990873201863614, -8.179991544870226505 ) ) ;
#35918=CARTESIAN_POINT ( 'NONE',  ( -21.77023485109867451, 148.7205309135917730, -2.145821470179948509 ) ) ;
#35919=CARTESIAN_POINT ( 'NONE',  ( 4.677687236059855813, 117.8847412557266239, -0.8181935875056758345 ) ) ;
#35920=CARTESIAN_POINT ( 'NONE',  ( 7.499048524200883747, 123.6595150816924047, 0.1842243911843320370 ) ) ;
#35921=CARTESIAN_POINT ( 'NONE',  ( 11.17088054096560334, 124.6236798342360856, -0.9649352710901085706 ) ) ;
#35922=CARTESIAN_POINT ( 'NONE',  ( -9.145901261935915016, 124.1724329610943300, -0.1484858654357238128 ) ) ;
#35924=CARTESIAN_POINT ( 'NONE',  ( -3.977359857055012604, 157.1622345443605582, -1.793852766001656329 ) ) ;
#35925=CARTESIAN_POINT ( 'NONE',  ( 3.918620257527314799, -15.59263167233598857, 4.836928646374421881 ) ) ;
#35928=EDGE_LOOP ( 'NONE', ( #20944, #9473, #23833, #10022 ) ) ;
#35929=CARTESIAN_POINT ( 'NONE',  ( 3.364155546990415857, 119.5845705363850442, 0.8331338896180615627 ) ) ;
#35930=CARTESIAN_POINT ( 'NONE',  ( 3.606404759574667995, -11.68799792153887296, 0.6759542868570080909 ) ) ;
#35931=CARTESIAN_POINT ( 'NONE',  ( 5.165779723667151657, 115.7029491485453008, 1.236970719217007408 ) ) ;
#35932=CARTESIAN_POINT ( 'NONE',  ( -3.175984444280743446, 117.6701293611589278, 0.8859276027576485912 ) ) ;
#35933=CARTESIAN_POINT ( 'NONE',  ( -8.304712878168881929, 22.30428017260781459, 1.495267265505846765 ) ) ;
#35934=CARTESIAN_POINT ( 'NONE',  ( 1.557716402914177012, 120.7946061759640486, 0.2396963980366531854 ) ) ;
#35935=CARTESIAN_POINT ( 'NONE',  ( 9.582280438405291534, 118.3624989119526418, -0.5072503739029415870 ) ) ;
#35936=CARTESIAN_POINT ( 'NONE',  ( -5.010144981628188887, 117.3993855238222608, -0.7522679339500687457 ) ) ;
#35938=CARTESIAN_POINT ( 'NONE',  ( -8.078287538471746743, 158.6595088495342338, -0.1614234102745197019 ) ) ;
#35940=CARTESIAN_POINT ( 'NONE',  ( 6.747353831446265104, 120.9730903663792247, -0.7368456446025557494 ) ) ;
#35941=CARTESIAN_POINT ( 'NONE',  ( 5.253579998758207914, -14.72808323979572442, 3.743261050348050123 ) ) ;
#35942=CARTESIAN_POINT ( 'NONE',  ( -15.39048793250127289, 143.5427300040290106, -0.9094471879209007348 ) ) ;
#35943=CARTESIAN_POINT ( 'NONE',  ( 3.464659682708206123, -14.15734315221130224, 4.609430909834149048 ) ) ;
#35944=DIRECTION ( 'NONE',  ( -4.017660918040594346E-17, 1.000000000000000000, 2.376309959284834438E-19 ) ) ;
#35945=CARTESIAN_POINT ( 'NONE',  ( 22.75563279970854325, 137.3797884758947703, 0.4783205966563214839 ) ) ;
#35947=CARTESIAN_POINT ( 'NONE',  ( -4.478778176974228309, 3.316883148187759645, 1.141857468124592101 ) ) ;
#35948=CARTESIAN_POINT ( 'NONE',  ( 1.511522926053362248, 105.1238775886715047, 5.125126382528155666 ) ) ;
#35949=CARTESIAN_POINT ( 'NONE',  ( -5.008842170714641107, 117.3975374489157133, 0.7756408261732131715 ) ) ;
#35951=CARTESIAN_POINT ( 'NONE',  ( -6.092137319721709687, 121.3195672157765728, 0.2700191901338648282 ) ) ;
#35952=CARTESIAN_POINT ( 'NONE',  ( -2.651420880294951488, 7.049774601622781134, -3.792306073587544901 ) ) ;
#35953=CARTESIAN_POINT ( 'NONE',  ( -0.01443894962469085066, 159.4760848062415732, 0.7225840825867287931 ) ) ;
#35956=CARTESIAN_POINT ( 'NONE',  ( 0.02768730785345232051, 158.9256195073445213, -1.385586103196075447 ) ) ;
#35957=CARTESIAN_POINT ( 'NONE',  ( -1.220754042303205500, 16.12054255322086860, -4.471266627502475721 ) ) ;
#35958=CARTESIAN_POINT ( 'NONE',  ( -14.73023064483748712, 156.1040168620350244, -1.249499669456201500 ) ) ;
#35960=CARTESIAN_POINT ( 'NONE',  ( -1.630522158633651797, 156.2764358050213787, 0.3353572448990094768 ) ) ;
#35962=CARTESIAN_POINT ( 'NONE',  ( 6.287662417442902552, -13.15673151805442309, 0.9153646538742283845 ) ) ;
#35963=CARTESIAN_POINT ( 'NONE',  ( -2.742874663339857744, 107.9144754008248981, -4.446420073853355248 ) ) ;
#35965=CARTESIAN_POINT ( 'NONE',  ( -0.03245814172817947096, 158.1186941186938952, 1.624338139048501439 ) ) ;
#35966=FACE_OUTER_BOUND ( 'NONE', #1909, .T. ) ;
#35967=CARTESIAN_POINT ( 'NONE',  ( 8.935197197525127422, 123.9063447689825779, 0.1785465045940572426 ) ) ;
#35969=CARTESIAN_POINT ( 'NONE',  ( -10.39199171643970665, 157.8614378686282862, 0.7539791864280581679 ) ) ;
#35970=CARTESIAN_POINT ( 'NONE',  ( 20.08431799972932907, 128.8637844977697569, -0.1093955315764415515 ) ) ;
#35978=CARTESIAN_POINT ( 'NONE',  ( -4.662175683825617867, 118.0285603771968965, 0.5801233676060106870 ) ) ;
#35982=CARTESIAN_POINT ( 'NONE',  ( -2.766040590020705903, 118.7629491485426172, -1.199722955718958151 ) ) ;
#35984=CARTESIAN_POINT ( 'NONE',  ( -8.379299793194181945, 119.6055850948818886, -1.415703317849449361 ) ) ;
#35985=CARTESIAN_POINT ( 'NONE',  ( -5.227922695814451792, 116.4790307410953289, -1.091139864702252327 ) ) ;
#35986=CARTESIAN_POINT ( 'NONE',  ( 4.571649082125946784, 118.0412581531131906, 0.8381018338667312051 ) ) ;
#35989=CARTESIAN_POINT ( 'NONE',  ( -16.45678414710234350, 146.8700648836752691, -1.605370559133787900 ) ) ;
#35992=CARTESIAN_POINT ( 'NONE',  ( 2.169980103648475378, 106.6933082031156772, -4.882050113528205948 ) ) ;
#35993=CARTESIAN_POINT ( 'NONE',  ( -17.05487166051804593, 147.7912591418244403, -2.046378512860587584 ) ) ;
#35996=CARTESIAN_POINT ( 'NONE',  ( -0.01645572339173941370, 159.4324016994384010, 0.8235116888278194436 ) ) ;
#35997=CARTESIAN_POINT ( 'NONE',  ( 8.343164213270776841, 120.0286413096534233, -1.117317573728690894 ) ) ;
#35998=CARTESIAN_POINT ( 'NONE',  ( -13.59213104125035265, 150.2515543379227267, -0.2066863870687406513 ) ) ;
#35999=CARTESIAN_POINT ( 'NONE',  ( 3.746277899330032302, -0.8937244826341392834, -2.755274729908455900 ) ) ;
#36000=CARTESIAN_POINT ( 'NONE',  ( 22.98914810635003647, 149.5377445326608665, 1.186953142822410490 ) ) ;
#36002=DIRECTION ( 'NONE',  ( 4.017660918040594346E-17, -1.000000000000000000, -2.376309959284834438E-19 ) ) ;
#36003=CARTESIAN_POINT ( 'NONE',  ( 3.303734845180175128, -14.82389436555148166, -0.08037074644983704941 ) ) ;
#36004=CARTESIAN_POINT ( 'NONE',  ( -4.252934711844699400, 157.4559852174668322, 1.675102021473321878 ) ) ;
#36005=CARTESIAN_POINT ( 'NONE',  ( 0.04477287412000752198, 14.82196177864132380, -0.9729305925282246692 ) ) ;
#36006=CARTESIAN_POINT ( 'NONE',  ( 0.004355829920540938045, 116.7171338949676738, -0.2179835409713597183 ) ) ;
#36007=CARTESIAN_POINT ( 'NONE',  ( 0.03652159268533760467, -3.380040448513521589, 0.9750733386546841519 ) ) ;
#36010=CARTESIAN_POINT ( 'NONE',  ( 4.757567707637461396, 116.6039038697339549, 1.126183464948452784 ) ) ;
#36012=CARTESIAN_POINT ( 'NONE',  ( -0.7306116569920545478, 156.4221767039705071, 0.6844267650493707222 ) ) ;
#36013=CARTESIAN_POINT ( 'NONE',  ( 4.292324012607982908, -12.68181061970326340, 2.304565294163185118 ) ) ;
#36014=CARTESIAN_POINT ( 'NONE',  ( 10.46700094992492680, 122.9580799906392343, -1.049763322952065536 ) ) ;
#36015=CARTESIAN_POINT ( 'NONE',  ( -2.271387047179101337, 118.5910164976458532, -0.7981300483413859004 ) ) ;
#36016=CARTESIAN_POINT ( 'NONE',  ( 2.781118144868611974, -14.77119122201073154, 4.489572933734862659 ) ) ;
#36017=CARTESIAN_POINT ( 'NONE',  ( -3.328555392133317525, 33.88165127674241717, 1.160568618710268174 ) ) ;
#36019=CARTESIAN_POINT ( 'NONE',  ( 0.003550340867663489587, 156.3099534201614631, -0.1776735749810080811 ) ) ;
#36024=TOROIDAL_SURFACE ( 'NONE', #19001, 5.080000000000005400, 0.5080000000000000071 ) ;
#36025=DIRECTION ( 'NONE',  ( 0.9998004120163608288, 5.205824365704081956E-17, 0.01997839162482748995 ) ) ;
#36026=ADVANCED_FACE ( 'NONE', ( #39023 ), #25644, .F. ) ;
#36028=B_SPLINE_CURVE_WITH_KNOTS ( 'NONE', 3,
 ( #10236, #29630, #19810, #17044 ),
 .UNSPECIFIED., .F., .F.,
 ( 4, 4 ),
 ( -5.999999999756005006E-08, 0.0002276942339102930096 ),
 .UNSPECIFIED. ) ;
#36029=CARTESIAN_POINT ( 'NONE',  ( 0.0008202526017140943961, 159.6052337359418800, -0.04104879434819951045 ) ) ;
#36030=CARTESIAN_POINT ( 'NONE',  ( -5.774381877465555313, 118.4424948052634647, 0.4329097047088600325 ) ) ;
#36031=CARTESIAN_POINT ( 'NONE',  ( -0.7418435039310978807, 115.6909491485452435, 1.732013647045983928 ) ) ;
#36033=CARTESIAN_POINT ( 'NONE',  ( 1.934221275448955391, 38.68736563468869605, -1.199403792597403706 ) ) ;
#36034=CARTESIAN_POINT ( 'NONE',  ( 14.93032553133218521, 154.7288491705591866, 2.132398917750006895 ) ) ;
#36035=CARTESIAN_POINT ( 'NONE',  ( -2.714482067202859561, 26.26591195808746448, -3.750338772627290762 ) ) ;
#36036=CARTESIAN_POINT ( 'NONE',  ( -5.435345482397000438, 30.30303275347894854, -6.432456514813170045 ) ) ;
#36037=CARTESIAN_POINT ( 'NONE',  ( 5.511471034203434094, 117.2322532230211749, -0.5987457750600796436 ) ) ;
#36038=CARTESIAN_POINT ( 'NONE',  ( -1.549819036667766659, 118.0223913815010377, -1.039293717761402336 ) ) ;
#36040=CARTESIAN_POINT ( 'NONE',  ( -2.697694248221544022, 107.8416071541323049, -4.476792151442584355 ) ) ;
#36041=CARTESIAN_POINT ( 'NONE',  ( 2.764046652421120243, 104.6144662015456959, 3.957270357869250521 ) ) ;
#36042=CARTESIAN_POINT ( 'NONE',  ( 4.458631606973747274, 16.91056413504885825, 1.251853190366734259 ) ) ;
#36045=CARTESIAN_POINT ( 'NONE',  ( 3.220330141560203696, -14.30903721375789317, 2.546581355196453345 ) ) ;
#36046=B_SPLINE_CURVE_WITH_KNOTS ( 'NONE', 3,
 ( #34212, #17785, #37602, #36990 ),
 .UNSPECIFIED., .F., .F.,
 ( 4, 4 ),
 ( 0.000000000000000000, 1.000000000000000000 ),
 .UNSPECIFIED. ) ;
#36047=CARTESIAN_POINT ( 'NONE',  ( 1.490732016122372716, 115.2915405621345144, -1.797152713846302818 ) ) ;
#36048=CARTESIAN_POINT ( 'NONE',  ( -15.74805233917012437, 121.4292885696920621, 0.3002298764450370694 ) ) ;
#36049=CARTESIAN_POINT ( 'NONE',  ( 4.922922108635476413, 117.4088122501876796, -0.9491512982636605145 ) ) ;
#36055=CARTESIAN_POINT ( 'NONE',  ( 2.008732664060286055, -15.70244684250787870, 5.701976698490775597 ) ) ;
#36056=CARTESIAN_POINT ( 'NONE',  ( -17.46960851010923577, 131.6241255656270255, 1.599527815159631938 ) ) ;
#36057=CARTESIAN_POINT ( 'NONE',  ( 13.98214753592664827, 155.8415165211600595, -1.292431576881028832 ) ) ;
#36058=CARTESIAN_POINT ( 'NONE',  ( 0.03997419820544263758, 30.08235846857972007, -0.9743396344490610206 ) ) ;
#36061=ORIENTED_EDGE ( 'NONE', *, *, #28465, .T. ) ;
#36063=CARTESIAN_POINT ( 'NONE',  ( -0.1065646865916383690, 105.8844662015456919, 5.332932678536313809 ) ) ;
#36064=SURFACE_SIDE_STYLE ('',( #26035 ) ) ;
#36065=CARTESIAN_POINT ( 'NONE',  ( -0.008308630153272997601, 120.0570981805881559, 0.4157978282972241701 ) ) ;
#36068=CARTESIAN_POINT ( 'NONE',  ( 6.644289941094775109, 120.1594786313440011, -0.9502652795725030632 ) ) ;
#36069=CARTESIAN_POINT ( 'NONE',  ( -2.160664645061537215, 117.9909145081919917, -0.7315704174731481046 ) ) ;
#36072=CARTESIAN_POINT ( 'NONE',  ( 4.554969932097885810, 118.0892972403241430, -0.5841261413086886733 ) ) ;
#36073=CARTESIAN_POINT ( 'NONE',  ( 13.80952258003148181, 150.2278160098252329, -0.4282869786672486856 ) ) ;
#36075=CARTESIAN_POINT ( 'NONE',  ( -6.563805965709591739, 120.5225452898634728, -1.124017915699711878 ) ) ;
#36076=CARTESIAN_POINT ( 'NONE',  ( 3.373996639098103323, -14.83046237366941789, 1.396824179944331723 ) ) ;
#36078=DIRECTION ( 'NONE',  ( 0.9998004120163610509, 4.016384292689131511E-17, 0.01997839162482749689 ) ) ;
#36082=CARTESIAN_POINT ( 'NONE',  ( -2.972019672840211513, 9.848453565018933986, 3.538668892428941781 ) ) ;
#36083=CARTESIAN_POINT ( 'NONE',  ( -0.009513407573742645174, 119.7614543879625586, 0.4760898169610157660 ) ) ;
#36084=CARTESIAN_POINT ( 'NONE',  ( -2.651199864046426491, 30.19476482558288311, -0.03810942705075580361 ) ) ;
#36085=EDGE_CURVE ( 'NONE', #12743, #24610, #20528, .T. ) ;
#36086=CARTESIAN_POINT ( 'NONE',  ( 4.037907715354051241, 27.70556447992504445, -2.267523456217593214 ) ) ;
#36087=CARTESIAN_POINT ( 'NONE',  ( 7.814053207647945420, 154.6216606121152495, 0.3474563751001367162 ) ) ;
#36088=CARTESIAN_POINT ( 'NONE',  ( -2.959623698042840534, 107.4064645821210462, 4.429364252002888414 ) ) ;
#36090=CARTESIAN_POINT ( 'NONE',  ( -5.562407735369682804, 116.6996333467663050, -0.1111501472963696002 ) ) ;
#36091=CARTESIAN_POINT ( 'NONE',  ( -4.801770124281918406, 117.3993836135855133, 1.016061139389656587 ) ) ;
#36094=CARTESIAN_POINT ( 'NONE',  ( -8.261285051657653256, 120.1778800549205073, -1.448705368892842849 ) ) ;
#36097=CARTESIAN_POINT ( 'NONE',  ( -4.074955089416341991, 118.2429491485453354, 0.1454234154749719787 ) ) ;
#36101=CARTESIAN_POINT ( 'NONE',  ( -21.87358050093881090, 151.4416708234707301, -0.1116233529550398618 ) ) ;
#36104=CARTESIAN_POINT ( 'NONE',  ( -6.979245073245229136, 121.9493068413915040, -0.1922076700199186194 ) ) ;
#36108=CARTESIAN_POINT ( 'NONE',  ( -15.37864313207211175, 147.8292851303062321, -0.3583584359702443045 ) ) ;
#36109=CARTESIAN_POINT ( 'NONE',  ( 2.081461833008368512, -15.42522581128935499, 5.972092850182497692 ) ) ;
#36110=CARTESIAN_POINT ( 'NONE',  ( -13.46025642088320673, 121.5866728338796463, 1.110021706884414483 ) ) ;
#36111=CARTESIAN_POINT ( 'NONE',  ( 4.300553167417687561, 27.50566818391071422, -1.719522505244270860 ) ) ;
#36112=CARTESIAN_POINT ( 'NONE',  ( 7.991309159113032301, 158.6817341734954425, 0.4848270063548279496 ) ) ;
#36113=CARTESIAN_POINT ( 'NONE',  ( 2.262096742913059622, -15.42953798115688535, 5.841406647620562609 ) ) ;
#36115=CARTESIAN_POINT ( 'NONE',  ( 0.3393679441828953980, -8.777600141791896959, -0.9147772600509928020 ) ) ;
#36116=CARTESIAN_POINT ( 'NONE',  ( -18.71175911766657762, 125.2636347375217838, -0.5504587009833170619 ) ) ;
#36117=CYLINDRICAL_SURFACE ( 'NONE', #38598, 3.175000000000001155 ) ;
#36120=CARTESIAN_POINT ( 'NONE',  ( -5.560790277979172025, 116.7475871101181895, 0.1053522238722745114 ) ) ;
#36122=CARTESIAN_POINT ( 'NONE',  ( -7.412650754288892863, 120.7277362223577768, 0.9451843054385556941 ) ) ;
#36124=CARTESIAN_POINT ( 'NONE',  ( 14.96081243412104200, 123.1914926142276130, 1.724312424550131784 ) ) ;
#36125=CARTESIAN_POINT ( 'NONE',  ( 15.81176147471969529, 128.5598958631237565, -1.562949982248214242 ) ) ;
#36126=CARTESIAN_POINT ( 'NONE',  ( 0.9435450883166688341, 2.505659174922684418, 0.2465458143858453577 ) ) ;
#36127=CARTESIAN_POINT ( 'NONE',  ( -21.97492997894005029, 149.1257232373000647, -2.026018130409337648 ) ) ;
#36128=CARTESIAN_POINT ( 'NONE',  ( 4.678169868823534472, 118.0125419685739416, -0.6044271497212726496 ) ) ;
#36129=CARTESIAN_POINT ( 'NONE',  ( 5.487604538598316317, 117.4962825466697467, 0.8290304003371103958 ) ) ;
#36130=CARTESIAN_POINT ( 'NONE',  ( 16.34996387626492620, 143.9496486471311698, -1.129508837753296469 ) ) ;
#36131=CARTESIAN_POINT ( 'NONE',  ( -7.044606587285223931, 122.0729346620515088, -0.1407680048458704314 ) ) ;
#36133=CARTESIAN_POINT ( 'NONE',  ( -1.321503922127654551, 119.3298839580929638, -0.6528639922554045905 ) ) ;
#36134=CARTESIAN_POINT ( 'NONE',  ( 3.743762692837560468, -15.60843739440008449, 4.988928788737716502 ) ) ;
#36136=CIRCLE ( 'NONE', #40864, 0.5080000000000002292 ) ;
#36139=CARTESIAN_POINT ( 'NONE',  ( 16.38646240326715287, 135.1966315799913900, 2.295807278541857954 ) ) ;
#36140=CARTESIAN_POINT ( 'NONE',  ( -5.176850267262477878, 31.60528704468920580, -0.07969122161898606338 ) ) ;
#36142=CIRCLE ( 'NONE', #2113, 5.588000000000006295 ) ;
#36144=CARTESIAN_POINT ( 'NONE',  ( -5.582679110870683026, 119.7830797108918688, 0.2735363082852449446 ) ) ;
#36145=CARTESIAN_POINT ( 'NONE',  ( 2.403447530314441583, 28.79142288871172539, -8.109455235164826803 ) ) ;
#36146=CARTESIAN_POINT ( 'NONE',  ( 5.883037304650295063, 121.3687970875902806, 0.4830333308872108433 ) ) ;
#36147=CARTESIAN_POINT ( 'NONE',  ( 11.36388202081341170, 118.9804978796424706, -0.4533785775503093030 ) ) ;
#36148=CARTESIAN_POINT ( 'NONE',  ( 5.339080835687772364, 115.7029491485453150, -0.2011480626654460757 ) ) ;
#36150=CARTESIAN_POINT ( 'NONE',  ( -13.43647848967396818, 156.9186530619738562, -0.2471310363275582567 ) ) ;
#36152=CARTESIAN_POINT ( 'NONE',  ( 8.061888348283327232, 121.3793065287195958, -0.9018960436474696696 ) ) ;
#36153=CARTESIAN_POINT ( 'NONE',  ( 6.309668351831440702, -13.80474515357695076, 1.045049453412914664 ) ) ;
#36154=CARTESIAN_POINT ( 'NONE',  ( -7.919085485410461089, 154.5997988942315260, -0.6546929905378091608 ) ) ;
#36155=CARTESIAN_POINT ( 'NONE',  ( 2.780001287168888613, -14.74817992026429536, 5.465600930587551254 ) ) ;
#36156=CARTESIAN_POINT ( 'NONE',  ( -3.950580610161007922, 117.4679918459733585, 0.5815556119072164964 ) ) ;
#36158=AXIS2_PLACEMENT_3D ( 'NONE', #40527, #8557, #21729 ) ;
#36159=CARTESIAN_POINT ( 'NONE',  ( 8.215520591712387244, 117.5015518944296247, 0.2087872862963604248 ) ) ;
#36161=CARTESIAN_POINT ( 'NONE',  ( -2.424025297795170619, -5.104216246930970868, 3.935102955759355758 ) ) ;
#36162=CARTESIAN_POINT ( 'NONE',  ( -22.76738278397264281, 137.3906169244638136, -0.4549464913834382340 ) ) ;
#36163=CARTESIAN_POINT ( 'NONE',  ( 3.682264917456193221, 78.32546620154573702, 0.07358041635424013294 ) ) ;
#36165=CARTESIAN_POINT ( 'NONE',  ( 7.799194557895424929, 122.5298883528417662, 0.4369513083720456548 ) ) ;
#36166=CARTESIAN_POINT ( 'NONE',  ( 4.099978103716023448, 4.450953565018914482, -2.131961072590273343 ) ) ;
#36167=CARTESIAN_POINT ( 'NONE',  ( 13.61640385012393928, 120.8017016962898396, 1.366196570323218396 ) ) ;
#36168=DIRECTION ( 'NONE',  ( -4.017660918040594346E-17, 1.000000000000000000, 2.376309959284834438E-19 ) ) ;
#36170=CARTESIAN_POINT ( 'NONE',  ( 20.47035330145901000, 150.0074677946399504, -1.517022030030164892 ) ) ;
#36172=CARTESIAN_POINT ( 'NONE',  ( 0.7003524534433175353, 11.14785949628657669, 4.567531960304466843 ) ) ;
#36173=CARTESIAN_POINT ( 'NONE',  ( -13.03166249679917321, 119.8917521002241955, -1.045815086349644707 ) ) ;
#36175=CARTESIAN_POINT ( 'NONE',  ( -8.112862105099743815, 122.9271997657465931, -0.1621142923986426398 ) ) ;
#36176=CARTESIAN_POINT ( 'NONE',  ( -6.492420186392395820, 121.7431354732680973, 0.05225946255319178363 ) ) ;
#36177=CARTESIAN_POINT ( 'NONE',  ( 4.721559244837001401, -14.40436002768456802, 4.408607674763740825 ) ) ;
#36179=CARTESIAN_POINT ( 'NONE',  ( -1.187539700871899528, 106.2993931590553274, -5.152244660853054548 ) ) ;
#36180=EDGE_LOOP ( 'NONE', ( #31711, #30321, #36902, #39982 ) ) ;
#36181=CARTESIAN_POINT ( 'NONE',  ( 7.606098120226983283, 119.7866739149480253, 1.386975461113101771 ) ) ;
#36183=CARTESIAN_POINT ( 'NONE',  ( 11.82813386268891165, 130.3161362890850512, 0.2363542639706544268 ) ) ;
#36184=VECTOR ( 'NONE', #205, 1000.000000000000000 ) ;
#36186=CARTESIAN_POINT ( 'NONE',  ( -14.76838793310970388, 156.1040168620350244, 0.6600470674582795683 ) ) ;
#36187=CARTESIAN_POINT ( 'NONE',  ( -7.601118931484537100, 27.11072341857771306, -3.643763446188946542 ) ) ;
#36188=CARTESIAN_POINT ( 'NONE',  ( 7.966904459259814608, 158.6775731370129279, -0.2701962758350452964 ) ) ;
#36192=CARTESIAN_POINT ( 'NONE',  ( 2.026452703349827633, -15.26483848100516916, 5.365780487320932934 ) ) ;
#36195=CARTESIAN_POINT ( 'NONE',  ( -4.414199990641388460, 118.1799141087742555, 0.3933343983828669899 ) ) ;
#36199=CARTESIAN_POINT ( 'NONE',  ( -8.302816400183525403, 119.9753945280262712, -1.448211312683703955 ) ) ;
#36200=CARTESIAN_POINT ( 'NONE',  ( -6.287821989302600834, 120.0808430858776887, -0.4528678087849540845 ) ) ;
#36201=CARTESIAN_POINT ( 'NONE',  ( 4.512686109237062482, 118.0696626847395976, 0.8150047576444854336 ) ) ;
#36202=CARTESIAN_POINT ( 'NONE',  ( -15.88363809060984799, 147.6644253265642135, -1.281895537487840464 ) ) ;
#36203=CARTESIAN_POINT ( 'NONE',  ( -2.438095677481897816, 115.7029724308332277, -1.698769770220674102 ) ) ;
#36205=CARTESIAN_POINT ( 'NONE',  ( 1.576215671565278864, 106.2483430537416638, -5.109971884176318646 ) ) ;
#36206=CARTESIAN_POINT ( 'NONE',  ( -16.09426298050584947, 139.8573806175465961, -2.037321532313223660 ) ) ;
#36208=CARTESIAN_POINT ( 'NONE',  ( -0.03212618750959882197, 158.2819368290249713, 1.607725792532325393 ) ) ;
#36209=CARTESIAN_POINT ( 'NONE',  ( 8.036149603167988431, 121.5005262100066830, -0.8572904197356677747 ) ) ;
#36210=CARTESIAN_POINT ( 'NONE',  ( -15.26612506134334524, 148.0236973083020473, -0.1719504695324379495 ) ) ;
#36211=EDGE_CURVE ( 'NONE', #24610, #3481, #12915, .T. ) ;
#36212=CARTESIAN_POINT ( 'NONE',  ( 1.686640475165922748, -9.627085671684914914, -4.319569293544198274 ) ) ;
#36213=CARTESIAN_POINT ( 'NONE',  ( 0.3250403508452471835, 116.7787044104018861, 0.2632219653755004107 ) ) ;
#36214=CARTESIAN_POINT ( 'NONE',  ( -6.474089935681887051E-14, 69.94346620154573202, 3.752704589293910110E-29 ) ) ;
#36215=CARTESIAN_POINT ( 'NONE',  ( 3.406014632911877893, -14.97454077108105430, 2.395711393442250259 ) ) ;
#36216=CARTESIAN_POINT ( 'NONE',  ( -18.78250995143904234, 149.1225091032880528, 1.736135053443003784 ) ) ;
#36217=CARTESIAN_POINT ( 'NONE',  ( 0.8366737682863060188, 2.078006455476229419, 0.4978880095337852585 ) ) ;
#36218=CARTESIAN_POINT ( 'NONE',  ( -11.50728102546042031, 118.8226552325407397, -0.6924515317502045741 ) ) ;
#36220=CARTESIAN_POINT ( 'NONE',  ( -0.1630216852218501489, 24.74361041950371032, -0.9604350664704873752 ) ) ;
#36223=CARTESIAN_POINT ( 'NONE',  ( 5.210481185491484979, 116.4925209815607730, 1.089480302653437871 ) ) ;
#36224=CARTESIAN_POINT ( 'NONE',  ( -15.65625195688312843, 148.1291547725267037, 0.6483782694814675951 ) ) ;
#36225=CARTESIAN_POINT ( 'NONE',  ( 3.965039388734942882, -13.93407386435618989, 4.333124597978631698 ) ) ;
#36226=CARTESIAN_POINT ( 'NONE',  ( 11.97328186178008380, 153.4554508723442439, -1.471200310048991433 ) ) ;
#36227=CARTESIAN_POINT ( 'NONE',  ( -5.837434872615095749, 119.2401804501882197, -1.198870938642750739 ) ) ;
#36228=CARTESIAN_POINT ( 'NONE',  ( -6.529493367164978770E-14, 72.99146620154573384, -7.899616498973244731E-18 ) ) ;
#36230=CARTESIAN_POINT ( 'NONE',  ( 2.904419875024614850, -13.46177902185440090, 0.8499660341922408158 ) ) ;
#36231=CARTESIAN_POINT ( 'NONE',  ( -6.444213031565760197, 30.20499910742390881, -0.3026784529137391822 ) ) ;
#36232=CARTESIAN_POINT ( 'NONE',  ( 8.581106358026191927, 123.3373102669514765, 0.01935445114830166430 ) ) ;
#36235=CARTESIAN_POINT ( 'NONE',  ( -3.041852915713540551, 107.5205933461800640, 4.373098560481015085 ) ) ;
#36236=CARTESIAN_POINT ( 'NONE',  ( -0.1058213901579904276, 105.9761915687788587, 5.295735085525931751 ) ) ;
#36241=CARTESIAN_POINT ( 'NONE',  ( 0.9075203043613222498, 116.4850453793277865, -0.07935580435194640458 ) ) ;
#36242=CARTESIAN_POINT ( 'NONE',  ( -2.177262389793364061, 106.6864334246082961, 4.884315812310542348 ) ) ;
#36244=CARTESIAN_POINT ( 'NONE',  ( -0.8426312062438860995, 115.6909491485452435, 1.724999377526929889 ) ) ;
#36245=CARTESIAN_POINT ( 'NONE',  ( -1.217056272985401533, 34.90614901474430098, 0.2337217464280959833 ) ) ;
#36246=CARTESIAN_POINT ( 'NONE',  ( 16.44465323483251495, 153.5550899668227203, 2.240181424793372678 ) ) ;
#36247=CARTESIAN_POINT ( 'NONE',  ( 4.064150447026247726, 23.66704930264554818, -2.198397014704132513 ) ) ;
#36248=CARTESIAN_POINT ( 'NONE',  ( 8.243228241119590294, 17.55835651096333194, -1.765626013165721320 ) ) ;
#36249=CARTESIAN_POINT ( 'NONE',  ( 2.354862059299378085, 117.2183826610675652, -0.5773916514328522043 ) ) ;
#36250=CARTESIAN_POINT ( 'NONE',  ( 0.1065646865915095137, 105.8844662015456777, -5.332932678536313809 ) ) ;
#36253=CARTESIAN_POINT ( 'NONE',  ( -1.940427529279133090, 104.6144662015434648, 4.971597247601878600 ) ) ;
#36255=CARTESIAN_POINT ( 'NONE',  ( 2.584458374606236841, 15.83607344512877368, 3.832284875798456447 ) ) ;
#36257=CARTESIAN_POINT ( 'NONE',  ( -23.42514220145546133, 142.8382549600663083, -0.4680900899251589919 ) ) ;
#36258=CARTESIAN_POINT ( 'NONE',  ( 3.171691571413298050, -13.57474810710837509, 1.775319381694977716 ) ) ;
#36260=CARTESIAN_POINT ( 'NONE',  ( 1.603046668355785132, 118.6366899268033279, -0.8036507178775275095 ) ) ;
#36261=CARTESIAN_POINT ( 'NONE',  ( -18.27977197196865689, 154.1370782493726210, 0.5456809356757471585 ) ) ;
#36263=CARTESIAN_POINT ( 'NONE',  ( 4.854507468356392685, 117.4057973178051526, -0.9983053292619181729 ) ) ;
#36266=( BOUNDED_CURVE ( )  B_SPLINE_CURVE ( 3, ( #2647, #28824, #28405, #35225 ),
 .UNSPECIFIED., .F., .F. ) 
 B_SPLINE_CURVE_WITH_KNOTS ( ( 4, 4 ),
 ( 0.6038647612415126709, 0.6486116422890977340 ),
 .UNSPECIFIED. ) 
 CURVE ( )  GEOMETRIC_REPRESENTATION_ITEM ( )  RATIONAL_B_SPLINE_CURVE ( ( 0.6708440640561601498, 0.6359688846130079343, 0.6064331274724894527, 0.5822367926346048161 ) ) 
 REPRESENTATION_ITEM ( '' )  );
#36267=ORIENTED_EDGE ( 'NONE', *, *, #38941, .F. ) ;
#36268=CARTESIAN_POINT ( 'NONE',  ( 1.957912617769093755, 35.96399040732271857, -0.5992445403938203574 ) ) ;
#36269=CARTESIAN_POINT ( 'NONE',  ( 2.867278011408870064, -15.71882806570827640, 4.918777663456151750 ) ) ;
#36270=CARTESIAN_POINT ( 'NONE',  ( -13.96578288426892911, 123.5874490550988014, 1.342688313448305637 ) ) ;
#36271=CARTESIAN_POINT ( 'NONE',  ( 16.82967018813376825, 125.2521365416322254, -1.031881933595589995 ) ) ;
#36272=CARTESIAN_POINT ( 'NONE',  ( 3.315635589170360831, -10.27688868798473720, -3.234826238065521053 ) ) ;
#36276=CARTESIAN_POINT ( 'NONE',  ( 0.9836305199213740691, 123.5966405200008325, 0.1412250206608575975 ) ) ;
#36277=CARTESIAN_POINT ( 'NONE',  ( -6.842818979164508875, 155.5980657034081105, 1.215443052661050682 ) ) ;
#36278=CARTESIAN_POINT ( 'NONE',  ( -6.069968983247740368, 28.54777132941064721, 0.2584723001727267100 ) ) ;
#36279=CARTESIAN_POINT ( 'NONE',  ( 18.38987645279111405, 147.6341482083243761, -1.661003423535650336 ) ) ;
#36280=AXIS2_PLACEMENT_3D ( 'NONE', #9940, #29550, #32526 ) ;
#36281=CARTESIAN_POINT ( 'NONE',  ( -10.46214381725873288, 120.0128241960130424, -1.483189230905844536 ) ) ;
#36282=CARTESIAN_POINT ( 'NONE',  ( 4.854633716284414646, 115.7029491485453292, -1.279498648767039448 ) ) ;
#36283=CIRCLE ( 'NONE', #17881, 3.683000000000001162 ) ;
#36284=ORIENTED_EDGE ( 'NONE', *, *, #15270, .F. ) ;
#36285=CARTESIAN_POINT ( 'NONE',  ( 4.401957988103021968, 118.1614069291599520, -0.4937243125134848087 ) ) ;
#36286=CARTESIAN_POINT ( 'NONE',  ( 0.004350076772657346554, 120.7058980590201429, -0.2176956299261766647 ) ) ;
#36288=CARTESIAN_POINT ( 'NONE',  ( -11.20916139128205025, 123.4744472594011739, -1.589032359792267535 ) ) ;
#36289=CARTESIAN_POINT ( 'NONE',  ( 3.154745640343158630, -14.88448557395780014, 3.454683184413806174 ) ) ;
#36290=CARTESIAN_POINT ( 'NONE',  ( -5.332935397695336199, 105.1224662015457199, -0.1065647409268299373 ) ) ;
#36294=CARTESIAN_POINT ( 'NONE',  ( -1.441504266290200897, 6.599927940091079748, -4.410093354674724964 ) ) ;
#36295=CARTESIAN_POINT ( 'NONE',  ( 7.123980356063992048, 155.7895407640516510, 1.727872795330590128 ) ) ;
#36296=CARTESIAN_POINT ( 'NONE',  ( -2.965274000540799815, 30.81687845933373637, 0.1006152140846759829 ) ) ;
#36297=CARTESIAN_POINT ( 'NONE',  ( 0.6590154617207463206, 19.50938314818779062, -4.574821423538240950 ) ) ;
#36298=CARTESIAN_POINT ( 'NONE',  ( 9.673174862101884486, 124.8500477395539576, 0.3609973675953366268 ) ) ;
#36302=CARTESIAN_POINT ( 'NONE',  ( 5.554579209606487211, 116.7832337216378562, -0.2016058634275091077 ) ) ;
#36303=CARTESIAN_POINT ( 'NONE',  ( 5.757472737270592944, 159.1136035536173097, 0.1150480073142623738 ) ) ;
#36305=CARTESIAN_POINT ( 'NONE',  ( -23.36555825341177339, 148.7788340588663800, -0.4668994608413308267 ) ) ;
#36306=DIRECTION ( 'NONE',  ( 4.017660918040594346E-17, -1.000000000000000000, -2.376309959284832031E-19 ) ) ;
#36310=CARTESIAN_POINT ( 'NONE',  ( -6.373576640880495633E-14, 50.63946620154572997, 5.832708929232124832E-29 ) ) ;
#36313=CARTESIAN_POINT ( 'NONE',  ( -14.60357043488722439, 120.3300541288867862, 0.1192926189779472401 ) ) ;
#36315=ORIENTED_EDGE ( 'NONE', *, *, #40967, .F. ) ;
#36317=CARTESIAN_POINT ( 'NONE',  ( -7.790776616239916130, 122.5816380323567927, -0.3271574360425709704 ) ) ;
#36318=ADVANCED_FACE ( 'NONE', ( #39230 ), #41293, .F. ) ;
#36320=CARTESIAN_POINT ( 'NONE',  ( 4.854633716284414646, 115.7029491485453292, -1.279498648767039448 ) ) ;
#36321=CARTESIAN_POINT ( 'NONE',  ( -11.85559104777375872, 130.3381101163291760, -0.2804367443601420984 ) ) ;
#36322=CARTESIAN_POINT ( 'NONE',  ( 5.858142917232623148, -13.84584594667595603, 2.526540219170608115 ) ) ;
#36323=CARTESIAN_POINT ( 'NONE',  ( -21.36781924117701337, 148.2102652567764380, 1.461444809879598239 ) ) ;
#36324=CARTESIAN_POINT ( 'NONE',  ( -1.648064503646425649, 29.87956589480163316, -4.325937074807028715 ) ) ;
#36326=CARTESIAN_POINT ( 'NONE',  ( 22.45364888651499768, 150.7739627601066275, 0.8979154079963821422 ) ) ;
#36328=CARTESIAN_POINT ( 'NONE',  ( 2.000623374115709563, -15.62324522779390179, 5.905393795144921576 ) ) ;
#36330=CARTESIAN_POINT ( 'NONE',  ( 0.5759086045921885111, -9.199343823100290862, -0.7873135961421041662 ) ) ;
#36331=CARTESIAN_POINT ( 'NONE',  ( -15.84538651563812195, 121.0146182718019645, -0.4760991727851860977 ) ) ;
#36334=CARTESIAN_POINT ( 'NONE',  ( -2.230307283400940310, 116.2698154044227294, 0.08777694382101131065 ) ) ;
#36335=EDGE_LOOP ( 'NONE', ( #40060, #41528 ) ) ;
#36336=CARTESIAN_POINT ( 'NONE',  ( -7.451643811072202084, 155.9567503867590972, 1.565497431107724102 ) ) ;
#36338=CARTESIAN_POINT ( 'NONE',  ( 20.57609261220299501, 150.0789294893613999, 2.287104906598478316 ) ) ;
#36339=CARTESIAN_POINT ( 'NONE',  ( 17.13393749618825268, 131.5760549582342094, -1.627836260134054580 ) ) ;
#36341=CARTESIAN_POINT ( 'NONE',  ( -0.1338072975148606736, -13.68656151007796495, -0.9662261747338762863 ) ) ;
#36342=CARTESIAN_POINT ( 'NONE',  ( -22.03849170948991443, 148.8299554149626260, -2.028895537808247607 ) ) ;
#36343=CARTESIAN_POINT ( 'NONE',  ( 4.643821608714259419, 118.0368167649473747, -0.6067757769337593921 ) ) ;
#36344=CARTESIAN_POINT ( 'NONE',  ( -3.009276887026424152, 50.42904571186020490, 1.210121013456479933 ) ) ;
#36345=CARTESIAN_POINT ( 'NONE',  ( 11.42136869062004756, 126.1532465342912985, -0.7903108812046735210 ) ) ;
#36346=EDGE_CURVE ( 'NONE', #19493, #9538, #35211, .T. ) ;
#36347=CARTESIAN_POINT ( 'NONE',  ( -15.78598348091628267, 146.2390805666957192, -0.2639793761055730381 ) ) ;
#36348=ORIENTED_EDGE ( 'NONE', *, *, #28571, .F. ) ;
#36349=CARTESIAN_POINT ( 'NONE',  ( -14.78649082109382640, 128.5561590274816126, -2.111834004041170498 ) ) ;
#36350=CARTESIAN_POINT ( 'NONE',  ( 4.512673509771836677, -15.64532105467335299, 2.834742450761120303 ) ) ;
#36353=CARTESIAN_POINT ( 'NONE',  ( -4.648568650443571926, 118.0134285438809911, -0.7934044273710590955 ) ) ;
#36356=CARTESIAN_POINT ( 'NONE',  ( 18.34612162485796460, 147.3262642721504960, 2.396769171045068703 ) ) ;
#36357=CARTESIAN_POINT ( 'NONE',  ( -4.975175664203050907, 32.06598106186588382, 0.7459204072935275986 ) ) ;
#36358=CARTESIAN_POINT ( 'NONE',  ( 22.98488057257191741, 150.1591296352320910, 0.4592926148156237232 ) ) ;
#36359=CARTESIAN_POINT ( 'NONE',  ( 7.690436415270363923, 8.290658626076512050, -3.468142284020285793 ) ) ;
#36360=CARTESIAN_POINT ( 'NONE',  ( 15.56637720654300061, 147.8873989650969918, 1.033077377765619920 ) ) ;
#36362=CARTESIAN_POINT ( 'NONE',  ( 11.23106549681877020, 119.1264784044212632, -0.5965447130870017434 ) ) ;
#36363=DIRECTION ( 'NONE',  ( 0.9998004120163608288, 5.205824365704082573E-17, 0.01997839162482760098 ) ) ;
#36366=CARTESIAN_POINT ( 'NONE',  ( 1.580596280061897341, 115.6909491485452719, 1.732191492244595565 ) ) ;
#36367=CARTESIAN_POINT ( 'NONE',  ( -15.19466275752374251, 156.0906695176550443, -0.2814020119901240458 ) ) ;
#36369=CARTESIAN_POINT ( 'NONE',  ( 7.973790791625233965, 121.7927018305182827, -0.7354518077562433032 ) ) ;
#36372=CARTESIAN_POINT ( 'NONE',  ( -12.12200908156761336, 130.5412724693565849, -0.6534646642625603352 ) ) ;
#36373=CARTESIAN_POINT ( 'NONE',  ( 3.088592312018083152, -14.58504802601380490, 5.263618629775349333 ) ) ;
#36374=CARTESIAN_POINT ( 'NONE',  ( -12.81731082034063363, 120.0678233105195716, 0.7045657984066410195 ) ) ;
#36375=DIRECTION ( 'NONE',  ( 4.017660918040594346E-17, -1.000000000000000000, -2.376309959284834438E-19 ) ) ;
#36376=CARTESIAN_POINT ( 'NONE',  ( 14.87533653215386131, 120.3210621052586475, 0.3471466443384770284 ) ) ;
#36379=CARTESIAN_POINT ( 'NONE',  ( 1.104432469574216480, -9.427232690354344413, -4.492858291722996888 ) ) ;
#36380=CARTESIAN_POINT ( 'NONE',  ( -23.36121599382910219, 148.8756354988261990, -0.4668126921608655722 ) ) ;
#36383=CARTESIAN_POINT ( 'NONE',  ( -4.589236464118411796, 118.7495122949379294, 0.8846585347348726591 ) ) ;
#36384=CARTESIAN_POINT ( 'NONE',  ( 0.6256056815405413030, -8.068247431453825058, 4.577905309659676014 ) ) ;
#36385=CARTESIAN_POINT ( 'NONE',  ( 20.05503673871676540, 132.0867704272472452, 1.718978086785435178 ) ) ;
#36388=CARTESIAN_POINT ( 'NONE',  ( 14.47132921234235958, 123.3930721568691382, -1.260850717050815861 ) ) ;
#36389=CARTESIAN_POINT ( 'NONE',  ( -4.070821798575407158, -9.904843093959119216, 2.245307785351264407 ) ) ;
#36390=CARTESIAN_POINT ( 'NONE',  ( -12.99089357651424770, 156.9259531928012734, -1.181820989919032616 ) ) ;
#36392=CARTESIAN_POINT ( 'NONE',  ( -9.191362964798114987, 123.9301100385560943, 0.1344743934557743881 ) ) ;
#36393=CARTESIAN_POINT ( 'NONE',  ( 2.665431962039443992, -15.40910046105366327, 5.814861676232141008 ) ) ;
#36395=CARTESIAN_POINT ( 'NONE',  ( -3.275932770776605274, 108.4907222760759282, -4.202228437981203157 ) ) ;
#36396=ORIENTED_EDGE ( 'NONE', *, *, #20631, .F. ) ;
#36397=CARTESIAN_POINT ( 'NONE',  ( 14.48730688186159199, 125.6573275863457866, 2.042335292678053360 ) ) ;
#36400=CARTESIAN_POINT ( 'NONE',  ( -21.20416308100202585, 151.2337125027825095, 0.8636963275675618723 ) ) ;
#36401=CARTESIAN_POINT ( 'NONE',  ( 0.04286443493920111952, 25.39157861068392208, -8.424000189867014043 ) ) ;
#36402=CARTESIAN_POINT ( 'NONE',  ( 13.09552101555870784, 130.8944540161131442, 1.428626934261719272 ) ) ;
#36403=CARTESIAN_POINT ( 'NONE',  ( 18.44111676445463388, 125.1790410860780298, -0.1047302884851512295 ) ) ;
#36404=LINE ( 'NONE', #20597, #3639 ) ;
#36410=CARTESIAN_POINT ( 'NONE',  ( -4.456310623878905197, 118.1611138379835779, 0.4358899058150005335 ) ) ;
#36414=CARTESIAN_POINT ( 'NONE',  ( 3.767507399439959936, 118.8938511920684107, -0.7849653907999185609 ) ) ;
#36415=CARTESIAN_POINT ( 'NONE',  ( -3.930440796539918402, 109.7948460773305897, -3.685213129881072192 ) ) ;
#36416=CARTESIAN_POINT ( 'NONE',  ( 4.571841262500583980, 118.0790968600936424, 0.7158236320836997013 ) ) ;
#36417=CARTESIAN_POINT ( 'NONE',  ( -15.82363114525499981, 143.7482200480382346, -1.443160993194752217 ) ) ;
#36418=CARTESIAN_POINT ( 'NONE',  ( -1.253177666489279973, 115.7029074776113191, -1.740281551268416216 ) ) ;
#36419=CARTESIAN_POINT ( 'NONE',  ( 4.005922464918031167, 117.9496054017496789, -1.072511926687662376 ) ) ;
#36420=CARTESIAN_POINT ( 'NONE',  ( 0.3646759018190506851, 105.8822825325953261, -5.328619312200441271 ) ) ;
#36421=CARTESIAN_POINT ( 'NONE',  ( -16.93203274801149405, 148.0818255213264365, -2.041866944467892520 ) ) ;
#36422=CARTESIAN_POINT ( 'NONE',  ( 5.336581877858352030, 116.0444662015457595, -0.07592003752709637621 ) ) ;
#36423=CARTESIAN_POINT ( 'NONE',  ( -0.01133107913651526001, 156.3792106723807649, 0.5670535347366658652 ) ) ;
#36424=CARTESIAN_POINT ( 'NONE',  ( 8.022816897867139474, 121.5631586913658140, -0.8332660241015871216 ) ) ;
#36425=CARTESIAN_POINT ( 'NONE',  ( -7.046335199868481780, 122.0731595262481051, -0.02430996038715024440 ) ) ;
#36426=CARTESIAN_POINT ( 'NONE',  ( 2.294499597581835193, -9.852027417895397932, -4.012603411698490774 ) ) ;
#36427=CARTESIAN_POINT ( 'NONE',  ( 14.96245403159064047, 120.9606250904355704, 1.059951836595168118 ) ) ;
#36429=CARTESIAN_POINT ( 'NONE',  ( 3.315889604118840150, -14.76599673617913488, 0.9486971755708663023 ) ) ;
#36430=CARTESIAN_POINT ( 'NONE',  ( -19.07204494652747329, 148.5750135429820205, 1.735237764431467822 ) ) ;
#36431=CARTESIAN_POINT ( 'NONE',  ( 0.7131539557513479899, -7.844638678481905103, 0.6656887750258669856 ) ) ;
#36432=CARTESIAN_POINT ( 'NONE',  ( -22.52188062635582710, 150.6069110094195764, -1.039808695286016160 ) ) ;
#36433=CARTESIAN_POINT ( 'NONE',  ( -0.9409916986186561694, 26.46864381685040257, -0.2619748070941995688 ) ) ;
#36436=CARTESIAN_POINT ( 'NONE',  ( -0.1065646865916381608, 105.8844662015456777, 5.332932678536313809 ) ) ;
#36437=COLOUR_RGB ( '', 0.72549020, 0.75294118, 0.79215686) ;
#36438=CARTESIAN_POINT ( 'NONE',  ( -0.004916276843202750484, 120.6356583033945782, 0.2460305967400717997 ) ) ;
#36439=CARTESIAN_POINT ( 'NONE',  ( 4.222548444470398010, -13.63200092856201096, 3.862739453107805421 ) ) ;
#36440=CARTESIAN_POINT ( 'NONE',  ( 17.11529127082739521, 148.4623951536435698, -1.463161431351220454 ) ) ;
#36441=CARTESIAN_POINT ( 'NONE',  ( -4.285767465938752352, 157.6046910967438066, -1.850878756276731263 ) ) ;
#36443=CARTESIAN_POINT ( 'NONE',  ( 3.221527947697278904, -14.19553219070161809, 2.775880300951635071 ) ) ;
#36445=CARTESIAN_POINT ( 'NONE',  ( 15.74722489594608454, 146.9052959264698757, 0.08484200870240335424 ) ) ;
#36446=EDGE_LOOP ( 'NONE', ( #1480, #6201, #26530, #11821 ) ) ;
#36447=LINE ( 'NONE', #33463, #34292 ) ;
#36450=CARTESIAN_POINT ( 'NONE',  ( 22.69744207413518922, 137.3157656003441787, 0.3098006952201959319 ) ) ;
#36451=CARTESIAN_POINT ( 'NONE',  ( -5.292163649236576894, 116.0761519159950552, 1.031159682278862455 ) ) ;
#36452=CARTESIAN_POINT ( 'NONE',  ( 2.160577569948397780, -15.38714209653413434, 5.933462479304245640 ) ) ;
#36454=CARTESIAN_POINT ( 'NONE',  ( -3.294745019374083039, 31.35739020231596896, 0.3090114964385932139 ) ) ;
#36455=CARTESIAN_POINT ( 'NONE',  ( 3.119203903361051911, 118.1710492231644736, 0.8508709904442465222 ) ) ;
#36457=CARTESIAN_POINT ( 'NONE',  ( -4.628372119175923949, 18.04465247731148381, -0.2036312542868722320 ) ) ;
#36458=CARTESIAN_POINT ( 'NONE',  ( 0.2611430735369592582, 24.48315862702271417, 8.432237392808469068 ) ) ;
#36459=CARTESIAN_POINT ( 'NONE',  ( -5.540182818362195505, 118.0041147760924076, -1.099220559926700647 ) ) ;
#36460=CARTESIAN_POINT ( 'NONE',  ( -0.7702483762746622498, 120.5370721568272216, -0.5278276654545120961 ) ) ;
#36463=CARTESIAN_POINT ( 'NONE',  ( -4.383044586904778050, 104.6144662015500870, 3.059726520723942134 ) ) ;
#36464=CARTESIAN_POINT ( 'NONE',  ( 0.05711764529616595448, 0.5181683540770932739, -4.631227783250111862 ) ) ;
#36466=CARTESIAN_POINT ( 'NONE',  ( -16.31694223957266843, 121.4173703750124531, -0.3260513381110076714 ) ) ;
#36467=CARTESIAN_POINT ( 'NONE',  ( 3.250423480262735421, -14.11372661294146802, 3.006569077614236196 ) ) ;
#36468=CARTESIAN_POINT ( 'NONE',  ( 3.173429932894971106, 117.8122656274855871, -0.8370585861429156171 ) ) ;
#36469=CARTESIAN_POINT ( 'NONE',  ( -14.99285373232509322, 120.9606250904355704, 0.4613734978017341448 ) ) ;
#36470=CARTESIAN_POINT ( 'NONE',  ( 6.657354856306101354, 117.1094500246672538, 0.1330297933348817407 ) ) ;
#36474=CARTESIAN_POINT ( 'NONE',  ( 4.776532240430319654, -15.60394515218366251, 2.960345780779299663 ) ) ;
#36475=CARTESIAN_POINT ( 'NONE',  ( -18.54838064703208644, 135.7714211226372640, 1.677382267734012666 ) ) ;
#36476=CARTESIAN_POINT ( 'NONE',  ( 2.121647970409600514, 117.6567184779878232, -0.5798693372496743770 ) ) ;
#36477=CARTESIAN_POINT ( 'NONE',  ( -0.7497900579835341528, 31.49133049583988608, -0.6186479539722394838 ) ) ;
#36481=CARTESIAN_POINT ( 'NONE',  ( 2.328338358121097240, 124.8000875644994068, 0.05398387088914125692 ) ) ;
#36483=CARTESIAN_POINT ( 'NONE',  ( -7.262759831279749001, 121.2980461901665308, 0.7361999724971877157 ) ) ;
#36484=CARTESIAN_POINT ( 'NONE',  ( -0.01822531903872333034, 118.1564764849152738, 0.9120692297075591037 ) ) ;
#36485=CARTESIAN_POINT ( 'NONE',  ( 18.72287149482784230, 147.1333978507680627, -1.701234099286256019 ) ) ;
#36486=CARTESIAN_POINT ( 'NONE',  ( -20.66962185543556529, 147.7542213611591535, -2.445644978772824718 ) ) ;
#36488=AXIS2_PLACEMENT_3D ( 'NONE', #5146, #40911, #24284 ) ;
#36489=CARTESIAN_POINT ( 'NONE',  ( 4.116435971365464574, 118.2429491485453354, -0.1883497800502350605 ) ) ;
#36490=CARTESIAN_POINT ( 'NONE',  ( 14.97557080935131779, 148.8997249754567349, -0.5399649533830230830 ) ) ;
#36493=CARTESIAN_POINT ( 'NONE',  ( 2.572675278006325339, -15.15086880438208716, 4.677806725582212444 ) ) ;
#36494=CARTESIAN_POINT ( 'NONE',  ( 5.285208019315508210, 105.1224194135358090, -0.7957335705207263521 ) ) ;
#36496=CARTESIAN_POINT ( 'NONE',  ( 4.198131962423935271, 12.64715247731088787, 1.959332076845688553 ) ) ;
#36497=CARTESIAN_POINT ( 'NONE',  ( -0.02400040557479750369, 156.7459281804771365, 1.201078436782489600 ) ) ;
#36498=CARTESIAN_POINT ( 'NONE',  ( 0.7097672177479600331, 33.90743241353141713, 1.308455980856628731 ) ) ;
#36499=CARTESIAN_POINT ( 'NONE',  ( -0.01876340930523686876, 19.73428105357427853, -4.634220987317214657 ) ) ;
#36500=CARTESIAN_POINT ( 'NONE',  ( 9.231158399652199975, 124.2544328994657405, 0.2701740761454697326 ) ) ;
#36504=CARTESIAN_POINT ( 'NONE',  ( 5.559215554539349569, 116.7531585254012327, -0.1425236539881735154 ) ) ;
#36505=CARTESIAN_POINT ( 'NONE',  ( -1.627181853488509411, 117.3993836203756302, 1.397816796450546128 ) ) ;
#36510=CARTESIAN_POINT ( 'NONE',  ( 5.237379388564934679, 115.7029491485453292, 1.024072862575109655 ) ) ;
#36515=CARTESIAN_POINT ( 'NONE',  ( -22.47159541194106680, 150.7739627601066275, 0.0002021107738997875169 ) ) ;
#36519=CARTESIAN_POINT ( 'NONE',  ( -7.787852718269741459, 122.6010352751677033, -0.2744241607441815223 ) ) ;
#36522=CARTESIAN_POINT ( 'NONE',  ( -1.562757238090153988, 156.2577446057484281, -0.06075558507430124655 ) ) ;
#36523=CARTESIAN_POINT ( 'NONE',  ( 2.466063760571058250, -15.50753052345275940, 5.840068263025540496 ) ) ;
#36524=CARTESIAN_POINT ( 'NONE',  ( -9.140851504705459263, 119.2843051134756536, 0.9831809102843883652 ) ) ;
#36525=CARTESIAN_POINT ( 'NONE',  ( 4.377640660406503237, 26.40621510375495973, 1.544744264128281364 ) ) ;
#36526=CARTESIAN_POINT ( 'NONE',  ( 5.687008767712439017, 159.1209727096294273, 0.4156250475054877880 ) ) ;
#36527=CARTESIAN_POINT ( 'NONE',  ( 14.11204817291316083, 138.8091675146647788, 0.4809352338920104275 ) ) ;
#36528=CARTESIAN_POINT ( 'NONE',  ( 3.400481176189167343, 25.78150505744974552, 3.158589348000393482 ) ) ;
#36529=CARTESIAN_POINT ( 'NONE',  ( 0.6613080194379835630, -2.301230296243127693, 0.7179688673762391060 ) ) ;
#36530=CARTESIAN_POINT ( 'NONE',  ( -5.799544261406411216, 116.9771394561422539, -0.2896453145609860225 ) ) ;
#36532=CARTESIAN_POINT ( 'NONE',  ( 4.962080476404062246, 117.4056796065936368, 1.029808796348710143 ) ) ;
#36533=ORIENTED_EDGE ( 'NONE', *, *, #5534, .T. ) ;
#36534=CARTESIAN_POINT ( 'NONE',  ( 2.201628648472980121, 116.2290761738841525, 0.1197410424596312972 ) ) ;
#36535=CARTESIAN_POINT ( 'NONE',  ( -0.9295719194793629070, 157.1975648536147787, 1.475660455335214838 ) ) ;
#36537=CARTESIAN_POINT ( 'NONE',  ( 21.19397400757779337, 145.8710773725474610, 2.320968965272669937 ) ) ;
#36538=CARTESIAN_POINT ( 'NONE',  ( 13.45896140341249847, 123.7870877700634509, -1.380644293323453065 ) ) ;
#36539=CARTESIAN_POINT ( 'NONE',  ( 0.3265437062995015238, -4.820036860806069967, -0.9201843903956486992 ) ) ;
#36540=CARTESIAN_POINT ( 'NONE',  ( -1.196040046930182399, 159.0162744061759099, -1.350631977726330479 ) ) ;
#36542=CARTESIAN_POINT ( 'NONE',  ( 4.690458750227413987, 118.0052497351821756, -0.5846114136641620274 ) ) ;
#36544=CARTESIAN_POINT ( 'NONE',  ( 5.262496720419017393, 105.1224535734649663, 0.9374057647381621727 ) ) ;
#36545=CARTESIAN_POINT ( 'NONE',  ( 1.787077659700166077, 156.4219299504922844, -0.8362026816545214958 ) ) ;
#36546=CARTESIAN_POINT ( 'NONE',  ( 7.799334277748505961, 122.5403225720764908, 0.4385505410406168036 ) ) ;
#36548=CARTESIAN_POINT ( 'NONE',  ( -0.4867666382967937300, 119.1670848682014281, -0.5956043695837970331 ) ) ;
#36549=CARTESIAN_POINT ( 'NONE',  ( 2.719191112037562252, -15.71471113085404170, 5.040136806425350002 ) ) ;
#36550=CARTESIAN_POINT ( 'NONE',  ( -4.575234526219186471, 118.0705373586567646, -0.7555243366678462413 ) ) ;
#36551=EDGE_CURVE ( 'NONE', #1729, #3642, #1251, .T. ) ;
#36555=CARTESIAN_POINT ( 'NONE',  ( 9.942133252021193357, 155.4362223408194836, 2.105659105541914045 ) ) ;
#36557=ADVANCED_FACE ( 'NONE', ( #33897 ), #18181, .F. ) ;
#36558=CARTESIAN_POINT ( 'NONE',  ( 15.54847974360315099, 120.7212560704218589, 0.2938029371637450038 ) ) ;
#36560=CARTESIAN_POINT ( 'NONE',  ( 7.942258639034435852, 16.71227948022357523, 2.857158061122382353 ) ) ;
#36561=CARTESIAN_POINT ( 'NONE',  ( 15.83096054209195991, 147.2950763206921181, 1.041347660067663439 ) ) ;
#36562=CARTESIAN_POINT ( 'NONE',  ( 16.32943869337475817, 155.1963085991477271, -0.7556961354993015911 ) ) ;
#36566=CARTESIAN_POINT ( 'NONE',  ( -18.76910502294238370, 125.2887878443791294, -0.2589991215523649304 ) ) ;
#36568=CARTESIAN_POINT ( 'NONE',  ( 7.988278544293920369, 121.7250811996676134, -0.7665462581867787950 ) ) ;
#36569=CARTESIAN_POINT ( 'NONE',  ( -8.798071503382049130, 117.6842349159514640, -0.1758064068840608507 ) ) ;
#36571=CARTESIAN_POINT ( 'NONE',  ( -6.437058721807690810E-14, 62.83146620154573014, 4.519164521849267879E-29 ) ) ;
#36572=CARTESIAN_POINT ( 'NONE',  ( -1.615823435711636780, 156.2764358050213787, -0.4002269557471576644 ) ) ;
#36573=CARTESIAN_POINT ( 'NONE',  ( 3.194768752100229925, -14.65262985833884457, 5.377959301279905624 ) ) ;
#36574=CARTESIAN_POINT ( 'NONE',  ( -9.403995501905267673, 118.7255599110314961, 0.7521618898589479407 ) ) ;
#36576=CARTESIAN_POINT ( 'NONE',  ( 23.10830587629915556, 149.8995197111492814, 0.5387578213853486675 ) ) ;
#36577=VERTEX_POINT ( 'NONE', #24920 ) ;
#36578=CARTESIAN_POINT ( 'NONE',  ( -3.974385726840726107, -7.478117039488521023, -2.359557994316856533 ) ) ;
#36579=CARTESIAN_POINT ( 'NONE',  ( -16.30293663320045994, 121.4145675751456253, -0.3429698291441254931 ) ) ;
#36580=DIRECTION ( 'NONE',  ( 0.01997839162482749689, 1.040247600000945640E-18, -0.9998004120163610509 ) ) ;
#36583=CARTESIAN_POINT ( 'NONE',  ( 8.163255772186461812, 120.6602155040159658, 1.404671597144966144 ) ) ;
#36584=CARTESIAN_POINT ( 'NONE',  ( -2.329872802932658082, -2.670747431267189498, -3.990024091085845548 ) ) ;
#36585=CARTESIAN_POINT ( 'NONE',  ( 22.33586214876074649, 148.6363688457942942, 1.892951199575522159 ) ) ;
#36587=DIRECTION ( 'NONE',  ( 4.017660918040594346E-17, -1.000000000000000000, -2.376309959284834438E-19 ) ) ;
#36588=CARTESIAN_POINT ( 'NONE',  ( 19.23923079580225348, 135.9655892003723636, -1.583918808943347578 ) ) ;
#36589=CARTESIAN_POINT ( 'NONE',  ( 3.857898856315107761, -6.768822978661375167, 2.551181839177400601 ) ) ;
#36590=CARTESIAN_POINT ( 'NONE',  ( -5.495761340641479364, 159.0395019988757781, -0.8742782617121152011 ) ) ;
#36594=CARTESIAN_POINT ( 'NONE',  ( -9.006799368204402967, 123.6974368934138226, 0.1328627719367738713 ) ) ;
#36595=CARTESIAN_POINT ( 'NONE',  ( 4.983883817524661808, -15.00518790705197780, 4.081033524500047527 ) ) ;
#36598=CARTESIAN_POINT ( 'NONE',  ( -4.549004567883367933, 112.0093730493565545, -2.856396963121139443 ) ) ;
#36599=EDGE_LOOP ( 'NONE', ( #20463, #5923, #25630, #25655 ) ) ;
#36600=CARTESIAN_POINT ( 'NONE',  ( 2.300165013715926854, 118.7486697826011977, 0.8022418554901109555 ) ) ;
#36603=CARTESIAN_POINT ( 'NONE',  ( -16.18247977474496224, 122.8183540351560907, 0.6517309543831908414 ) ) ;
#36605=CARTESIAN_POINT ( 'NONE',  ( 5.111951166545567027, 11.99449087320206431, 6.736519543253151276 ) ) ;
#36606=CARTESIAN_POINT ( 'NONE',  ( 1.501069045181515849, 120.4980338609919386, 0.3776272143368912815 ) ) ;
#36607=DIRECTION ( 'NONE',  ( -5.206863593109713661E-17, 1.000000000000000000, -1.077750396879097183E-30 ) ) ;
#36609=CARTESIAN_POINT ( 'NONE',  ( 11.47343314416673010, 118.8698716516685465, -0.3113556051519839607 ) ) ;
#36610=CARTESIAN_POINT ( 'NONE',  ( 4.745385786424318297, 117.8992089115141226, -0.7661195729942593680 ) ) ;
#36613=CARTESIAN_POINT ( 'NONE',  ( -4.323668712555765126, 118.1588900175947856, 0.5145642005610773229 ) ) ;
#36616=CARTESIAN_POINT ( 'NONE',  ( -4.366622630093331736, 118.1827404141456128, 0.4454535902724743313 ) ) ;
#36617=CARTESIAN_POINT ( 'NONE',  ( 4.369338447829433925, 112.0483952545421857, -2.684113968122932459 ) ) ;
#36618=VERTEX_POINT ( 'NONE', #11092 ) ;
#36620=CARTESIAN_POINT ( 'NONE',  ( -6.022744270120071519, 119.3729936414536326, -1.265161215359080327 ) ) ;
#36621=CARTESIAN_POINT ( 'NONE',  ( -4.746159770738358041, 112.7696648386057632, -2.567419849205245796 ) ) ;
#36622=CARTESIAN_POINT ( 'NONE',  ( 4.467051862462757761, 118.1153619260469156, 0.7452539832175895107 ) ) ;
#36623=CARTESIAN_POINT ( 'NONE',  ( -8.365438877267290962, 122.6561726160659731, -0.7803013885889897860 ) ) ;
#36624=CARTESIAN_POINT ( 'NONE',  ( -0.8282417804140018713, 115.7028554972107059, -1.753370426095431256 ) ) ;
#36625=CARTESIAN_POINT ( 'NONE',  ( 1.626927334713244466, 117.3993836556012269, -1.397841868528616249 ) ) ;
#36626=CARTESIAN_POINT ( 'NONE',  ( 2.177262389793235720, 106.6864334246082961, -4.884315812310542348 ) ) ;
#36627=CARTESIAN_POINT ( 'NONE',  ( -10.07755082079049025, 123.5826510519420509, -1.213607387526569159 ) ) ;
#36630=CARTESIAN_POINT ( 'NONE',  ( 8.321979263998503740, 120.1320355853846991, -1.118248183737061696 ) ) ;
#36631=CARTESIAN_POINT ( 'NONE',  ( -10.39508997167191495, 153.1476119741804496, -0.08737454559994831116 ) ) ;
#36633=CARTESIAN_POINT ( 'NONE',  ( 16.47501798513116000, 155.2380866766625047, 1.211716152346587583 ) ) ;
#36634=CARTESIAN_POINT ( 'NONE',  ( -4.835467458963106147, 104.6144662015457385, 0.09735812545712563271 ) ) ;
#36635=CARTESIAN_POINT ( 'NONE',  ( 2.867866294591228993, -15.05265924143639467, 4.220695585399262484 ) ) ;
#36636=CARTESIAN_POINT ( 'NONE',  ( -4.045847121365472532, 157.1622345443605582, 1.633529996401409834 ) ) ;
#36637=CARTESIAN_POINT ( 'NONE',  ( 0.2395577018624739096, -8.716993574909102094, 0.9436776969787653568 ) ) ;
#36638=CARTESIAN_POINT ( 'NONE',  ( -22.98914810635016792, 149.5377445326608665, -1.186953142822410268 ) ) ;
#36639=CARTESIAN_POINT ( 'NONE',  ( -0.9667957141098567631, 26.69201124214932719, -0.1227653459084327853 ) ) ;
#36642=CARTESIAN_POINT ( 'NONE',  ( 7.424629525399723207, 123.6670498955208473, 0.1830506623709854119 ) ) ;
#36643=CARTESIAN_POINT ( 'NONE',  ( -12.22709855250477418, 151.9982576965888654, 0.6666368699087852345 ) ) ;
#36644=CARTESIAN_POINT ( 'NONE',  ( 4.626636300257242596, -12.70421170364453900, 2.362638098592509284 ) ) ;
#36645=CARTESIAN_POINT ( 'NONE',  ( 8.163394002857623732, 121.3802920439979118, -0.9196017894915150537 ) ) ;
#36646=VERTEX_POINT ( 'NONE', #7909 ) ;
#36647=CARTESIAN_POINT ( 'NONE',  ( -18.85674122909617978, 149.4003703399637288, -2.492295690319126678 ) ) ;
#36649=CARTESIAN_POINT ( 'NONE',  ( -4.548286217995207714, 104.6144662015457669, 1.646238831218158616 ) ) ;
#36650=CARTESIAN_POINT ( 'NONE',  ( 3.219973314159829680, -14.13069947154231620, 2.606357176882864390 ) ) ;
#36652=CARTESIAN_POINT ( 'NONE',  ( 11.18446751737354461, 128.1157469881088105, 0.03160020415517778708 ) ) ;
#36654=CARTESIAN_POINT ( 'NONE',  ( -2.353032276821629853, 107.1110135075323200, 4.697993892905302005 ) ) ;
#36655=CARTESIAN_POINT ( 'NONE',  ( 5.044654562628557493, 113.8200073110732973, 1.826596097189477907 ) ) ;
#36657=CARTESIAN_POINT ( 'NONE',  ( -5.008948584507882273, 27.92152162925472325, 0.4889012661100834434 ) ) ;
#36660=CARTESIAN_POINT ( 'NONE',  ( 11.66036501707579021, 118.7334002725740874, 0.02296568806519975331 ) ) ;
#36663=CARTESIAN_POINT ( 'NONE',  ( 1.689848471312014322, -15.51967327416042863, 5.544298522819651076 ) ) ;
#36665=CARTESIAN_POINT ( 'NONE',  ( -2.803395127021860223, 31.26063551530791074, 0.8708390753670086637 ) ) ;
#36666=CARTESIAN_POINT ( 'NONE',  ( 8.976454200711021514, 119.5326672034033777, 1.412516637748555404 ) ) ;
#36668=CARTESIAN_POINT ( 'NONE',  ( -1.630640499631123452, 19.93121390510496838, -8.274862188801900942 ) ) ;
#36669=CARTESIAN_POINT ( 'NONE',  ( 8.703198793585960047, 118.2213482221532246, -0.5883035892448743587 ) ) ;
#36670=CARTESIAN_POINT ( 'NONE',  ( -3.138057391968792409, 117.6701293611589278, -1.012097185230346197 ) ) ;
#36671=CARTESIAN_POINT ( 'NONE',  ( -5.237832120027548832, 115.7029491485453860, -1.023639123012231034 ) ) ;
#36673=CARTESIAN_POINT ( 'NONE',  ( -5.314278422745060126, 105.1224610256965235, 0.4583187270701635785 ) ) ;
#36674=CARTESIAN_POINT ( 'NONE',  ( -3.998286381996895233, 3.741657206818807424, 2.332027183294827832 ) ) ;
#36676=CARTESIAN_POINT ( 'NONE',  ( -4.966115162882106304, 115.6909491485453003, 1.258873721200368445 ) ) ;
#36677=CARTESIAN_POINT ( 'NONE',  ( 3.236250843111535769, -14.18372432684703099, 3.165927027233770286 ) ) ;
#36678=CARTESIAN_POINT ( 'NONE',  ( 0.7414234751011252733, 107.0594419416054848, -4.828671665556863779 ) ) ;
#36679=CARTESIAN_POINT ( 'NONE',  ( -6.911158149689350161, 117.5201695557886410, 0.4259063301137959723 ) ) ;
#36680=CARTESIAN_POINT ( 'NONE',  ( -5.040295590206522292, 27.95035695144725452, 0.8066306925778705672 ) ) ;
#36682=ORIENTED_EDGE ( 'NONE', *, *, #34822, .T. ) ;
#36683=CARTESIAN_POINT ( 'NONE',  ( -3.198460053303494366, 104.6144662015424416, -4.272252451844696708 ) ) ;
#36684=CARTESIAN_POINT ( 'NONE',  ( 4.909888997889673590, -15.31669448615230422, -0.4577950299049654559 ) ) ;
#36685=CARTESIAN_POINT ( 'NONE',  ( -1.222221009663208457, 118.4063602595805946, 0.6323148984906141745 ) ) ;
#36686=CARTESIAN_POINT ( 'NONE',  ( 3.745621265272091716, -10.50169880513956322, -2.708184146228840294 ) ) ;
#36688=CARTESIAN_POINT ( 'NONE',  ( 0.7595712053400294206, 120.2878791493615296, 0.5727019010319394088 ) ) ;
#36689=CARTESIAN_POINT ( 'NONE',  ( -0.8098364334002190468, 156.6562795458349910, 1.088908734543433177 ) ) ;
#36692=CARTESIAN_POINT ( 'NONE',  ( 11.83945725349111910, 123.3160021321619695, -1.255757047829673789 ) ) ;
#36694=CARTESIAN_POINT ( 'NONE',  ( -4.042996894205825420, 118.2594131075661608, -0.9467780975002213495 ) ) ;
#36695=DIRECTION ( 'NONE',  ( 4.017660918040594346E-17, -1.000000000000000000, -2.376309959284832031E-19 ) ) ;
#36696=ORIENTED_EDGE ( 'NONE', *, *, #15920, .T. ) ;
#36697=CARTESIAN_POINT ( 'NONE',  ( 4.293837942828126586, 118.2142420844534172, -0.3502869236174088741 ) ) ;
#36698=CARTESIAN_POINT ( 'NONE',  ( 0.6885929357777421655, 156.3445873232922736, -0.4144571531603682968 ) ) ;
#36700=CARTESIAN_POINT ( 'NONE',  ( 3.040187153003802933, -14.59799761600802448, -0.3075781077882258630 ) ) ;
#36704=CARTESIAN_POINT ( 'NONE',  ( 4.382351430540762927, 4.226039240006542741, -1.512498627010908647 ) ) ;
#36705=CARTESIAN_POINT ( 'NONE',  ( 3.490201360801168384, 120.2313485970928326, 0.6717870626964186354 ) ) ;
#36706=CARTESIAN_POINT ( 'NONE',  ( -2.669449998271343993, 31.09737671526713143, 0.9610299433493049159 ) ) ;
#36707=CARTESIAN_POINT ( 'NONE',  ( 4.326043401919948295, 8.289558097378858292, -1.648119079657388353 ) ) ;
#36708=CARTESIAN_POINT ( 'NONE',  ( 15.37864313207198208, 147.8292851303062321, 0.3583584359702445266 ) ) ;
#36712=CARTESIAN_POINT ( 'NONE',  ( -5.549029403653766401, 116.7532827020298072, -0.3649044722746688230 ) ) ;
#36713=CARTESIAN_POINT ( 'NONE',  ( 0.0002200197269699131770, 124.8375573595198063, -0.01101068683960091353 ) ) ;
#36718=CARTESIAN_POINT ( 'NONE',  ( 8.391957350906555035, -2.082342975431243026, 0.7039615705134369961 ) ) ;
#36719=DIRECTION ( 'NONE',  ( -0.9998004120163608288, 0.000000000000000000, -0.01997839162482749342 ) ) ;
#36723=CARTESIAN_POINT ( 'NONE',  ( -15.71820687823864304, 121.0099257824619627, 0.007297392930742367494 ) ) ;
#36726=CARTESIAN_POINT ( 'NONE',  ( 7.797685292537829049, 122.5814106518984943, -0.01624766703686477201 ) ) ;
#36728=CARTESIAN_POINT ( 'NONE',  ( -5.293395377538041124, 115.7029491485389769, -0.7213471474272098449 ) ) ;
#36729=CARTESIAN_POINT ( 'NONE',  ( -15.26129097679461921, 148.0152273645666980, -0.3559380457717281621 ) ) ;
#36730=CARTESIAN_POINT ( 'NONE',  ( 4.984919470525341012, -14.71752327621497791, 4.178560682339194976 ) ) ;
#36731=CARTESIAN_POINT ( 'NONE',  ( -12.96767020122751646, 121.2479969211051127, 1.095090382205327284 ) ) ;
#36732=CARTESIAN_POINT ( 'NONE',  ( -2.768688662514669385, 30.30441277318858440, -3.700580903672975097 ) ) ;
#36733=CARTESIAN_POINT ( 'NONE',  ( 0.3142790036445871626, 116.6413645472259617, 0.2007485675953370186 ) ) ;
#36734=CARTESIAN_POINT ( 'NONE',  ( -0.002141067027474409870, 156.3034662015459446, 0.1071477492456789499 ) ) ;
#36736=CARTESIAN_POINT ( 'NONE',  ( 0.6269268744496204748, 0.2942410971610713855, -0.7472855871245592807 ) ) ;
#36737=CARTESIAN_POINT ( 'NONE',  ( -15.99642297876449604, 121.2237126890796191, -0.5535212332769010590 ) ) ;
#36738=DIRECTION ( 'NONE',  ( -5.206863593109713661E-17, 1.000000000000000000, -1.077750396879097183E-30 ) ) ;
#36739=CARTESIAN_POINT ( 'NONE',  ( 4.973583767358946695, 117.3966162183520510, 0.9753880923065370023 ) ) ;
#36741=CARTESIAN_POINT ( 'NONE',  ( 8.737166540455065800, 117.9300049749956827, 0.7016146402485585742 ) ) ;
#36742=CARTESIAN_POINT ( 'NONE',  ( -17.96630583390862057, 147.4621342421176848, 1.576657649719084064 ) ) ;
#36745=CARTESIAN_POINT ( 'NONE',  ( 6.974227900756624798, 158.0922581832940921, 1.731937547952115519 ) ) ;
#36746=CARTESIAN_POINT ( 'NONE',  ( 19.74506706576308090, 148.5147687316951135, -1.724011100433735955 ) ) ;
#36747=CARTESIAN_POINT ( 'NONE',  ( 0.1402366131884419942, -14.11417690215759713, -0.9622292808001302600 ) ) ;
#36748=CARTESIAN_POINT ( 'NONE',  ( -7.913941031674717408, 118.5968412048868288, -1.173277403367298355 ) ) ;
#36750=CARTESIAN_POINT ( 'NONE',  ( 5.262484858994872283, 104.6144662015456959, 0.9373981974370197978 ) ) ;
#36751=ADVANCED_FACE ( 'NONE', ( #41549 ), #15540, .T. ) ;
#36753=CARTESIAN_POINT ( 'NONE',  ( 10.06202586252257980, 123.8737202207250618, -0.7052144931501600489 ) ) ;
#36754=CARTESIAN_POINT ( 'NONE',  ( 7.839459231152404506, 122.3084256158383880, 0.7153501415338812119 ) ) ;
#36756=CARTESIAN_POINT ( 'NONE',  ( -0.5061634396316659901, 119.4440140289964774, -0.5640781084940279522 ) ) ;
#36757=CARTESIAN_POINT ( 'NONE',  ( 4.902411944313367798, -15.42400938342815309, 0.6670879667284028702 ) ) ;
#36759=CARTESIAN_POINT ( 'NONE',  ( -4.384749978537653803, 118.1630025941448849, -0.6641520118282725482 ) ) ;
#36760=EDGE_CURVE ( 'NONE', #276, #39424, #23540, .T. ) ;
#36762=DIRECTION ( 'NONE',  ( 4.017660918040594346E-17, -1.000000000000000000, -2.376309959284834438E-19 ) ) ;
#36763=CARTESIAN_POINT ( 'NONE',  ( 10.71425622041610204, 122.7614441063800399, 1.568315134061841087 ) ) ;
#36765=CARTESIAN_POINT ( 'NONE',  ( 23.21373371908085304, 149.6306211361744829, 0.4638656453230914356 ) ) ;
#36766=CARTESIAN_POINT ( 'NONE',  ( 7.178138493693461797, 8.485180552427815215, -4.444891729080387321 ) ) ;
#36767=CARTESIAN_POINT ( 'NONE',  ( 9.178653662903458965, 123.9301100385560943, 0.5015510438870898202 ) ) ;
#36769=CARTESIAN_POINT ( 'NONE',  ( 19.19817178191683027, 128.6826163344482268, -0.7403421610261617936 ) ) ;
#36772=CARTESIAN_POINT ( 'NONE',  ( 0.9748426025018137597, 115.6909491485452719, 1.750969170851022216 ) ) ;
#36774=CARTESIAN_POINT ( 'NONE',  ( -5.750520748247168079, 159.1178304044242964, -0.06386070104996817431 ) ) ;
#36775=ORIENTED_EDGE ( 'NONE', *, *, #38896, .F. ) ;
#36778=CARTESIAN_POINT ( 'NONE',  ( 5.628418590827510393, 120.8807329490735043, -0.4524337895730209391 ) ) ;
#36782=CARTESIAN_POINT ( 'NONE',  ( -6.481656071630233384, 121.7133186976561205, -0.3761587846782801225 ) ) ;
#36783=CARTESIAN_POINT ( 'NONE',  ( 4.598504975971844821, -12.83055836278033901, 2.569316529143384820 ) ) ;
#36784=CARTESIAN_POINT ( 'NONE',  ( -22.19718911286656393, 149.5167998366165989, 0.9981983707184386434 ) ) ;
#36786=CARTESIAN_POINT ( 'NONE',  ( 15.52158573417665544, 120.7153972339879715, 0.3606909788719011578 ) ) ;
#36789=CARTESIAN_POINT ( 'NONE',  ( 2.551540157903699146, -0.3564265548712530207, -3.854280124997286450 ) ) ;
#36791=CARTESIAN_POINT ( 'NONE',  ( -21.90516586211597883, 151.4314113202728436, -0.4630247046772878461 ) ) ;
#36793=ORIENTED_EDGE ( 'NONE', *, *, #12262, .F. ) ;
#36794=CARTESIAN_POINT ( 'NONE',  ( -6.620801883579276570, 119.9392975627847733, 0.9773581895118412799 ) ) ;
#36795=CARTESIAN_POINT ( 'NONE',  ( 2.198398128136354934, 2.077049112184502278, 4.064154346441791965 ) ) ;
#36796=CARTESIAN_POINT ( 'NONE',  ( -0.01887972822151342753, 159.3676309965788960, 0.9448188026860502298 ) ) ;
#36799=CARTESIAN_POINT ( 'NONE',  ( 15.93384955644675038, 125.3951846505478329, -1.286024093939968305 ) ) ;
#36800=CARTESIAN_POINT ( 'NONE',  ( -4.603752034695621553, -0.9465464349810851497, 0.4006815057252178236 ) ) ;
#36801=CARTESIAN_POINT ( 'NONE',  ( -12.91997107708633052, 119.9671592456446803, -1.126112081325366443 ) ) ;
#36802=CIRCLE ( 'NONE', #21794, 0.5080000000000002292 ) ;
#36805=CARTESIAN_POINT ( 'NONE',  ( -7.846345427436888897, 154.6110463214094182, 0.1182179892959123735 ) ) ;
#36806=CARTESIAN_POINT ( 'NONE',  ( 2.663097075550662662, -15.49037753074605739, 5.782289944512356783 ) ) ;
#36809=CARTESIAN_POINT ( 'NONE',  ( -0.3873250690985411970, 117.3993820573415974, -1.495214769458282245 ) ) ;
#36811=CARTESIAN_POINT ( 'NONE',  ( 16.83022555070501625, 151.2926467857828072, 2.419188160499603057 ) ) ;
#36812=CARTESIAN_POINT ( 'NONE',  ( 4.850929972935443146, 117.7610086971114356, 0.9074237114610381738 ) ) ;
#36814=CARTESIAN_POINT ( 'NONE',  ( -5.868821994818715027, 117.5931221156369730, 0.5844160582045567764 ) ) ;
#36815=CARTESIAN_POINT ( 'NONE',  ( 3.644365486686961919, 11.68381519529092216, 7.647779612420950279 ) ) ;
#36816=CARTESIAN_POINT ( 'NONE',  ( 16.31317273256060574, 147.4903123243063590, 1.598834895054539240 ) ) ;
#36818=CARTESIAN_POINT ( 'NONE',  ( 16.70010949199478034, 122.7093839631038463, -0.3053630257279364435 ) ) ;
#36819=CARTESIAN_POINT ( 'NONE',  ( -6.527452395418614125E-14, 72.48346620154573827, -8.020333044904917549E-18 ) ) ;
#36825=CARTESIAN_POINT ( 'NONE',  ( -4.601694216786480496, 118.0766578999420204, 0.5256003764881748141 ) ) ;
#36826=CARTESIAN_POINT ( 'NONE',  ( 1.506052270138783067, 106.1074135845622379, -5.119289084907052256 ) ) ;
#36827=B_SPLINE_SURFACE_WITH_KNOTS ( 'NONE', 1, 3, ( 
 ( #14489, #30684, #1322, #36891, #26869, #27502, #33903, #24085, #40510, #36676, #33273, #39877, #10674, #14279 ),
 ( #4102, #11097, #11304, #27080, #20457, #24289, #37294, #24492, #40088, #20878, #7913, #7709, #27289, #33486 ) ),
 .UNSPECIFIED., .F., .F., .F.,
 ( 2, 2 ),
 ( 4, 3, 2, 2, 3, 4 ),
 ( 0.000000000000000000, 1.000000000000000000 ),
 ( -0.01000000000000000021, 0.000000000000000000, 0.2500000000000000000, 0.5000000000000000000, 1.000000000000000000, 1.016440741388755287 ),
 .UNSPECIFIED. ) ;
#36828=ORIENTED_EDGE ( 'NONE', *, *, #15270, .T. ) ;
#36830=CARTESIAN_POINT ( 'NONE',  ( 3.722225234581910236, 118.8509950637502754, -0.7881369688021256925 ) ) ;
#36831=CARTESIAN_POINT ( 'NONE',  ( -5.928176885185754585, 118.9717589635377664, -0.5867527899620111898 ) ) ;
#36832=AXIS2_PLACEMENT_3D ( 'NONE', #17407, #34037, #17612 ) ;
#36833=CARTESIAN_POINT ( 'NONE',  ( 4.458613046552058812, 118.1301588028213985, 0.7148097977274291415 ) ) ;
#36834=CARTESIAN_POINT ( 'NONE',  ( -8.219871311007542758, 154.6505398758502849, -1.119353551822956927 ) ) ;
#36835=DIRECTION ( 'NONE',  ( -4.017660918040594346E-17, 1.000000000000000000, 2.376309959284834438E-19 ) ) ;
#36836=CARTESIAN_POINT ( 'NONE',  ( 0.5670302775938013129, 118.1651003848106996, -0.8699756239007430114 ) ) ;
#36837=CARTESIAN_POINT ( 'NONE',  ( 5.120189775498607432, 114.3381464724725447, -1.761508159713760735 ) ) ;
#36838=CARTESIAN_POINT ( 'NONE',  ( -11.23392777908764550, 153.2158294759273360, -1.564101052410651116 ) ) ;
#36839=CARTESIAN_POINT ( 'NONE',  ( 4.530977940126489578, 116.0444662015457595, 3.792717828883179543 ) ) ;
#36841=CARTESIAN_POINT ( 'NONE',  ( 7.920006352636749902, 122.0419191725283099, -0.5993308652498051670 ) ) ;
#36842=CARTESIAN_POINT ( 'NONE',  ( -7.772909586817207561, 154.6794531666453167, -0.04377667875137248449 ) ) ;
#36844=DIRECTION ( 'NONE',  ( -0.9998004120163608288, 0.000000000000000000, -0.01997839162482747608 ) ) ;
#36845=CARTESIAN_POINT ( 'NONE',  ( 0.3355986945387293696, 116.9201722098172382, 0.3169108175686568551 ) ) ;
#36847=CARTESIAN_POINT ( 'NONE',  ( 3.252851485128089415, -14.73889851401814788, 2.797586445667359811 ) ) ;
#36848=CARTESIAN_POINT ( 'NONE',  ( -0.01111639999524573208, 119.1634951276629550, 0.5563101126475828995 ) ) ;
#36850=CARTESIAN_POINT ( 'NONE',  ( -0.9711860326002300647, -2.018343210913434493, -0.07513956953184577903 ) ) ;
#36851=CARTESIAN_POINT ( 'NONE',  ( -10.56633813141753286, 157.9214973357695158, -0.8874509626871485146 ) ) ;
#36853=CARTESIAN_POINT ( 'NONE',  ( -0.7929698604315037480, -4.880942799695234591, 0.5714185140920283734 ) ) ;
#36856=CARTESIAN_POINT ( 'NONE',  ( 6.287821989302472048, 120.0808430858776887, 0.4528678087849543066 ) ) ;
#36858=CARTESIAN_POINT ( 'NONE',  ( -7.681492011331976677, 122.2986020547093915, 0.2830363146464230928 ) ) ;
#36859=CARTESIAN_POINT ( 'NONE',  ( 4.664530445857379526, -12.43571634592606578, 1.922475882534872449 ) ) ;
#36860=CARTESIAN_POINT ( 'NONE',  ( 16.72891957527388485, 148.5304741467402323, -1.365449702224203810 ) ) ;
#36861=ORIENTED_EDGE ( 'NONE', *, *, #36760, .F. ) ;
#36863=CARTESIAN_POINT ( 'NONE',  ( -10.89600635431589382, 121.6366708983051836, -1.687201357748379094 ) ) ;
#36864=CARTESIAN_POINT ( 'NONE',  ( 3.627172221952804865, 115.7029588638002480, 1.619983893740152059 ) ) ;
#36865=AXIS2_PLACEMENT_3D ( 'NONE', #17731, #21337, #40137 ) ;
#36866=CARTESIAN_POINT ( 'NONE',  ( 3.131463087139035206, -14.49961247625831895, 3.567833873788547550 ) ) ;
#36867=CARTESIAN_POINT ( 'NONE',  ( -4.748912967724773004, 117.5371765964522126, -1.178473615865876400 ) ) ;
#36868=CARTESIAN_POINT ( 'NONE',  ( 0.001255909994464627982, 120.9722815239556439, -0.06285087176068919479 ) ) ;
#36870=CARTESIAN_POINT ( 'NONE',  ( -4.875672548457829159, 115.9539541688493642, 1.177672081078976252 ) ) ;
#36871=CARTESIAN_POINT ( 'NONE',  ( 5.078986093043053707, 94.32746620154571815, 0.1014902294541237954 ) ) ;
#36873=CARTESIAN_POINT ( 'NONE',  ( -2.613900097597573247, 28.43811729901509722, 0.3641677077667250795 ) ) ;
#36875=CARTESIAN_POINT ( 'NONE',  ( 18.61428830734542217, 154.1511370093759865, 0.1565858633853993154 ) ) ;
#36877=CARTESIAN_POINT ( 'NONE',  ( 1.866554170971439275, -15.20651402204141434, 5.950605956638611360 ) ) ;
#36879=CARTESIAN_POINT ( 'NONE',  ( -3.148634455474565108, 30.89457961443325118, -0.4672107454865901954 ) ) ;
#36880=CARTESIAN_POINT ( 'NONE',  ( 6.672308397275171110, 157.8130281244853279, 1.874701415657104464 ) ) ;
#36882=CARTESIAN_POINT ( 'NONE',  ( -4.342437030201590886, 23.60747082334219371, 7.218840658967335067 ) ) ;
#36883=CARTESIAN_POINT ( 'NONE',  ( 8.715377116203347541, 118.1578518853687427, -0.5461487580537397468 ) ) ;
#36884=CARTESIAN_POINT ( 'NONE',  ( -2.726848673931784539, 121.4869043954268903, -0.3408589522888660905 ) ) ;
#36887=CARTESIAN_POINT ( 'NONE',  ( -0.009645608629898889952, 120.9711055683165597, 0.4827056984856005761 ) ) ;
#36889=CARTESIAN_POINT ( 'NONE',  ( -4.609222696788063622, 3.091975128091568159, 0.4746723485708761459 ) ) ;
#36891=CARTESIAN_POINT ( 'NONE',  ( -5.276425599434917402, 115.6909491485453003, 0.8138454675775167457 ) ) ;
#36892=CARTESIAN_POINT ( 'NONE',  ( 3.259676495098780880, -13.96886708669151034, 2.676229364769742158 ) ) ;
#36893=CARTESIAN_POINT ( 'NONE',  ( 5.433597316833147062, 122.7706071131974994, -0.004560450986766740981 ) ) ;
#36894=CARTESIAN_POINT ( 'NONE',  ( -22.30840772692687324, 150.5193240506149550, 0.5167903241875736464 ) ) ;
#36895=CARTESIAN_POINT ( 'NONE',  ( 0.9857937726801648815, 36.25851983645378596, 2.381811577489552523 ) ) ;
#36898=CARTESIAN_POINT ( 'NONE',  ( 4.438132741721911856, -15.66483130081081043, 3.040968155030625120 ) ) ;
#36899=CARTESIAN_POINT ( 'NONE',  ( -6.741493414765860948, 119.3011930948910759, 1.016225879973854829 ) ) ;
#36900=EDGE_CURVE ( 'NONE', #24401, #5382, #29763, .T. ) ;
#36901=CARTESIAN_POINT ( 'NONE',  ( 0.7259983000635549244, 26.63096242550804860, 0.6518668477890779966 ) ) ;
#36902=ORIENTED_EDGE ( 'NONE', *, *, #34822, .F. ) ;
#36903=CARTESIAN_POINT ( 'NONE',  ( -3.983954973735330363, 31.42523109854115049, -0.6611907497737663508 ) ) ;
#36904=CARTESIAN_POINT ( 'NONE',  ( 2.327868625978029016, 124.9344662015457175, 0.04651635516647365659 ) ) ;
#36905=CARTESIAN_POINT ( 'NONE',  ( -15.52878352361693004, 139.6011575924185877, 1.142358493343924364 ) ) ;
#36906=CARTESIAN_POINT ( 'NONE',  ( -3.682264917456322895, 63.33946620154573282, -0.07358041635423923088 ) ) ;
#36908=CARTESIAN_POINT ( 'NONE',  ( 16.36721571005495690, 151.0861551944122141, -1.708847769304776110 ) ) ;
#36909=CARTESIAN_POINT ( 'NONE',  ( 0.03067001211929198945, 158.6015251912307633, -1.534852821454057770 ) ) ;
#36911=CARTESIAN_POINT ( 'NONE',  ( 4.170329027945798295, 118.2393515795533148, -0.2194353840718009652 ) ) ;
#36912=CARTESIAN_POINT ( 'NONE',  ( 0.7006168245643282777, 156.3636429644085695, -0.4970284052464095104 ) ) ;
#36914=CARTESIAN_POINT ( 'NONE',  ( 2.463764682325012778, -15.17880951736275108, 4.811303307383569816 ) ) ;
#36918=CARTESIAN_POINT ( 'NONE',  ( 1.748379858460863856, 5.525481214791113871, -4.283037568778763848 ) ) ;
#36919=CARTESIAN_POINT ( 'NONE',  ( 10.21894633145440245, 123.0849000269954701, 1.386333990434162944 ) ) ;
#36920=CARTESIAN_POINT ( 'NONE',  ( 2.383981540283352629, 36.81846344528510429, 1.803752045214196853 ) ) ;
#36921=CARTESIAN_POINT ( 'NONE',  ( -7.070147686296687439, 122.4340714744230496, -0.03157745743911240244 ) ) ;
#36922=CARTESIAN_POINT ( 'NONE',  ( 2.584458374606236841, 15.83607344512877368, 3.832284875798456447 ) ) ;
#36923=CARTESIAN_POINT ( 'NONE',  ( 3.750075860242078729, 121.0949217282140182, 0.1016972523499030667 ) ) ;
#36924=CARTESIAN_POINT ( 'NONE',  ( -1.424374813699339715, 106.0672060291940539, 5.142970079757129831 ) ) ;
#36925=CIRCLE ( 'NONE', #13780, 5.080000000000006288 ) ;
#36927=CARTESIAN_POINT ( 'NONE',  ( 5.560045425373370875, 116.7476357771200242, -0.1303784914585657262 ) ) ;
#36930=CARTESIAN_POINT ( 'NONE',  ( -0.6790824029981872290, 105.9268256211374393, 5.296885899767392658 ) ) ;
#36932=CARTESIAN_POINT ( 'NONE',  ( -3.848622047617309860, 1.169161361801722032, -7.524129562738414378 ) ) ;
#36937=CARTESIAN_POINT ( 'NONE',  ( -15.92845220574659315, 121.2232988859741027, 0.005268350931750771793 ) ) ;
#36940=CARTESIAN_POINT ( 'NONE',  ( -6.068413118431933206, 121.4395679076997823, -0.1212613395058407956 ) ) ;
#36943=CARTESIAN_POINT ( 'NONE',  ( -8.948282891152253171, 123.9641325482187426, -0.1345489399228556593 ) ) ;
#36944=CARTESIAN_POINT ( 'NONE',  ( 4.535621022044703743, -15.16026073378742822, 4.605481170969206062 ) ) ;
#36945=CARTESIAN_POINT ( 'NONE',  ( -11.66006228966227454, 156.3395478113760362, 1.582478695429108351 ) ) ;
#36947=CARTESIAN_POINT ( 'NONE',  ( 15.37635245578016630, 120.8297411738997624, 0.7275678838439408880 ) ) ;
#36948=CARTESIAN_POINT ( 'NONE',  ( 15.77809098948537780, 146.2329395987594012, 0.5167778558810404155 ) ) ;
#36950=B_SPLINE_CURVE_WITH_KNOTS ( 'NONE', 3,
 ( #30017, #23611, #34069, #4896, #24449, #857 ),
 .UNSPECIFIED., .F., .F.,
 ( 4, 2, 4 ),
 ( 0.000000000000000000, 0.1265415849040014140, 0.2530831698080028280 ),
 .UNSPECIFIED. ) ;
#36951=CARTESIAN_POINT ( 'NONE',  ( -15.55067499035036604, 120.8127473925414108, -0.5415919938617848040 ) ) ;
#36953=VERTEX_POINT ( 'NONE', #6039 ) ;
#36954=CARTESIAN_POINT ( 'NONE',  ( -5.559546751422816513, 116.7637306756996338, 0.1380498186195938948 ) ) ;
#36955=CARTESIAN_POINT ( 'NONE',  ( -0.02969003158485089208, 157.1787724364823760, 1.485810588193620552 ) ) ;
#36957=CARTESIAN_POINT ( 'NONE',  ( 0.01152893261307403987, 118.7114655739656257, -0.5769549317675699562 ) ) ;
#36958=CARTESIAN_POINT ( 'NONE',  ( -0.8939936458071766623, -10.86866097718376523, 0.3889025406916932770 ) ) ;
#36959=CARTESIAN_POINT ( 'NONE',  ( 0.02615207601215727498, 159.0391464308674756, -1.308756824028193044 ) ) ;
#36962=VECTOR ( 'NONE', #13807, 1000.000000000000227 ) ;
#36963=FACE_OUTER_BOUND ( 'NONE', #30398, .T. ) ;
#36964=CARTESIAN_POINT ( 'NONE',  ( 11.28744401931954577, 153.2158294759273360, -1.114070445992415781 ) ) ;
#36965=CARTESIAN_POINT ( 'NONE',  ( -0.6412933796113865492, 156.3034662015457741, -0.01281456791805602943 ) ) ;
#36966=ORIENTED_EDGE ( 'NONE', *, *, #22254, .T. ) ;
#36967=CARTESIAN_POINT ( 'NONE',  ( -11.51381720411944620, 123.3156264706956478, -1.674137098916062438 ) ) ;
#36968=CARTESIAN_POINT ( 'NONE',  ( 4.580902669819289841, -15.62468711146633460, 2.622166941725792899 ) ) ;
#36970=CARTESIAN_POINT ( 'NONE',  ( -4.388233089188608105, 118.1817579657902542, -0.5768122195966850496 ) ) ;
#36973=CARTESIAN_POINT ( 'NONE',  ( 12.17039870458260076, 124.2599011343719155, 1.750469281869919014 ) ) ;
#36975=AXIS2_PLACEMENT_3D ( 'NONE', #39134, #35944, #32107 ) ;
#36976=CARTESIAN_POINT ( 'NONE',  ( 15.56076557482319700, 120.7233670659379214, 0.3109411287488704767 ) ) ;
#36977=CARTESIAN_POINT ( 'NONE',  ( -4.930748812479134990, 13.88268055242722987, 6.853499169485068876 ) ) ;
#36978=CARTESIAN_POINT ( 'NONE',  ( 9.378755113003604649, 124.2036136473707018, 0.5113998741172594009 ) ) ;
#36979=AXIS2_PLACEMENT_3D ( 'NONE', #31446, #34653, #30813 ) ;
#36980=CARTESIAN_POINT ( 'NONE',  ( 20.14555658732719934, 152.4688535085772685, -0.7444337660854590810 ) ) ;
#36981=DIRECTION ( 'NONE',  ( 0.08575086330566537851, 4.464930482241040583E-18, 0.9963166110440663248 ) ) ;
#36982=CARTESIAN_POINT ( 'NONE',  ( 0.3689803932068112524, 115.6909491485452719, 1.766244566112858738 ) ) ;
#36985=CARTESIAN_POINT ( 'NONE',  ( -23.43370484584250590, 146.8275480241000253, -0.3132885061830181783 ) ) ;
#36988=CARTESIAN_POINT ( 'NONE',  ( -7.868921389075623551, 122.1502739528543771, -0.8431891051951234672 ) ) ;
#36989=PLANE ( 'NONE',  #30534 ) ;
#36990=CARTESIAN_POINT ( 'NONE',  ( -4.757248700628498916, 117.4032733054477973, -1.206458840162573543 ) ) ;
#36991=CARTESIAN_POINT ( 'NONE',  ( -14.33905310436375480, 139.0340687859245463, -0.7442083991839666401 ) ) ;
#36992=CARTESIAN_POINT ( 'NONE',  ( 4.995837928452414367, -12.01622098921958859, 1.211524600846092481 ) ) ;
#36993=CARTESIAN_POINT ( 'NONE',  ( -21.01108318401078279, 151.1643092826112138, 1.006483555388256290 ) ) ;
#36995=CARTESIAN_POINT ( 'NONE',  ( 16.14716650825965161, 121.2501203052637493, 0.3739013473229990669 ) ) ;
#36998=CARTESIAN_POINT ( 'NONE',  ( 0.7336086519982951692, 0.2932837538699786251, -4.563195415240439701 ) ) ;
#37000=CARTESIAN_POINT ( 'NONE',  ( -2.735903701988665393, 116.5290148844309357, -0.06805092059891044987 ) ) ;
#37003=VERTEX_POINT ( 'NONE', #16432 ) ;
#37004=CARTESIAN_POINT ( 'NONE',  ( -6.655208740269098477, 120.0178561674164115, 0.9687501452866643659 ) ) ;
#37005=CARTESIAN_POINT ( 'NONE',  ( -4.027482788729651375, -0.2968512080594384317, 2.264360808822050597 ) ) ;
#37006=CARTESIAN_POINT ( 'NONE',  ( 22.29769713523675634, 148.9358926463403918, 1.890714429241201922 ) ) ;
#37008=CARTESIAN_POINT ( 'NONE',  ( 13.89335097268673280, 122.2371923977168109, -1.173247377384143642 ) ) ;
#37010=CARTESIAN_POINT ( 'NONE',  ( -4.627572956979934204, -1.171460759993483647, -0.2796867628226345492 ) ) ;
#37011=CARTESIAN_POINT ( 'NONE',  ( -19.95201466422913228, 152.4248492066682559, -1.669502467017324632 ) ) ;
#37013=CARTESIAN_POINT ( 'NONE',  ( -4.566879893416770031, 121.1702857069421100, 0.02052890071062577274 ) ) ;
#37015=CARTESIAN_POINT ( 'NONE',  ( 2.110383923269381512, -15.54165552008020335, 5.912460941884730481 ) ) ;
#37016=( BOUNDED_CURVE ( )  B_SPLINE_CURVE ( 3, ( #38126, #9357, #35560, #29366 ),
 .UNSPECIFIED., .F., .T. ) 
 B_SPLINE_CURVE_WITH_KNOTS ( ( 4, 4 ),
 ( 0.0001874388305180640468, 0.2498838476046065793 ),
 .UNSPECIFIED. ) 
 CURVE ( )  GEOMETRIC_REPRESENTATION_ITEM ( )  RATIONAL_B_SPLINE_CURVE ( ( 0.9999925516704997186, 0.6670664864091201407, 0.5004025452935453311, 0.5000007283237750677 ) ) 
 REPRESENTATION_ITEM ( '' )  );
#37019=CARTESIAN_POINT ( 'NONE',  ( -0.4922460975656830495, 117.3993826272291869, -1.493757915153530735 ) ) ;
#37021=CARTESIAN_POINT ( 'NONE',  ( 18.97908907040207538, 145.0145856610025987, 2.515253529532921917 ) ) ;
#37025=CARTESIAN_POINT ( 'NONE',  ( -3.102616959202407099, 159.2904672602661549, 0.8345756338990469869 ) ) ;
#37026=CARTESIAN_POINT ( 'NONE',  ( 8.086262078954034038, 3.373778641329666872, 2.357548046588672008 ) ) ;
#37028=CARTESIAN_POINT ( 'NONE',  ( 9.985636026282364242, 124.1433363813624311, 1.001463123883985729 ) ) ;
#37030=CARTESIAN_POINT ( 'NONE',  ( 14.51632629332712909, 120.3567457872619997, -0.2133257594814960689 ) ) ;
#37035=CARTESIAN_POINT ( 'NONE',  ( -4.170396868163473769, 118.2393519985668746, 0.2194165179955171185 ) ) ;
#37036=CARTESIAN_POINT ( 'NONE',  ( -5.078986093043186045, 88.48546620154573361, -0.1014902294541231709 ) ) ;
#37039=CARTESIAN_POINT ( 'NONE',  ( 8.289722630716616081, 120.2889166620582131, -1.113928890953434170 ) ) ;
#37040=CARTESIAN_POINT ( 'NONE',  ( -5.608813212978156493, 117.9149360781225937, -0.7492264055198124550 ) ) ;
#37041=CARTESIAN_POINT ( 'NONE',  ( 4.155982282308561260, 118.2394341885533038, 0.3882798843181367032 ) ) ;
#37042=CARTESIAN_POINT ( 'NONE',  ( -16.16038979459568381, 146.4165046419237228, -1.293905914731260598 ) ) ;
#37044=CARTESIAN_POINT ( 'NONE',  ( 4.425820884885741435, 117.3993836135481530, -1.092143121358476687 ) ) ;
#37047=CARTESIAN_POINT ( 'NONE',  ( 5.292163649236448109, 116.0761519159950552, -1.031159682278862233 ) ) ;
#37048=CARTESIAN_POINT ( 'NONE',  ( -4.757797086070440606, 156.0326374431741385, -1.238355579604159873 ) ) ;
#37052=CARTESIAN_POINT ( 'NONE',  ( 7.784012322544599627, 122.6313477034872506, 0.1555430911242069170 ) ) ;
#37053=DIRECTION ( 'NONE',  ( 4.017660918040594346E-17, -1.000000000000000000, -2.376309959284834438E-19 ) ) ;
#37054=CARTESIAN_POINT ( 'NONE',  ( 15.49230080900811402, 121.3130774642648220, 1.004719031932798767 ) ) ;
#37056=CARTESIAN_POINT ( 'NONE',  ( 3.208040786519721355, -14.49217647381938257, 1.686337311097440894 ) ) ;
#37057=CARTESIAN_POINT ( 'NONE',  ( -2.342076541036599124, 157.5529522918930638, 1.611985001046909005 ) ) ;
#37058=CARTESIAN_POINT ( 'NONE',  ( 0.7944722411588411859, -7.641519016208866866, 0.5639076281424253434 ) ) ;
#37059=CARTESIAN_POINT ( 'NONE',  ( -7.903286925170654342, 158.6683511845044734, -0.6884992853041225214 ) ) ;
#37060=CARTESIAN_POINT ( 'NONE',  ( -0.9746272421432693456, 17.39786500698104277, 0.06925455797152506310 ) ) ;
#37061=ORIENTED_EDGE ( 'NONE', *, *, #28462, .T. ) ;
#37065=CARTESIAN_POINT ( 'NONE',  ( -2.740744172220349384, 120.7841308545065431, 0.2151145298216796120 ) ) ;
#37066=CARTESIAN_POINT ( 'NONE',  ( 4.431203275146504694, -13.68733396499126265, 3.949578922469492603 ) ) ;
#37067=CARTESIAN_POINT ( 'NONE',  ( 8.085704850285637235, 121.5393406094847819, -0.8545391641419386453 ) ) ;
#37069=CARTESIAN_POINT ( 'NONE',  ( -3.347088983278076579, 104.6144662015457811, 3.489637925767542725 ) ) ;
#37070=CARTESIAN_POINT ( 'NONE',  ( 3.347306494706169477, -13.94864326390300668, 3.303819676456750898 ) ) ;
#37071=CARTESIAN_POINT ( 'NONE',  ( -4.957019470562856078, 117.4692298950752161, -0.9989214207450358707 ) ) ;
#37072=CARTESIAN_POINT ( 'NONE',  ( 15.79259660498968643, 146.2429432508320417, 0.1870566092231163435 ) ) ;
#37074=CARTESIAN_POINT ( 'NONE',  ( 20.22999339756068693, 148.7458375694471044, 2.474301912364148315 ) ) ;
#37075=CARTESIAN_POINT ( 'NONE',  ( 1.300340531814593081, 106.1074135845529582, 5.175367491933112518 ) ) ;
#37076=CARTESIAN_POINT ( 'NONE',  ( -5.180755175387888656, 27.96082930289568935, 0.4723356417371947225 ) ) ;
#37078=CARTESIAN_POINT ( 'NONE',  ( 23.09707919911549467, 149.8924475812327159, 0.2317116236470735946 ) ) ;
#37079=EDGE_CURVE ( 'NONE', #19701, #929, #39541, .T. ) ;
#37082=CARTESIAN_POINT ( 'NONE',  ( 1.759694577103611213, -15.65007286489543326, 5.607714211663698656 ) ) ;
#37083=DIRECTION ( 'NONE',  ( -0.9998004120163609398, 0.000000000000000000, -0.01997839162482749689 ) ) ;
#37084=CARTESIAN_POINT ( 'NONE',  ( -4.980269422504584043, 117.5911954193708908, -0.7465893992053445061 ) ) ;
#37085=CARTESIAN_POINT ( 'NONE',  ( 20.51324802173755657, 148.8605967840894095, 2.436527653975322227 ) ) ;
#37087=CARTESIAN_POINT ( 'NONE',  ( 2.510961470319720501, 15.29743382693132148, 8.092466016612050339 ) ) ;
#37088=CARTESIAN_POINT ( 'NONE',  ( -8.586090317502511837, 118.6238329966567306, -1.141930902790657898 ) ) ;
#37089=CARTESIAN_POINT ( 'NONE',  ( -3.197921176416423261, 118.4615047536228047, -0.7906167528392610278 ) ) ;
#37090=CARTESIAN_POINT ( 'NONE',  ( 4.973153598853037316, 117.3993852231080268, 0.9753024529967266876 ) ) ;
#37091=CARTESIAN_POINT ( 'NONE',  ( -4.724244202807499349, 117.6625551699878827, -1.131988795082268240 ) ) ;
#37092=CARTESIAN_POINT ( 'NONE',  ( -4.572702043008527895, 104.6144662015325224, 2.768430063960745979 ) ) ;
#37093=CARTESIAN_POINT ( 'NONE',  ( -4.157303687089163979, 2.242350289152962528, -2.029258473605290103 ) ) ;
#37095=FACE_OUTER_BOUND ( 'NONE', #18400, .T. ) ;
#37096=CARTESIAN_POINT ( 'NONE',  ( 3.188489192988832155, -14.31930622237681483, 3.473944028487384372 ) ) ;
#37097=CARTESIAN_POINT ( 'NONE',  ( 4.210090452738473488, 118.4033805524614849, -0.5735154781215827668 ) ) ;
#37099=CARTESIAN_POINT ( 'NONE',  ( 1.928079173006373104, 38.28172739177303896, 1.429945915702467651 ) ) ;
#37101=ORIENTED_EDGE ( 'NONE', *, *, #31623, .T. ) ;
#37102=CARTESIAN_POINT ( 'NONE',  ( -5.344453801630723255, 105.1225221600350466, 0.1077189844379473072 ) ) ;
#37103=CARTESIAN_POINT ( 'NONE',  ( 4.930802857217395641, -15.55747185075553851, 2.516589264972601825 ) ) ;
#37104=CARTESIAN_POINT ( 'NONE',  ( -4.459427130834483499, 157.7533977378147654, 1.670975814381038926 ) ) ;
#37105=CARTESIAN_POINT ( 'NONE',  ( -0.6497956273327881727, 21.66276798020532013, -0.7290388503713802759 ) ) ;
#37108=CARTESIAN_POINT ( 'NONE',  ( 0.007549346801170758389, 106.0530876078258586, 5.266739608401566741 ) ) ;
#37109=CARTESIAN_POINT ( 'NONE',  ( -10.28583081752403139, 123.7737839053064022, 0.8195368008302437168 ) ) ;
#37111=CARTESIAN_POINT ( 'NONE',  ( 17.99030040960589005, 148.1388135707062474, -1.617688361210429582 ) ) ;
#37112=CARTESIAN_POINT ( 'NONE',  ( -13.20682171306295238, 121.8780043825237982, -1.728041046422398086 ) ) ;
#37113=FACE_OUTER_BOUND ( 'NONE', #21028, .T. ) ;
#37114=CARTESIAN_POINT ( 'NONE',  ( 4.246255474397634622, 118.2246697035938752, -0.3144686129305331868 ) ) ;
#37115=CARTESIAN_POINT ( 'NONE',  ( 9.260187833317498729, 153.8817031120973411, -0.3320757922997037426 ) ) ;
#37118=CARTESIAN_POINT ( 'NONE',  ( 3.044219152853963717, -14.30162947539197127, 0.8262259773895895831 ) ) ;
#37121=CARTESIAN_POINT ( 'NONE',  ( -1.146732334619779969, -3.095543821355960734, -4.488006035213349953 ) ) ;
#37122=CARTESIAN_POINT ( 'NONE',  ( 1.917342111448682607, 156.7095495334699535, 1.310369884728257217 ) ) ;
#37123=CARTESIAN_POINT ( 'NONE',  ( -0.01131193556908014278, 32.98573834278982986, 2.219894021788903160 ) ) ;
#37124=CARTESIAN_POINT ( 'NONE',  ( -4.405468973772928010, 113.1344509532474376, 2.291157639236350185 ) ) ;
#37126=CARTESIAN_POINT ( 'NONE',  ( -4.151662239014343392, 13.23730288530712862, 2.070234887608822572 ) ) ;
#37127=CARTESIAN_POINT ( 'NONE',  ( 10.40832821182515033, 153.0987333575537548, 0.3246753324606913016 ) ) ;
#37131=CARTESIAN_POINT ( 'NONE',  ( -8.783221293945311814, 117.7336977213016382, -0.4113777022403178329 ) ) ;
#37134=CARTESIAN_POINT ( 'NONE',  ( 1.896617635523347944, -15.61750365820154407, 5.464805439086086736 ) ) ;
#37136=CARTESIAN_POINT ( 'NONE',  ( -2.691543149356179665, 0.9405793051805824145, -7.980626778548312927 ) ) ;
#37138=DIRECTION ( 'NONE',  ( -0.9998004118909472604, 1.039228058384960363E-20, -0.01997839790104462970 ) ) ;
#37140=CARTESIAN_POINT ( 'NONE',  ( -5.010144981628188887, 117.3993855238222608, -0.7522679339500687457 ) ) ;
#37141=CARTESIAN_POINT ( 'NONE',  ( -23.20995092461745202, 148.9919839608952827, 0.1323997120335726196 ) ) ;
#37142=ORIENTED_EDGE ( 'NONE', *, *, #25382, .F. ) ;
#37146=CARTESIAN_POINT ( 'NONE',  ( -15.38000172822634326, 147.8312228277220868, -0.3073290368998167210 ) ) ;
#37147=CARTESIAN_POINT ( 'NONE',  ( 6.371418708240476292, -13.42079056852439578, 0.8326245159988630018 ) ) ;
#37148=CARTESIAN_POINT ( 'NONE',  ( -4.057542840006509444, 118.1249481555716301, 0.7600096289331684796 ) ) ;
#37149=CARTESIAN_POINT ( 'NONE',  ( 11.13388036866224873, 119.2389763063149388, -0.6860836662663821750 ) ) ;
#37151=CARTESIAN_POINT ( 'NONE',  ( -8.041834545247111166, 158.6767594643193604, -0.3248513814034965641 ) ) ;
#37153=ORIENTED_EDGE ( 'NONE', *, *, #26154, .T. ) ;
#37155=CARTESIAN_POINT ( 'NONE',  ( 5.559147133327456025, 116.7105361058337252, 0.2236709051713111351 ) ) ;
#37156=CARTESIAN_POINT ( 'NONE',  ( -7.347594966877752043, 120.9764928074160082, 0.8683198564056586743 ) ) ;
#37158=CARTESIAN_POINT ( 'NONE',  ( 2.466025220844119126, 157.8629595415303584, -1.630325060746250498 ) ) ;
#37159=CARTESIAN_POINT ( 'NONE',  ( 0.8685042297821888857, -7.415843212509670934, 0.4410767154842855642 ) ) ;
#37160=CARTESIAN_POINT ( 'NONE',  ( -1.224709079186641514, 159.1407128229522527, -1.247756218451904209 ) ) ;
#37162=CARTESIAN_POINT ( 'NONE',  ( 15.62653493684484651, 149.1167355181319181, -1.114087811593069688 ) ) ;
#37163=CARTESIAN_POINT ( 'NONE',  ( -6.439802323014594534E-14, 156.3034662015457172, 9.765829976239106842E-17 ) ) ;
#37164=B_SPLINE_CURVE_WITH_KNOTS ( 'NONE', 5,
 ( #41670, #31006, #18424, #25254, #18852, #9076 ),
 .UNSPECIFIED., .F., .F.,
 ( 6, 6 ),
 ( 0.000000000000000000, 0.2175306174020106287 ),
 .UNSPECIFIED. ) ;
#37166=CARTESIAN_POINT ( 'NONE',  ( -17.12878219156706905, 140.2562023718666353, -2.330665938063504417 ) ) ;
#37167=CARTESIAN_POINT ( 'NONE',  ( 4.104683988343100332, -15.63859574289259946, 3.129333468668611840 ) ) ;
#37168=PLANE ( 'NONE',  #27191 ) ;
#37169=CARTESIAN_POINT ( 'NONE',  ( -4.274993567701977248, 118.2142329864754799, -0.5231303911420034369 ) ) ;
#37171=CARTESIAN_POINT ( 'NONE',  ( -4.932986805861466095, 117.5466154476640952, 0.8856657162804417727 ) ) ;
#37172=CARTESIAN_POINT ( 'NONE',  ( 3.791208754741518305, 156.9018388488748883, 1.699278904607349094 ) ) ;
#37174=CARTESIAN_POINT ( 'NONE',  ( 22.53527615164620101, 150.7831677823008363, 0.4503084484864737225 ) ) ;
#37176=CARTESIAN_POINT ( 'NONE',  ( 8.243228241119590294, 17.55835651096333194, -1.765626013165721320 ) ) ;
#37177=CARTESIAN_POINT ( 'NONE',  ( 15.85571122620632245, 146.2799285973741519, 0.7709397856434243579 ) ) ;
#37179=AXIS2_PLACEMENT_3D ( 'NONE', #33308, #17098, #7120 ) ;
#37183=CARTESIAN_POINT ( 'NONE',  ( -4.735783051744410166, 116.7698466342620378, -0.01422048256815223663 ) ) ;
#37186=CARTESIAN_POINT ( 'NONE',  ( 6.902403728792015691, 121.7324704480519983, -0.3323477824281221849 ) ) ;
#37187=CARTESIAN_POINT ( 'NONE',  ( -8.764399874728846740, 117.8902759020840421, 0.3181776094565136881 ) ) ;
#37189=CARTESIAN_POINT ( 'NONE',  ( 3.259383964624091412, 115.6909491485452435, -1.531612751755973223 ) ) ;
#37190=CARTESIAN_POINT ( 'NONE',  ( -5.263358945736734462, 121.3020066425206807, -0.2711714534586359138 ) ) ;
#37191=CARTESIAN_POINT ( 'NONE',  ( 2.546550616605329775, -14.95902107118821078, 5.737972450990987738 ) ) ;
#37192=CARTESIAN_POINT ( 'NONE',  ( -21.13693409061731998, 150.2702755442954583, 1.277357359820448846 ) ) ;
#37194=CARTESIAN_POINT ( 'NONE',  ( 4.801338745261147345, 117.3993836135855275, -1.016148444996444189 ) ) ;
#37195=CARTESIAN_POINT ( 'NONE',  ( 0.3005257795022526213, 116.4832816433156069, 0.09989594597631686057 ) ) ;
#37196=CARTESIAN_POINT ( 'NONE',  ( 15.38000172822621536, 147.8312228277220868, 0.3073290368998169431 ) ) ;
#37198=CARTESIAN_POINT ( 'NONE',  ( -0.1020318426323372635, 30.30579279289823802, -0.9687052925327788166 ) ) ;
#37199=CARTESIAN_POINT ( 'NONE',  ( -8.078287538471746743, 158.6595088495342338, -0.1614234102745197019 ) ) ;
#37202=CARTESIAN_POINT ( 'NONE',  ( 3.456281358658134906, 50.63946620154572997, 1.847419665314800064 ) ) ;
#37204=CARTESIAN_POINT ( 'NONE',  ( 8.451590122553549023, 119.2591792085226103, 1.352863054565908607 ) ) ;
#37205=CARTESIAN_POINT ( 'NONE',  ( 3.951836011467571907, -5.044640503713330837, -2.394960105287299523 ) ) ;
#37206=CARTESIAN_POINT ( 'NONE',  ( 21.80375291804136140, 148.4185114426368841, 2.147915116047498962 ) ) ;
#37208=TOROIDAL_SURFACE ( 'NONE', #33149, 3.683000000000000718, 0.5080000000000000071 ) ;
#37209=CARTESIAN_POINT ( 'NONE',  ( 14.68166051447191123, 123.3142630313093377, -1.213898157370195241 ) ) ;
#37210=CARTESIAN_POINT ( 'NONE',  ( -0.05192310401019068627, -8.293124787585329116, 4.627658001227512585 ) ) ;
#37211=CARTESIAN_POINT ( 'NONE',  ( -5.840790351889599386, 117.5931221156369730, -0.8184019802203832405 ) ) ;
#37212=CARTESIAN_POINT ( 'NONE',  ( 4.793196582158109287, 117.7334801314650008, -0.8915230911338991593 ) ) ;
#37215=CARTESIAN_POINT ( 'NONE',  ( -15.57078937218329173, 147.5402044622178153, 0.01782986306386609779 ) ) ;
#37216=CARTESIAN_POINT ( 'NONE',  ( 4.375071722208805802, -15.20633266255931559, 4.762636924185132514 ) ) ;
#37218=CARTESIAN_POINT ( 'NONE',  ( -4.824733838022108756, 115.9539541688524622, -1.371509286363743030 ) ) ;
#37220=CARTESIAN_POINT ( 'NONE',  ( 18.69815986816969655, 149.1225091032880528, 2.485088035475524038 ) ) ;
#37221=CARTESIAN_POINT ( 'NONE',  ( -3.174366308152013705, 104.6144662015457243, -0.06343139340882732180 ) ) ;
#37223=CARTESIAN_POINT ( 'NONE',  ( -2.940475496281335310, 117.1197906563906344, 0.4390297717439134995 ) ) ;
#37224=CARTESIAN_POINT ( 'NONE',  ( 8.413794655563325620, 13.29309125005104164, 0.5966991197660089785 ) ) ;
#37225=CARTESIAN_POINT ( 'NONE',  ( 16.14046266016579878, 146.7365623387580342, 1.292066526867236220 ) ) ;
#37227=CARTESIAN_POINT ( 'NONE',  ( 11.52575769572317377, 118.8226552325407397, -0.2321966025152968904 ) ) ;
#37228=CARTESIAN_POINT ( 'NONE',  ( 4.825452542548434920, 117.8355215987486275, -0.7438749666106165837 ) ) ;
#37229=VECTOR ( 'NONE', #30352, 1000.000000000000000 ) ;
#37234=CARTESIAN_POINT ( 'NONE',  ( -4.246359198923776113, 118.2246726177936580, 0.3144336963837771615 ) ) ;
#37235=CARTESIAN_POINT ( 'NONE',  ( 1.969389160195163857, 106.3931338143290475, -4.957017173386934594 ) ) ;
#37239=CARTESIAN_POINT ( 'NONE',  ( -4.228505362209877383, 119.3620910118516321, -0.9269648930420215649 ) ) ;
#37240=CARTESIAN_POINT ( 'NONE',  ( -5.028795574735199558, 114.3519703858145959, -1.961426316196308361 ) ) ;
#37241=CARTESIAN_POINT ( 'NONE',  ( 4.340305978642269302, 118.1815293345206896, 0.6239748096490277396 ) ) ;
#37242=CARTESIAN_POINT ( 'NONE',  ( -16.06762827093127299, 146.3760696504137684, -1.175121962453930635 ) ) ;
#37243=CARTESIAN_POINT ( 'NONE',  ( -6.656543858376176668E-14, 104.6144662015457243, -3.850115147268248130E-19 ) ) ;
#37246=CARTESIAN_POINT ( 'NONE',  ( 3.110646482806172397, 107.8085536575111689, -4.359277737140974551 ) ) ;
#37247=CARTESIAN_POINT ( 'NONE',  ( -15.47075146591473072, 139.6011575924185877, -1.761802977227842293 ) ) ;
#37251=CARTESIAN_POINT ( 'NONE',  ( -15.53206457832155785, 147.5381829847979702, -0.1100152830077117949 ) ) ;
#37253=CARTESIAN_POINT ( 'NONE',  ( 13.07250590169503823, 156.9444350391594014, 1.084824903291609743 ) ) ;
#37255=CARTESIAN_POINT ( 'NONE',  ( 3.076715286590720133, -14.17522324541667444, 1.337940584860995319 ) ) ;
#37256=CARTESIAN_POINT ( 'NONE',  ( 7.994725381675307219, 118.4344479264803169, -0.7928399906090749516 ) ) ;
#37257=CARTESIAN_POINT ( 'NONE',  ( -11.72911894083935458, 122.8035986606355152, 1.269020613264102204 ) ) ;
#37258=CARTESIAN_POINT ( 'NONE',  ( -0.6334066649623988354, -12.81304641701132851, -0.7396855475671405555 ) ) ;
#37259=CARTESIAN_POINT ( 'NONE',  ( 0.004913308685967637639, 116.7872217978203224, -0.2458820580207658202 ) ) ;
#37260=CARTESIAN_POINT ( 'NONE',  ( 0.3889013835376298744, 10.72134676413487142, 0.8939893681288630933 ) ) ;
#37263=CARTESIAN_POINT ( 'NONE',  ( -14.97557080935144569, 148.8997249754567349, 0.5399649533830233050 ) ) ;
#37264=CARTESIAN_POINT ( 'NONE',  ( 4.144384115003134639, -13.99490941865914806, 4.432938699676250316 ) ) ;
#37265=CARTESIAN_POINT ( 'NONE',  ( 8.809140270325693578, 122.1986804192922875, -0.8245386672919368110 ) ) ;
#37267=CARTESIAN_POINT ( 'NONE',  ( 1.784992122055886199, 115.7029483427795782, 1.723372422334099152 ) ) ;
#37268=CARTESIAN_POINT ( 'NONE',  ( 2.843374750741399559, -13.00285448706176084, 0.5077109796929276664 ) ) ;
#37270=CARTESIAN_POINT ( 'NONE',  ( 11.84655969407677567, 151.9972573545839225, 0.1156591128142185482 ) ) ;
#37272=CARTESIAN_POINT ( 'NONE',  ( 14.15513794057036989, 123.4894365733723447, 1.873888081047781595 ) ) ;
#37273=CARTESIAN_POINT ( 'NONE',  ( 1.247874008749637165, 106.2090255614403276, 5.187965977526303618 ) ) ;
#37274=CARTESIAN_POINT ( 'NONE',  ( -10.08214312826213721, 118.0934564804969114, -0.2014652138697927419 ) ) ;
#37276=CARTESIAN_POINT ( 'NONE',  ( 0.03245814172805025488, 157.7902383798253538, -1.624338139048501439 ) ) ;
#37277=CARTESIAN_POINT ( 'NONE',  ( 21.89150648822671030, 151.4414241944827495, 0.2106634337039131888 ) ) ;
#37279=CARTESIAN_POINT ( 'NONE',  ( 1.871143833745863239, -15.59325378310091814, 5.931567052087414638 ) ) ;
#37280=LINE ( 'NONE', #28102, #6565 ) ;
#37283=CARTESIAN_POINT ( 'NONE',  ( -4.720317703858613712, 117.8402133106318246, 0.8448306392985246438 ) ) ;
#37284=EDGE_LOOP ( 'NONE', ( #28040, #31224, #22140, #5701 ) ) ;
#37285=CARTESIAN_POINT ( 'NONE',  ( -4.801770124281918406, 117.3993836135855133, 1.016061139389656587 ) ) ;
#37286=CARTESIAN_POINT ( 'NONE',  ( -2.554268019588743943, 117.5995512635590643, -0.7715010912678383903 ) ) ;
#37287=CARTESIAN_POINT ( 'NONE',  ( -1.451835205608249080, 110.3135721340718334, -3.567596948272937496 ) ) ;
#37288=CARTESIAN_POINT ( 'NONE',  ( 4.820214878024821736, 117.6751674563618053, 1.076090311930151255 ) ) ;
#37290=CARTESIAN_POINT ( 'NONE',  ( -0.03040743766756944313, 116.4813942609868178, 1.521712522323421579 ) ) ;
#37291=VECTOR ( 'NONE', #621, 1000.000000000000000 ) ;
#37292=CARTESIAN_POINT ( 'NONE',  ( 4.364008504204949013, 7.202613900313124873, 1.580794030135405537 ) ) ;
#37293=CARTESIAN_POINT ( 'NONE',  ( -3.527324519276147541, 50.63946620154572997, 1.707870599815379364 ) ) ;
#37294=CARTESIAN_POINT ( 'NONE',  ( -4.815530361150011984, 118.5264896598256854, 0.7999101472927785395 ) ) ;
#37295=CARTESIAN_POINT ( 'NONE',  ( 3.910559219094527528, -13.09373064504072737, 2.776858670901594994 ) ) ;
#37296=CARTESIAN_POINT ( 'NONE',  ( 4.048024155119271050, 117.4230540797109938, -0.8140401526052125636 ) ) ;
#37297=PRODUCT_DEFINITION ( 'UNKNOWN', '', #18251, #6535 ) ;
#37298=CARTESIAN_POINT ( 'NONE',  ( -3.575185924110746871, 29.88618740006140584, 3.683134272688635580 ) ) ;
#37300=CARTESIAN_POINT ( 'NONE',  ( -0.5927862973117289380, 115.7030772917255490, 1.739502740807663095 ) ) ;
#37302=CARTESIAN_POINT ( 'NONE',  ( -2.612664856745740671, 104.6144662015509681, -4.653567239894925933 ) ) ;
#37303=CARTESIAN_POINT ( 'NONE',  ( 4.169050558263453610, -15.30144204372030359, -0.4701337638493395255 ) ) ;
#37304=CARTESIAN_POINT ( 'NONE',  ( -18.61143607275154466, 150.2488615152233820, 1.729315005182988418 ) ) ;
#37305=CARTESIAN_POINT ( 'NONE',  ( -0.08934464221186895483, 15.61415217803747169, 0.9739947352787643453 ) ) ;
#37308=ORIENTED_EDGE ( 'NONE', *, *, #8984, .F. ) ;
#37310=CARTESIAN_POINT ( 'NONE',  ( 2.266726881631522694, 118.5759350612125900, 0.8281820106640960244 ) ) ;
#37311=CARTESIAN_POINT ( 'NONE',  ( -3.544426656953535204, 120.3814187630814132, 0.4774784233729821303 ) ) ;
#37314=CARTESIAN_POINT ( 'NONE',  ( 4.601497379863265458, 118.0704624899502164, -0.5722604949035791089 ) ) ;
#37315=CARTESIAN_POINT ( 'NONE',  ( 1.363824289596507588, 119.4570717772418220, -0.5813626927913072562 ) ) ;
#37316=CARTESIAN_POINT ( 'NONE',  ( -2.213841846844945671, 118.2767885243204944, -0.7726204694312125421 ) ) ;
#37319=VERTEX_POINT ( 'NONE', #13881 ) ;
#37320=CARTESIAN_POINT ( 'NONE',  ( 4.116109897646406779, 118.2429491485453354, -0.1887006734943049158 ) ) ;
#37321=CARTESIAN_POINT ( 'NONE',  ( 14.81827458270670128, 148.8567844064068026, -0.2884810962875100637 ) ) ;
#37323=CARTESIAN_POINT ( 'NONE',  ( 3.216700609619024931, -14.42020774479446921, 2.887214088933996337 ) ) ;
#37326=CARTESIAN_POINT ( 'NONE',  ( -5.006118277528749161, 117.4009255802263283, 0.7893014723888780448 ) ) ;
#37328=CARTESIAN_POINT ( 'NONE',  ( 1.861163356255745915, -7.643417679262992870, 4.233688895527200735 ) ) ;
#37329=CARTESIAN_POINT ( 'NONE',  ( 11.93440950959098323, 126.0992317015783328, 1.505959514896210827 ) ) ;
#37330=CARTESIAN_POINT ( 'NONE',  ( -3.933769473788125026, 27.98561731294367050, 0.4889718192695881038 ) ) ;
#37331=CARTESIAN_POINT ( 'NONE',  ( -7.563607548680848502, 124.2956292408697863, -0.1420234171030813897 ) ) ;
#37332=CARTESIAN_POINT ( 'NONE',  ( -1.251853189678833411, -4.679435864505671283, 4.458631606201990394 ) ) ;
#37333=CARTESIAN_POINT ( 'NONE',  ( 15.22644562805675328, 143.4365109762209158, 0.4329964906482477449 ) ) ;
#37336=CARTESIAN_POINT ( 'NONE',  ( -5.489085054281237497, 117.1391964092379965, -0.7660907124981986005 ) ) ;
#37337=CARTESIAN_POINT ( 'NONE',  ( 0.007670926890785616931, 121.5961256765098284, -0.3838845493044710233 ) ) ;
#37340=CARTESIAN_POINT ( 'NONE',  ( 0.7770267621822702919, 9.899933826931993863, -8.437367074289049640 ) ) ;
#37344=CARTESIAN_POINT ( 'NONE',  ( 0.04081796246445149740, 114.7739974199301969, -2.042697753608868627 ) ) ;
#37345=CARTESIAN_POINT ( 'NONE',  ( -22.64827982350394464, 150.3405807453409579, 0.2709709482530831548 ) ) ;
#37351=ORIENTED_EDGE ( 'NONE', *, *, #15141, .T. ) ;
#37353=CARTESIAN_POINT ( 'NONE',  ( -15.52687642492895037, 147.5330934759543879, -0.3102639428822864254 ) ) ;
#37354=CARTESIAN_POINT ( 'NONE',  ( 5.820489720963992752, -14.55473177801069795, 2.572867947693331381 ) ) ;
#37355=CARTESIAN_POINT ( 'NONE',  ( -19.67014042257531869, 150.6586468064772646, 1.570413873854537457 ) ) ;
#37356=CARTESIAN_POINT ( 'NONE',  ( 12.81731082034050573, 120.0678233105195716, -0.7045657984066407975 ) ) ;
#37357=CARTESIAN_POINT ( 'NONE',  ( -2.136650056307613621, 10.86338872207680950, -4.114640003288728920 ) ) ;
#37358=CARTESIAN_POINT ( 'NONE',  ( -9.724873038622067867, 118.0756159837034716, -0.5523889259422301024 ) ) ;
#37361=CARTESIAN_POINT ( 'NONE',  ( -5.322365003949023787, 156.4258374981641282, 1.486226487625613712 ) ) ;
#37364=CARTESIAN_POINT ( 'NONE',  ( 0.01133701094394712686, 119.0130636887059410, -0.5673503866435171128 ) ) ;
#37365=CARTESIAN_POINT ( 'NONE',  ( -0.3947855200659833863, 117.7785671674745771, -0.5311790665990139271 ) ) ;
#37368=CARTESIAN_POINT ( 'NONE',  ( 16.05848832435423290, 147.7157881801689427, -0.7882342824236391321 ) ) ;
#37370=CARTESIAN_POINT ( 'NONE',  ( 0.03066982525775523508, 157.3074135339440147, -1.534843470138540278 ) ) ;
#37371=CARTESIAN_POINT ( 'NONE',  ( 3.754758974503722868, -15.60599068302642678, 3.401513958955031836 ) ) ;
#37373=CARTESIAN_POINT ( 'NONE',  ( -4.426261876493431835, 118.1635320031892178, -0.6236544883123098515 ) ) ;
#37375=CARTESIAN_POINT ( 'NONE',  ( -4.997723913362575487, 117.4043970260275813, 0.8231665828273773133 ) ) ;
#37376=CARTESIAN_POINT ( 'NONE',  ( 2.103759425340601119, 157.1282018749678002, 1.585319646506186730 ) ) ;
#37377=DIRECTION ( 'NONE',  ( -0.9998004120163608288, -5.205824365704082573E-17, -0.01997839162482749342 ) ) ;
#37380=CARTESIAN_POINT ( 'NONE',  ( 22.83607019214376521, 150.4065277667444036, 0.4307393832409500134 ) ) ;
#37381=CARTESIAN_POINT ( 'NONE',  ( -8.161197318747062113, 2.438352165997351495, -2.203247879407881804 ) ) ;
#37382=CARTESIAN_POINT ( 'NONE',  ( 13.65930421665831851, 150.2105054413494543, 0.7115039165091188167 ) ) ;
#37383=CARTESIAN_POINT ( 'NONE',  ( 0.4044265971210334598, 118.1627375710014007, -0.8899864531652206256 ) ) ;
#37385=CARTESIAN_POINT ( 'NONE',  ( -3.147325619572344468, 118.1588897472110773, 0.6788706689571556430 ) ) ;
#37386=CARTESIAN_POINT ( 'NONE',  ( -7.819160365854489037, 122.4258430437401159, -0.5979938724132283223 ) ) ;
#37388=CARTESIAN_POINT ( 'NONE',  ( -20.69264154312393700, 152.5691845998198346, -0.2640292844866432009 ) ) ;
#37391=CARTESIAN_POINT ( 'NONE',  ( 5.907666735792171053, 121.3440877105034019, -0.1410375414887058143 ) ) ;
#37392=CARTESIAN_POINT ( 'NONE',  ( -7.784012322544769269, 122.6313477034873074, -0.1555430911242075831 ) ) ;
#37393=EDGE_LOOP ( 'NONE', ( #4645, #40309, #41371, #29224 ) ) ;
#37394=CARTESIAN_POINT ( 'NONE',  ( 0.8084953953736374599, 118.7629491485454025, -1.239640985604131274 ) ) ;
#37395=CARTESIAN_POINT ( 'NONE',  ( -9.106360905785223281, 123.9337093609977529, -0.4112724569044293177 ) ) ;
#37396=CARTESIAN_POINT ( 'NONE',  ( 4.626636300257242596, -12.70421170364453900, 2.362638098592509284 ) ) ;
#37397=CARTESIAN_POINT ( 'NONE',  ( -0.02156508032628448243, 159.2730288250082538, 1.079204802879467850 ) ) ;
#37399=CARTESIAN_POINT ( 'NONE',  ( 3.735388766124958515, 116.6566025657135413, 0.1875874814615932362 ) ) ;
#37400=CARTESIAN_POINT ( 'NONE',  ( 11.83237999055733525, 152.0315156623530015, 0.2988832620038224253 ) ) ;
#37401=CARTESIAN_POINT ( 'NONE',  ( 0.8332047475417917459, 28.58290516567101491, -0.5069163209656499802 ) ) ;
#37402=CARTESIAN_POINT ( 'NONE',  ( -18.84770637050854347, 125.3331924886369961, -0.3953412214710179673 ) ) ;
#37405=ORIENTED_EDGE ( 'NONE', *, *, #32873, .T. ) ;
#37408=CARTESIAN_POINT ( 'NONE',  ( -8.410730074438736992, 119.6967890130903527, 1.093143251542445293 ) ) ;
#37410=CARTESIAN_POINT ( 'NONE',  ( 4.887760029584741872, 117.7409041207840090, 0.8724161813180757452 ) ) ;
#37412=CARTESIAN_POINT ( 'NONE',  ( 19.78169998575264898, 149.7343351798865285, -1.666391814173802777 ) ) ;
#37413=CARTESIAN_POINT ( 'NONE',  ( -8.287855504117665362, 18.49606730478969752, 1.603550922811438406 ) ) ;
#37414=CARTESIAN_POINT ( 'NONE',  ( -1.978713825503293000, 117.0827246868714013, -0.4887249842031141656 ) ) ;
#37415=CARTESIAN_POINT ( 'NONE',  ( 4.765286331752896842, 117.6625230355866734, -0.9424543435797743118 ) ) ;
#37418=CARTESIAN_POINT ( 'NONE',  ( -15.28873023128513431, 143.4753230507764670, 0.02859522846259937578 ) ) ;
#37419=CARTESIAN_POINT ( 'NONE',  ( 6.478224611219328466, -13.79365725417489053, 0.02984861787792387686 ) ) ;
#37420=CARTESIAN_POINT ( 'NONE',  ( -5.243373088111836999, 115.7725975576125421, -0.9931249584465892122 ) ) ;
#37422=CARTESIAN_POINT ( 'NONE',  ( 12.47579035109649936, 122.9501582372872406, 1.831147514963964884 ) ) ;
#37423=DIRECTION ( 'NONE',  ( -4.017660918040594346E-17, 1.000000000000000000, 2.376309959284834438E-19 ) ) ;
#37425=CARTESIAN_POINT ( 'NONE',  ( -0.8718816746735710277, 108.7514562038770976, 4.146788293844217321 ) ) ;
#37426=CARTESIAN_POINT ( 'NONE',  ( -6.647063868753328997, 9.619588520696709111, 5.217091374630535405 ) ) ;
#37427=CARTESIAN_POINT ( 'NONE',  ( 8.365438877267163065, 122.6561726160659731, 0.7803013885889898971 ) ) ;
#37429=CARTESIAN_POINT ( 'NONE',  ( 13.37627446016221811, 119.7032035076741465, -0.2201875619950499907 ) ) ;
#37432=CARTESIAN_POINT ( 'NONE',  ( 2.958531772299236362, 39.20946620154573736, 1.329372033065076453 ) ) ;
#37434=DIRECTION ( 'NONE',  ( -0.9998004120163608288, 0.000000000000000000, -0.01997839162482747608 ) ) ;
#37435=CARTESIAN_POINT ( 'NONE',  ( -4.118424193844660408, 118.2429491485453354, 0.1861966408306291454 ) ) ;
#37436=CARTESIAN_POINT ( 'NONE',  ( 3.765733841297878470, 109.1680412998367018, -3.784223926032564744 ) ) ;
#37439=CARTESIAN_POINT ( 'NONE',  ( -8.260936656145158707, 120.1795542499276337, -1.448930651378003365 ) ) ;
#37441=CARTESIAN_POINT ( 'NONE',  ( 4.269754544072226210, 118.2136401199853850, 0.5281557113276503790 ) ) ;
#37442=CARTESIAN_POINT ( 'NONE',  ( -4.491182069977996072, 120.9948550335633115, -0.4087774027959018563 ) ) ;
#37443=CARTESIAN_POINT ( 'NONE',  ( -2.958531772299361595, 50.13146620154573441, -1.329372033065077119 ) ) ;
#37447=CARTESIAN_POINT ( 'NONE',  ( 0.9564925537785137211, 29.00497265395555857, -4.523030980006896407 ) ) ;
#37448=CARTESIAN_POINT ( 'NONE',  ( 0.006810764310280531704, 120.3493709785083183, -0.3408384964863777622 ) ) ;
#37452=CARTESIAN_POINT ( 'NONE',  ( 7.784761315929978664, 122.6240617022501169, 0.1928303156072929958 ) ) ;
#37453=CARTESIAN_POINT ( 'NONE',  ( 4.610398055573782905, 23.01736123548795021, -0.3254830233858732602 ) ) ;
#37454=CARTESIAN_POINT ( 'NONE',  ( 22.22941764614895277, 150.1947564971097222, 1.617977611002929805 ) ) ;
#37456=CARTESIAN_POINT ( 'NONE',  ( 3.046489168745748266, -14.83993489217504091, 3.784491786591300588 ) ) ;
#37457=CARTESIAN_POINT ( 'NONE',  ( 21.08161885447492168, 149.3892802667211868, -1.460526482899864309 ) ) ;
#37458=CARTESIAN_POINT ( 'NONE',  ( -7.897101653775167485, 156.2605297791399437, 1.696642280025655758 ) ) ;
#37459=CARTESIAN_POINT ( 'NONE',  ( 4.518289034361447243, 23.24227448397437001, -0.9983406360900146659 ) ) ;
#37460=CARTESIAN_POINT ( 'NONE',  ( -0.9708930699732380987, 116.8374933757159795, -0.3283832199399771001 ) ) ;
#37461=CARTESIAN_POINT ( 'NONE',  ( 0.2555639604167124768, 10.49987491555810593, 0.9396316490698124468 ) ) ;
#37465=CARTESIAN_POINT ( 'NONE',  ( -11.61789020275273110, 128.2970750771678752, 0.3952796010287949469 ) ) ;
#37466=CARTESIAN_POINT ( 'NONE',  ( 5.673176617818914913, -13.06232935199844114, 2.160669506476638357 ) ) ;
#37467=CARTESIAN_POINT ( 'NONE',  ( 5.070296302330485894, 156.2174774745075183, -1.306674740328298112 ) ) ;
#37469=CARTESIAN_POINT ( 'NONE',  ( 2.906445675538798845, 115.7029491485453434, 1.674890049949036896 ) ) ;
#37470=CARTESIAN_POINT ( 'NONE',  ( 1.985452195540454934, -15.12483337350742296, 5.348831821476924375 ) ) ;
#37471=CARTESIAN_POINT ( 'NONE',  ( -4.796665243919449928, 117.7368776771948831, -1.049558999684713667 ) ) ;
#37472=CARTESIAN_POINT ( 'NONE',  ( 0.001367086239692558765, 156.3041635968983485, -0.06841458569046209026 ) ) ;
#37473=VERTEX_POINT ( 'NONE', #16645 ) ;
#37474=CARTESIAN_POINT ( 'NONE',  ( 2.242647228084396982, 118.4336326928681729, 0.7879290844312368813 ) ) ;
#37477=CIRCLE ( 'NONE', #7539, 5.080000000000006288 ) ;
#37479=CARTESIAN_POINT ( 'NONE',  ( 1.415223785869755613, 159.6020224343070026, -0.1017758242917465722 ) ) ;
#37481=TOROIDAL_SURFACE ( 'NONE', #18402, 5.080000000000005400, 0.5080000000000000071 ) ;
#37482=CARTESIAN_POINT ( 'NONE',  ( 1.693218665641037735, -15.38421670575504407, 5.480670678043046529 ) ) ;
#37485=CARTESIAN_POINT ( 'NONE',  ( -4.743057898818983986, 117.8454596101170750, 0.8300490160943797546 ) ) ;
#37488=CARTESIAN_POINT ( 'NONE',  ( -1.008980461684340080, 118.7629491485454025, 1.225333421752663021 ) ) ;
#37489=EDGE_CURVE ( 'NONE', #24814, #30281, #3873, .T. ) ;
#37490=CARTESIAN_POINT ( 'NONE',  ( 2.640464088051889480, 117.6788351930554199, -0.6858096912303740522 ) ) ;
#37491=CARTESIAN_POINT ( 'NONE',  ( -1.881281939329409125, 113.2583846565721757, -2.513576850050686318 ) ) ;
#37492=CARTESIAN_POINT ( 'NONE',  ( 4.873962307784054815, 117.4785107143119092, 1.135666542019568404 ) ) ;
#37493=CARTESIAN_POINT ( 'NONE',  ( -4.611806494114576438, 117.9324678712513759, -0.9633187536371230486 ) ) ;
#37494=CARTESIAN_POINT ( 'NONE',  ( -0.1289837059588684054, 106.1822392402443143, 5.211597877332949658 ) ) ;
#37498=CARTESIAN_POINT ( 'NONE',  ( 2.953219771904812774, -14.51063682438745417, 4.500484459945554683 ) ) ;
#37499=CARTESIAN_POINT ( 'NONE',  ( 6.983605877934210504, 124.9344662015457175, 0.1395490654994204494 ) ) ;
#37500=CARTESIAN_POINT ( 'NONE',  ( -2.127773614577548766, 31.68089970468614069, 4.228698531287117035 ) ) ;
#37501=CARTESIAN_POINT ( 'NONE',  ( -0.1384325697538203448, 115.7030669245054497, 1.759162187147021550 ) ) ;
#37502=CARTESIAN_POINT ( 'NONE',  ( 0.6590154617207463206, 19.50938314818779062, -4.574821423538240950 ) ) ;
#37505=CARTESIAN_POINT ( 'NONE',  ( 2.770358398913809861, -15.65020961539316602, 4.804192819214700982 ) ) ;
#37506=CARTESIAN_POINT ( 'NONE',  ( -5.031139012175450453, 119.0545008048120366, 0.9043826811606223703 ) ) ;
#37507=CARTESIAN_POINT ( 'NONE',  ( -0.7929698604315037480, -4.880942799695234591, 0.5714185140920283734 ) ) ;
#37509=CARTESIAN_POINT ( 'NONE',  ( 0.9036657058557058253, 17.56215383894848614, 0.3677562154327245758 ) ) ;
#37510=EDGE_CURVE ( 'NONE', #36953, #29654, #38543, .T. ) ;
#37512=ORIENTED_EDGE ( 'NONE', *, *, #25820, .T. ) ;
#37514=CARTESIAN_POINT ( 'NONE',  ( 0.1346051971225362132, 106.5118632461160217, 5.080372420286161095 ) ) ;
#37515=CARTESIAN_POINT ( 'NONE',  ( -1.846154440359773385, 156.5029897098349636, 0.9826124536999809589 ) ) ;
#37517=CARTESIAN_POINT ( 'NONE',  ( 4.515008956836783049, 118.0822181440858287, -0.6204359177205427400 ) ) ;
#37518=CARTESIAN_POINT ( 'NONE',  ( 10.90225753734626757, 122.6724665872831679, -1.173089625842028472 ) ) ;
#37520=CARTESIAN_POINT ( 'NONE',  ( -15.05911097818686883, 125.5446871707752763, -2.024973821723874856 ) ) ;
#37522=CARTESIAN_POINT ( 'NONE',  ( 4.123312261480172047, 118.2429491485453354, -0.1806149775832581461 ) ) ;
#37523=CARTESIAN_POINT ( 'NONE',  ( 13.24427968334902062, 134.0707761029912035, -0.3110103029741251857 ) ) ;
#37525=CARTESIAN_POINT ( 'NONE',  ( 2.101618670382315646, -15.21789252882688182, 5.187277112784037136 ) ) ;
#37526=AXIS2_PLACEMENT_3D ( 'NONE', #35625, #32844, #12615 ) ;
#37529=CARTESIAN_POINT ( 'NONE',  ( 4.168288449772385995, -6.568960759998498489, 2.029292378399509378 ) ) ;
#37530=CARTESIAN_POINT ( 'NONE',  ( 16.52407570443671148, 148.2569838091642964, 1.909119861936069640 ) ) ;
#37531=CARTESIAN_POINT ( 'NONE',  ( 0.03201377673046579275, 33.52827609515317420, 3.383309648808628278 ) ) ;
#37532=CARTESIAN_POINT ( 'NONE',  ( -4.210090452738601385, 118.4033805524614849, 0.5735154781215828779 ) ) ;
#37535=CARTESIAN_POINT ( 'NONE',  ( -0.5842699607273857954, -4.454521554441356557, 4.585487691134133570 ) ) ;
#37536=CARTESIAN_POINT ( 'NONE',  ( 13.59447973938432241, 150.2262467139961473, 0.3969463805754211427 ) ) ;
#37537=B_SPLINE_CURVE_WITH_KNOTS ( 'NONE', 3,
 ( #37285, #24484, #5142, #18096, #29591, #6177 ),
 .UNSPECIFIED., .F., .F.,
 ( 4, 2, 4 ),
 ( 0.000000000000000000, 0.5000000000000000000, 1.000000000000000000 ),
 .UNSPECIFIED. ) ;
#37538=EDGE_CURVE ( 'NONE', #27974, #1598, #7013, .T. ) ;
#37539=CARTESIAN_POINT ( 'NONE',  ( 4.614102091175348086, 5.327238342305563812, -7.074968232746598140 ) ) ;
#37541=CARTESIAN_POINT ( 'NONE',  ( -5.507236293901328850, 116.9742688490489684, -0.6495416791669329504 ) ) ;
#37542=DIRECTION ( 'NONE',  ( -0.01997839162482737546, -1.040247600000940825E-18, 0.9998004120163610509 ) ) ;
#37546=CARTESIAN_POINT ( 'NONE',  ( -4.785772612713214080, 1.365856510964248649, -6.940074030798050408 ) ) ;
#37547=CARTESIAN_POINT ( 'NONE',  ( 0.6939153454146552713, 117.9394491594808159, 1.403384569749132282 ) ) ;
#37549=CARTESIAN_POINT ( 'NONE',  ( 2.568134854143032442, -15.02010252187911554, 4.714990346623905815 ) ) ;
#37550=CARTESIAN_POINT ( 'NONE',  ( 0.5256976547265018729, 110.0486234891351245, -3.677594289785357518 ) ) ;
#37551=CARTESIAN_POINT ( 'NONE',  ( -15.13173320725188553, 120.7387302883610118, 0.2100629019518970853 ) ) ;
#37556=CARTESIAN_POINT ( 'NONE',  ( -2.846496745999657740, 121.0294354067666802, -0.02263809173328865804 ) ) ;
#37557=CARTESIAN_POINT ( 'NONE',  ( 5.316001070410483642, -15.20466279102368468, 3.045604417706107458 ) ) ;
#37558=CARTESIAN_POINT ( 'NONE',  ( -13.28772774122556122, 155.5383117973235585, 1.582857276444406658 ) ) ;
#37559=CARTESIAN_POINT ( 'NONE',  ( 22.37379725164909416, 146.3189071340513294, -1.009121573351525303 ) ) ;
#37560=CARTESIAN_POINT ( 'NONE',  ( 1.893578447776079754, 19.08455809737888487, -4.224370802633358402 ) ) ;
#37561=CARTESIAN_POINT ( 'NONE',  ( -14.67516008282149897, 120.3119357913517291, -0.6057029122735547721 ) ) ;
#37564=CARTESIAN_POINT ( 'NONE',  ( 2.183095549435995597, 116.1905277699444952, 0.05681614786306111303 ) ) ;
#37565=DIRECTION ( 'NONE',  ( -0.9998004120163609398, 0.000000000000000000, -0.01997839162482749689 ) ) ;
#37566=CARTESIAN_POINT ( 'NONE',  ( -2.082154424533116721, 156.9412006218898057, 1.407003841209468753 ) ) ;
#37568=CARTESIAN_POINT ( 'NONE',  ( 6.702632528927829902, 119.6463993818898359, -1.017002412926887311 ) ) ;
#37569=CARTESIAN_POINT ( 'NONE',  ( -21.00644369030287351, 149.3892802667211868, -2.301546136566545275 ) ) ;
#37573=CARTESIAN_POINT ( 'NONE',  ( 4.574562528865535604, 155.9125706774115940, -0.7527123864290742317 ) ) ;
#37574=ORIENTED_EDGE ( 'NONE', *, *, #34966, .T. ) ;
#37575=CARTESIAN_POINT ( 'NONE',  ( -18.30884121703848066, 147.6341482083243761, -2.394331140672893099 ) ) ;
#37576=CARTESIAN_POINT ( 'NONE',  ( 3.404406166340397277, -15.64019586361782643, 4.053891870528842922 ) ) ;
#37577=CARTESIAN_POINT ( 'NONE',  ( -4.381873770367138654, 118.1622909913610187, -0.6666483627925274824 ) ) ;
#37580=CARTESIAN_POINT ( 'NONE',  ( -4.998096739426165946, 117.4661840451863100, 0.7739782158464477702 ) ) ;
#37581=CARTESIAN_POINT ( 'NONE',  ( 12.00230265366658600, 124.3217332413628640, 1.707838685025481418 ) ) ;
#37584=CARTESIAN_POINT ( 'NONE',  ( 6.515560366292186600, -0.8950661730705262720, -5.416678580889517924 ) ) ;
#37585=CARTESIAN_POINT ( 'NONE',  ( 9.426771831325547524, 124.2753396726362780, 0.5138045435804897698 ) ) ;
#37590=CARTESIAN_POINT ( 'NONE',  ( -2.609053440593664508, 117.3993834727424286, 1.321828139561898041 ) ) ;
#37591=CARTESIAN_POINT ( 'NONE',  ( -7.869668022420311715, 122.1460381220860540, -0.8492931709348270353 ) ) ;
#37592=AXIS2_PLACEMENT_3D ( 'NONE', #36571, #3406, #7597 ) ;
#37596=CARTESIAN_POINT ( 'NONE',  ( -22.65693159617103802, 137.2763855621842026, -0.2353725067100884694 ) ) ;
#37597=ORIENTED_EDGE ( 'NONE', *, *, #2971, .F. ) ;
#37599=CARTESIAN_POINT ( 'NONE',  ( -5.844832110966546423, 121.2807673435547571, -0.4307865532411910281 ) ) ;
#37600=CARTESIAN_POINT ( 'NONE',  ( -7.895606690698891761, 122.1535174891447468, 0.5249436039529434828 ) ) ;
#37601=EDGE_LOOP ( 'NONE', ( #38772, #10356, #18787, #23023 ) ) ;
#37602=CARTESIAN_POINT ( 'NONE',  ( -4.757281688282281706, 117.4019771528195690, -1.206666768175857385 ) ) ;
#37603=CARTESIAN_POINT ( 'NONE',  ( -3.721623402434381056, 121.0563512343167645, -0.1807651092205456167 ) ) ;
#37604=CARTESIAN_POINT ( 'NONE',  ( 3.016199308703121140, -15.16462411293013979, 5.702656747445028707 ) ) ;
#37605=CARTESIAN_POINT ( 'NONE',  ( -5.259787267153689605, 158.8115599018184412, 1.116423854902496071 ) ) ;
#37606=LINE ( 'NONE', #41236, #25440 ) ;
#37608=CARTESIAN_POINT ( 'NONE',  ( 20.36427691206291257, 129.0035756037533758, 0.5974333909176805513 ) ) ;
#37609=CARTESIAN_POINT ( 'NONE',  ( 7.783246152616065672, 154.6561476914895081, 0.1555277812256516956 ) ) ;
#37610=CARTESIAN_POINT ( 'NONE',  ( -4.876368518028720622, 117.7626870461374580, 0.7578736298905299762 ) ) ;
#37611=CARTESIAN_POINT ( 'NONE',  ( -0.9636992805836054332, 23.18535052081312386, 0.1494942155713751553 ) ) ;
#37612=CARTESIAN_POINT ( 'NONE',  ( -15.48069746188187956, 120.7065362441885981, -0.4134764081404141978 ) ) ;
#37614=CIRCLE ( 'NONE', #41699, 0.5079999999999997851 ) ;
#37618=CARTESIAN_POINT ( 'NONE',  ( 6.232159320193214391, 119.2349664191863070, 1.255280209171262040 ) ) ;
#37620=CARTESIAN_POINT ( 'NONE',  ( -5.334819979684278124, 105.1224662015457199, -0.01225255181739587709 ) ) ;
#37621=CARTESIAN_POINT ( 'NONE',  ( -0.02156508032628448243, 159.2730288250082538, 1.079204802879467850 ) ) ;
#37623=CARTESIAN_POINT ( 'NONE',  ( 10.28923284337270871, 120.3038588096988803, -1.141564125291498089 ) ) ;
#37624=CARTESIAN_POINT ( 'NONE',  ( 4.543739712435177047, -15.19060223592207137, -0.8445694877862246486 ) ) ;
#37625=CARTESIAN_POINT ( 'NONE',  ( 0.007599820978684407140, 117.2191897141855179, -0.3803261187632671625 ) ) ;
#37626=CARTESIAN_POINT ( 'NONE',  ( 4.832896482213426381, 117.6748455158117395, -0.9055039834170672819 ) ) ;
#37627=CARTESIAN_POINT ( 'NONE',  ( 0.6661646497576521053, 105.9485402691003060, 5.310688274649121077 ) ) ;
#37629=CARTESIAN_POINT ( 'NONE',  ( -15.73538347863352804, 145.6958675726371553, -0.1858358763210236630 ) ) ;
#37630=CARTESIAN_POINT ( 'NONE',  ( -12.47579035109662726, 122.9501582372872406, -1.831147514963964662 ) ) ;
#37631=CARTESIAN_POINT ( 'NONE',  ( 5.947420766284201576, -14.61438673846185488, 1.993024607196187459 ) ) ;
#37632=AXIS2_PLACEMENT_3D ( 'NONE', #26822, #14025, #10624 ) ;
#37636=CARTESIAN_POINT ( 'NONE',  ( -0.7954092736443492129, 117.3993835805549537, -1.485886877084427571 ) ) ;
#37638=CARTESIAN_POINT ( 'NONE',  ( 7.518309192797149265, 120.1328256275108828, 1.363123692563724454 ) ) ;
#37640=CARTESIAN_POINT ( 'NONE',  ( 3.682264917456193665, 69.94346620154573202, 0.07358041635423968885 ) ) ;
#37641=AXIS2_PLACEMENT_3D ( 'NONE', #819, #27209, #16980 ) ;
#37642=CARTESIAN_POINT ( 'NONE',  ( -0.6471768874971802754, 112.6282971158091470, 2.732684515117584034 ) ) ;
#37643=CARTESIAN_POINT ( 'NONE',  ( 0.3193725800214416988, -13.04287899337829515, -8.422265478599168631 ) ) ;
#37644=CARTESIAN_POINT ( 'NONE',  ( 9.846098633339698480, 123.9483309312939099, 0.9889573185143103462 ) ) ;
#37647=CARTESIAN_POINT ( 'NONE',  ( 20.34281169216118101, 152.5255278361454145, -0.5339126128458229203 ) ) ;
#37651=ADVANCED_FACE ( 'NONE', ( #29165 ), #13199, .T. ) ;
#37652=CARTESIAN_POINT ( 'NONE',  ( -6.517733866319332394E-14, 78.32546620154573702, 2.848871684924056535E-29 ) ) ;
#37653=CARTESIAN_POINT ( 'NONE',  ( -4.248938432191276426, 118.2248689806160797, 0.3116314407555961230 ) ) ;
#37654=CARTESIAN_POINT ( 'NONE',  ( 5.113597892238037623, 113.8200073110514836, -1.623610037850725218 ) ) ;
#37657=CARTESIAN_POINT ( 'NONE',  ( 4.133480150819543120, 119.2345050349130702, -0.7621166359342830265 ) ) ;
#37658=CARTESIAN_POINT ( 'NONE',  ( -2.934015389105513183, 107.8085536575111689, -4.480064466837520243 ) ) ;
#37659=CARTESIAN_POINT ( 'NONE',  ( 4.378792325076509506, 118.1614122340369875, 0.6691606409793376953 ) ) ;
#37660=CARTESIAN_POINT ( 'NONE',  ( -6.199776539618502724, 155.3658059236344684, -0.8002054381730364652 ) ) ;
#37664=CARTESIAN_POINT ( 'NONE',  ( 2.488009491785908800, 18.85968022696138391, -3.895047602898422223 ) ) ;
#37666=DIRECTION ( 'NONE',  ( 4.017660918040594346E-17, -1.000000000000000000, -2.376309959284834438E-19 ) ) ;
#37667=CARTESIAN_POINT ( 'NONE',  ( 3.174366308151880922, 104.6144662015457243, 0.06343139340882769650 ) ) ;
#37669=CARTESIAN_POINT ( 'NONE',  ( -6.062815761959031491, 121.4378744781062096, -0.02555828286107298536 ) ) ;
#37670=CARTESIAN_POINT ( 'NONE',  ( -4.628372119175923949, 18.04465247731148381, -0.2036312542868722320 ) ) ;
#37671=CARTESIAN_POINT ( 'NONE',  ( 14.85510260296663176, 121.0052616771249347, 1.128405194827190705 ) ) ;
#37673=CARTESIAN_POINT ( 'NONE',  ( 3.205116352530840373, -14.62692654125133451, 3.000134484400556190 ) ) ;
#37674=CARTESIAN_POINT ( 'NONE',  ( 13.76672422736534607, 155.7522398296385404, -1.402631553274309217 ) ) ;
#37675=CARTESIAN_POINT ( 'NONE',  ( -9.425666535144351599, 121.4347015428822374, 1.122958709584368053 ) ) ;
#37676=CARTESIAN_POINT ( 'NONE',  ( 4.103230867730633058, 22.16771668783608007, 2.168033597859526651 ) ) ;
#37677=CARTESIAN_POINT ( 'NONE',  ( -1.374325311230039093, 159.5643428290674990, -0.4556871491110245365 ) ) ;
#37679=CARTESIAN_POINT ( 'NONE',  ( 0.05984739657028866761, 19.78266025878678391, 0.9748693421377304658 ) ) ;
#37682=CARTESIAN_POINT ( 'NONE',  ( -13.89276580153831020, 150.2454140652271803, 0.5485491450630710641 ) ) ;
#37683=CARTESIAN_POINT ( 'NONE',  ( 4.441035242322985965, -14.03446645907663282, 4.353459135924754086 ) ) ;
#37684=CARTESIAN_POINT ( 'NONE',  ( 11.42483690514958461, 124.5424752485109963, -1.054873134768183895 ) ) ;
#37686=CARTESIAN_POINT ( 'NONE',  ( 0.7772691865734456806, 115.7028435863886386, 1.754949168150819583 ) ) ;
#37688=CARTESIAN_POINT ( 'NONE',  ( 3.240066224740343781, -14.18897675264189928, 3.749338592554243288 ) ) ;
#37689=CARTESIAN_POINT ( 'NONE',  ( -4.710974563145049032, 117.8981397293982667, -0.9559088427545711086 ) ) ;
#37690=CARTESIAN_POINT ( 'NONE',  ( 9.118838228053421702, 124.0847320388339625, 0.09724818526966655385 ) ) ;
#37692=CARTESIAN_POINT ( 'NONE',  ( 19.76635024033924992, 141.2215177107240436, 2.477633452034131434 ) ) ;
#37693=CARTESIAN_POINT ( 'NONE',  ( 13.59117098936144075, 150.2425924485622772, 0.2715839415567424808 ) ) ;
#37696=CARTESIAN_POINT ( 'NONE',  ( 0.001640166039734963777, 159.6041700698465036, -0.08208061555506483697 ) ) ;
#37697=CARTESIAN_POINT ( 'NONE',  ( 21.87358050093867945, 151.4416708234707301, 0.1116233529550400561 ) ) ;
#37699=CARTESIAN_POINT ( 'NONE',  ( 1.865576733372334761, -15.48222874659857595, 5.392302077751139677 ) ) ;
#37702=CARTESIAN_POINT ( 'NONE',  ( -4.740160372624219853, 117.9514375547949925, 0.6504355775612526980 ) ) ;
#37705=CARTESIAN_POINT ( 'NONE',  ( 5.266140447862612817, 115.7029491485453150, -0.8695525029155279917 ) ) ;
#37706=CARTESIAN_POINT ( 'NONE',  ( -8.413693646442473195, 119.4405076545267548, -1.388540977510597685 ) ) ;
#37707=CARTESIAN_POINT ( 'NONE',  ( -5.744069310734515987, 120.3160329940760818, -0.4351690567359401407 ) ) ;
#37708=CARTESIAN_POINT ( 'NONE',  ( 4.871458131390602020, 117.6697264362294533, 1.013602582129945473 ) ) ;
#37710=CARTESIAN_POINT ( 'NONE',  ( -0.8647483397479580614, 121.9014879524050343, 0.2897378433829553290 ) ) ;
#37711=CARTESIAN_POINT ( 'NONE',  ( -0.5842699607273857954, -4.454521554441356557, 4.585487691134133570 ) ) ;
#37714=CARTESIAN_POINT ( 'NONE',  ( 2.454477138217164178, -14.79624793513299785, 5.258896552041426808 ) ) ;
#37715=CARTESIAN_POINT ( 'NONE',  ( 7.256067632580297300, 123.0461458356614628, 0.07605313119184042847 ) ) ;
#37718=DIRECTION ( 'NONE',  ( -0.9998004120163609398, 0.000000000000000000, -0.01997839162482749689 ) ) ;
#37719=CARTESIAN_POINT ( 'NONE',  ( 3.935102970030662117, 16.48578375386999539, 2.424025302511324309 ) ) ;
#37720=CARTESIAN_POINT ( 'NONE',  ( 15.83212890848021281, 121.4040080620525117, 0.8411940925737090291 ) ) ;
#37722=CARTESIAN_POINT ( 'NONE',  ( 3.864505497398623923, 104.6144662015456959, -2.895664945016856784 ) ) ;
#37723=CARTESIAN_POINT ( 'NONE',  ( 4.238804029399687145, -15.60588767656335918, 2.735912002563000822 ) ) ;
#37724=CARTESIAN_POINT ( 'NONE',  ( -4.562247774926802002, 157.9011380394538833, 1.652341844578318453 ) ) ;
#37725=CARTESIAN_POINT ( 'NONE',  ( 0.2465545558977290663, 24.09562519341298170, -0.9435640554424079562 ) ) ;
#37726=CARTESIAN_POINT ( 'NONE',  ( -0.8313783143457759151, 22.10655722792919065, -0.5139362334944024280 ) ) ;
#37727=VERTEX_POINT ( 'NONE', #7452 ) ;
#37729=DIRECTION ( 'NONE',  ( -0.01997839162482764261, -1.040247600000952381E-18, 0.9998004120163609398 ) ) ;
#37730=CARTESIAN_POINT ( 'NONE',  ( 1.302594956492339584, 113.6455945353133643, 2.391525302099168471 ) ) ;
#37732=CARTESIAN_POINT ( 'NONE',  ( -8.687188811298957702, 122.3401343867201945, 0.7349857017399259451 ) ) ;
#37734=CARTESIAN_POINT ( 'NONE',  ( 3.022112892507086812, -12.39725416092116106, 0.4273193741429963666 ) ) ;
#37735=CARTESIAN_POINT ( 'NONE',  ( 18.17603978048560620, 146.7121067869193496, -1.621728993581971645 ) ) ;
#37736=CARTESIAN_POINT ( 'NONE',  ( -2.242647228084525324, 118.4336326928681729, -0.7879290844312367703 ) ) ;
#37739=CARTESIAN_POINT ( 'NONE',  ( -4.873850642958227120, 32.38564726215445688, 3.744354677719523572 ) ) ;
#37740=CARTESIAN_POINT ( 'NONE',  ( 4.537977675602582472, 121.1059516323014549, -0.1178196913276177149 ) ) ;
#37741=VERTEX_POINT ( 'NONE', #29603 ) ;
#37742=CARTESIAN_POINT ( 'NONE',  ( 1.979187190576821465, -15.21425526833739639, 5.301287498526151332 ) ) ;
#37743=CARTESIAN_POINT ( 'NONE',  ( 4.979814073991923884, 117.5943741255363477, 0.7446744892861771881 ) ) ;
#37745=CARTESIAN_POINT ( 'NONE',  ( -4.567530434605131084, -10.44214056487004250, 0.7003524306260878740 ) ) ;
#37746=CARTESIAN_POINT ( 'NONE',  ( 8.727673846237058441, 154.8283212766472445, 1.585547369736020062 ) ) ;
#37747=CARTESIAN_POINT ( 'NONE',  ( 2.944162091193518904, 38.75495963859787452, 0.7149833688506975760 ) ) ;
#37748=CARTESIAN_POINT ( 'NONE',  ( -1.576215671565407650, 106.2483430537416638, 5.109971884176318646 ) ) ;
#37749=CARTESIAN_POINT ( 'NONE',  ( -0.5496829067194369811, 0.7180641350488168317, -4.598301960397928489 ) ) ;
#37750=CARTESIAN_POINT ( 'NONE',  ( -2.579283729523311308, 34.63205429821886838, 0.7922911722492685938 ) ) ;
#37751=CARTESIAN_POINT ( 'NONE',  ( 4.653112868187331941, 2.303567304790777648, 7.043327697551765354 ) ) ;
#37753=CARTESIAN_POINT ( 'NONE',  ( 8.775998379516696701, 117.8320079785639365, -0.2360308319456460580 ) ) ;
#37754=CARTESIAN_POINT ( 'NONE',  ( -0.3606724330769058295, 121.2597428844643161, -0.4428036157107447801 ) ) ;
#37757=CARTESIAN_POINT ( 'NONE',  ( 4.619096255015035624, 27.05588869245799089, -0.3994036469054788596 ) ) ;
#37758=CARTESIAN_POINT ( 'NONE',  ( -0.02983097946891679134, 117.3993836135855702, 1.492864285907040456 ) ) ;
#37761=CARTESIAN_POINT ( 'NONE',  ( 0.9377939088480686802, 122.9246775559910390, -0.1697371007065931747 ) ) ;
#37762=CARTESIAN_POINT ( 'NONE',  ( -4.803851041827917001, 116.9482543694763166, 0.2466672064845016887 ) ) ;
#37763=ORIENTED_EDGE ( 'NONE', *, *, #8676, .F. ) ;
#37765=ORIENTED_EDGE ( 'NONE', *, *, #13693, .T. ) ;
#37767=CARTESIAN_POINT ( 'NONE',  ( -8.027194241900888372, 122.8503413726703428, -0.1191878892407382262 ) ) ;
#37768=CARTESIAN_POINT ( 'NONE',  ( 3.423347803338410156, -15.46749709811699702, 5.412694551837634371 ) ) ;
#37769=CARTESIAN_POINT ( 'NONE',  ( -2.188165212810393445, 117.9909145081919917, 0.6446704472730119262 ) ) ;
#37770=CARTESIAN_POINT ( 'NONE',  ( 15.97727112977735686, 122.8751182158008959, -0.7600457325971274880 ) ) ;
#37771=CARTESIAN_POINT ( 'NONE',  ( 3.935102970030661673, 16.48578375386999539, 2.424025302511324309 ) ) ;
#37772=CARTESIAN_POINT ( 'NONE',  ( -6.906622810364809517, 117.2343425291504104, -0.3847307661620059105 ) ) ;
#37775=CARTESIAN_POINT ( 'NONE',  ( 8.797618036347394366, 117.6845732567335290, 0.1950281128173915746 ) ) ;
#37777=B_SPLINE_SURFACE_WITH_KNOTS ( 'NONE', 1, 3, ( 
 ( #34251, #31033, #11650, #14836, #34454, #8884, #34662, #5490, #21636, #37853, #27630, #8471 ),
 ( #5081, #38067, #40641, #34876, #31672, #11435, #15260, #1671, #18237, #2082, #21426, #21221 ) ),
 .UNSPECIFIED., .F., .F., .F.,
 ( 2, 2 ),
 ( 4, 3, 2, 3, 4 ),
 ( 0.000000000000000000, 1.000000000000000000 ),
 ( -0.01866551247456825838, 0.000000000000000000, 0.5000000000000000000, 1.000000000000000000, 1.010000000000000009 ),
 .UNSPECIFIED. ) ;
#37778=CARTESIAN_POINT ( 'NONE',  ( -10.46700094992505647, 122.9580799906392343, 1.049763322952065758 ) ) ;
#37780=CARTESIAN_POINT ( 'NONE',  ( 8.634969826328919851, 120.3810071108087243, -1.137220218559220619 ) ) ;
#37781=CARTESIAN_POINT ( 'NONE',  ( -1.172210521474351452, 158.9035955689636523, -1.423060353815112089 ) ) ;
#37783=CARTESIAN_POINT ( 'NONE',  ( 8.467456592458612263, 122.5794309061019618, -0.5337204191277989951 ) ) ;
#37785=CARTESIAN_POINT ( 'NONE',  ( -11.12287255170445022, 123.1247571232444784, -1.608126361149618821 ) ) ;
#37786=CARTESIAN_POINT ( 'NONE',  ( 2.046246934637348858, -15.60107924929197942, 5.318501171315276999 ) ) ;
#37789=CARTESIAN_POINT ( 'NONE',  ( -4.950256445730226496, 117.4773595571565608, 0.8982803358397978277 ) ) ;
#37790=CARTESIAN_POINT ( 'NONE',  ( 16.72996320514137736, 149.5530097695598215, 2.252745029998448167 ) ) ;
#37793=CARTESIAN_POINT ( 'NONE',  ( -7.483757832938788823, -7.479835662595867518, -3.861840502031824940 ) ) ;
#37794=CARTESIAN_POINT ( 'NONE',  ( 9.737435037572364394, 124.8671652961716489, 0.4371131421146306484 ) ) ;
#37797=EDGE_LOOP ( 'NONE', ( #12206, #37308, #31082, #4327 ) ) ;
#37802=EDGE_CURVE ( 'NONE', #34625, #32786, #25264, .T. ) ;
#37803=CARTESIAN_POINT ( 'NONE',  ( -16.06481930096632027, 121.2308719818149712, -0.1605585295567894255 ) ) ;
#37804=AXIS2_PLACEMENT_3D ( 'NONE', #36163, #13572, #29964 ) ;
#37805=ORIENTED_EDGE ( 'NONE', *, *, #28238, .F. ) ;
#37807=CARTESIAN_POINT ( 'NONE',  ( 6.887288372000457848, 121.6289117458970850, -0.4154818992412157019 ) ) ;
#37809=ORIENTED_EDGE ( 'NONE', *, *, #2569, .F. ) ;
#37810=CARTESIAN_POINT ( 'NONE',  ( 0.7417783677999320036, 115.6909491485452719, -1.732018146620468046 ) ) ;
#37811=CARTESIAN_POINT ( 'NONE',  ( -3.706155879762023098, 121.0264708767875561, -0.2234555574396432376 ) ) ;
#37812=CARTESIAN_POINT ( 'NONE',  ( 4.778253948640466042, -14.19231145175180231, 4.234097743872750286 ) ) ;
#37813=CARTESIAN_POINT ( 'NONE',  ( -12.48318382086466904, 120.3283006479967128, 0.8937555771000559313 ) ) ;
#37814=CARTESIAN_POINT ( 'NONE',  ( -6.573280687130626123E-14, 88.99346620154574339, 1.699031322814114629E-29 ) ) ;
#37815=CARTESIAN_POINT ( 'NONE',  ( 15.60991558517063815, 120.8175431576145940, 0.4704071646738435253 ) ) ;
#37816=CARTESIAN_POINT ( 'NONE',  ( 1.623171908765614901, 120.9965112475868096, 0.06597297138143794204 ) ) ;
#37818=CARTESIAN_POINT ( 'NONE',  ( 0.9750733387068674096, 18.20995955126885590, -0.03652159252302569076 ) ) ;
#37819=CARTESIAN_POINT ( 'NONE',  ( -15.52158573417678511, 120.7153972339879715, -0.3606909788719010468 ) ) ;
#37824=CARTESIAN_POINT ( 'NONE',  ( -2.917723067105041146, 117.2534023856253782, 0.5932563568887373462 ) ) ;
#37826=CARTESIAN_POINT ( 'NONE',  ( 14.28642979620150300, 121.5541609676003389, 1.504719748795722234 ) ) ;
#37828=CARTESIAN_POINT ( 'NONE',  ( 13.37375235405023588, 122.3357896625302459, -1.257830042033918128 ) ) ;
#37829=CARTESIAN_POINT ( 'NONE',  ( 1.466575460758787530, 20.86946789039323491, 8.308456332865098659 ) ) ;
#37830=CARTESIAN_POINT ( 'NONE',  ( -15.68124023389198385, 122.9504679175852573, -1.501494826411869932 ) ) ;
#37831=CARTESIAN_POINT ( 'NONE',  ( 4.902322516856424173, 117.7191841120239673, -0.7486650477168125262 ) ) ;
#37832=CARTESIAN_POINT ( 'NONE',  ( 5.211883163658348472, 116.1034411669277375, 1.237845179234434267 ) ) ;
#37835=CARTESIAN_POINT ( 'NONE',  ( -0.6395209782510218322, 120.9735524437166561, 0.05055770394172671295 ) ) ;
#37836=CARTESIAN_POINT ( 'NONE',  ( -12.03045567952079331, 122.8144071692085504, -1.784322758991244040 ) ) ;
#37838=CARTESIAN_POINT ( 'NONE',  ( 3.031078967112608158, -15.50598464685963584, 5.611516622434578494 ) ) ;
#37844=EDGE_LOOP ( 'NONE', ( #24738, #10369, #1917, #37405 ) ) ;
#37845=CARTESIAN_POINT ( 'NONE',  ( 18.63996327081343907, 147.1333978507680627, 2.447832456508666876 ) ) ;
#37846=CIRCLE ( 'NONE', #28990, 3.683000000000001162 ) ;
#37847=LINE ( 'NONE', #12070, #7952 ) ;
#37849=CARTESIAN_POINT ( 'NONE',  ( -1.135428393696731098, 110.6314368487224300, 3.415474402745806604 ) ) ;
#37850=B_SPLINE_CURVE_WITH_KNOTS ( 'NONE', 3,
 ( #20623, #36634, #11893, #22088, #8702, #18265, #18901, #9127, #21665, #28074, #24882, #21452, #2326, #31481, #12315, #35115, #34482, #2748, #41085, #37879, #31698, #14864, #15286, #5942, #31911, #15703, #5314, #28291, #34689, #1901, #25091, #41717, #25303, #5518, #31268, #18476 ),
 .UNSPECIFIED., .F., .F.,
 ( 4, 2, 2, 2, 2, 2, 2, 2, 2, 2, 2, 2, 2, 2, 2, 2, 2, 4 ),
 ( 0.02988307654956906881, 0.03083251118258813206, 0.03178194581560719878, 0.03273138044862625856, 0.03368081508164531834, 0.03463024971466438506, 0.03557968434768345178, 0.03652911898070251157, 0.03747855361372157829, 0.03842798824674063807, 0.03937742287975970479, 0.04032685751277876457, 0.04127629214579783129, 0.04222572677881689801, 0.04270044409532643137, 0.04317516141183595779, 0.04412459604485502451, 0.04507403067787408429 ),
 .UNSPECIFIED. ) ;
#37851=CARTESIAN_POINT ( 'NONE',  ( -6.736519641741455899, -9.595509028896938020, 5.111951147309959254 ) ) ;
#37852=CARTESIAN_POINT ( 'NONE',  ( 7.104091076028325347, 121.8059686962219672, 0.6844636119373688210 ) ) ;
#37853=CARTESIAN_POINT ( 'NONE',  ( -5.240108103846050192, 115.6909491485453003, -1.021770142138806792 ) ) ;
#37854=CARTESIAN_POINT ( 'NONE',  ( 7.827178552123568167, 158.6358315003295161, -0.5664908120210206954 ) ) ;
#37859=CARTESIAN_POINT ( 'NONE',  ( -4.117464183752013618, 118.2429491485453354, 0.1872741133385840973 ) ) ;
#37860=FACE_OUTER_BOUND ( 'NONE', #21485, .T. ) ;
#37861=ORIENTED_EDGE ( 'NONE', *, *, #42074, .T. ) ;
#37863=CARTESIAN_POINT ( 'NONE',  ( -8.238205950790057130, 120.2908699818124916, -1.444131204026530391 ) ) ;
#37864=CARTESIAN_POINT ( 'NONE',  ( 5.299048467822902175, 104.6144662015457527, -1.294354682138050050 ) ) ;
#37865=CARTESIAN_POINT ( 'NONE',  ( -1.678671165333144533, 156.3322054215483092, -0.6622483832023352557 ) ) ;
#37866=CARTESIAN_POINT ( 'NONE',  ( 4.907841372110366862, 117.4079477242360525, -0.9677383763118554416 ) ) ;
#37869=CARTESIAN_POINT ( 'NONE',  ( 0.4746723515649934888, 24.68197512780947278, 4.609222710213416896 ) ) ;
#37873=EDGE_CURVE ( 'NONE', #25568, #28106, #1131, .T. ) ;
#37874=CIRCLE ( 'NONE', #33114, 5.588000000000006295 ) ;
#37876=CARTESIAN_POINT ( 'NONE',  ( 7.785935935534881835, 122.6147637717617727, 0.2294641480035215786 ) ) ;
#37877=CARTESIAN_POINT ( 'NONE',  ( -4.580899860306842264, 27.87760619330545708, 0.5121266511161914892 ) ) ;
#37878=CARTESIAN_POINT ( 'NONE',  ( 16.43260349481032279, 122.7513851185756693, 1.135385547233646264 ) ) ;
#37879=CARTESIAN_POINT ( 'NONE',  ( 0.8484574697436598756, 104.6144662015457243, -4.760796931819447408 ) ) ;
#37880=CARTESIAN_POINT ( 'NONE',  ( 2.670684053127368784, -15.04618456763519241, 4.548342027319769443 ) ) ;
#37881=CARTESIAN_POINT ( 'NONE',  ( 1.249041419371635930, 159.0162744061759099, -1.301773431059132458 ) ) ;
#37882=CARTESIAN_POINT ( 'NONE',  ( -12.69375283655744724, 153.7453525671159298, 1.672805011026381017 ) ) ;
#37883=CARTESIAN_POINT ( 'NONE',  ( 4.466176584706416541, 22.48015689762229030, 1.290832665783417488 ) ) ;
#37884=CARTESIAN_POINT ( 'NONE',  ( -6.894332492628214126, 117.4533518774869947, -0.6472591412684409740 ) ) ;
#37885=CARTESIAN_POINT ( 'NONE',  ( 0.3177745610913299545, 14.38516025884261929, -0.9235644396001725376 ) ) ;
#37886=ORIENTED_EDGE ( 'NONE', *, *, #9514, .T. ) ;
#37888=CARTESIAN_POINT ( 'NONE',  ( -4.520495148373047556, 121.0527503406816123, 0.1761357111252132845 ) ) ;
#37889=CARTESIAN_POINT ( 'NONE',  ( 5.611934155553572445, -13.19144435144412064, 2.399925970747030846 ) ) ;
#37890=CARTESIAN_POINT ( 'NONE',  ( 16.77072586670511356, 146.3384789841921361, -1.111521918641044104 ) ) ;
#37891=ORIENTED_EDGE ( 'NONE', *, *, #29465, .T. ) ;
#37893=CARTESIAN_POINT ( 'NONE',  ( 1.287233266581064184, 115.7028696085538115, 1.739241353082145780 ) ) ;
#37896=CARTESIAN_POINT ( 'NONE',  ( -4.721710813556387443, 117.8486367688393557, -1.008509401085505575 ) ) ;
#37897=CARTESIAN_POINT ( 'NONE',  ( 9.001127587916124995, 123.9218113011205986, 0.09563458650452050236 ) ) ;
#37899=CARTESIAN_POINT ( 'NONE',  ( 12.76651978940611620, 122.1393999080170971, 1.787974849574114122 ) ) ;
#37900=DIRECTION ( 'NONE',  ( -0.9998004120163609398, -4.016384292689130894E-17, -0.01997839162482749689 ) ) ;
#37903=CARTESIAN_POINT ( 'NONE',  ( 0.02399864187730229442, 159.1630378086529731, -1.200990174154242141 ) ) ;
#37904=CIRCLE ( 'NONE', #12724, 0.5080000000000002292 ) ;
#37905=CARTESIAN_POINT ( 'NONE',  ( 15.31729018078742932, 120.6995131204970875, -0.01165691202436091103 ) ) ;
#37906=CARTESIAN_POINT ( 'NONE',  ( 0.06282972276035359016, 111.5577547982949227, -3.144256248693377387 ) ) ;
#37907=CARTESIAN_POINT ( 'NONE',  ( 1.796294892211930838, -15.43586790762843641, 5.400043117830624517 ) ) ;
#37910=CARTESIAN_POINT ( 'NONE',  ( -4.692573795977630802, 117.8898090967043402, 0.8100504932816339210 ) ) ;
#37912=ORIENTED_EDGE ( 'NONE', *, *, #3337, .F. ) ;
#37914=CARTESIAN_POINT ( 'NONE',  ( 5.858941820532026057, 118.8838138049209050, -1.014455745328361802 ) ) ;
#37915=CARTESIAN_POINT ( 'NONE',  ( -0.09082259786515388400, 105.9597790263619146, -5.306270932934927131 ) ) ;
#37916=CARTESIAN_POINT ( 'NONE',  ( 4.899517741242162217, 117.6566515308719829, 0.9517905942164465172 ) ) ;
#37918=CARTESIAN_POINT ( 'NONE',  ( -0.7687070661362833679, 118.7604188656930120, 0.8775891873661260112 ) ) ;
#37921=CARTESIAN_POINT ( 'NONE',  ( -4.774057941417253481, 114.7514248375596111, 1.662848932301731031 ) ) ;
#37922=DIRECTION ( 'NONE',  ( -4.017660918040594346E-17, 1.000000000000000000, 2.376309959284834438E-19 ) ) ;
#37923=CARTESIAN_POINT ( 'NONE',  ( 2.851896361732738860, -14.59419570037479019, 4.638016276237491020 ) ) ;
#37924=CARTESIAN_POINT ( 'NONE',  ( 7.563607548680719717, 124.2956292408697863, 0.1420234171030815562 ) ) ;
#37925=CARTESIAN_POINT ( 'NONE',  ( -11.90495122372371384, 153.4554508723442439, -1.948344234133813080 ) ) ;
#37926=CARTESIAN_POINT ( 'NONE',  ( 7.000096156874491271, 121.9564310754924321, 0.1322597535296755333 ) ) ;
#37927=CARTESIAN_POINT ( 'NONE',  ( -0.01632536679074437017, 38.84944212800221663, 1.323018725044087018 ) ) ;
#37928=CARTESIAN_POINT ( 'NONE',  ( -0.08720133927422249465, 115.7029491485439792, 1.760460350643238581 ) ) ;
#37929=CARTESIAN_POINT ( 'NONE',  ( 1.719524320724281852, 5.915668354077111779, 4.300554535892874064 ) ) ;
#37930=CARTESIAN_POINT ( 'NONE',  ( 22.52188062635569565, 150.6069110094195764, 1.039808695286016382 ) ) ;
#37932=CARTESIAN_POINT ( 'NONE',  ( -1.649594635467665826, 104.6144662015457527, -4.544680953048276351 ) ) ;
#37933=CARTESIAN_POINT ( 'NONE',  ( 3.954393197012034733, -15.56809308616131915, 2.853032214330836869 ) ) ;
#37934=CARTESIAN_POINT ( 'NONE',  ( -2.359155998022535172, 118.9063233352275972, 0.7056007782052504673 ) ) ;
#37935=CARTESIAN_POINT ( 'NONE',  ( -0.03357488772870852872, 24.54038786010652728, -0.9749811203568246043 ) ) ;
#37936=CARTESIAN_POINT ( 'NONE',  ( 0.1941685572964340079, 16.06069190514159928, 0.9568941237268799860 ) ) ;
#37937=ORIENTED_EDGE ( 'NONE', *, *, #5220, .F. ) ;
#37941=CARTESIAN_POINT ( 'NONE',  ( 3.617430929662223349, 113.7286232773062125, 2.299356966923025158 ) ) ;
#37943=CARTESIAN_POINT ( 'NONE',  ( -16.32790441640426238, 146.1553843108282820, 0.7912819366082540773 ) ) ;
#37946=CARTESIAN_POINT ( 'NONE',  ( 2.175557056806384448, -14.94057515128023539, 5.440454282391695706 ) ) ;
#37947=CARTESIAN_POINT ( 'NONE',  ( 7.718355369771759733, 156.1362479297160348, -1.656311413603696936 ) ) ;
#37948=CARTESIAN_POINT ( 'NONE',  ( -12.93098116229908001, 122.2940260782629451, -1.802317002068888785 ) ) ;
#37951=CARTESIAN_POINT ( 'NONE',  ( -15.72550100231863368, 145.6881679641610674, -0.3142329346387550681 ) ) ;
#37952=CARTESIAN_POINT ( 'NONE',  ( -4.970415085658511423, 32.57053289346710301, 3.417355655074298948 ) ) ;
#37953=CARTESIAN_POINT ( 'NONE',  ( 6.107944937931459428, 155.3491548655973133, -0.3423801154807229463 ) ) ;
#37955=CARTESIAN_POINT ( 'NONE',  ( 2.232013814210268343, -15.18320146713449148, 5.067049754691558050 ) ) ;
#37960=CARTESIAN_POINT ( 'NONE',  ( 3.573240411403531436, -4.819783300376494495, -2.961220487682876268 ) ) ;
#37961=CARTESIAN_POINT ( 'NONE',  ( 16.69533394573240770, 146.9696287467501179, 1.777152765835339876 ) ) ;
#37963=CARTESIAN_POINT ( 'NONE',  ( -5.736215069875440165, 118.4654530710369329, 0.4324765805296821308 ) ) ;
#37964=CARTESIAN_POINT ( 'NONE',  ( -2.983771112188844832, -5.329111280313512999, 3.548611825089460048 ) ) ;
#37965=CARTESIAN_POINT ( 'NONE',  ( 13.59117098933499790, 150.2425924485890505, 0.2715839415562140702 ) ) ;
#37966=CARTESIAN_POINT ( 'NONE',  ( -3.806420843250353681, -2.673146571556306750, -7.510622214715559686 ) ) ;
#37968=CARTESIAN_POINT ( 'NONE',  ( 5.541113904439527005, 116.8730092650452974, -0.3263445822601490076 ) ) ;
#37969=CARTESIAN_POINT ( 'NONE',  ( 0.04081796247057428717, 114.7739974199301969, -2.042697753608746059 ) ) ;
#37971=CARTESIAN_POINT ( 'NONE',  ( -4.873850642958228008, 32.38564726215445688, 3.744354677719523572 ) ) ;
#37972=CARTESIAN_POINT ( 'NONE',  ( -3.290491044589036740, 30.52917213649525507, -3.264312889705288878 ) ) ;
#37973=CARTESIAN_POINT ( 'NONE',  ( 3.153090565069621487, 117.9394477917076784, 1.303659228010183080 ) ) ;
#37974=CYLINDRICAL_SURFACE ( 'NONE', #4935, 5.334000000000001407 ) ;
#37976=CARTESIAN_POINT ( 'NONE',  ( 0.4103500344925852250, 124.0591982226670211, -0.08506156519360527635 ) ) ;
#37977=CARTESIAN_POINT ( 'NONE',  ( -14.51632629332725699, 120.3567457872619997, 0.2133257594814961799 ) ) ;
#37983=CARTESIAN_POINT ( 'NONE',  ( -15.26437740606669458, 148.0206351893604619, -0.2384670674966477832 ) ) ;
#37984=CARTESIAN_POINT ( 'NONE',  ( 2.643346398695107347, -15.60183157139904964, 5.704389875863137505 ) ) ;
#37985=CARTESIAN_POINT ( 'NONE',  ( -15.69714418277277268, 125.4375369430449609, 1.335551531390729130 ) ) ;
#37987=CARTESIAN_POINT ( 'NONE',  ( 12.68208805480593604, 156.8164516032445306, -1.015108139269342402 ) ) ;
#37988=CARTESIAN_POINT ( 'NONE',  ( 4.256838582791900194, 16.71066835407712858, 1.825063967593055558 ) ) ;
#37989=CARTESIAN_POINT ( 'NONE',  ( -5.687008767712567803, 159.1209727096294273, -0.4156250475054875659 ) ) ;
#37991=VERTEX_POINT ( 'NONE', #2106 ) ;
#37992=CARTESIAN_POINT ( 'NONE',  ( -5.562874253636517885, 116.7208863047924012, 0.03685954551894467940 ) ) ;
#37994=CARTESIAN_POINT ( 'NONE',  ( -10.76607124212195288, 123.2317624570580534, 1.067040512904773975 ) ) ;
#37996=CARTESIAN_POINT ( 'NONE',  ( 13.42639911875428815, 154.0568829568526041, -1.747011766586976655 ) ) ;
#37997=CARTESIAN_POINT ( 'NONE',  ( -1.123502178401431850, 117.8708904510121016, -0.6147983682407555106 ) ) ;
#37999=B_SPLINE_CURVE_WITH_KNOTS ( 'NONE', 3,
 ( #9734, #15690, #35732, #22702, #19518, #15901, #3357, #16324, #29327, #13350 ),
 .UNSPECIFIED., .F., .F.,
 ( 4, 2, 2, 2, 4 ),
 ( 1.172921298844514755E-05, 0.0004645486371682156618, 0.0006909583492580865160, 0.0008041632053030119956, 0.0009173680613479374751 ),
 .UNSPECIFIED. ) ;
#38001=CARTESIAN_POINT ( 'NONE',  ( 5.197063283114264465, 120.9449653624321144, -0.4048198106261541307 ) ) ;
#38002=ORIENTED_EDGE ( 'NONE', *, *, #31641, .T. ) ;
#38003=CARTESIAN_POINT ( 'NONE',  ( -17.63007963961423386, 148.6960320134204210, -2.325091492104032209 ) ) ;
#38004=CARTESIAN_POINT ( 'NONE',  ( 1.896617635523351053, -15.61750365820154052, 5.464805439086081407 ) ) ;
#38006=CARTESIAN_POINT ( 'NONE',  ( -4.160092557021775939, 118.2392543099457782, -0.3840812368330563942 ) ) ;
#38008=CARTESIAN_POINT ( 'NONE',  ( -4.980827880492125992, 117.4083494260662661, 0.8692259800077603016 ) ) ;
#38009=CARTESIAN_POINT ( 'NONE',  ( 10.58192191572908669, 122.8495954190337898, 1.525858888728604867 ) ) ;
#38011=CARTESIAN_POINT ( 'NONE',  ( 5.949252453048933909, -3.155934468320678921, 5.972130579448434951 ) ) ;
#38012=CARTESIAN_POINT ( 'NONE',  ( 15.41061421316642033, 147.8340308814284754, 0.6362464400602068082 ) ) ;
#38019=CARTESIAN_POINT ( 'NONE',  ( -7.889001465740365759, 122.0455370848547290, -0.9156369006618222395 ) ) ;
#38022=CARTESIAN_POINT ( 'NONE',  ( -5.797208421814709745, 116.9567987913546006, 0.006983082090869513134 ) ) ;
#38025=CARTESIAN_POINT ( 'NONE',  ( 6.006691951566636156, 121.4393142041827787, 0.03230195852056535338 ) ) ;
#38026=EDGE_CURVE ( 'NONE', #9800, #38197, #39900, .T. ) ;
#38029=CARTESIAN_POINT ( 'NONE',  ( 3.475237304863611154, 115.7029637511447646, -1.501298408546675178 ) ) ;
#38030=CARTESIAN_POINT ( 'NONE',  ( 0.002455802209154075121, 120.8958299794632438, -0.1228983847502210514 ) ) ;
#38031=CARTESIAN_POINT ( 'NONE',  ( 5.381753124113789255, -12.14417964010665330, 1.193960664996519094 ) ) ;
#38032=CARTESIAN_POINT ( 'NONE',  ( -21.94752568715520979, 149.4141677464492091, 1.146579238551070468 ) ) ;
#38034=CARTESIAN_POINT ( 'NONE',  ( 22.69169950426937987, 137.3157656003441787, 0.5971823736698287366 ) ) ;
#38035=CARTESIAN_POINT ( 'NONE',  ( 15.26171895222979735, 148.0206345167940469, 0.3715023683812953004 ) ) ;
#38037=CARTESIAN_POINT ( 'NONE',  ( -0.4212773433310383342, 21.23346528477927819, -0.8800754956890687319 ) ) ;
#38038=CARTESIAN_POINT ( 'NONE',  ( -5.748481425938979150, 159.1178304044242964, -0.1659167284945112786 ) ) ;
#38042=ORIENTED_EDGE ( 'NONE', *, *, #14937, .F. ) ;
#38043=CARTESIAN_POINT ( 'NONE',  ( -3.928350486978025469, 118.1770297339553366, 0.8034371862843084910 ) ) ;
#38045=CARTESIAN_POINT ( 'NONE',  ( 21.76696383529558432, 149.6930991844618291, 2.018179159957718127 ) ) ;
#38046=CARTESIAN_POINT ( 'NONE',  ( 20.20415560162845736, 149.0333503175929479, -1.664251383091793546 ) ) ;
#38047=CARTESIAN_POINT ( 'NONE',  ( -1.997604609866625580, -12.39122764300357105, -4.168859717980781809 ) ) ;
#38048=CARTESIAN_POINT ( 'NONE',  ( -17.34281104028706721, 125.1846915036903027, -1.498326104650645751 ) ) ;
#38049=CARTESIAN_POINT ( 'NONE',  ( 4.818088273131546195, 117.7361865335809483, -0.8720296992808537206 ) ) ;
#38051=CARTESIAN_POINT ( 'NONE',  ( 7.112984908206815504, 122.4243137415680280, 0.2517356677811186105 ) ) ;
#38052=CARTESIAN_POINT ( 'NONE',  ( -1.582738162022960804, 156.2580631240469415, 0.1078144505905373474 ) ) ;
#38053=CARTESIAN_POINT ( 'NONE',  ( -14.93497932922885596, 152.9649416503947634, -2.345758529409812443 ) ) ;
#38055=CARTESIAN_POINT ( 'NONE',  ( 5.672040739448011237, -14.80640238898532601, 2.735881018706089129 ) ) ;
#38057=CARTESIAN_POINT ( 'NONE',  ( -6.515206564940426254E-14, 69.43546620154573645, -8.744632320494937509E-18 ) ) ;
#38060=ORIENTED_EDGE ( 'NONE', *, *, #33646, .T. ) ;
#38061=CARTESIAN_POINT ( 'NONE',  ( 5.834721624102704673, 119.7498067647950961, 1.158144809029191924 ) ) ;
#38062=CARTESIAN_POINT ( 'NONE',  ( -6.566230858599542383E-14, 82.13546620154573930, -5.726718672203201028E-18 ) ) ;
#38064=CARTESIAN_POINT ( 'NONE',  ( -3.233068332335842676, 124.0549386377059307, -0.01378491165287840797 ) ) ;
#38065=CARTESIAN_POINT ( 'NONE',  ( 8.407117359195193984, -5.923529430292941989, 0.7350785369227282873 ) ) ;
#38066=CARTESIAN_POINT ( 'NONE',  ( 1.544162262333905522, 120.7289827521893670, 0.2751094044070052647 ) ) ;
#38067=CARTESIAN_POINT ( 'NONE',  ( -4.726878620523991437, 118.5930653697794384, -1.020485165756037205 ) ) ;
#38068=CARTESIAN_POINT ( 'NONE',  ( 13.22272649419657142, 119.7880570645780978, -0.3832108753485273245 ) ) ;
#38072=CARTESIAN_POINT ( 'NONE',  ( 8.797993348169676153, 117.6946419546766833, 0.07291966862306284436 ) ) ;
#38074=DIRECTION ( 'NONE',  ( -0.9998004120163610509, -4.016384292689131511E-17, -0.01997839162482749689 ) ) ;
#38077=CARTESIAN_POINT ( 'NONE',  ( -22.98488057257204886, 150.1591296352320910, -0.4592926148156235011 ) ) ;
#38078=VERTEX_POINT ( 'NONE', #34275 ) ;
#38081=CARTESIAN_POINT ( 'NONE',  ( 8.228572315554057326, 120.5845575724618186, -1.087623535237762784 ) ) ;
#38083=CARTESIAN_POINT ( 'NONE',  ( -0.6895396258586810045, 156.3865044363621450, -0.6062415235663758395 ) ) ;
#38084=DIRECTION ( 'NONE',  ( 0.9998004120163610509, 4.016384292689131511E-17, 0.01997839162482749689 ) ) ;
#38088=CARTESIAN_POINT ( 'NONE',  ( 4.573446973487649281, 17.56025517495590904, -0.6989348988664985107 ) ) ;
#38089=CARTESIAN_POINT ( 'NONE',  ( -5.285086173029821310, 105.1224018833269440, 0.7974957520148617807 ) ) ;
#38093=CARTESIAN_POINT ( 'NONE',  ( -7.787533413562373497, 122.6196154471950024, -0.09973116279183735777 ) ) ;
#38094=CARTESIAN_POINT ( 'NONE',  ( 4.518289034361447243, 23.24227448397437001, -0.9983406360900147769 ) ) ;
#38095=CARTESIAN_POINT ( 'NONE',  ( 17.89857548597107950, 125.1504969321615164, 1.218861057454597052 ) ) ;
#38097=CARTESIAN_POINT ( 'NONE',  ( 2.669030664778226480, -13.79969672238709499, -0.04828590215123814561 ) ) ;
#38098=CARTESIAN_POINT ( 'NONE',  ( 21.36781924117688192, 148.2102652567764380, -1.461444809879598017 ) ) ;
#38099=CARTESIAN_POINT ( 'NONE',  ( -7.441788261791943526, 120.6159063994810055, 0.9748553081951376598 ) ) ;
#38100=CARTESIAN_POINT ( 'NONE',  ( -4.621022795674669226, 27.76579825817536218, 0.1735962381356405959 ) ) ;
#38101=CARTESIAN_POINT ( 'NONE',  ( -7.798299699696711329, 158.6358315003295161, -0.8787250540639036656 ) ) ;
#38102=CARTESIAN_POINT ( 'NONE',  ( -0.5824522774871869757, -3.319493544524417583, -0.7801697309090062094 ) ) ;
#38105=CARTESIAN_POINT ( 'NONE',  ( -11.48476400923512131, 128.2561452373498980, 0.2810130423614018436 ) ) ;
#38106=CARTESIAN_POINT ( 'NONE',  ( 4.746351668907457189, -13.71804649124164222, 3.839566941389735977 ) ) ;
#38107=CARTESIAN_POINT ( 'NONE',  ( 9.584070499013346733, 122.7780075402122151, -0.8664194973949995715 ) ) ;
#38108=ORIENTED_EDGE ( 'NONE', *, *, #11578, .F. ) ;
#38109=CARTESIAN_POINT ( 'NONE',  ( 3.160156207961041019, 115.7029629711633021, 1.658234469206849804 ) ) ;
#38111=CARTESIAN_POINT ( 'NONE',  ( -4.861882094779772068, 117.7423377195431726, -0.9144347828526824262 ) ) ;
#38113=CARTESIAN_POINT ( 'NONE',  ( 10.40273896401435039, 153.1126597504080280, 0.1617772828476139180 ) ) ;
#38116=CARTESIAN_POINT ( 'NONE',  ( 4.978738709155149600, 118.8869175073591578, 1.099525347370199135 ) ) ;
#38117=FACE_OUTER_BOUND ( 'NONE', #16187, .T. ) ;
#38118=CARTESIAN_POINT ( 'NONE',  ( 4.801216665947148243, 117.4032681888235459, -1.015537427445656782 ) ) ;
#38119=CARTESIAN_POINT ( 'NONE',  ( 0.003073183581685161574, 116.5806198863164838, -0.1537946732117060067 ) ) ;
#38124=CARTESIAN_POINT ( 'NONE',  ( 1.720531155625569797, -15.47675250719444939, 5.459092711723419811 ) ) ;
#38126=CARTESIAN_POINT ( 'NONE',  ( 4.581716828367337513, -15.30239761468843973, -0.5121115983836379559 ) ) ;
#38127=CARTESIAN_POINT ( 'NONE',  ( -4.745831499507636941, 117.9479565618830463, 0.6405143620768928292 ) ) ;
#38130=CARTESIAN_POINT ( 'NONE',  ( 4.964802256754270893, 115.7029491485453150, -1.257203431686519712 ) ) ;
#38132=CARTESIAN_POINT ( 'NONE',  ( 8.484504387306683881, 119.3307393024920202, -1.028660563731210731 ) ) ;
#38133=CARTESIAN_POINT ( 'NONE',  ( -1.486515533886103801, 107.1743931308027129, -4.786382923486936392 ) ) ;
#38135=CARTESIAN_POINT ( 'NONE',  ( 4.773560218005917122, 117.6391202506862044, 1.128671190400995616 ) ) ;
#38137=CARTESIAN_POINT ( 'NONE',  ( -0.4220321208937833357, 124.6436471961814050, 0.02396868521112080139 ) ) ;
#38138=CARTESIAN_POINT ( 'NONE',  ( 4.560281875334545099, -11.68902278883368595, 0.6958564903332965512 ) ) ;
#38142=CARTESIAN_POINT ( 'NONE',  ( 3.722123463297008605, -13.62806973238828157, 3.608531954378976891 ) ) ;
#38143=CARTESIAN_POINT ( 'NONE',  ( 4.933025141171929029, 117.5302216577071874, -0.6666291745611303554 ) ) ;
#38144=CARTESIAN_POINT ( 'NONE',  ( -7.307041242074705956, 120.9764928074160082, -1.161154363956387492 ) ) ;
#38147=CARTESIAN_POINT ( 'NONE',  ( -0.8976751760525136792, 115.7028555646716370, 1.718879955640483015 ) ) ;
#38148=CARTESIAN_POINT ( 'NONE',  ( -0.8823465807374654135, 5.041073445128725794, 4.537322665494407659 ) ) ;
#38149=CARTESIAN_POINT ( 'NONE',  ( 6.903056240601945781, 117.3320596397172721, 0.5256612950045382870 ) ) ;
#38150=EDGE_LOOP ( 'NONE', ( #35106, #17861, #17758, #28343 ) ) ;
#38151=CARTESIAN_POINT ( 'NONE',  ( 4.130052816961541140, 104.6144662015457811, -2.503261204555655706 ) ) ;
#38152=CARTESIAN_POINT ( 'NONE',  ( 4.521904862512733381, -15.32733325190937990, -0.1948396341466702986 ) ) ;
#38153=CARTESIAN_POINT ( 'NONE',  ( -6.185003182635424146, 157.2590385278250267, 1.713690555389224324 ) ) ;
#38154=CARTESIAN_POINT ( 'NONE',  ( 0.05984739657028866761, 19.78266025878678391, 0.9748693421377304658 ) ) ;
#38155=CARTESIAN_POINT ( 'NONE',  ( -0.4793318477812648082, 11.74037758575859058, -0.8492235504747065455 ) ) ;
#38156=VERTEX_POINT ( 'NONE', #2945 ) ;
#38157=ORIENTED_EDGE ( 'NONE', *, *, #30316, .F. ) ;
#38159=CARTESIAN_POINT ( 'NONE',  ( 5.704032853997349939, 123.8402959710505087, 0.1558735912124265544 ) ) ;
#38161=CARTESIAN_POINT ( 'NONE',  ( -15.22619620759370918, 139.4722935914273307, 0.9828944228028649865 ) ) ;
#38162=CYLINDRICAL_SURFACE ( 'NONE', #19800, 0.5080000000000000071 ) ;
#38163=CARTESIAN_POINT ( 'NONE',  ( 3.475384634610537038, -12.95405113104661154, 1.817132104271814264 ) ) ;
#38164=CARTESIAN_POINT ( 'NONE',  ( 14.06576283519498460, 128.5416456306063253, -1.400350009575090038 ) ) ;
#38165=CARTESIAN_POINT ( 'NONE',  ( -20.12154232503860740, 149.0333503175929479, -2.470054797493931975 ) ) ;
#38168=CARTESIAN_POINT ( 'NONE',  ( 2.568134854143032442, -15.02010252187911554, 4.714990346623905815 ) ) ;
#38169=CARTESIAN_POINT ( 'NONE',  ( 4.074910602682932925, 118.2429491485453354, -0.1454311599470142491 ) ) ;
#38170=CARTESIAN_POINT ( 'NONE',  ( 15.87385217746171584, 146.2799285973741519, -0.1369075966739883299 ) ) ;
#38172=CARTESIAN_POINT ( 'NONE',  ( 2.664052010559913253, -13.52006206191685322, 0.08958796903007473778 ) ) ;
#38174=CIRCLE ( 'NONE', #39547, 3.683000000000001162 ) ;
#38177=CARTESIAN_POINT ( 'NONE',  ( -8.365627035046871995, 27.56796056798338057, -1.282220400777004388 ) ) ;
#38178=CARTESIAN_POINT ( 'NONE',  ( 8.539651237459528588, 154.7538831414287870, 1.439145765679522793 ) ) ;
#38179=DIRECTION ( 'NONE',  ( -0.9998004120163609398, -4.016384292689130894E-17, -0.01997839162482749689 ) ) ;
#38180=CARTESIAN_POINT ( 'NONE',  ( 21.67502463668045110, 132.7302833492884417, 0.4113505826877429938 ) ) ;
#38181=CARTESIAN_POINT ( 'NONE',  ( -5.187812668267249627, 115.4810986995850755, 1.301936727496811663 ) ) ;
#38182=CARTESIAN_POINT ( 'NONE',  ( 0.7336086519982951692, 0.2932837538699786251, -4.563195415240439701 ) ) ;
#38183=CARTESIAN_POINT ( 'NONE',  ( 7.783246152616065672, 154.6561476914895081, 0.1555277812256516956 ) ) ;
#38184=CARTESIAN_POINT ( 'NONE',  ( 5.585279946883024316, 5.098922668322787288, -6.300588543511215001 ) ) ;
#38185=CARTESIAN_POINT ( 'NONE',  ( 2.159339310776008602, 116.5957718504302818, -0.3424589834756739393 ) ) ;
#38186=CARTESIAN_POINT ( 'NONE',  ( -0.3562792453295428041, 120.3637084677653633, -0.5982640298941753754 ) ) ;
#38188=CARTESIAN_POINT ( 'NONE',  ( 0.1058213901577000071, 105.9761915687834772, -5.295735085524063024 ) ) ;
#38190=CARTESIAN_POINT ( 'NONE',  ( 1.523114390242035210, -9.429190846093893796, -8.291516064885865234 ) ) ;
#38192=CARTESIAN_POINT ( 'NONE',  ( 3.159224709476080140, 117.3993812142055191, 1.388978621109378198 ) ) ;
#38193=DIRECTION ( 'NONE',  ( -0.9998004120163609398, 0.000000000000000000, -0.01997839162482749342 ) ) ;
#38195=CARTESIAN_POINT ( 'NONE',  ( 0.3929232564620411261, 123.1683257372383054, -0.1777898040562596038 ) ) ;
#38196=CARTESIAN_POINT ( 'NONE',  ( -22.34885681094302967, 150.7328461917231550, 0.2743282927392731718 ) ) ;
#38197=VERTEX_POINT ( 'NONE', #22289 ) ;
#38202=CARTESIAN_POINT ( 'NONE',  ( -10.14111963374837444, 125.9557236484601361, -0.1537744135814335389 ) ) ;
#38203=CARTESIAN_POINT ( 'NONE',  ( 3.960108094477612806, -15.52904141176333930, 4.900792037362536213 ) ) ;
#38204=CARTESIAN_POINT ( 'NONE',  ( -20.05916364549921127, 149.8444905389382882, 1.617669260345511395 ) ) ;
#38205=CARTESIAN_POINT ( 'NONE',  ( 0.02156508032615568615, 159.2730288250082538, -1.079204802879467406 ) ) ;
#38206=CARTESIAN_POINT ( 'NONE',  ( 4.203610184846851894, 17.99761390031315500, -1.968029828111186319 ) ) ;
#38207=CARTESIAN_POINT ( 'NONE',  ( -23.23349130944704299, 142.6711341654318801, -0.9216821775544485895 ) ) ;
#38210=CARTESIAN_POINT ( 'NONE',  ( -0.09221630143976956850, 107.6766875080336376, 4.614880812453268533 ) ) ;
#38211=DIRECTION ( 'NONE',  ( -5.206863593109713661E-17, 1.000000000000000000, -1.077750396879097183E-30 ) ) ;
#38212=CARTESIAN_POINT ( 'NONE',  ( -17.22014391273219047, 144.2986879860016529, 1.480874425454277388 ) ) ;
#38213=DIRECTION ( 'NONE',  ( 0.9998004120163609398, 0.000000000000000000, 0.01997839162482749689 ) ) ;
#38214=CARTESIAN_POINT ( 'NONE',  ( 8.556073751109414260, 120.5511696877957775, -1.121754095281913388 ) ) ;
#38216=CARTESIAN_POINT ( 'NONE',  ( -15.09010836182855186, 154.7927800759015042, -2.085168164864714235 ) ) ;
#38218=CARTESIAN_POINT ( 'NONE',  ( 16.32790441640413093, 146.1553843108282820, -0.7912819366082538552 ) ) ;
#38219=EDGE_LOOP ( 'NONE', ( #6976, #11308, #18384, #35146 ) ) ;
#38220=CARTESIAN_POINT ( 'NONE',  ( -15.79265013068004109, 150.9007765090757971, -2.261858994468948225 ) ) ;
#38221=CARTESIAN_POINT ( 'NONE',  ( 1.871808270187516943, -15.45276866356297418, 5.379583495939216142 ) ) ;
#38223=CARTESIAN_POINT ( 'NONE',  ( -4.246385623344072435, 118.2248598242946827, -0.4674709900806769958 ) ) ;
#38224=CIRCLE ( 'NONE', #21189, 0.5080000000000002292 ) ;
#38226=CIRCLE ( 'NONE', #16340, 0.5080000000000002292 ) ;
#38227=CARTESIAN_POINT ( 'NONE',  ( -4.784818766354882236, 117.7320628736595012, 0.8970813257759844284 ) ) ;
#38228=CARTESIAN_POINT ( 'NONE',  ( 0.5205939700076258614, 119.6443647996702566, 0.5336935438815136878 ) ) ;
#38230=CARTESIAN_POINT ( 'NONE',  ( 0.8402904295469701967, 0.2923264105788614398, -8.379105243356319122 ) ) ;
#38231=CARTESIAN_POINT ( 'NONE',  ( 11.24781102592741355, 128.1602342495223468, 0.5025223919565851016 ) ) ;
#38234=ORIENTED_EDGE ( 'NONE', *, *, #16267, .F. ) ;
#38235=DIRECTION ( 'NONE',  ( 0.9998004120163610509, 4.016384292689131511E-17, 0.01997839162482749689 ) ) ;
#38238=CARTESIAN_POINT ( 'NONE',  ( -7.785313187783981626, 122.6175865491890420, -0.2316613915245773481 ) ) ;
#38241=CARTESIAN_POINT ( 'NONE',  ( -3.739900805225333524, 116.6566025657135413, 0.03821340562556417575 ) ) ;
#38244=CARTESIAN_POINT ( 'NONE',  ( 6.954509501169718000, 121.9349451668512927, -0.03177431777482942615 ) ) ;
#38245=CARTESIAN_POINT ( 'NONE',  ( -8.438003980598709930, 119.5616927475976894, 1.071839762751747749 ) ) ;
#38247=CARTESIAN_POINT ( 'NONE',  ( 2.441884256694776933, 115.7029470329614327, -1.605188886483090105 ) ) ;
#38248=CARTESIAN_POINT ( 'NONE',  ( -0.6475778113726436969, 156.3069099058775748, -0.1429049811405684878 ) ) ;
#38249=CARTESIAN_POINT ( 'NONE',  ( 4.090168366125579880, -14.63905918998462141, 5.005671547667302157 ) ) ;
#38250=CARTESIAN_POINT ( 'NONE',  ( -0.02615207601228260181, 159.0391464308674756, 1.308756824028193488 ) ) ;
#38253=CARTESIAN_POINT ( 'NONE',  ( 18.60568445592635456, 154.1511370093759865, 0.5871577710369986214 ) ) ;
#38254=CARTESIAN_POINT ( 'NONE',  ( 10.09730246939192178, 125.9371240743049611, 0.2994852486458426943 ) ) ;
#38256=CARTESIAN_POINT ( 'NONE',  ( 0.9048393610272945642, 9.142100508531621372, -0.3649321582425499311 ) ) ;
#38257=CARTESIAN_POINT ( 'NONE',  ( 0.0007535234281849903688, 116.4338605912342786, -0.03770939363766603186 ) ) ;
#38260=VERTEX_POINT ( 'NONE', #15909 ) ;
#38261=CARTESIAN_POINT ( 'NONE',  ( -2.285527320723312439, 116.3691792070813733, 0.1865855086054521439 ) ) ;
#38263=CARTESIAN_POINT ( 'NONE',  ( 1.109551233970408335, 117.7697124030934077, 0.5969493375118323231 ) ) ;
#38264=CARTESIAN_POINT ( 'NONE',  ( 0.01111639779256734344, 118.2594330468507593, -0.5563100024230162033 ) ) ;
#38265=CARTESIAN_POINT ( 'NONE',  ( -6.300109353874518980, 26.68925120273002705, -5.586516568188822696 ) ) ;
#38266=CARTESIAN_POINT ( 'NONE',  ( -15.04114430247513035, 121.6710330000183546, -1.338242383117114853 ) ) ;
#38267=CARTESIAN_POINT ( 'NONE',  ( 4.839331864970178643, 117.8306479882070050, -0.7070860029426544457 ) ) ;
#38268=CARTESIAN_POINT ( 'NONE',  ( 5.328278062782956681, 116.9387654363850260, 0.9571818161585843310 ) ) ;
#38269=AXIS2_PLACEMENT_3D ( 'NONE', #12801, #34991, #24961 ) ;
#38270=CARTESIAN_POINT ( 'NONE',  ( -15.28485850284635283, 148.0141687878753203, -0.07717638215565292281 ) ) ;
#38271=CARTESIAN_POINT ( 'NONE',  ( -17.07725563869816199, 135.3907879583883869, -2.389267674572352451 ) ) ;
#38272=CARTESIAN_POINT ( 'NONE',  ( 3.960108094477612806, -15.52904141176333930, 4.900792037362536213 ) ) ;
#38274=CARTESIAN_POINT ( 'NONE',  ( -4.771503349878651434, 117.9496054766768225, -1.116523703797990263 ) ) ;
#38275=EDGE_LOOP ( 'NONE', ( #29572, #18196, #8735, #22321 ) ) ;
#38276=CARTESIAN_POINT ( 'NONE',  ( 8.000928410381797917, 156.3870133935118076, 2.044342179695390893 ) ) ;
#38277=DIRECTION ( 'NONE',  ( 4.017660918040594346E-17, -1.000000000000000000, -2.376309959284834438E-19 ) ) ;
#38278=DIRECTION ( 'NONE',  ( -0.9998004120163608288, 0.000000000000000000, -0.01997839162482749342 ) ) ;
#38280=CARTESIAN_POINT ( 'NONE',  ( -1.397093717039429972, 113.6455945353133643, 2.337579097500038561 ) ) ;
#38281=CARTESIAN_POINT ( 'NONE',  ( -8.384998746481384657, -10.44493509673469767, 0.7792886224267949746 ) ) ;
#38282=CARTESIAN_POINT ( 'NONE',  ( 1.678671165333015747, 156.3322054215483092, 0.6622483832023354777 ) ) ;
#38283=CARTESIAN_POINT ( 'NONE',  ( 15.09612904044924697, 120.9194639129320734, -0.3833380168901105445 ) ) ;
#38286=CARTESIAN_POINT ( 'NONE',  ( 8.798547045555515922, 117.6874503704031127, 0.1190114001730665366 ) ) ;
#38287=EDGE_CURVE ( 'NONE', #3139, #7830, #18819, .T. ) ;
#38289=CIRCLE ( 'NONE', #6332, 5.334000000000001407 ) ;
#38290=CARTESIAN_POINT ( 'NONE',  ( -22.66375647020928952, 150.6386093215955100, -0.4528757910175258972 ) ) ;
#38292=CARTESIAN_POINT ( 'NONE',  ( -6.379245509003030890, 120.1349722450784725, -1.192449620425102941 ) ) ;
#38293=CARTESIAN_POINT ( 'NONE',  ( 5.336610043934060243, 104.6144662015457527, -0.07732958313162717479 ) ) ;
#38294=CARTESIAN_POINT ( 'NONE',  ( -8.816380758798688433, 123.2701452714374568, -0.6637701367642925288 ) ) ;
#38296=CARTESIAN_POINT ( 'NONE',  ( 22.53492722140441629, 150.7843406352268687, 0.4757920170715053132 ) ) ;
#38298=CARTESIAN_POINT ( 'NONE',  ( -3.158589313471108273, 4.191505055319898254, 3.400481138232230194 ) ) ;
#38300=CARTESIAN_POINT ( 'NONE',  ( -1.421603664355800101, 159.6054662015457666, -0.02840702444251828190 ) ) ;
#38303=CARTESIAN_POINT ( 'NONE',  ( -6.064067160211926932, 121.4300801654758146, 0.02073022162667565588 ) ) ;
#38304=CARTESIAN_POINT ( 'NONE',  ( 1.677595020332960152, 24.74158224480939339, -4.309653081027373211 ) ) ;
#38305=CARTESIAN_POINT ( 'NONE',  ( 9.554367121731589307, 118.3624989119526418, 0.8896461348445369177 ) ) ;
#38308=CARTESIAN_POINT ( 'NONE',  ( 4.024684254631489821, 117.9114980025989752, -0.7134393008021913118 ) ) ;
#38310=CARTESIAN_POINT ( 'NONE',  ( -11.32523555543272487, 123.0403929720162495, 1.197004354367268153 ) ) ;
#38311=CARTESIAN_POINT ( 'NONE',  ( -4.384008014420753163, 17.61986127277741332, -1.463615122064717111 ) ) ;
#38312=CARTESIAN_POINT ( 'NONE',  ( -3.843811238687901533, 117.0275016673472663, -0.5328274117395519482 ) ) ;
#38315=CARTESIAN_POINT ( 'NONE',  ( -0.8659212883131867100, -1.167510040683709560, 0.4517697218592801600 ) ) ;
#38318=CARTESIAN_POINT ( 'NONE',  ( -7.078188358610653985, 121.9740017686541194, 0.1969649471280498776 ) ) ;
#38319=CARTESIAN_POINT ( 'NONE',  ( 5.778079093609060024, -12.78747091716041240, 1.651671850763037463 ) ) ;
#38320=CARTESIAN_POINT ( 'NONE',  ( 12.96210878518737708, 128.4900567078429390, -1.108396809849303777 ) ) ;
#38323=CARTESIAN_POINT ( 'NONE',  ( -4.903208392033640450, 117.6536421438997451, -0.9409563386690815712 ) ) ;
#38324=EDGE_CURVE ( 'NONE', #36953, #4283, #31727, .T. ) ;
#38325=CARTESIAN_POINT ( 'NONE',  ( 0.0005468344958423734022, 156.3034662015456604, -0.02736583427618467443 ) ) ;
#38327=CARTESIAN_POINT ( 'NONE',  ( 17.65052098649041667, 151.6044147853587845, 2.418251502674879649 ) ) ;
#38328=DIRECTION ( 'NONE',  ( -0.9998004120163609398, 0.000000000000000000, -0.01997839162482749689 ) ) ;
#38329=DIRECTION ( 'NONE',  ( -0.9998004120163608288, 0.000000000000000000, -0.01997839162482749342 ) ) ;
#38331=CARTESIAN_POINT ( 'NONE',  ( 23.32076472591247196, 148.8446908248229477, 0.1342014517686429820 ) ) ;
#38332=CARTESIAN_POINT ( 'NONE',  ( 0.07157677169882613322, 110.3683645023726569, -3.581994345755985076 ) ) ;
#38336=CARTESIAN_POINT ( 'NONE',  ( 1.736649427362045861, -15.40716104390517316, 5.430039758140377870 ) ) ;
#38338=FACE_OUTER_BOUND ( 'NONE', #5363, .T. ) ;
#38340=TOROIDAL_SURFACE ( 'NONE', #19963, 5.080000000000005400, 0.5080000000000000071 ) ;
#38341=CARTESIAN_POINT ( 'NONE',  ( -4.575171740070761217, 118.0742775853333768, 0.6029512648002022246 ) ) ;
#38342=VERTEX_POINT ( 'NONE', #6347 ) ;
#38344=CARTESIAN_POINT ( 'NONE',  ( -5.913856609602897940, 119.1282656376870364, -1.263485629223820794 ) ) ;
#38345=CARTESIAN_POINT ( 'NONE',  ( -5.397835693418398861, 119.2618716387835747, -0.5632668535983702540 ) ) ;
#38346=CARTESIAN_POINT ( 'NONE',  ( 4.625168964342468492, 117.9841153801070561, 0.8982682689321210834 ) ) ;
#38347=CARTESIAN_POINT ( 'NONE',  ( 2.857130780617909149, -14.87311083204414786, 4.269097905712053276 ) ) ;
#38348=CARTESIAN_POINT ( 'NONE',  ( -0.3869134157277939190, 116.4813942609866899, 1.514588684444738709 ) ) ;
#38353=CARTESIAN_POINT ( 'NONE',  ( 6.476067766296546679, 120.6581566633936404, -0.1355830077277814794 ) ) ;
#38354=CARTESIAN_POINT ( 'NONE',  ( -10.68802918394767687, 123.5542795626547417, -1.432819001183019969 ) ) ;
#38356=CARTESIAN_POINT ( 'NONE',  ( 16.18905205736044906, 121.2598130428683447, 0.3234957879086921562 ) ) ;
#38357=CARTESIAN_POINT ( 'NONE',  ( -6.003866115224264277, 28.47055935836900176, 0.6261310066654243167 ) ) ;
#38358=CARTESIAN_POINT ( 'NONE',  ( -3.961103147347932119, 115.7035856650175418, 1.436382292835700625 ) ) ;
#38359=CARTESIAN_POINT ( 'NONE',  ( 4.364008504204949013, 7.202613900313124873, 1.580794030135405537 ) ) ;
#38360=CARTESIAN_POINT ( 'NONE',  ( 15.70934801585141116, 121.2535323456646523, 0.8362899507430230361 ) ) ;
#38362=CARTESIAN_POINT ( 'NONE',  ( 0.9340703678216289996, 104.6144662015456674, -5.263168525813664900 ) ) ;
#38364=CARTESIAN_POINT ( 'NONE',  ( 2.947576629936649706, -15.31278845794613375, 4.223034005107467515 ) ) ;
#38365=CARTESIAN_POINT ( 'NONE',  ( -0.03256023585726924852, 157.9544661776888290, 1.629447346748784664 ) ) ;
#38366=CARTESIAN_POINT ( 'NONE',  ( -0.8940008744714061928, 26.26452439613007428, -0.3861867617640990513 ) ) ;
#38367=CARTESIAN_POINT ( 'NONE',  ( -0.8857237343455648393, 3.096269703755229141, -0.4102451188256627801 ) ) ;
#38370=DIRECTION ( 'NONE',  ( -0.9998004120163608288, -4.016384292689131511E-17, -0.01997839162482749342 ) ) ;
#38371=CARTESIAN_POINT ( 'NONE',  ( 3.281580062219306093, 118.9685052735122355, 0.6847577310700790898 ) ) ;
#38373=CARTESIAN_POINT ( 'NONE',  ( -5.197063283114393251, 120.9449653624321144, 0.4048198106261542417 ) ) ;
#38374=CARTESIAN_POINT ( 'NONE',  ( -15.21351360038775802, 143.4186079242255119, -0.3040022078858783949 ) ) ;
#38375=CARTESIAN_POINT ( 'NONE',  ( 3.260250311156894121, -12.89034478651954174, 1.323980178024680043 ) ) ;
#38376=CARTESIAN_POINT ( 'NONE',  ( 2.123774309200863630, 157.0334531201187644, -1.456117127909798192 ) ) ;
#38378=CARTESIAN_POINT ( 'NONE',  ( -20.22999339756081838, 148.7458375694471044, -2.474301912364147871 ) ) ;
#38380=CARTESIAN_POINT ( 'NONE',  ( 8.631261618837783089, 118.4117623764986007, 1.057671270618954829 ) ) ;
#38381=CARTESIAN_POINT ( 'NONE',  ( -3.044072069279135206, 34.44269722464345307, 3.574075509920750626 ) ) ;
#38382=EDGE_CURVE ( 'NONE', #6660, #21896, #42136, .T. ) ;
#38383=CARTESIAN_POINT ( 'NONE',  ( 8.625872078176229252, 123.3364012560002578, -0.04702935286775003498 ) ) ;
#38385=CARTESIAN_POINT ( 'NONE',  ( 0.1058213901578615862, 105.9761915687788729, -5.295735085525930863 ) ) ;
#38387=CARTESIAN_POINT ( 'NONE',  ( 4.867434175510519268, 117.7629967458994287, 0.8046164465094345353 ) ) ;
#38390=CARTESIAN_POINT ( 'NONE',  ( -7.817010796087602742, 17.61996943312679775, -3.135079784279759085 ) ) ;
#38391=CARTESIAN_POINT ( 'NONE',  ( 15.81386139960065051, 149.2064892436030163, 1.885719434888957879 ) ) ;
#38393=CARTESIAN_POINT ( 'NONE',  ( 20.69945920510660997, 152.5542719854981044, 0.3887601451951304132 ) ) ;
#38394=CARTESIAN_POINT ( 'NONE',  ( -2.162697817503842934, 106.7001829816230725, 4.879784414745867771 ) ) ;
#38396=B_SPLINE_CURVE_WITH_KNOTS ( 'NONE', 3,
 ( #6352, #6986, #39357, #9745, #16119, #12936, #22502, #182, #26144, #13362, #10161, #35532 ),
 .UNSPECIFIED., .F., .F.,
 ( 4, 1, 1, 1, 1, 1, 1, 1, 1, 4 ),
 ( 0.5426758968252777260, 0.5876249999999998419, 0.6700999999999999179, 0.7525749999999999940, 0.7938125000000000320, 0.8350499999999998479, 0.8762874999999994419, 0.9175249999999994799, 0.9587624999999999620, 0.9957666935384927864 ),
 .UNSPECIFIED. ) ;
#38398=CARTESIAN_POINT ( 'NONE',  ( 1.562757238090025202, 156.2577446057484281, 0.06075558507430143390 ) ) ;
#38399=CARTESIAN_POINT ( 'NONE',  ( 11.89465070410498093, 120.7721054874162974, 1.583610710261881049 ) ) ;
#38400=CARTESIAN_POINT ( 'NONE',  ( -5.729511908840139611, -2.247816343263548511, -6.181412921048518250 ) ) ;
#38401=CARTESIAN_POINT ( 'NONE',  ( 5.511179323772147143, 117.2417087625145626, -0.6038106809302513645 ) ) ;
#38402=CARTESIAN_POINT ( 'NONE',  ( -0.3561418115365337367, 119.9741034315941732, -0.6738560125758273900 ) ) ;
#38404=LINE ( 'NONE', #18991, #32549 ) ;
#38405=CARTESIAN_POINT ( 'NONE',  ( 2.306944209869228768, 107.0587059723494860, -4.722744024792687512 ) ) ;
#38406=CARTESIAN_POINT ( 'NONE',  ( -4.212901951478492890, -8.356617434558033963, -7.328762184035659821 ) ) ;
#38407=CARTESIAN_POINT ( 'NONE',  ( 0.7953399164170903424, 117.3993835805238035, 1.485889010799970489 ) ) ;
#38408=CARTESIAN_POINT ( 'NONE',  ( -4.854186777038641765, 117.7557277303023966, -0.9091791526384296329 ) ) ;
#38409=CARTESIAN_POINT ( 'NONE',  ( 2.827333099181600584, -13.37427733298611443, 0.6166582517569209054 ) ) ;
#38410=CARTESIAN_POINT ( 'NONE',  ( 0.1065646865914870178, 105.8844662015456919, -5.332932678536313809 ) ) ;
#38411=CARTESIAN_POINT ( 'NONE',  ( -15.19762206999210186, 120.8830733721255370, 0.2994679608661980907 ) ) ;
#38416=CARTESIAN_POINT ( 'NONE',  ( 2.105506875138051459, -15.57594099408041188, 5.887502213194136580 ) ) ;
#38417=CARTESIAN_POINT ( 'NONE',  ( -6.741874166124567580, 157.8130281244853279, 1.606654124060122424 ) ) ;
#38418=CARTESIAN_POINT ( 'NONE',  ( 5.873718653373081189, 117.7475948868982698, -0.6546600694323944092 ) ) ;
#38419=CARTESIAN_POINT ( 'NONE',  ( 4.326043401919948295, 8.289558097378858292, -1.648119079657388353 ) ) ;
#38423=CARTESIAN_POINT ( 'NONE',  ( -0.005099097581101574329, 122.5569158606516993, 0.2551796940110860890 ) ) ;
#38424=DIRECTION ( 'NONE',  ( 0.9998004120163609398, 4.016384292689130894E-17, 0.01997839162482749689 ) ) ;
#38425=CARTESIAN_POINT ( 'NONE',  ( -12.26974321764567932, 126.0625018263836807, 1.123002009909297660 ) ) ;
#38427=CARTESIAN_POINT ( 'NONE',  ( 8.076210525097339499, 156.3870133935118076, -1.723082682300313806 ) ) ;
#38428=CARTESIAN_POINT ( 'NONE',  ( -20.60480707444014570, 141.5323519391372997, -2.354057365763566168 ) ) ;
#38430=CARTESIAN_POINT ( 'NONE',  ( 8.149220328376060252, 154.6259123219959690, -0.6607633090041662438 ) ) ;
#38432=CARTESIAN_POINT ( 'NONE',  ( -17.44789039799423591, 148.6234142586927476, -2.276312578826294342 ) ) ;
#38433=CARTESIAN_POINT ( 'NONE',  ( 3.716361853963529249, -15.42594482578084403, 2.788391211141477921 ) ) ;
#38434=CARTESIAN_POINT ( 'NONE',  ( -4.229144778596610976, 118.2245657482411474, -0.4851207049587970555 ) ) ;
#38437=EDGE_CURVE ( 'NONE', #38156, #450, #30273, .T. ) ;
#38438=CARTESIAN_POINT ( 'NONE',  ( -4.937121216058332429, 117.6323291441971861, 0.7898849711784506900 ) ) ;
#38439=CARTESIAN_POINT ( 'NONE',  ( 14.65736332902321060, 131.2156652454908112, 2.020252246219832681 ) ) ;
#38441=CARTESIAN_POINT ( 'NONE',  ( 6.518667233416390872, -10.50300228728784901, -5.332001816399940530 ) ) ;
#38442=CARTESIAN_POINT ( 'NONE',  ( 3.721623402434252714, 121.0563512343167645, 0.1807651092205457555 ) ) ;
#38451=CARTESIAN_POINT ( 'NONE',  ( -23.17968947452053996, 149.6103952014060212, -0.1325215592567119405 ) ) ;
#38454=CARTESIAN_POINT ( 'NONE',  ( -5.981523321826031747, 121.4283444620903367, -0.2204012826164671313 ) ) ;
#38455=CARTESIAN_POINT ( 'NONE',  ( 4.828520450080895365, 117.4049894591484673, -1.009733177510003799 ) ) ;
#38456=ORIENTED_EDGE ( 'NONE', *, *, #16476, .F. ) ;
#38457=CARTESIAN_POINT ( 'NONE',  ( 0.9904753432905314403, 115.7029491485453008, -1.712273171734945976 ) ) ;
#38458=CARTESIAN_POINT ( 'NONE',  ( -9.115443861534034298, 124.0847320388339625, -0.2671161660598813103 ) ) ;
#38459=CARTESIAN_POINT ( 'NONE',  ( 4.834931622272050866, -13.60668467239417545, 3.655623996717635382 ) ) ;
#38460=CARTESIAN_POINT ( 'NONE',  ( -1.113991634874509806, 117.6437429425539420, 0.5281592773360505033 ) ) ;
#38462=CARTESIAN_POINT ( 'NONE',  ( 23.08789804466225704, 149.8924475812327159, 0.6911741358207285080 ) ) ;
#38463=CARTESIAN_POINT ( 'NONE',  ( 5.334492475561027902, 121.3506618966597728, 0.2156469154756605611 ) ) ;
#38465=CARTESIAN_POINT ( 'NONE',  ( 0.9253733321238560849, 8.064964547470342637, 0.3089666344597190029 ) ) ;
#38466=CARTESIAN_POINT ( 'NONE',  ( -15.93236088550710861, 121.0320206851898206, -0.3693416020086464080 ) ) ;
#38470=CARTESIAN_POINT ( 'NONE',  ( 2.362235608990936431, 116.5348030743598287, 0.3959731454556020824 ) ) ;
#38472=CARTESIAN_POINT ( 'NONE',  ( 9.211590693262500906, 119.0402042963619351, 1.266790605762086575 ) ) ;
#38473=CARTESIAN_POINT ( 'NONE',  ( 10.16662615958531291, 120.4647147465577461, -1.171017801134732084 ) ) ;
#38474=CARTESIAN_POINT ( 'NONE',  ( 8.270632439779459943, 13.09856730479051912, 1.690137114335896751 ) ) ;
#38475=CARTESIAN_POINT ( 'NONE',  ( -14.52885936862958793, 121.1548589120785095, -1.307706137645302302 ) ) ;
#38476=CARTESIAN_POINT ( 'NONE',  ( 4.691175111891225491, 117.9633576474440986, -0.7151038522473830428 ) ) ;
#38477=CARTESIAN_POINT ( 'NONE',  ( 7.694725746745239015, 124.7202454748262710, 0.1536377669325636464 ) ) ;
#38478=CARTESIAN_POINT ( 'NONE',  ( -15.54908666625173730, 147.5346097818530211, -0.08167737433607544228 ) ) ;
#38479=CARTESIAN_POINT ( 'NONE',  ( -17.96932707993158473, 150.0321773811041339, -2.460285709456810022 ) ) ;
#38481=CARTESIAN_POINT ( 'NONE',  ( 6.046978665186544255, -14.69723126592269224, 0.3844556930898083702 ) ) ;
#38483=EDGE_CURVE ( 'NONE', #32528, #33565, #24797, .T. ) ;
#38486=CARTESIAN_POINT ( 'NONE',  ( 18.13772925547819170, 148.8986565181125457, 2.425799293919265853 ) ) ;
#38489=CARTESIAN_POINT ( 'NONE',  ( -3.904686386324561997, 121.5791280715047122, 0.1678698840778540258 ) ) ;
#38490=CARTESIAN_POINT ( 'NONE',  ( 6.343129774801278487, 27.92810111164739340, -5.540698593559898910 ) ) ;
#38491=CARTESIAN_POINT ( 'NONE',  ( 10.15204665306222687, 124.8647468421599598, 0.8418846390287858528 ) ) ;
#38493=CARTESIAN_POINT ( 'NONE',  ( 0.3417028577847283088, 116.8490449975401617, -0.2775575361029120613 ) ) ;
#38496=B_SPLINE_CURVE_WITH_KNOTS ( 'NONE', 3,
 ( #25370, #38374, #15562, #35175, #10168, #22144, #22352, #6002, #3805, #18964, #39364, #31971, #28774, #23137, #41363, #36175, #16767, #35377 ),
 .UNSPECIFIED., .F., .F.,
 ( 4, 1, 1, 1, 1, 1, 2, 1, 1, 1, 2, 1, 1, 4 ),
 ( 0.000000000000000000, 0.1631003137318065010, 0.3262006274636130021, 0.4077507843295162804, 0.4893009411954195031, 0.5708510980613228369, 0.6524012549272261152, 0.6576100072399927443, 0.6628187595527594844, 0.6680275118655262245, 0.6732362641782929646, 0.7053937736304702888, 0.7375512830826476129, 0.7543499533659702161 ),
 .UNSPECIFIED. ) ;
#38498=CARTESIAN_POINT ( 'NONE',  ( -16.86202032626315628, 155.2029898760372646, -0.3369432954968343275 ) ) ;
#38499=EDGE_LOOP ( 'NONE', ( #40523, #34582, #21884, #39340 ) ) ;
#38500=CARTESIAN_POINT ( 'NONE',  ( -8.208076046625514266, 120.4389588540418714, -1.432247049196957667 ) ) ;
#38502=CARTESIAN_POINT ( 'NONE',  ( -15.44906575790740888, 148.0679034673509875, -1.029643479621237256 ) ) ;
#38504=CARTESIAN_POINT ( 'NONE',  ( 23.11076619426176393, 149.9001102426712748, 0.4874744954944871811 ) ) ;
#38506=CARTESIAN_POINT ( 'NONE',  ( -3.366035089439492811, 13.68705809737886447, 3.178168622443589886 ) ) ;
#38508=CARTESIAN_POINT ( 'NONE',  ( -15.19604463793445959, 156.0859089222169587, -0.3036531364422413448 ) ) ;
#38509=FACE_OUTER_BOUND ( 'NONE', #16776, .T. ) ;
#38511=CARTESIAN_POINT ( 'NONE',  ( 6.989499183820137240, 121.3060156903671043, 0.9293008224528782613 ) ) ;
#38512=CARTESIAN_POINT ( 'NONE',  ( -3.128764270554720728, 7.249652477310866594, -3.416742352092642321 ) ) ;
#38513=CARTESIAN_POINT ( 'NONE',  ( 20.32146383345304130, 132.1502320877631007, 1.598207211936853556 ) ) ;
#38515=CARTESIAN_POINT ( 'NONE',  ( 3.075357915497110017, -13.94103813162880989, 1.416127232796946966 ) ) ;
#38516=CARTESIAN_POINT ( 'NONE',  ( 20.89924265627218603, 149.3152741295656369, -1.514357740512880968 ) ) ;
#38517=CARTESIAN_POINT ( 'NONE',  ( -11.83945725349124878, 123.3160021321619695, 1.255757047829674011 ) ) ;
#38518=CARTESIAN_POINT ( 'NONE',  ( -3.469956624915944587, 9.623539240006554252, 3.074419811715999984 ) ) ;
#38519=CARTESIAN_POINT ( 'NONE',  ( -22.70904429024585980, 149.7444054411783441, -1.421740456058895985 ) ) ;
#38520=ORIENTED_EDGE ( 'NONE', *, *, #9741, .F. ) ;
#38522=CARTESIAN_POINT ( 'NONE',  ( -15.86984883002240387, 146.9522167609303267, 0.2762592943789939914 ) ) ;
#38523=CARTESIAN_POINT ( 'NONE',  ( 5.936869294410564990, -12.97241973064336484, 1.608696005067407953 ) ) ;
#38525=CARTESIAN_POINT ( 'NONE',  ( -4.563637803650490099, 118.0730259387059391, -0.7686314647840511993 ) ) ;
#38526=B_SPLINE_CURVE_WITH_KNOTS ( 'NONE', 3,
 ( #37140, #23702, #20721, #1369 ),
 .UNSPECIFIED., .F., .F.,
 ( 4, 4 ),
 ( 0.001532986024144806884, 0.001758754979876016875 ),
 .UNSPECIFIED. ) ;
#38527=CARTESIAN_POINT ( 'NONE',  ( 5.308493528853203358, 121.3525139070573147, 0.1060763342189517539 ) ) ;
#38530=CARTESIAN_POINT ( 'NONE',  ( 12.43266001442890278, 122.1796674805547980, 1.793313828261402287 ) ) ;
#38532=DIRECTION ( 'NONE',  ( 0.01997839162482749689, 1.040247600000945640E-18, -0.9998004120163610509 ) ) ;
#38533=CARTESIAN_POINT ( 'NONE',  ( -0.006370369177395581589, 117.0014201992989058, 0.3187993231787208948 ) ) ;
#38534=CARTESIAN_POINT ( 'NONE',  ( 4.971096433842443041, 117.4753406598250223, -0.8637816793092503165 ) ) ;
#38535=MANIFOLD_SOLID_BREP ( 'Stock-MAS-162-1', #26468 ) ;
#38536=CARTESIAN_POINT ( 'NONE',  ( 8.206428610460235973, 117.5568930537867800, -0.09596530983984018215 ) ) ;
#38537=DIRECTION ( 'NONE',  ( 0.9998004120163608288, 0.000000000000000000, 0.01997839162482736852 ) ) ;
#38540=CARTESIAN_POINT ( 'NONE',  ( 1.964815052535200168, -15.28087767662020191, 5.362322688996490783 ) ) ;
#38542=PLANE ( 'NONE',  #10462 ) ;
#38543=CIRCLE ( 'NONE', #9301, 3.683000000000001162 ) ;
#38544=CARTESIAN_POINT ( 'NONE',  ( -4.620544706279255287, 118.0223899981905618, 0.6740461278582655646 ) ) ;
#38546=ORIENTED_EDGE ( 'NONE', *, *, #32124, .T. ) ;
#38547=VERTEX_POINT ( 'NONE', #14214 ) ;
#38549=CARTESIAN_POINT ( 'NONE',  ( -5.896308022760929468, 119.0874697000712388, -1.261715751646591999 ) ) ;
#38550=CARTESIAN_POINT ( 'NONE',  ( -4.040061035763231168, 117.6466181296975151, -0.9125624508345165919 ) ) ;
#38551=CARTESIAN_POINT ( 'NONE',  ( 4.780600333925313805, 117.8746637532869670, 0.8584492858400551984 ) ) ;
#38553=CARTESIAN_POINT ( 'NONE',  ( -12.30032609686878153, 128.4316967252784991, -1.345898664372764175 ) ) ;
#38554=CARTESIAN_POINT ( 'NONE',  ( -3.601659165084134973, 115.7029493297849285, -1.622342836042594216 ) ) ;
#38555=CARTESIAN_POINT ( 'NONE',  ( -3.222237999455158430, 108.4800421235064363, 4.089189990378621964 ) ) ;
#38557=CARTESIAN_POINT ( 'NONE',  ( 4.473299935328610033, 111.2795884869231173, -2.951234740152492986 ) ) ;
#38558=CARTESIAN_POINT ( 'NONE',  ( -1.975234429548569537, 156.8313070664539168, -1.415192030232628850 ) ) ;
#38559=DIRECTION ( 'NONE',  ( -0.9998004120163608288, 0.000000000000000000, -0.01997839162482749342 ) ) ;
#38561=CARTESIAN_POINT ( 'NONE',  ( -2.569109746590555687, 115.7029491485453150, 1.594660097005825117 ) ) ;
#38562=CARTESIAN_POINT ( 'NONE',  ( -4.374560056058969693, 13.03735028915297534, 1.504755201125916875 ) ) ;
#38563=CARTESIAN_POINT ( 'NONE',  ( 23.01936977803462625, 148.9204423966469335, 1.315221278248082548 ) ) ;
#38565=CARTESIAN_POINT ( 'NONE',  ( 0.9339135649851527665, 105.1229431022307779, -5.262705770857304621 ) ) ;
#38566=CARTESIAN_POINT ( 'NONE',  ( 3.824421424077324883, -15.38127155850414773, 2.203493915304267858 ) ) ;
#38567=CARTESIAN_POINT ( 'NONE',  ( -14.55733092780593019, 125.6573275863457866, 1.461954306844538864 ) ) ;
#38568=CARTESIAN_POINT ( 'NONE',  ( 0.6142125404598580696, 23.44653936994281906, -0.7587870835084352672 ) ) ;
#38570=CARTESIAN_POINT ( 'NONE',  ( -0.2244654480080381653, 11.31155722793083918, -0.9512810396025579429 ) ) ;
#38571=ORIENTED_EDGE ( 'NONE', *, *, #20697, .T. ) ;
#38575=CARTESIAN_POINT ( 'NONE',  ( 6.294717182677755041, 121.9812576474260055, 0.2818399057506481009 ) ) ;
#38576=CARTESIAN_POINT ( 'NONE',  ( -12.09414715658302875, 128.3964238929853252, 0.7197952935306337618 ) ) ;
#38578=CARTESIAN_POINT ( 'NONE',  ( 3.537338181458673070, -13.91857904597952533, 4.048280000481319973 ) ) ;
#38579=CARTESIAN_POINT ( 'NONE',  ( 10.94646760555348308, 123.1276765127550021, -1.119819633367153067 ) ) ;
#38580=CIRCLE ( 'NONE', #27680, 5.080000000000006288 ) ;
#38581=CARTESIAN_POINT ( 'NONE',  ( -8.716850226171729332, 156.9002828235886966, -2.058648441535007478 ) ) ;
#38583=ADVANCED_FACE ( 'NONE', ( #33836 ), #4664, .T. ) ;
#38584=CARTESIAN_POINT ( 'NONE',  ( 8.060526367258390223, 121.1727610582439780, 1.293028985890418925 ) ) ;
#38585=CARTESIAN_POINT ( 'NONE',  ( -5.478259115505812460, 32.09053017494222360, 1.574172154844436289 ) ) ;
#38586=CARTESIAN_POINT ( 'NONE',  ( 15.60869185768498113, 147.5518517437054982, -0.1389895172399196188 ) ) ;
#38592=EDGE_CURVE ( 'NONE', #7084, #27091, #24427, .T. ) ;
#38593=CARTESIAN_POINT ( 'NONE',  ( -8.398906084147393258, 18.04027321918359306, -0.8732425085428288103 ) ) ;
#38594=CARTESIAN_POINT ( 'NONE',  ( 5.862724111891608025, 121.1554468101848130, 0.6631653705238501617 ) ) ;
#38595=CARTESIAN_POINT ( 'NONE',  ( -6.637366883016756296E-14, 101.1854662015457365, -1.207165459283692464E-19 ) ) ;
#38596=CARTESIAN_POINT ( 'NONE',  ( 23.11138188961074746, 149.8995197111492814, 0.3848215369211052117 ) ) ;
#38597=CARTESIAN_POINT ( 'NONE',  ( -5.927223324825597217, 118.9825038774357466, 0.3493763292145123378 ) ) ;
#38598=AXIS2_PLACEMENT_3D ( 'NONE', #3959, #4166, #30130 ) ;
#38599=CARTESIAN_POINT ( 'NONE',  ( -3.682264917456323783, 82.64346620154573486, -0.07358041635423923088 ) ) ;
#38600=CARTESIAN_POINT ( 'NONE',  ( 0.02537255736346739551, 39.20946620154573026, -1.269746523260778970 ) ) ;
#38601=CARTESIAN_POINT ( 'NONE',  ( 20.78747236883564398, 145.7124547906547889, 2.408930808681182256 ) ) ;
#38603=CARTESIAN_POINT ( 'NONE',  ( 6.343129774801278487, 27.92810111164739340, -5.540698593559898910 ) ) ;
#38604=CARTESIAN_POINT ( 'NONE',  ( 8.753617840798051830, 117.9548258552378002, -0.3763906928539145214 ) ) ;
#38605=CARTESIAN_POINT ( 'NONE',  ( 0.1065646865915095692, 105.8844662015456919, -5.332932678536313809 ) ) ;
#38608=CARTESIAN_POINT ( 'NONE',  ( -3.347088983057015632, 104.6144662015458096, 3.489637925356170456 ) ) ;
#38609=CARTESIAN_POINT ( 'NONE',  ( 0.9564925537785137211, 29.00497265395555857, -4.523030980006896407 ) ) ;
#38610=PLANE ( 'NONE',  #37526 ) ;
#38612=CARTESIAN_POINT ( 'NONE',  ( 2.569204629087775693, -14.95572128602136530, 4.738577790166504933 ) ) ;
#38613=EDGE_CURVE ( 'NONE', #19493, #41093, #20748, .T. ) ;
#38614=CARTESIAN_POINT ( 'NONE',  ( 1.593197492609314647, 110.3135721340718334, -3.506749948187484200 ) ) ;
#38615=CARTESIAN_POINT ( 'NONE',  ( -0.9832365512849939870, 116.8374933757159795, 0.2893350595372073952 ) ) ;
#38618=CARTESIAN_POINT ( 'NONE',  ( 5.028141926494226865, 117.3993840561512485, -0.6263463072690832467 ) ) ;
#38622=CARTESIAN_POINT ( 'NONE',  ( 4.515093156845158440, -15.50826969562475810, 4.181389551362865831 ) ) ;
#38623=CARTESIAN_POINT ( 'NONE',  ( -10.28923284337283661, 120.3038588096988803, 1.141564125291498311 ) ) ;
#38624=CARTESIAN_POINT ( 'NONE',  ( 0.3839177515434519794, 117.3568105388816321, -0.4297925318014834684 ) ) ;
#38626=CARTESIAN_POINT ( 'NONE',  ( 4.513502956352341222, 8.064680226961385756, -0.9949261897555528034 ) ) ;
#38630=CARTESIAN_POINT ( 'NONE',  ( -0.01254005783545543429, 120.1716774721351157, 0.6275557724548022076 ) ) ;
#38631=CARTESIAN_POINT ( 'NONE',  ( -4.747830334022490106, 117.7228629901014614, 0.9149653662667899257 ) ) ;
#38632=CARTESIAN_POINT ( 'NONE',  ( -17.30282355392138172, 146.5563353440282981, 1.366477706345458287 ) ) ;
#38633=CARTESIAN_POINT ( 'NONE',  ( 5.138887090645153144, 116.8853669287380797, 0.2852080145627308716 ) ) ;
#38634=CARTESIAN_POINT ( 'NONE',  ( 18.16172641238590657, 140.6071502257508143, -1.752259283733317297 ) ) ;
#38635=CARTESIAN_POINT ( 'NONE',  ( -20.83122434882630003, 148.6614476615901594, -2.397187407820276395 ) ) ;
#38639=CARTESIAN_POINT ( 'NONE',  ( 9.542276680740265249, 123.9284174147966269, -0.4124357159827418684 ) ) ;
#38641=CARTESIAN_POINT ( 'NONE',  ( -3.383623802199918984, 119.6896249646678569, -0.8128912582704552747 ) ) ;
#38642=CARTESIAN_POINT ( 'NONE',  ( 3.491209331645790837, -14.97137451562302601, 1.144833103274278230 ) ) ;
#38643=DIRECTION ( 'NONE',  ( 0.9998004120163610509, 4.016384292689131511E-17, 0.01997839162482749689 ) ) ;
#38645=CARTESIAN_POINT ( 'NONE',  ( -4.781588677966720269, 117.7629110891638362, 0.8765192077237911050 ) ) ;
#38646=CARTESIAN_POINT ( 'NONE',  ( 12.10021064141416502, 153.5325627063460843, 2.025425248842404269 ) ) ;
#38647=CARTESIAN_POINT ( 'NONE',  ( -0.7387659178326326792, 32.94979111317254450, 0.8178967711910595240 ) ) ;
#38648=CARTESIAN_POINT ( 'NONE',  ( -4.460028654926622593, 22.53297844546955631, 1.214995109042491528 ) ) ;
#38649=CARTESIAN_POINT ( 'NONE',  ( 8.124409605001838841, 122.8458379852381910, 0.3720714147651332793 ) ) ;
#38653=ADVANCED_FACE ( 'NONE', ( #39492 ), #14015, .T. ) ;
#38657=CARTESIAN_POINT ( 'NONE',  ( -8.232873692804936638, 120.3172065538984015, -1.441392283162307830 ) ) ;
#38661=CARTESIAN_POINT ( 'NONE',  ( -3.277668934457586669, 159.4655167044000166, 0.1355973003551880496 ) ) ;
#38664=CARTESIAN_POINT ( 'NONE',  ( -6.954920274790141299, 121.9415326885807929, -0.2649906444065315281 ) ) ;
#38667=CARTESIAN_POINT ( 'NONE',  ( 0.7269968954376242465, 115.7031256804406780, -1.730797724436444307 ) ) ;
#38668=CARTESIAN_POINT ( 'NONE',  ( -15.64343260727715013, 147.2205073051419504, -0.4407941163815355390 ) ) ;
#38669=CARTESIAN_POINT ( 'NONE',  ( 3.596007053926196573, -14.96754207850672991, 5.407624617413868684 ) ) ;
#38670=CARTESIAN_POINT ( 'NONE',  ( -13.76672422736547396, 155.7522398296385404, 1.402631553274309439 ) ) ;
#38672=CARTESIAN_POINT ( 'NONE',  ( 18.63890302240343999, 125.2334963081946313, 0.6306532867605573189 ) ) ;
#38673=EDGE_CURVE ( 'NONE', #30834, #20737, #13966, .T. ) ;
#38674=CARTESIAN_POINT ( 'NONE',  ( 2.863236596730719619, 121.0282055654512163, 0.1599167813194848631 ) ) ;
#38675=CARTESIAN_POINT ( 'NONE',  ( 4.844094425375155666, 115.6909491485453145, -1.283570666956070694 ) ) ;
#38676=CARTESIAN_POINT ( 'NONE',  ( -0.4248780512631177841, 5.470267980206036107, 0.8793239699972363876 ) ) ;
#38677=CARTESIAN_POINT ( 'NONE',  ( -23.10027255048459693, 149.8968678342272653, -0.6153025774343640064 ) ) ;
#38680=EDGE_LOOP ( 'NONE', ( #29075, #9233, #7151, #30653 ) ) ;
#38681=CARTESIAN_POINT ( 'NONE',  ( -2.485165897956930880, 116.7121408797957400, 0.3916859838625323387 ) ) ;
#38684=CARTESIAN_POINT ( 'NONE',  ( 3.034986042679733487, 117.6993298527280984, 0.7527370910433335283 ) ) ;
#38685=CARTESIAN_POINT ( 'NONE',  ( 8.792132358471045350, 156.9002828235886966, -1.708777300431143509 ) ) ;
#38686=CARTESIAN_POINT ( 'NONE',  ( 4.144591825430580911, 15.01708852069707945, -7.363685156706923252 ) ) ;
#38687=CARTESIAN_POINT ( 'NONE',  ( -5.210988722241271631, 158.8115599018184412, -1.325654878232527478 ) ) ;
#38688=CARTESIAN_POINT ( 'NONE',  ( 4.674864129759326303, 117.9626304797967720, -0.7310746242011807450 ) ) ;
#38689=CARTESIAN_POINT ( 'NONE',  ( 15.47023807670824525, 120.6682698389898576, 0.3091321738930620788 ) ) ;
#38690=CARTESIAN_POINT ( 'NONE',  ( -8.507314851146933421, 123.3280575159016905, -0.1373787248657619975 ) ) ;
#38691=CARTESIAN_POINT ( 'NONE',  ( -0.9722352627953847470, 157.7941190989783991, -1.644571785473255998 ) ) ;
#38692=CARTESIAN_POINT ( 'NONE',  ( 2.911953930276938607, -15.74143402046077078, 5.333341296191352221 ) ) ;
#38696=CARTESIAN_POINT ( 'NONE',  ( 11.80606196054485579, 122.9427978038690270, 1.750206178813383806 ) ) ;
#38701=CARTESIAN_POINT ( 'NONE',  ( -4.022785008251061889, 122.0441497943765370, 0.1183375255305478546 ) ) ;
#38702=CARTESIAN_POINT ( 'NONE',  ( 8.340720164204880049, -15.19402286670749191, -1.049415519506536665 ) ) ;
#38703=CARTESIAN_POINT ( 'NONE',  ( 10.85076598842368334, 126.1616406593870607, 0.8982697194533709739 ) ) ;
#38704=CARTESIAN_POINT ( 'NONE',  ( 2.917496378899068432, 117.0242007548465608, -0.3950530357975749474 ) ) ;
#38707=CARTESIAN_POINT ( 'NONE',  ( -23.36108720469573186, 148.8745345081378559, -0.4410421544236567959 ) ) ;
#38709=CARTESIAN_POINT ( 'NONE',  ( 8.198008058078954718, 120.7314922977370912, -1.065926864482704683 ) ) ;
#38710=CARTESIAN_POINT ( 'NONE',  ( 5.586884702347365561, 75.27746620154573520, 0.1116392523995368286 ) ) ;
#38711=CARTESIAN_POINT ( 'NONE',  ( -15.93611381433512264, 145.8030804522035737, -1.048911189365803631 ) ) ;
#38713=CARTESIAN_POINT ( 'NONE',  ( 23.45208337669170007, 146.8499405026647651, 0.4686284387228156212 ) ) ;
#38716=CARTESIAN_POINT ( 'NONE',  ( 2.003160574663116034, 15.61121511114846960, 4.187759092076685619 ) ) ;
#38717=CARTESIAN_POINT ( 'NONE',  ( -23.34372044207216845, 149.0681261006882039, -0.4664630893996629113 ) ) ;
#38718=CARTESIAN_POINT ( 'NONE',  ( -4.901945799063080145, 117.4108088126838112, 0.9677811563769884717 ) ) ;
#38721=CARTESIAN_POINT ( 'NONE',  ( 5.726410507774571279, 120.0273765416552578, 1.077413901059734114 ) ) ;
#38723=CARTESIAN_POINT ( 'NONE',  ( -0.5507456681092424144, 15.89564879194059799, -4.587442282481805300 ) ) ;
#38724=CARTESIAN_POINT ( 'NONE',  ( 10.35357550766347678, 157.8614378686282862, 1.168524991271691738 ) ) ;
#38725=DIRECTION ( 'NONE',  ( -4.017660918040594346E-17, 1.000000000000000000, 2.376309959284834438E-19 ) ) ;
#38726=CARTESIAN_POINT ( 'NONE',  ( 3.543852116809842467, 109.5877551946028632, 3.777766483051805846 ) ) ;
#38727=CARTESIAN_POINT ( 'NONE',  ( 20.68240061501449389, 141.5323519391372997, -1.529040698034871637 ) ) ;
#38729=CARTESIAN_POINT ( 'NONE',  ( -0.5165578309945342284, 6.287656885725535716, -4.620190224396742984 ) ) ;
#38730=CARTESIAN_POINT ( 'NONE',  ( -6.888626713468250173, 117.5201695557886410, -0.7016588733424086177 ) ) ;
#38732=CARTESIAN_POINT ( 'NONE',  ( -11.98620439842969887, 151.9649008058812569, 0.3157042427443432775 ) ) ;
#38733=CARTESIAN_POINT ( 'NONE',  ( 5.096701352355580639, -14.12304281641942083, 3.871056799387667002 ) ) ;
#38735=CARTESIAN_POINT ( 'NONE',  ( -4.537028399616379382, 118.0323947479856770, -0.8637156260805385344 ) ) ;
#38736=CARTESIAN_POINT ( 'NONE',  ( 15.72781737677511593, 145.6903699455376113, 0.2627434299976846854 ) ) ;
#38738=CARTESIAN_POINT ( 'NONE',  ( 8.716850226171599658, 156.9002828235886966, 2.058648441535007922 ) ) ;
#38741=CARTESIAN_POINT ( 'NONE',  ( -22.70688998881783505, 149.0844379882532849, 0.7271790501850814437 ) ) ;
#38742=CARTESIAN_POINT ( 'NONE',  ( 4.815708689467896875, 117.5416844730284680, -0.9797437855538944085 ) ) ;
#38744=CARTESIAN_POINT ( 'NONE',  ( 13.30261597551684360, 156.9705208988102640, -0.2305920065817561315 ) ) ;
#38749=CARTESIAN_POINT ( 'NONE',  ( 1.877026549479959172, -15.08352304062032800, 5.583147605863830520 ) ) ;
#38752=CARTESIAN_POINT ( 'NONE',  ( -4.614943955948183074, 118.0411468392323400, 0.6409247712607968328 ) ) ;
#38756=CARTESIAN_POINT ( 'NONE',  ( -0.7730009467963616654, 115.6909491485452435, -1.757285791594641822 ) ) ;
#38757=CARTESIAN_POINT ( 'NONE',  ( -8.352514336526260408, 119.7346528407997255, -1.431646670230054541 ) ) ;
#38758=CARTESIAN_POINT ( 'NONE',  ( -5.553235467069472797, 117.9513286348681476, -0.7459228754688890239 ) ) ;
#38759=CARTESIAN_POINT ( 'NONE',  ( 4.623035167900726883, 118.0214275984946113, 0.8252090714975102159 ) ) ;
#38760=CARTESIAN_POINT ( 'NONE',  ( 3.212496809824684441, -14.25148094350509353, 2.370051959060230473 ) ) ;
#38761=CARTESIAN_POINT ( 'NONE',  ( -11.38067935084468552, 126.1532465342912985, -1.245950066931532874 ) ) ;
#38762=CARTESIAN_POINT ( 'NONE',  ( -2.906692822798004006, 115.7029491485453576, -1.674875336659100489 ) ) ;
#38764=CARTESIAN_POINT ( 'NONE',  ( -6.439703808512989190E-14, 63.33946620154573282, 4.464395889055755859E-29 ) ) ;
#38765=CARTESIAN_POINT ( 'NONE',  ( 5.398477100378374693, 117.1940586887245388, -0.6826447346010610095 ) ) ;
#38766=CARTESIAN_POINT ( 'NONE',  ( -16.41634355132965695, 139.9843038322558186, -2.146987391100668496 ) ) ;
#38768=CARTESIAN_POINT ( 'NONE',  ( -0.01289612358334801118, 159.5048567107479585, 0.6453747585945883714 ) ) ;
#38770=CARTESIAN_POINT ( 'NONE',  ( -2.948169924849943335, 1.592661447142720732, -3.562413953034572867 ) ) ;
#38771=CARTESIAN_POINT ( 'NONE',  ( 1.907136510351249870, 116.7789519286944966, 0.3469662120689608886 ) ) ;
#38772=ORIENTED_EDGE ( 'NONE', *, *, #26151, .F. ) ;
#38774=CARTESIAN_POINT ( 'NONE',  ( 2.939911579247540541, -15.51555475658629391, 4.434558482745560859 ) ) ;
#38775=CARTESIAN_POINT ( 'NONE',  ( -19.35587726549920262, 148.6897983921382433, 1.735459330159159208 ) ) ;
#38776=CARTESIAN_POINT ( 'NONE',  ( -0.2928493810785644524, 9.627489959316354984, 0.9317482488014678932 ) ) ;
#38777=CARTESIAN_POINT ( 'NONE',  ( -0.9401033786448180773, 4.191251494893229790, 0.2723526238743522732 ) ) ;
#38782=CARTESIAN_POINT ( 'NONE',  ( -0.1065646865916382163, 105.8844662015457061, 5.332932678536314697 ) ) ;
#38784=CARTESIAN_POINT ( 'NONE',  ( -4.453624852893828034, 120.7762672505206041, 0.3811677228292795205 ) ) ;
#38785=CARTESIAN_POINT ( 'NONE',  ( 4.304563788583176454, -12.55325912034982494, 2.095985231258857162 ) ) ;
#38786=CARTESIAN_POINT ( 'NONE',  ( 13.85457725998112011, 128.5353789189983900, -1.357273257441080849 ) ) ;
#38787=CARTESIAN_POINT ( 'NONE',  ( -4.389113801267393811, 157.7533977378147654, -1.847790720561485411 ) ) ;
#38788=DIRECTION ( 'NONE',  ( -4.017660918040594346E-17, 1.000000000000000000, 2.376309959284834438E-19 ) ) ;
#38789=CARTESIAN_POINT ( 'NONE',  ( 8.243466591241450203, 120.2651585749115668, 1.445033792603914513 ) ) ;
#38790=CARTESIAN_POINT ( 'NONE',  ( -5.541434792369814843, 31.48360339932893126, -0.006023868707823998130 ) ) ;
#38791=CARTESIAN_POINT ( 'NONE',  ( 9.165091971927566306, 123.9989874199980022, -0.04717021870285740409 ) ) ;
#38793=DIRECTION ( 'NONE',  ( 1.254648257879299356E-08, -1.000000000000000000, 2.507086335409856190E-10 ) ) ;
#38795=CARTESIAN_POINT ( 'NONE',  ( -4.583145339712576316, 27.87760190724945275, 0.5120832130390071679 ) ) ;
#38796=CARTESIAN_POINT ( 'NONE',  ( 11.02756477914268629, 153.1537610418535849, 1.395931567138233298 ) ) ;
#38798=CARTESIAN_POINT ( 'NONE',  ( 1.417759636995359784, 159.6040221172770259, -0.05833233067434073077 ) ) ;
#38799=CARTESIAN_POINT ( 'NONE',  ( -5.274668375481318172, 116.0897965414613964, 1.029904101180854514 ) ) ;
#38800=CIRCLE ( 'NONE', #20415, 0.5080000000000002292 ) ;
#38803=CARTESIAN_POINT ( 'NONE',  ( -3.257474687714740913, 31.88364938939399096, 0.8587021535642015424 ) ) ;
#38804=CARTESIAN_POINT ( 'NONE',  ( 20.39340916383837055, 150.0074677946399504, 2.333577254436574044 ) ) ;
#38805=CARTESIAN_POINT ( 'NONE',  ( -4.282102574861781363, 27.11529131024228434, -1.748715980913516876 ) ) ;
#38806=CARTESIAN_POINT ( 'NONE',  ( 7.184910528696541121, -14.53812136005497280, -4.413989948622978332 ) ) ;
#38807=CARTESIAN_POINT ( 'NONE',  ( -2.164707726640842544, 116.7454174419857935, -0.4974148364468519712 ) ) ;
#38808=CARTESIAN_POINT ( 'NONE',  ( -1.507062556099493245, 116.9323294830472122, -1.352967057238088300 ) ) ;
#38809=CARTESIAN_POINT ( 'NONE',  ( -23.29144772315980916, 149.3526176766912101, -0.4654185560736369132 ) ) ;
#38810=CARTESIAN_POINT ( 'NONE',  ( 1.151906140154263847, 104.6144662015478843, 5.219791793463544494 ) ) ;
#38811=CARTESIAN_POINT ( 'NONE',  ( -4.191205975170537279, 21.45845178295031630, -1.961646697876042511 ) ) ;
#38814=CARTESIAN_POINT ( 'NONE',  ( 3.197553254331486183, -13.99644925588092192, 2.254757065552156714 ) ) ;
#38817=EDGE_CURVE ( 'NONE', #929, #10591, #30301, .T. ) ;
#38818=CARTESIAN_POINT ( 'NONE',  ( 1.559908931542361099, 116.9323294830472122, -1.291681667928520794 ) ) ;
#38819=CARTESIAN_POINT ( 'NONE',  ( -23.05353557640037820, 148.9204423966469335, 0.3945749818456248392 ) ) ;
#38823=CARTESIAN_POINT ( 'NONE',  ( -3.148524768479886937, 30.89467502894793327, -0.4672404312464801812 ) ) ;
#38824=CARTESIAN_POINT ( 'NONE',  ( 5.741009826001572947, -15.03722989464144355, 1.207582410354154145 ) ) ;
#38825=CARTESIAN_POINT ( 'NONE',  ( -0.03067001211942338088, 158.6015251912307633, 1.534852821454057770 ) ) ;
#38827=CARTESIAN_POINT ( 'NONE',  ( 2.090077592200443313, 117.5043770775735510, -0.5427014567576282644 ) ) ;
#38828=CARTESIAN_POINT ( 'NONE',  ( 4.586363120317823672, -1.655842793181455663, -0.6244342276643227718 ) ) ;
#38830=VERTEX_POINT ( 'NONE', #12149 ) ;
#38832=CARTESIAN_POINT ( 'NONE',  ( 0.3558893179480882574, 120.1716774721349168, 0.6349178681961805681 ) ) ;
#38833=B_SPLINE_SURFACE_WITH_KNOTS ( 'NONE', 1, 3, ( 
 ( #11402, #14380, #5041, #37189, #30994, #14799, #7811, #18201, #18413, #17996, #10990, #40195, #37810, #24389, #27389, #20773, #8211, #5453 ),
 ( #1835, #21598, #1423, #31202, #30584, #31420, #27802, #23972, #24595, #34626, #11194, #37394, #40810, #15010, #14588, #11611, #33797, #21183 ) ),
 .UNSPECIFIED., .F., .F., .F.,
 ( 2, 2 ),
 ( 4, 2, 2, 2, 2, 2, 2, 2, 4 ),
 ( 0.000000000000000000, 1.000000000000000000 ),
 ( 0.000000000000000000, 0.2500000000000000000, 0.5000000000000000000, 0.6250000000000000000, 0.7500000000000000000, 0.8125000000000000000, 0.8750000000000000000, 0.9375000000000000000, 1.000000000000000000 ),
 .UNSPECIFIED. ) ;
#38834=CARTESIAN_POINT ( 'NONE',  ( -10.62684080304162393, 123.4307455932968765, 0.9978443992970126297 ) ) ;
#38836=CARTESIAN_POINT ( 'NONE',  ( 11.99432760026347466, 123.0912118827050108, -1.285395851362399755 ) ) ;
#38838=CARTESIAN_POINT ( 'NONE',  ( -20.91256836843385614, 148.0559997909317644, -2.401931445155506939 ) ) ;
#38841=CARTESIAN_POINT ( 'NONE',  ( 4.459839028410091721, 118.1598638495170377, -0.4314496914423903151 ) ) ;
#38842=CARTESIAN_POINT ( 'NONE',  ( 0.01133107913638646547, 156.3792106723807649, -0.5670535347366656431 ) ) ;
#38844=CARTESIAN_POINT ( 'NONE',  ( -2.483060992037719572, 119.7126118883416410, -0.6995635895845424557 ) ) ;
#38845=CARTESIAN_POINT ( 'NONE',  ( 3.489657270499090025, -15.47349394630789732, 3.491754635552897668 ) ) ;
#38847=CARTESIAN_POINT ( 'NONE',  ( -6.591743005429100447E-14, 88.48546620154573361, -4.217761848057333172E-18 ) ) ;
#38848=CARTESIAN_POINT ( 'NONE',  ( -4.865414317926856747, 117.7603977766165571, 0.7856990298424358921 ) ) ;
#38849=CARTESIAN_POINT ( 'NONE',  ( 9.877803879600188353, 122.5082557396031291, 1.415055850893564449 ) ) ;
#38851=CIRCLE ( 'NONE', #30034, 3.175000000000001155 ) ;
#38852=CARTESIAN_POINT ( 'NONE',  ( 4.619096255015035624, 27.05588869245799089, -0.3994036469054788596 ) ) ;
#38853=CARTESIAN_POINT ( 'NONE',  ( 5.992274430538982344, 155.3621521873626534, 0.2980204051088304884 ) ) ;
#38856=ORIENTED_EDGE ( 'NONE', *, *, #15449, .T. ) ;
#38858=CIRCLE ( 'NONE', #36832, 5.080000000000006288 ) ;
#38866=CARTESIAN_POINT ( 'NONE',  ( -4.773421586889413426, 116.8420656028321218, 0.1264526730306987090 ) ) ;
#38867=EDGE_LOOP ( 'NONE', ( #32337, #4959 ) ) ;
#38869=CARTESIAN_POINT ( 'NONE',  ( 6.015849376199521537, 121.4427344782352947, 0.04688609515921689230 ) ) ;
#38871=CARTESIAN_POINT ( 'NONE',  ( 1.708365387639474431, 115.7028613512742226, -1.661208468116264214 ) ) ;
#38872=CARTESIAN_POINT ( 'NONE',  ( -2.908234975202577122, 156.0868537499222839, -0.2102064236019247079 ) ) ;
#38873=CARTESIAN_POINT ( 'NONE',  ( 4.359322289182287591, -14.87073230766630694, 4.862486896750754184 ) ) ;
#38874=CARTESIAN_POINT ( 'NONE',  ( -1.249041419371764716, 159.0162744061759099, 1.301773431059132680 ) ) ;
#38876=CARTESIAN_POINT ( 'NONE',  ( 22.96225337745231343, 150.1545470440437953, 0.6883021358963680170 ) ) ;
#38877=CARTESIAN_POINT ( 'NONE',  ( 7.529841678698274698, 122.4254555285577339, 0.2702288470472028470 ) ) ;
#38878=CARTESIAN_POINT ( 'NONE',  ( 5.275990361836075060, 115.6909491485453145, -0.8142983086533037707 ) ) ;
#38879=CARTESIAN_POINT ( 'NONE',  ( 0.6724949529566155437, 16.91434809748496804, 0.7070771739444717818 ) ) ;
#38880=CARTESIAN_POINT ( 'NONE',  ( -10.80923569951307250, 157.9177219752764358, -0.3353067243844871093 ) ) ;
#38881=CARTESIAN_POINT ( 'NONE',  ( 5.078986093043053707, 78.83346620154574680, 0.1014902294541244060 ) ) ;
#38885=CARTESIAN_POINT ( 'NONE',  ( 8.512041645113450627, 118.9720402044547996, 1.274280440602515441 ) ) ;
#38888=CARTESIAN_POINT ( 'NONE',  ( 7.089439975188524201, 158.1912585135832785, 1.657816039754273607 ) ) ;
#38889=CARTESIAN_POINT ( 'NONE',  ( 12.64706598677940974, 155.2353133052689032, -1.715565181845534415 ) ) ;
#38890=CARTESIAN_POINT ( 'NONE',  ( -5.321447747238043036, 7.245273219182337243, -6.556399146060885919 ) ) ;
#38891=CARTESIAN_POINT ( 'NONE',  ( -5.844042411599879472, 117.9059190437751141, -0.9510131463654530881 ) ) ;
#38892=CARTESIAN_POINT ( 'NONE',  ( 4.657082998918331107, 117.9833643526148705, -0.7124481076139314029 ) ) ;
#38895=CARTESIAN_POINT ( 'NONE',  ( -10.40273896401448006, 153.1126597504080280, -0.1617772828476136959 ) ) ;
#38896=EDGE_CURVE ( 'NONE', #35057, #20737, #5153, .T. ) ;
#38898=CARTESIAN_POINT ( 'NONE',  ( -11.80606196054498369, 122.9427978038690270, -1.750206178813383584 ) ) ;
#38899=CARTESIAN_POINT ( 'NONE',  ( 5.836094479182562189, -14.94293577981173371, 0.6207079514943552034 ) ) ;
#38903=VERTEX_POINT ( 'NONE', #9785 ) ;
#38904=CARTESIAN_POINT ( 'NONE',  ( 1.339510839693822453, 119.4570717772418220, 0.6353817622545780974 ) ) ;
#38907=CARTESIAN_POINT ( 'NONE',  ( -5.705706447001241521, 123.8402959710505087, -0.07212015369193661152 ) ) ;
#38909=CARTESIAN_POINT ( 'NONE',  ( -2.203247880972440065, 24.02835216854757405, 8.161197317184477384 ) ) ;
#38910=CARTESIAN_POINT ( 'NONE',  ( 0.6802018490771016834, 156.3636429644085695, 0.5246204485115754101 ) ) ;
#38911=CARTESIAN_POINT ( 'NONE',  ( 9.616121018674252952, 118.2964180356302961, -0.4479623223841151525 ) ) ;
#38917=CARTESIAN_POINT ( 'NONE',  ( -23.11179153581203494, 149.9001102426712748, -0.4361622115260938015 ) ) ;
#38920=CARTESIAN_POINT ( 'NONE',  ( 4.403632403658274796, 119.4899321720584737, -0.7529549363037313370 ) ) ;
#38922=CARTESIAN_POINT ( 'NONE',  ( -3.666883307181661777, 120.9289264519876070, -0.3209655359951389952 ) ) ;
#38923=CARTESIAN_POINT ( 'NONE',  ( 4.087908758852305091, -13.37781719547838399, 3.422002167429263331 ) ) ;
#38925=CARTESIAN_POINT ( 'NONE',  ( 22.53527615164620101, 150.7831677823008363, 0.4503084484864737225 ) ) ;
#38927=CARTESIAN_POINT ( 'NONE',  ( -2.136650056307613621, 10.86338872207680950, -4.114640003288728920 ) ) ;
#38928=CARTESIAN_POINT ( 'NONE',  ( 5.332935397695205637, 105.1224662015457199, 0.1065647409268305201 ) ) ;
#38929=CARTESIAN_POINT ( 'NONE',  ( -3.302029177305334073, 159.4671159221996959, -0.06598240135525369754 ) ) ;
#38931=CARTESIAN_POINT ( 'NONE',  ( 6.875583424705200564, 120.7192244753876338, 1.121239711753028168 ) ) ;
#38932=CIRCLE ( 'NONE', #30082, 3.683000000000001162 ) ;
#38933=CARTESIAN_POINT ( 'NONE',  ( 4.198131962423935271, 12.64715247731088787, 1.959332076845688553 ) ) ;
#38934=CARTESIAN_POINT ( 'NONE',  ( 19.15327062675849135, 128.6826163344482268, 1.506695251711823058 ) ) ;
#38936=CARTESIAN_POINT ( 'NONE',  ( 14.04756362465202280, 122.1591959312462592, -1.132115996748545239 ) ) ;
#38937=CARTESIAN_POINT ( 'NONE',  ( -2.972019672840211513, 9.848453565018933986, 3.538668892428941781 ) ) ;
#38938=CARTESIAN_POINT ( 'NONE',  ( -22.03992273305667382, 150.6352520364973486, -1.509874617927602802 ) ) ;
#38939=ORIENTED_EDGE ( 'NONE', *, *, #12282, .T. ) ;
#38941=EDGE_CURVE ( 'NONE', #11376, #35682, #35359, .T. ) ;
#38942=CARTESIAN_POINT ( 'NONE',  ( -0.003052472355933761282, 120.8426702770480148, 0.1527581987772201888 ) ) ;
#38943=CARTESIAN_POINT ( 'NONE',  ( 2.663994046441380270, -15.36521416583532051, 5.826768514169494040 ) ) ;
#38947=CARTESIAN_POINT ( 'NONE',  ( 19.27109647334602016, 148.6897983921382433, 2.507318192549734981 ) ) ;
#38950=CARTESIAN_POINT ( 'NONE',  ( -17.79905452297358437, 125.1550653296939970, 0.5857557929999464008 ) ) ;
#38954=CARTESIAN_POINT ( 'NONE',  ( 9.710933996004669666, 118.1218853900603136, -0.2424195399123781347 ) ) ;
#38958=CARTESIAN_POINT ( 'NONE',  ( 1.913223137500898341, -15.30302091211069282, 5.362660726125270116 ) ) ;
#38960=DIRECTION ( 'NONE',  ( 4.017660918040594346E-17, -1.000000000000000000, -2.376309959284832031E-19 ) ) ;
#38961=CARTESIAN_POINT ( 'NONE',  ( -4.523630674469822033, 118.0850806367477190, 0.6137328214149938566 ) ) ;
#38965=CARTESIAN_POINT ( 'NONE',  ( 5.078986093043053707, 88.48546620154573361, 0.1014902294541237954 ) ) ;
#38966=CARTESIAN_POINT ( 'NONE',  ( -8.360168168866218608, 119.6977264182660576, -1.427561477091477737 ) ) ;
#38967=CARTESIAN_POINT ( 'NONE',  ( -5.451337559846766823, 117.5214873295501405, -0.8265904065678291168 ) ) ;
#38968=CARTESIAN_POINT ( 'NONE',  ( 4.670575340268697140, 117.8934551130230517, 0.9881073750738181838 ) ) ;
#38970=CARTESIAN_POINT ( 'NONE',  ( -8.439375761976453560, 122.5794309061019618, -0.8715591655942094285 ) ) ;
#38972=CARTESIAN_POINT ( 'NONE',  ( -2.413257664290607618, 115.7029552727873352, -1.699853810109273278 ) ) ;
#38974=CARTESIAN_POINT ( 'NONE',  ( -4.854186777038641765, 117.7557277303023966, -0.9091791526384296329 ) ) ;
#38975=CARTESIAN_POINT ( 'NONE',  ( 6.719914377343970457, 121.2247800624193133, -0.07397671124164055534 ) ) ;
#38976=CARTESIAN_POINT ( 'NONE',  ( -11.93440950959111291, 126.0992317015783328, -1.505959514896210605 ) ) ;
#38977=CARTESIAN_POINT ( 'NONE',  ( 23.45208337669092913, 146.8499405025503961, 0.4686284387228002446 ) ) ;
#38978=CARTESIAN_POINT ( 'NONE',  ( -0.03212616895158381530, 157.6269964811067155, 1.607724863813389415 ) ) ;
#38980=CARTESIAN_POINT ( 'NONE',  ( -8.012499360674619098, 122.8488795790854766, -0.07767969516895584237 ) ) ;
#38981=CARTESIAN_POINT ( 'NONE',  ( 3.745621265272091716, -10.50169880513956322, -2.708184146228840294 ) ) ;
#38982=CARTESIAN_POINT ( 'NONE',  ( 18.16683071450844267, 125.1529741258727597, 1.044517495177846422 ) ) ;
#38985=CARTESIAN_POINT ( 'NONE',  ( 2.381491173306826248, -15.37068253093559811, 4.932168965620852497 ) ) ;
#38986=CARTESIAN_POINT ( 'NONE',  ( -2.404146712672539099, 157.7073581658784178, 1.626633079703769358 ) ) ;
#38987=CARTESIAN_POINT ( 'NONE',  ( 0.2616662591921395387, 4.880059721033824793, -0.9399936778652994152 ) ) ;
#38988=CARTESIAN_POINT ( 'NONE',  ( -16.79208607122050978, 122.6968688451475771, -0.8807046615161948644 ) ) ;
#38990=CARTESIAN_POINT ( 'NONE',  ( 0.3959014520675726012, 0.7218480974852773402, -0.8918910426260873159 ) ) ;
#38991=EDGE_LOOP ( 'NONE', ( #36315, #18110, #596, #5509 ) ) ;
#38994=CARTESIAN_POINT ( 'NONE',  ( 6.868335724905528572, 121.8312213470058225, 0.2935230024867369059 ) ) ;
#38996=CARTESIAN_POINT ( 'NONE',  ( -6.503815726752127269, 121.4942169270607053, 0.3795357812798489383 ) ) ;
#38997=CARTESIAN_POINT ( 'NONE',  ( 4.031918519141627577, -13.48391852982397410, 3.589295450856327729 ) ) ;
#38998=CARTESIAN_POINT ( 'NONE',  ( 10.18365381109002854, 122.2967958330617648, -1.106735498401915763 ) ) ;
#38999=CARTESIAN_POINT ( 'NONE',  ( -12.54651694896177538, 122.2722385251898771, -1.803108555445325223 ) ) ;
#39001=CARTESIAN_POINT ( 'NONE',  ( 2.857130780617909149, -14.87311083204414786, 4.269097905712053276 ) ) ;
#39002=CARTESIAN_POINT ( 'NONE',  ( -1.091745343399155299, 36.70702312047181692, 0.5241475151901328067 ) ) ;
#39003=CARTESIAN_POINT ( 'NONE',  ( 13.67682410656400727, 150.2105054413494543, -0.1652630162413759318 ) ) ;
#39010=CARTESIAN_POINT ( 'NONE',  ( -6.376221727585796537E-14, 51.14746620154573264, 5.777789833161707559E-29 ) ) ;
#39011=CARTESIAN_POINT ( 'NONE',  ( 18.76910502294225225, 125.2887878443791294, 0.2589991215523650414 ) ) ;
#39012=CARTESIAN_POINT ( 'NONE',  ( -5.222556791543373045, 115.4535745449993982, 1.305545271932168960 ) ) ;
#39013=CIRCLE ( 'NONE', #24705, 5.080000000000006288 ) ;
#39014=DIRECTION ( 'NONE',  ( 4.017660918040594346E-17, -1.000000000000000000, -2.376309959284834438E-19 ) ) ;
#39016=CARTESIAN_POINT ( 'NONE',  ( -3.738651510184325399, 31.35217495388765840, -0.6318812681667338449 ) ) ;
#39017=CARTESIAN_POINT ( 'NONE',  ( 20.82206258336668014, 149.3152741295656369, 2.348048710389011973 ) ) ;
#39018=CARTESIAN_POINT ( 'NONE',  ( 1.391598188199559161, 15.24595356501894017, -4.406646451508545503 ) ) ;
#39019=CARTESIAN_POINT ( 'NONE',  ( -7.004517537292900720, 30.72436916340981838, -4.697416855195242213 ) ) ;
#39020=CARTESIAN_POINT ( 'NONE',  ( 2.192952236640623109, 116.7858836396481053, -0.4274597272194167741 ) ) ;
#39021=CARTESIAN_POINT ( 'NONE',  ( -0.9980778803428626000, 110.6314368487224300, -3.458106935563855622 ) ) ;
#39023=FACE_OUTER_BOUND ( 'NONE', #4151, .T. ) ;
#39024=CARTESIAN_POINT ( 'NONE',  ( -0.8468149500948856101, 104.6144662015456390, 4.761320281557485323 ) ) ;
#39025=CARTESIAN_POINT ( 'NONE',  ( -3.453265078539333288, 21.00871511114837276, -3.102408547967784092 ) ) ;
#39026=CARTESIAN_POINT ( 'NONE',  ( -4.757248700628498916, 117.4032733054477973, -1.206458840162573543 ) ) ;
#39027=CARTESIAN_POINT ( 'NONE',  ( 0.02983097946976470335, 117.3993836135854707, -1.492864285907033572 ) ) ;
#39028=CARTESIAN_POINT ( 'NONE',  ( 3.212496809824684441, -14.25148094350509353, 2.370051959060230473 ) ) ;
#39029=CARTESIAN_POINT ( 'NONE',  ( 1.272828668259097462, 111.9985432423065959, -2.911558293332169089 ) ) ;
#39030=CARTESIAN_POINT ( 'NONE',  ( -3.845766519666914629, 116.9593488885201538, 0.3368132424836106087 ) ) ;
#39034=CARTESIAN_POINT ( 'NONE',  ( 2.912792906754999134, 38.59631781016217644, -1.173005823891349220 ) ) ;
#39036=CARTESIAN_POINT ( 'NONE',  ( 2.040901337265842663, -15.69771917786945359, 5.688463219523050896 ) ) ;
#39037=CARTESIAN_POINT ( 'NONE',  ( -12.70950188986288154, 122.0451665396574725, 1.271450951352564251 ) ) ;
#39038=CARTESIAN_POINT ( 'NONE',  ( 13.26523119301593212, 121.0513591912305316, -0.9938426049807239648 ) ) ;
#39039=CARTESIAN_POINT ( 'NONE',  ( 4.627880361116947228, 7.839802885307131319, -0.3238752845059330032 ) ) ;
#39043=CARTESIAN_POINT ( 'NONE',  ( -0.07157677170311223247, 110.3683645023726569, 3.581994345755902032 ) ) ;
#39045=CARTESIAN_POINT ( 'NONE',  ( -15.43236126668712949, 134.8939017613128328, 1.443262610673741397 ) ) ;
#39046=CARTESIAN_POINT ( 'NONE',  ( 4.808131379915038472, 105.1224662015457625, -0.4149153341867673483 ) ) ;
#39047=CARTESIAN_POINT ( 'NONE',  ( 0.01111639999511693754, 119.1634951276629550, -0.5563101126475827884 ) ) ;
#39048=CARTESIAN_POINT ( 'NONE',  ( -9.041969115052843620, 119.3941581119689204, -1.378656440977003239 ) ) ;
#39052=CARTESIAN_POINT ( 'NONE',  ( 4.431862760627758746, 118.1653681970028913, -0.4638930779344027089 ) ) ;
#39053=CARTESIAN_POINT ( 'NONE',  ( 6.498933901768258359, 121.5572409441427482, -0.3210307352789208979 ) ) ;
#39054=ORIENTED_EDGE ( 'NONE', *, *, #38324, .T. ) ;
#39055=CARTESIAN_POINT ( 'NONE',  ( -5.074328365123786710, 120.0747842884402132, -0.9638994778299827537 ) ) ;
#39056=CARTESIAN_POINT ( 'NONE',  ( 3.395721326281507579, -14.88725931823228699, 0.4187095049187871121 ) ) ;
#39057=TOROIDAL_SURFACE ( 'NONE', #13870, 5.080000000000005400, 0.5080000000000000071 ) ;
#39059=CARTESIAN_POINT ( 'NONE',  ( -0.8462821048516611100, 105.1230362821993083, -5.276608005300069237 ) ) ;
#39060=B_SPLINE_CURVE_WITH_KNOTS ( 'NONE', 3,
 ( #6594, #32793, #22961, #19563, #29159, #19153, #3624, #26176, #16372, #16589, #41966, #38554, #32158, #2991, #32572, #41762, #9367, #3404, #29597, #19358, #38762, #3192, #430, #12562, #9573, #13401, #36203, #38972, #5, #29377, #22331, #217, #32364, #12971, #35571, #25964, #13192, #26390, #23169, #15952, #39396, #6184, #7025, #13822, #26820, #27235, #40458, #30634, #36418, #30009, #39827, #10621, #7444, #23603, #1058, #27443, #23386, #14228, #10415, #40038, #36624, #1478, #33642, #39610, #848, #30218, #17009, #7236, #20402, #17426, #29805, #7861, #24027, #33431, #4259, #20196, #20611, #20822, #11248, #40250, #23813, #30424, #17222, #1271, #14022 ),
 .UNSPECIFIED., .F., .F.,
 ( 4, 2, 2, 1, 1, 1, 1, 2, 2, 2, 1, 2, 2, 2, 2, 1, 1, 1, 2, 2, 2, 2, 1, 1, 1, 1, 2, 2, 2, 2, 1, 1, 2, 2, 2, 2, 2, 2, 2, 2, 2, 2, 2, 1, 2, 2, 2, 2, 2, 4 ),
 ( 0.000000000000000000, 0.1250000000000058842, 0.1875000000000088263, 0.2187500000000101308, 0.2343750000000107692, 0.2421875000000111300, 0.2460937500000114631, 0.2480468750000118794, 0.2500000000000122680, 0.3125000000000180411, 0.3437500000000208167, 0.3593750000000222045, 0.3750000000000235922, 0.4375000000000284772, 0.4687500000000308087, 0.4843750000000319189, 0.4921875000000324740, 0.4960937500000326961, 0.4980468750000327516, 0.5000000000000328626, 0.5625000000000327516, 0.5937500000000326406, 0.6093750000000326406, 0.6171875000000326406, 0.6210937500000325295, 0.6230468750000324185, 0.6240234375000324185, 0.6250000000000323075, 0.6875000000000266454, 0.7187500000000239808, 0.7343750000000224265, 0.7421875000000216493, 0.7460937500000212053, 0.7500000000000208722, 0.7812500000000180966, 0.7968750000000167644, 0.8125000000000153211, 0.8281250000000139888, 0.8359375000000132117, 0.8398437500000129896, 0.8437500000000127676, 0.8593750000000114353, 0.8671875000000108802, 0.8710937500000104361, 0.8730468750000103251, 0.8750000000000102141, 0.9062500000000076605, 0.9218750000000064393, 0.9375000000000051070, 1.000000000000000000 ),
 .UNSPECIFIED. ) ;
#39062=CARTESIAN_POINT ( 'NONE',  ( -4.869611397611841141, 117.6445991000119022, 0.8937056924343703690 ) ) ;
#39063=CARTESIAN_POINT ( 'NONE',  ( 8.888678185456905467, 122.0520977060996586, 1.259005013942402940 ) ) ;
#39066=CARTESIAN_POINT ( 'NONE',  ( 4.496586626007489151, 27.28078351817337222, -1.068494511273165193 ) ) ;
#39067=CARTESIAN_POINT ( 'NONE',  ( 8.997762725187955724, 123.9218113011205986, 0.2640260769295986187 ) ) ;
#39070=CARTESIAN_POINT ( 'NONE',  ( 5.563856532153242718, 116.6986126813221034, 0.08223999505859086456 ) ) ;
#39076=CARTESIAN_POINT ( 'NONE',  ( -4.074955089416341991, 118.2429491485453354, 0.1454234154749719787 ) ) ;
#39080=CARTESIAN_POINT ( 'NONE',  ( -1.411700740068628779, 159.5982469381528972, 0.1593474270858734332 ) ) ;
#39083=CARTESIAN_POINT ( 'NONE',  ( -6.977722893427367623, 121.9489747943516420, -0.1966404063935860980 ) ) ;
#39085=CARTESIAN_POINT ( 'NONE',  ( -5.326630349062241088, 115.7029491485453718, -0.4164715811699009618 ) ) ;
#39086=CARTESIAN_POINT ( 'NONE',  ( -14.23422759389739944, 138.9464670490549452, -0.5149110934774580040 ) ) ;
#39087=CARTESIAN_POINT ( 'NONE',  ( 5.341071565670632459, -14.32387631201759248, 3.633538872802142716 ) ) ;
#39088=CARTESIAN_POINT ( 'NONE',  ( -4.934953413367899167, 117.8999350694477926, 0.7268823312289468541 ) ) ;
#39089=CARTESIAN_POINT ( 'NONE',  ( -5.144468029576237278, 116.8626782701987565, -0.2538742916674817662 ) ) ;
#39090=CARTESIAN_POINT ( 'NONE',  ( 1.872007501980861299, 116.6503132507590124, 0.2654151457657344393 ) ) ;
#39091=CARTESIAN_POINT ( 'NONE',  ( 13.58790511794221523, 150.2605122904624011, 0.4013236421570368084 ) ) ;
#39093=CARTESIAN_POINT ( 'NONE',  ( -0.1566604602083998543, 5.914057227930348049, 0.9647682902456425902 ) ) ;
#39094=CARTESIAN_POINT ( 'NONE',  ( -23.26558566580239784, 149.3390083238215595, -0.6953334291057010619 ) ) ;
#39096=CARTESIAN_POINT ( 'NONE',  ( -0.02983097946891718685, 117.3993836135855418, 1.492864285907047561 ) ) ;
#39098=CARTESIAN_POINT ( 'NONE',  ( -2.526976701386534963, 116.7749708623049401, 0.4200550213075466832 ) ) ;
#39099=EDGE_LOOP ( 'NONE', ( #39799, #34166, #2763, #20779 ) ) ;
#39101=CARTESIAN_POINT ( 'NONE',  ( 15.17292428814148764, 123.1171956318823533, 1.668999667383225471 ) ) ;
#39102=CARTESIAN_POINT ( 'NONE',  ( 13.14453721617477733, 122.4605402651681487, -1.292199650740640138 ) ) ;
#39103=CARTESIAN_POINT ( 'NONE',  ( 0.8080343152487895475, 3.801264818822497560, -0.5430376807499140979 ) ) ;
#39104=CARTESIAN_POINT ( 'NONE',  ( -7.252988161461171757, 9.422892264050933164, 4.294140714350721311 ) ) ;
#39105=CARTESIAN_POINT ( 'NONE',  ( -1.070729637574143522, 117.4935207075373569, -0.5386181289574427655 ) ) ;
#39106=CARTESIAN_POINT ( 'NONE',  ( 4.892581560886663183, 117.7439198456695664, -0.7245015596533974644 ) ) ;
#39107=CARTESIAN_POINT ( 'NONE',  ( 4.762298162519684297, 112.7561542417671916, 2.571201254457596175 ) ) ;
#39108=CARTESIAN_POINT ( 'NONE',  ( 14.75676393591414026, 134.6798445586954927, -1.238239479614487770 ) ) ;
#39109=CARTESIAN_POINT ( 'NONE',  ( -0.6477285649444898263, 156.3042436901572216, 0.05974520555407247802 ) ) ;
#39111=CARTESIAN_POINT ( 'NONE',  ( -7.823018779267129297, 156.2605297791399437, -2.010767698085225152 ) ) ;
#39112=CARTESIAN_POINT ( 'NONE',  ( 6.083905389560601229, -14.65912421694762280, 0.09720023197589457153 ) ) ;
#39113=FACE_OUTER_BOUND ( 'NONE', #13034, .T. ) ;
#39114=EDGE_CURVE ( 'NONE', #37003, #28325, #15052, .T. ) ;
#39116=ORIENTED_EDGE ( 'NONE', *, *, #9741, .T. ) ;
#39117=CARTESIAN_POINT ( 'NONE',  ( 5.835067757121013443, 120.0568572605186546, 1.100767069290504940 ) ) ;
#39118=DIRECTION ( 'NONE',  ( -4.017660918040594346E-17, 1.000000000000000000, 2.376309959284834438E-19 ) ) ;
#39120=CARTESIAN_POINT ( 'NONE',  ( -3.173429932895099448, 117.8122656274855871, 0.8370585861429157282 ) ) ;
#39121=CARTESIAN_POINT ( 'NONE',  ( 2.561087359964590249, 24.90515699240134495, 8.022552078460996938 ) ) ;
#39122=CARTESIAN_POINT ( 'NONE',  ( 15.44906575790727921, 148.0679034673509875, 1.029643479621237478 ) ) ;
#39124=CARTESIAN_POINT ( 'NONE',  ( 6.906891541952338009, 117.5897289630162987, -0.4768185843253516798 ) ) ;
#39127=CARTESIAN_POINT ( 'NONE',  ( -0.2965531742116714331, 116.4333835968663919, 0.03207532894271102747 ) ) ;
#39130=CARTESIAN_POINT ( 'NONE',  ( -5.130992841088942491, 120.2796509446399398, -0.8476419795031335802 ) ) ;
#39131=CARTESIAN_POINT ( 'NONE',  ( 4.536516067734830848, -15.04041621514964255, 4.646661483318791142 ) ) ;
#39132=CARTESIAN_POINT ( 'NONE',  ( -0.6142257358153485614, 120.7813932625355307, -0.2072529566615756436 ) ) ;
#39133=CARTESIAN_POINT ( 'NONE',  ( 4.057314763829551474, -13.83595378911055285, 4.182047561617943110 ) ) ;
#39134=CARTESIAN_POINT ( 'NONE',  ( -6.540718711769984318E-14, 75.78546620154573077, -7.235675496349066572E-18 ) ) ;
#39135=CARTESIAN_POINT ( 'NONE',  ( 16.30293663320032849, 121.4145675751456253, 0.3429698291441256042 ) ) ;
#39137=CARTESIAN_POINT ( 'NONE',  ( -4.550674770548566173, 2.667180226961371137, -0.8080508602523945871 ) ) ;
#39138=ADVANCED_FACE ( 'NONE', ( #33014 ), #41168, .F. ) ;
#39139=CARTESIAN_POINT ( 'NONE',  ( 2.445891218400001232, 105.1244718176544524, 4.749792414014113895 ) ) ;
#39140=FACE_OUTER_BOUND ( 'NONE', #74, .T. ) ;
#39141=CARTESIAN_POINT ( 'NONE',  ( 5.237379388564934679, 115.7029491485453292, 1.024072862575109655 ) ) ;
#39142=CARTESIAN_POINT ( 'NONE',  ( -7.002513491937036427, 121.1574795575269263, 0.7090189476666535207 ) ) ;
#39144=CARTESIAN_POINT ( 'NONE',  ( 2.551181839206869917, 14.82117702134586779, -3.857898856385788999 ) ) ;
#39145=CARTESIAN_POINT ( 'NONE',  ( 6.873244579178494185, 117.6856483911789581, 0.8154597436780149922 ) ) ;
#39146=CARTESIAN_POINT ( 'NONE',  ( -15.47023807670837314, 120.6682698389898434, -0.3091321738930619678 ) ) ;
#39147=CARTESIAN_POINT ( 'NONE',  ( 1.146080138889219446, 106.2781093257879803, 5.162130396633914486 ) ) ;
#39148=CARTESIAN_POINT ( 'NONE',  ( 9.089826843846916304, 119.3941581119689204, -1.016340006442031152 ) ) ;
#39149=CARTESIAN_POINT ( 'NONE',  ( 4.064497669612420871, 2.951628549105334898, 2.233594334442648766 ) ) ;
#39150=CARTESIAN_POINT ( 'NONE',  ( -1.957152676258903323, 116.9869758084673208, -0.4489687564533212938 ) ) ;
#39151=ADVANCED_FACE ( 'NONE', ( #30222 ), #25051, .T. ) ;
#39152=ORIENTED_EDGE ( 'NONE', *, *, #41983, .T. ) ;
#39153=CARTESIAN_POINT ( 'NONE',  ( -8.172795105213701561, 122.8283871457973362, 0.1257892658093058003 ) ) ;
#39154=CARTESIAN_POINT ( 'NONE',  ( 5.943076596790061394, -13.74187730036333122, 2.284392803971454278 ) ) ;
#39156=CARTESIAN_POINT ( 'NONE',  ( -3.009709740711283388, 107.7307366742582104, -4.394550567200004920 ) ) ;
#39159=CARTESIAN_POINT ( 'NONE',  ( 19.50074546578241907, 147.2819018089465715, 2.521100153936117749 ) ) ;
#39160=PLANE ( 'NONE',  #4560 ) ;
#39161=CARTESIAN_POINT ( 'NONE',  ( 8.487687333566158898, 123.3253871723413368, 0.1696041924978713422 ) ) ;
#39162=CARTESIAN_POINT ( 'NONE',  ( -22.42204277426977299, 149.9331680011685251, 0.7277228188736590830 ) ) ;
#39163=CARTESIAN_POINT ( 'NONE',  ( 15.83110339195386729, 121.2341309109925334, -0.1099079758964731507 ) ) ;
#39167=CARTESIAN_POINT ( 'NONE',  ( -4.862674337261732482, 117.4104240214870885, -1.165717098571217747 ) ) ;
#39170=CARTESIAN_POINT ( 'NONE',  ( -4.543708444177163130, 118.0889193232460599, 0.5957003991893521366 ) ) ;
#39172=B_SPLINE_SURFACE_WITH_KNOTS ( 'NONE', 3, 3, ( 
 ( #25242, #13880, #6083, #22231, #4107, #25458, #31843, #16643 ),
 ( #29651, #20046, #36263, #35259, #36049, #489, #907, #25658 ),
 ( #23660, #38455, #26661, #33064, #23229, #39669, #7083, #3895 ),
 ( #10473, #19046, #16859, #9273, #12464, #10049, #23442, #5877 ) ),
 .UNSPECIFIED., .F., .F., .F.,
 ( 4, 4 ),
 ( 4, 2, 2, 4 ),
 ( 0.000000000000000000, 1.000000000000000000 ),
 ( 0.000000000000000000, 0.2500000000000000000, 0.5000000000000000000, 1.000000000000000000 ),
 .UNSPECIFIED. ) ;
#39173=EDGE_LOOP ( 'NONE', ( #23279, #34327, #1248, #14787 ) ) ;
#39174=CARTESIAN_POINT ( 'NONE',  ( -4.000258988046152098, 115.6909491485452719, -1.587041804271255296 ) ) ;
#39175=CARTESIAN_POINT ( 'NONE',  ( -5.905050715485153034, 119.1078666374620667, -1.262661138395162697 ) ) ;
#39177=CARTESIAN_POINT ( 'NONE',  ( -6.094139411022071684, 119.5248422734510427, -0.5163842741021831273 ) ) ;
#39178=CARTESIAN_POINT ( 'NONE',  ( 4.697508090083865717, 117.7521314560283088, 1.088652043387917434 ) ) ;
#39180=CARTESIAN_POINT ( 'NONE',  ( -9.631798221454433317, 123.4354624054469980, -1.070950170652381184 ) ) ;
#39181=CARTESIAN_POINT ( 'NONE',  ( -3.691024713256037870, 109.5877217411341320, 3.633260444712922865 ) ) ;
#39182=CARTESIAN_POINT ( 'NONE',  ( 7.614108603649442308, 124.2930771091975117, 0.1432033155151097026 ) ) ;
#39183=CARTESIAN_POINT ( 'NONE',  ( -16.97388159461598534, 146.7604995623492243, -1.927701477367710803 ) ) ;
#39185=CARTESIAN_POINT ( 'NONE',  ( -0.02874440110946554008, 158.8294072187990196, 1.438487372358303595 ) ) ;
#39187=CARTESIAN_POINT ( 'NONE',  ( -2.452794397974936036, 115.7029491485453434, 1.604287042619627845 ) ) ;
#39188=CARTESIAN_POINT ( 'NONE',  ( -15.72516475228267652, 145.6852934652650902, -0.2469506351165625946 ) ) ;
#39189=CARTESIAN_POINT ( 'NONE',  ( -3.832284926465886254, -5.753926550059754064, 2.584458424559757272 ) ) ;
#39190=CARTESIAN_POINT ( 'NONE',  ( 22.80460045200408814, 149.7823008822066697, 1.306974408439632640 ) ) ;
#39192=DIRECTION ( 'NONE',  ( -4.017660918040594346E-17, 1.000000000000000000, 2.376309959284834438E-19 ) ) ;
#39193=CARTESIAN_POINT ( 'NONE',  ( 3.509229686425914707, -14.99732357267335914, 1.369000748440630799 ) ) ;
#39194=CARTESIAN_POINT ( 'NONE',  ( -18.49981012119521750, 140.7300538122508726, 1.765484999878023098 ) ) ;
#39195=CARTESIAN_POINT ( 'NONE',  ( -0.01433812918766144522, 10.07226683256953947, 0.9740319587662029654 ) ) ;
#39196=CARTESIAN_POINT ( 'NONE',  ( -20.55326960831574823, 152.5775223076369400, -0.9856637426460332918 ) ) ;
#39198=CARTESIAN_POINT ( 'NONE',  ( -0.4866770014159069180, -4.230873095947595530, 0.8487236227246106601 ) ) ;
#39202=CARTESIAN_POINT ( 'NONE',  ( 6.110436517261101486, 121.4157903421748301, 0.3281350463252858951 ) ) ;
#39204=CARTESIAN_POINT ( 'NONE',  ( -3.160209531531049887, 156.1781389015385457, 0.7303267873898459106 ) ) ;
#39205=CARTESIAN_POINT ( 'NONE',  ( 3.526842715273949214, -14.30601272375732513, 4.884018970202873788 ) ) ;
#39206=CARTESIAN_POINT ( 'NONE',  ( 10.84737219364637362, 123.3109526380878833, -1.071866780254095985 ) ) ;
#39207=CARTESIAN_POINT ( 'NONE',  ( -3.201321489863747871, 118.6508749770327995, -0.9018090777949858694 ) ) ;
#39210=CARTESIAN_POINT ( 'NONE',  ( 3.150244473240279675, -14.07033042043420146, 1.813758411523331393 ) ) ;
#39211=CARTESIAN_POINT ( 'NONE',  ( -2.466321628261904042, 35.32195945946419613, 2.380963110963009832 ) ) ;
#39212=CARTESIAN_POINT ( 'NONE',  ( 7.582677863711187349, 122.4179301937671767, 0.01237541680613138753 ) ) ;
#39214=CARTESIAN_POINT ( 'NONE',  ( -4.429001560254139491, 111.0463454453107346, 3.038333220475521124 ) ) ;
#39218=DIRECTION ( 'NONE',  ( 0.9998004120163609398, 0.000000000000000000, 0.01997839162482749689 ) ) ;
#39220=CARTESIAN_POINT ( 'NONE',  ( 15.48485754026165750, 120.7065362441885981, 0.2052890747276165107 ) ) ;
#39221=CARTESIAN_POINT ( 'NONE',  ( -5.335400302754746527, 116.6867539651165373, 0.8102459553323390073 ) ) ;
#39222=CARTESIAN_POINT ( 'NONE',  ( -4.060687707471794639, 115.6909491485396728, 1.425937899757264926 ) ) ;
#39223=CARTESIAN_POINT ( 'NONE',  ( -3.113637796910019961, 33.63258992088869093, 1.040732188486675591 ) ) ;
#39224=CARTESIAN_POINT ( 'NONE',  ( 17.48279436891377969, 128.5781302034472162, 2.030760391889158800 ) ) ;
#39225=CARTESIAN_POINT ( 'NONE',  ( 2.794707274389933715, 24.31675177525179876, -3.679445548267922916 ) ) ;
#39226=CARTESIAN_POINT ( 'NONE',  ( -8.418873817481639321, -10.66996252118913091, -0.4581590610697409693 ) ) ;
#39227=CARTESIAN_POINT ( 'NONE',  ( 5.513305492129709329, 117.1850219934554502, -0.5726549213627184498 ) ) ;
#39228=CARTESIAN_POINT ( 'NONE',  ( -0.7406220848565643333, 119.3684187487962305, -0.7644009012486648880 ) ) ;
#39229=CARTESIAN_POINT ( 'NONE',  ( -22.46755768833301303, 150.8526571111528654, -0.4489552724284875951 ) ) ;
#39230=FACE_OUTER_BOUND ( 'NONE', #34967, .T. ) ;
#39231=CARTESIAN_POINT ( 'NONE',  ( -3.165966136369845696, 105.1242010218709169, 4.304718551588531561 ) ) ;
#39232=CARTESIAN_POINT ( 'NONE',  ( 2.332027132427558769, 25.33165720878049498, 3.998286310156994983 ) ) ;
#39234=CARTESIAN_POINT ( 'NONE',  ( -15.97340373827834270, 121.0409387471171101, -0.3191866212789525314 ) ) ;
#39235=CARTESIAN_POINT ( 'NONE',  ( 2.660183686505937839, -13.21883649654037640, 0.1900507390742080804 ) ) ;
#39236=CARTESIAN_POINT ( 'NONE',  ( 3.233068332335714334, 124.0549386377059307, 0.01378491165287854328 ) ) ;
#39237=CARTESIAN_POINT ( 'NONE',  ( -22.71566531765394714, 150.0520759213295889, 0.3958359165339127017 ) ) ;
#39245=CARTESIAN_POINT ( 'NONE',  ( 5.683854215195817794, -15.08228171793801664, 1.486458664383613293 ) ) ;
#39246=CARTESIAN_POINT ( 'NONE',  ( -20.17069300908759999, 147.5185649274072830, 1.704009200980389993 ) ) ;
#39247=B_SPLINE_CURVE_WITH_KNOTS ( 'NONE', 3,
 ( #13309, #1176, #33551, #26296, #39304, #14139 ),
 .UNSPECIFIED., .F., .F.,
 ( 4, 2, 4 ),
 ( 0.000000000000000000, 0.0001537973894545544668, 0.0003075947789091089337 ),
 .UNSPECIFIED. ) ;
#39248=CARTESIAN_POINT ( 'NONE',  ( 21.13693409061718853, 150.2702755442954583, -1.277357359820448623 ) ) ;
#39250=CARTESIAN_POINT ( 'NONE',  ( 4.087030650986479330, 6.990161447142720696, 2.163025551504125232 ) ) ;
#39252=ORIENTED_EDGE ( 'NONE', *, *, #19781, .F. ) ;
#39253=CARTESIAN_POINT ( 'NONE',  ( -4.757248700628498916, 117.4032733054477973, -1.206458840162573543 ) ) ;
#39255=CARTESIAN_POINT ( 'NONE',  ( 0.7702483762745334639, 120.5370721568272216, 0.5278276654545123181 ) ) ;
#39256=CARTESIAN_POINT ( 'NONE',  ( -0.02400040557479403425, 156.7459281804771365, 1.201078436782489822 ) ) ;
#39259=CARTESIAN_POINT ( 'NONE',  ( 14.49813937024303989, 152.7616507467334372, -1.711219460879523924 ) ) ;
#39260=CARTESIAN_POINT ( 'NONE',  ( 0.02874440110933761117, 158.8294072187990196, -1.438487372358303151 ) ) ;
#39263=CARTESIAN_POINT ( 'NONE',  ( 4.463198846623864569, 118.1257892472388420, -0.5548194780705337781 ) ) ;
#39264=CARTESIAN_POINT ( 'NONE',  ( 1.703787162446163128, 156.3322054215483092, -0.5946588160098701392 ) ) ;
#39266=CARTESIAN_POINT ( 'NONE',  ( -11.27861017918435316, 123.5700555580090594, -1.596916299002706596 ) ) ;
#39267=CARTESIAN_POINT ( 'NONE',  ( 3.190981477959303980, -15.14443901668413517, 3.594454035019850835 ) ) ;
#39270=DIRECTION ( 'NONE',  ( -4.017660918040594346E-17, 1.000000000000000000, 2.376309959284834438E-19 ) ) ;
#39271=CARTESIAN_POINT ( 'NONE',  ( 2.854375549615681962, 5.100648791940559867, -3.633247542873777380 ) ) ;
#39272=CARTESIAN_POINT ( 'NONE',  ( 11.62460634082105493, 124.4569610989641859, 1.598101315089358154 ) ) ;
#39273=CARTESIAN_POINT ( 'NONE',  ( -2.571890136738498978, 30.56018956238373363, 0.9273410376875194094 ) ) ;
#39274=CARTESIAN_POINT ( 'NONE',  ( 8.369638709285570854, -11.69152869469262157, 0.7709884470677680346 ) ) ;
#39275=CARTESIAN_POINT ( 'NONE',  ( 5.920896852643619646, 121.5237468798633955, 0.2406035128457659489 ) ) ;
#39279=CARTESIAN_POINT ( 'NONE',  ( 2.182419039857114385, 116.2183432897882653, -0.07172189831550286609 ) ) ;
#39282=FACE_OUTER_BOUND ( 'NONE', #40833, .T. ) ;
#39283=CARTESIAN_POINT ( 'NONE',  ( -8.788223396658947806, 117.7098387909605748, -0.3782402184110820742 ) ) ;
#39285=CARTESIAN_POINT ( 'NONE',  ( -4.074955089416341991, 118.2429491485453354, 0.1454234154749719787 ) ) ;
#39289=CARTESIAN_POINT ( 'NONE',  ( -22.80463473692780241, 150.3987591554885626, -0.1267456695372859987 ) ) ;
#39292=CARTESIAN_POINT ( 'NONE',  ( 7.802319612832663509, 122.5629922761574306, -0.05915617574866657152 ) ) ;
#39294=CARTESIAN_POINT ( 'NONE',  ( 3.517175496330608997, 50.13146620154573441, -1.199971990511068398 ) ) ;
#39295=CARTESIAN_POINT ( 'NONE',  ( -13.59447973938445031, 150.2262467139961473, -0.3969463805754209207 ) ) ;
#39296=CARTESIAN_POINT ( 'NONE',  ( 6.095337826619875443, -12.40160515274643593, 0.5428006832284221206 ) ) ;
#39297=CARTESIAN_POINT ( 'NONE',  ( -13.58393798013060838, 155.6725583577350278, 1.480266515874766542 ) ) ;
#39298=CARTESIAN_POINT ( 'NONE',  ( -4.507778648822867495, 31.37953541088120346, -1.025544427737863362 ) ) ;
#39299=CARTESIAN_POINT ( 'NONE',  ( 15.70536794749878240, 121.0099257824619627, 0.6352152019007784034 ) ) ;
#39300=CARTESIAN_POINT ( 'NONE',  ( 2.049679743348181038, -15.55809256208866209, 5.945888963465825405 ) ) ;
#39301=CARTESIAN_POINT ( 'NONE',  ( 4.815088043200419499, 118.5266822147775940, -0.8000015276336421843 ) ) ;
#39302=CARTESIAN_POINT ( 'NONE',  ( -0.7776641127062334791, -6.825634839940509124, -0.5883101582535473772 ) ) ;
#39303=CARTESIAN_POINT ( 'NONE',  ( 0.001838942458790341966, 116.4858755864912183, -0.09202820039585828116 ) ) ;
#39304=CARTESIAN_POINT ( 'NONE',  ( -4.697434178460381027, 117.9270761130219256, 0.7736398133629062146 ) ) ;
#39305=ADVANCED_FACE ( 'NONE', ( #1275 ), #12642, .F. ) ;
#39307=VERTEX_POINT ( 'NONE', #1895 ) ;
#39308=CARTESIAN_POINT ( 'NONE',  ( 5.549484939100879366, 116.7640263767076050, 0.3607275616457042977 ) ) ;
#39309=ORIENTED_EDGE ( 'NONE', *, *, #30969, .T. ) ;
#39310=CARTESIAN_POINT ( 'NONE',  ( -17.67908073341003217, 148.3509993576462307, 1.576626744559513682 ) ) ;
#39312=CARTESIAN_POINT ( 'NONE',  ( 7.848884907109186848, 118.8455990504009492, 1.250143668394028351 ) ) ;
#39313=CARTESIAN_POINT ( 'NONE',  ( 4.459427130834354713, 157.7533977378147654, -1.670975814381038704 ) ) ;
#39314=CARTESIAN_POINT ( 'NONE',  ( 0.2616662591921395387, 4.880059721033824793, -0.9399936778652994152 ) ) ;
#39315=CARTESIAN_POINT ( 'NONE',  ( -21.74240605069427446, 146.0876064316611860, -2.155783927327832306 ) ) ;
#39317=CARTESIAN_POINT ( 'NONE',  ( 4.634426409561430482, 118.0229150531969680, -0.6600590983778304999 ) ) ;
#39318=DIRECTION ( 'NONE',  ( -5.206863593109713661E-17, 1.000000000000000000, -1.077750396879097183E-30 ) ) ;
#39319=CARTESIAN_POINT ( 'NONE',  ( 10.91797240702838501, 124.6990478933366404, -0.8611562105571394232 ) ) ;
#39320=CARTESIAN_POINT ( 'NONE',  ( -5.659105795943250034E-14, 120.9974662015457341, 1.217662469992124504E-16 ) ) ;
#39321=EDGE_LOOP ( 'NONE', ( #40735, #9697, #3256, #4678 ) ) ;
#39322=CARTESIAN_POINT ( 'NONE',  ( -2.387603053075764592, 119.2205458019918751, -0.7760930522211748617 ) ) ;
#39323=CARTESIAN_POINT ( 'NONE',  ( 5.510877305967752271, -15.11690630435501248, 2.581843384194929758 ) ) ;
#39326=CARTESIAN_POINT ( 'NONE',  ( 5.834672723501171276, 119.9178398404649926, 1.129903066036338055 ) ) ;
#39327=CARTESIAN_POINT ( 'NONE',  ( -4.974001918040873882, 117.3966124607983659, -0.9751453929904890794 ) ) ;
#39329=( GEOMETRIC_REPRESENTATION_CONTEXT ( 3 ) GLOBAL_UNCERTAINTY_ASSIGNED_CONTEXT ( ( #3570 ) ) GLOBAL_UNIT_ASSIGNED_CONTEXT ( ( #19633, #13045, #22819 ) ) REPRESENTATION_CONTEXT ( 'NONE', 'WORKASPACE' ) );
#39330=CARTESIAN_POINT ( 'NONE',  ( -0.5697667371462552532, 106.2969274751293938, 5.150121607182108541 ) ) ;
#39331=CARTESIAN_POINT ( 'NONE',  ( -7.836836066720379357, 21.45871166075947656, -3.113543590022962881 ) ) ;
#39332=CARTESIAN_POINT ( 'NONE',  ( 8.208845571667657381, 122.7966848691156514, 0.5426025200548866279 ) ) ;
#39333=CARTESIAN_POINT ( 'NONE',  ( 11.30743779403327487, 119.0414093155750379, -0.5171725168954617313 ) ) ;
#39336=CARTESIAN_POINT ( 'NONE',  ( -6.606029807653651701E-14, 92.04146620154574521, -3.372746026535634231E-18 ) ) ;
#39339=CARTESIAN_POINT ( 'NONE',  ( -3.301441731159381998, 159.4676453237595410, -0.05120667577156005901 ) ) ;
#39340=ORIENTED_EDGE ( 'NONE', *, *, #28217, .F. ) ;
#39341=CARTESIAN_POINT ( 'NONE',  ( -5.387388416630612298, 120.5907514897421606, -0.7742399106899608974 ) ) ;
#39342=CARTESIAN_POINT ( 'NONE',  ( -3.517175496330734674, 50.63946620154572997, 1.199971990511067954 ) ) ;
#39343=CARTESIAN_POINT ( 'NONE',  ( -0.6635084510829686311, 156.3292479207028407, -0.3574603001491368781 ) ) ;
#39344=CARTESIAN_POINT ( 'NONE',  ( 2.161572811135036964, -15.02537755669194830, 5.771884496758437066 ) ) ;
#39345=CARTESIAN_POINT ( 'NONE',  ( -0.3839177515435807653, 117.3568105388816321, 0.4297925318014835794 ) ) ;
#39346=CARTESIAN_POINT ( 'NONE',  ( 6.079889189570776509, 121.4459138077559714, 0.1214906566337395633 ) ) ;
#39347=CARTESIAN_POINT ( 'NONE',  ( 4.723387343850681042, 116.7592613395855352, 0.1361797943638455854 ) ) ;
#39350=CARTESIAN_POINT ( 'NONE',  ( 4.560443952884764229, -11.68867000232777542, 0.6947937212093100445 ) ) ;
#39354=CARTESIAN_POINT ( 'NONE',  ( -6.866951340267982040, 120.5627663870395452, 0.8828549736221562583 ) ) ;
#39355=CARTESIAN_POINT ( 'NONE',  ( 3.363087486136625337, 4.875765145370108300, -3.182472177310056605 ) ) ;
#39356=CARTESIAN_POINT ( 'NONE',  ( 14.51109376910509496, 156.0472725025049954, 1.459756479172739319 ) ) ;
#39357=CARTESIAN_POINT ( 'NONE',  ( -0.04257260548303649222, 114.5099076536771321, 2.130507264987370863 ) ) ;
#39358=FACE_OUTER_BOUND ( 'NONE', #39099, .T. ) ;
#39359=CARTESIAN_POINT ( 'NONE',  ( 13.43626322254335470, 155.6061939908119882, -1.534180175809178426 ) ) ;
#39360=CARTESIAN_POINT ( 'NONE',  ( -4.255528399684056495, 7.899375212487111497, -1.818898740287305138 ) ) ;
#39361=CARTESIAN_POINT ( 'NONE',  ( -19.35449845750125419, 128.7092500879292345, -1.403651888282934079 ) ) ;
#39364=CARTESIAN_POINT ( 'NONE',  ( -9.049782359939607446, 124.0675141969884692, -0.1808361888366265546 ) ) ;
#39366=CARTESIAN_POINT ( 'NONE',  ( -4.553626923285223782, 121.1438296405421937, 0.06679122792761502114 ) ) ;
#39367=VECTOR ( 'NONE', #3722, 1000.000000000000114 ) ;
#39368=CARTESIAN_POINT ( 'NONE',  ( 6.383535934857802907, -12.90002020050165576, 0.3830569482466484321 ) ) ;
#39371=CARTESIAN_POINT ( 'NONE',  ( -3.155546303928757457, 108.2676741415912858, -4.292845182925542069 ) ) ;
#39373=CARTESIAN_POINT ( 'NONE',  ( 4.132678194918469217, 118.9132445967212419, 1.007338114003851537 ) ) ;
#39376=CARTESIAN_POINT ( 'NONE',  ( -22.63811803560004421, 149.3758529064199934, 0.7269731895922281195 ) ) ;
#39377=CARTESIAN_POINT ( 'NONE',  ( 4.581910832313284665, -15.30292673639559098, -0.5105377408573423814 ) ) ;
#39379=CARTESIAN_POINT ( 'NONE',  ( 10.70371904046263190, 157.9381250348597234, -0.2505172755855809563 ) ) ;
#39387=CARTESIAN_POINT ( 'NONE',  ( -4.459910022453251521, 118.1246115026546732, 0.5576706506857700418 ) ) ;
#39392=CARTESIAN_POINT ( 'NONE',  ( -8.279947364166304169, 120.0867420158548811, -1.450008613624738762 ) ) ;
#39393=CARTESIAN_POINT ( 'NONE',  ( -6.487065698695111848, 120.6500652548963899, -0.3947850323583859677 ) ) ;
#39394=CARTESIAN_POINT ( 'NONE',  ( 4.635084781736964032, 118.0285823782326986, 0.7661035724334133157 ) ) ;
#39395=CARTESIAN_POINT ( 'NONE',  ( -9.696059495791558902, 123.7664141286412871, -0.9760873372638445566 ) ) ;
#39396=CARTESIAN_POINT ( 'NONE',  ( -1.785155554672699596, 115.7029483421136860, -1.723366978510304071 ) ) ;
#39397=CARTESIAN_POINT ( 'NONE',  ( 0.4168181486211068876, 118.1651002420108512, -0.8784302966413096714 ) ) ;
#39398=CARTESIAN_POINT ( 'NONE',  ( 6.109903564962296585, 119.5248422734510427, -0.2725184514339174524 ) ) ;
#39399=CARTESIAN_POINT ( 'NONE',  ( -12.90748236152463413, 128.4900567078429390, -1.625332807165861260 ) ) ;
#39402=CARTESIAN_POINT ( 'NONE',  ( 8.730044398488933766, 118.0746546384499851, -0.4875147713271585914 ) ) ;
#39403=CARTESIAN_POINT ( 'NONE',  ( -4.621900518278277303, 121.2009512970921037, -0.02108223683487064209 ) ) ;
#39404=CARTESIAN_POINT ( 'NONE',  ( -2.983771112188844832, -5.329111280313512999, 3.548611825089460048 ) ) ;
#39405=CARTESIAN_POINT ( 'NONE',  ( 16.56062761363012825, 155.2525159475892167, 1.104293791145710024 ) ) ;
#39407=CARTESIAN_POINT ( 'NONE',  ( 3.044219152853963717, -14.30162947539197127, 0.8262259773895895831 ) ) ;
#39408=CARTESIAN_POINT ( 'NONE',  ( -19.01335237852168092, 147.2511928822236769, 1.726116106780064108 ) ) ;
#39409=CARTESIAN_POINT ( 'NONE',  ( -0.4197673533123916778, 5.974963139197415174, -0.8815698914671175057 ) ) ;
#39410=CARTESIAN_POINT ( 'NONE',  ( -21.76232006938128194, 151.4242408681541008, -1.019401482499525669 ) ) ;
#39411=CARTESIAN_POINT ( 'NONE',  ( -0.9274737138984842089, 27.34353985424608524, 0.2860612317039745167 ) ) ;
#39416=CARTESIAN_POINT ( 'NONE',  ( 6.266908424742160477, 120.0898888515776264, 0.4521870875522998046 ) ) ;
#39417=CARTESIAN_POINT ( 'NONE',  ( -13.64865021167028836, 134.2686865373913463, 0.6688813089635640141 ) ) ;
#39418=CARTESIAN_POINT ( 'NONE',  ( 3.244298476066852732, -14.49340328532226785, 5.143112664727522265 ) ) ;
#39419=CARTESIAN_POINT ( 'NONE',  ( 16.40043613793195476, 149.3997711511537148, -1.468335723160356432 ) ) ;
#39420=CARTESIAN_POINT ( 'NONE',  ( -16.38264815551540465, 131.4813445454897192, -2.297577408150382805 ) ) ;
#39421=CARTESIAN_POINT ( 'NONE',  ( 2.664052010559913253, -13.52006206191685322, 0.08958796903007473778 ) ) ;
#39422=CARTESIAN_POINT ( 'NONE',  ( -1.651955067937024291, 36.17532580612054005, 1.851243363282029764 ) ) ;
#39423=CARTESIAN_POINT ( 'NONE',  ( 9.057492758458241866, 123.9289873439938674, 0.02221773104347221292 ) ) ;
#39424=VERTEX_POINT ( 'NONE', #12095 ) ;
#39432=CARTESIAN_POINT ( 'NONE',  ( 2.757293845589572356, 116.5489981622532127, -0.01971897987843767783 ) ) ;
#39434=CARTESIAN_POINT ( 'NONE',  ( -6.150459292200251227, 119.5049778551863682, 0.2724401547530462819 ) ) ;
#39436=CARTESIAN_POINT ( 'NONE',  ( -2.721379687168246075, 118.0926204763706693, 0.8515759891865197773 ) ) ;
#39438=CARTESIAN_POINT ( 'NONE',  ( -4.679832524073478162, 32.47693947602098063, 1.143146696348500635 ) ) ;
#39439=CARTESIAN_POINT ( 'NONE',  ( 18.42009423903789411, 151.8926627062091086, 2.314360763190140613 ) ) ;
#39440=CARTESIAN_POINT ( 'NONE',  ( 4.626035402534343532, 22.79242798913371360, 0.3558936578225105341 ) ) ;
#39441=CARTESIAN_POINT ( 'NONE',  ( -8.293629857537270667, 31.38027257336059250, -1.381021427861755635 ) ) ;
#39442=CARTESIAN_POINT ( 'NONE',  ( 5.580386988971347328, 118.0037885632721668, -0.8768600884250703498 ) ) ;
#39443=CARTESIAN_POINT ( 'NONE',  ( -0.7055264248722583620, 108.7514562038770976, -4.178308661695779413 ) ) ;
#39445=CARTESIAN_POINT ( 'NONE',  ( -2.943103431893902666, 108.2626378167148573, -4.302975101750876163 ) ) ;
#39446=CARTESIAN_POINT ( 'NONE',  ( 1.821065711545410970, 105.1241838947191525, 5.023790078975794771 ) ) ;
#39447=CARTESIAN_POINT ( 'NONE',  ( 1.141857472271699425, 24.90688314728939190, 4.478778191171412182 ) ) ;
#39450=CARTESIAN_POINT ( 'NONE',  ( 2.467608985616319472, -14.95545905184315849, 4.893820528943690462 ) ) ;
#39451=CARTESIAN_POINT ( 'NONE',  ( 2.040875107092296137, 122.5452913651401587, -0.1521094801190006895 ) ) ;
#39452=CARTESIAN_POINT ( 'NONE',  ( -21.87092457242496479, 136.8312970274703844, 0.6093905233339396155 ) ) ;
#39455=ORIENTED_EDGE ( 'NONE', *, *, #25847, .F. ) ;
#39458=ORIENTED_EDGE ( 'NONE', *, *, #10228, .T. ) ;
#39460=CARTESIAN_POINT ( 'NONE',  ( 5.927515451590630313, -14.79481669900410701, -0.3156388015035426764 ) ) ;
#39461=CARTESIAN_POINT ( 'NONE',  ( -1.145842520593037150, 158.4310823543925721, 1.558676969884219554 ) ) ;
#39462=CARTESIAN_POINT ( 'NONE',  ( 19.46267448186331350, 131.9512773411433670, -1.172478082078345363 ) ) ;
#39463=CARTESIAN_POINT ( 'NONE',  ( 1.686640475165922748, -9.627085671684914914, -4.319569293544198274 ) ) ;
#39466=CARTESIAN_POINT ( 'NONE',  ( -4.942124793971827579, 117.4083539704047183, -1.067544502694063979 ) ) ;
#39467=CARTESIAN_POINT ( 'NONE',  ( 0.7330347863449895307, 118.7604188656930120, 0.9075975635256807728 ) ) ;
#39468=DIRECTION ( 'NONE',  ( 1.000000000000000000, 0.000000000000000000, 0.000000000000000000 ) ) ;
#39469=CARTESIAN_POINT ( 'NONE',  ( -15.03323000681570498, 150.5987129668814077, 1.374706190065595690 ) ) ;
#39471=CARTESIAN_POINT ( 'NONE',  ( 18.70798771669547378, 146.9271955717142930, -1.702497825003243648 ) ) ;
#39472=CARTESIAN_POINT ( 'NONE',  ( -19.77411333694952233, 150.7280352275851101, -2.313572189391364109 ) ) ;
#39474=ORIENTED_EDGE ( 'NONE', *, *, #25445, .T. ) ;
#39475=CARTESIAN_POINT ( 'NONE',  ( 4.558708663912786285, 118.0891419347824751, -0.5801029092231412276 ) ) ;
#39477=CARTESIAN_POINT ( 'NONE',  ( 10.06005632938184924, 124.8772485319846055, -0.3443025955426558538 ) ) ;
#39478=ORIENTED_EDGE ( 'NONE', *, *, #28238, .T. ) ;
#39479=CARTESIAN_POINT ( 'NONE',  ( -5.258743330460844412, 156.4258374981641282, -1.697662213785431140 ) ) ;
#39480=CARTESIAN_POINT ( 'NONE',  ( 1.834459164715513291, -15.41678468052755413, 5.387059099755636460 ) ) ;
#39483=CARTESIAN_POINT ( 'NONE',  ( 0.9983407785579379023, 1.652274601622760741, 4.518288805521794238 ) ) ;
#39484=CARTESIAN_POINT ( 'NONE',  ( 5.146579651471712147, 156.3268443366877989, 1.619031734741228190 ) ) ;
#39485=CARTESIAN_POINT ( 'NONE',  ( 2.247056820894810958, 36.23569059189157571, 0.3352685789618618517 ) ) ;
#39487=CARTESIAN_POINT ( 'NONE',  ( 4.364008504204949013, 7.202613900313124873, 1.580794030135405537 ) ) ;
#39488=CARTESIAN_POINT ( 'NONE',  ( 15.78121303607979797, 145.9231181611787918, 0.5460855120906794591 ) ) ;
#39492=FACE_OUTER_BOUND ( 'NONE', #12110, .T. ) ;
#39493=CARTESIAN_POINT ( 'NONE',  ( -0.4298579492383440281, 117.3993833036474825, 1.480795459422332039 ) ) ;
#39494=DIRECTION ( 'NONE',  ( 4.017660918040594346E-17, -1.000000000000000000, -2.376309959284834438E-19 ) ) ;
#39495=FACE_OUTER_BOUND ( 'NONE', #39884, .T. ) ;
#39499=CARTESIAN_POINT ( 'NONE',  ( -4.074955089416341991, 118.2429491485453354, 0.1454234154749719787 ) ) ;
#39503=CARTESIAN_POINT ( 'NONE',  ( -6.918378865934497135, 117.2797055272990292, 0.1815168674402110049 ) ) ;
#39504=EDGE_LOOP ( 'NONE', ( #7393, #19230, #9791, #36775 ) ) ;
#39506=CARTESIAN_POINT ( 'NONE',  ( 6.065828256571993649, 121.4399732366076137, 0.1127446937255504045 ) ) ;
#39508=DIRECTION ( 'NONE',  ( -0.9998004120163608288, 0.000000000000000000, -0.01997839162482750383 ) ) ;
#39510=CARTESIAN_POINT ( 'NONE',  ( -8.506011814013426431, 123.3280575159016905, -0.2025880313713109560 ) ) ;
#39511=CARTESIAN_POINT ( 'NONE',  ( 5.747688368404943127, -13.35872296688338245, 2.372087187842143674 ) ) ;
#39512=CARTESIAN_POINT ( 'NONE',  ( -13.77700084449478091, 121.8522644830672590, 1.120765626652496350 ) ) ;
#39513=CARTESIAN_POINT ( 'NONE',  ( -2.029258473809828711, 23.83235028914373288, 4.157303687431403993 ) ) ;
#39514=CARTESIAN_POINT ( 'NONE',  ( 8.183336086940839138, 117.5993832199734328, 0.5018928202873277344 ) ) ;
#39516=FACE_OUTER_BOUND ( 'NONE', #3010, .T. ) ;
#39517=CARTESIAN_POINT ( 'NONE',  ( -0.6834205802178441314, -7.050398998296187436, -0.6963091382628930903 ) ) ;
#39519=CARTESIAN_POINT ( 'NONE',  ( -4.741236776274016407, 116.7839080817633430, -0.2126559219428778014 ) ) ;
#39520=CARTESIAN_POINT ( 'NONE',  ( -6.629500982736845120E-14, 97.88346620154572975, -1.984505748321436882E-18 ) ) ;
#39521=CARTESIAN_POINT ( 'NONE',  ( 4.756845622061588230, 117.4019745679933067, 1.206737437952059455 ) ) ;
#39523=CARTESIAN_POINT ( 'NONE',  ( 2.257035569276631293, 116.3299305444832612, 0.2435412801458599619 ) ) ;
#39525=CARTESIAN_POINT ( 'NONE',  ( -17.90094693680112314, 147.7668373613703352, 1.576197898085538007 ) ) ;
#39527=CARTESIAN_POINT ( 'NONE',  ( 19.95554629013488324, 150.7967616730061593, 2.267143661507363017 ) ) ;
#39528=CARTESIAN_POINT ( 'NONE',  ( 19.58589350844858146, 147.2819018089465715, -1.740056086200069574 ) ) ;
#39529=CARTESIAN_POINT ( 'NONE',  ( -0.9543378889979354796, -1.596235181177088291, 0.1924800533990675688 ) ) ;
#39530=CARTESIAN_POINT ( 'NONE',  ( -14.57523308444403476, 121.8773232776577942, -1.525373117076484153 ) ) ;
#39531=CARTESIAN_POINT ( 'NONE',  ( 4.590426568450723721, 118.0729213092444070, -0.5858333982661567685 ) ) ;
#39532=CARTESIAN_POINT ( 'NONE',  ( 5.339716761587360416, 104.6144662015456959, 0.2456556763167710433 ) ) ;
#39533=CARTESIAN_POINT ( 'NONE',  ( 16.21676096112145871, 148.3349945484709451, -1.109893536416838966 ) ) ;
#39534=CARTESIAN_POINT ( 'NONE',  ( -5.301853325284237251, 121.3529869156830046, -0.07809170188345482266 ) ) ;
#39536=CARTESIAN_POINT ( 'NONE',  ( -17.41382892593916765, 149.8167423968465073, -2.401583459992671976 ) ) ;
#39537=CARTESIAN_POINT ( 'NONE',  ( 3.468122426543017500, -15.77657449013483770, 4.627414140463686820 ) ) ;
#39538=CARTESIAN_POINT ( 'NONE',  ( -4.557708454346482085, 31.49133016986147737, -0.6947391169727166194 ) ) ;
#39539=CARTESIAN_POINT ( 'NONE',  ( -4.578719595877105419, 118.0757894456264978, -0.7068121871710010273 ) ) ;
#39541=B_SPLINE_CURVE_WITH_KNOTS ( 'NONE', 3,
 ( #10051, #12420, #38618, #32852 ),
 .UNSPECIFIED., .F., .F.,
 ( 4, 4 ),
 ( -5.999999999774938839E-08, 0.0002260494465124368644 ),
 .UNSPECIFIED. ) ;
#39544=B_SPLINE_SURFACE_WITH_KNOTS ( 'NONE', 3, 3, ( 
 ( #38118, #9349, #9149, #19134, #31931, #2969, #15523, #22106, #19337, #5757, #12544, #35134, #5961, #18920, #2768, #32137 ),
 ( #34930, #22312, #3172, #15724, #29138, #28728, #41741, #28313, #25534, #15309, #38534, #28930, #8933, #18709, #21900, #41948 ),
 ( #12748, #25735, #38742, #31719, #28525, #41532, #12338, #41040, #11850, #5473, #11423, #40625, #21003, #34233, #8032, #2282 ),
 ( #17809, #24836, #5063, #34028, #34645, #21831, #27615, #2066, #8450, #18018, #1858, #11631, #14610, #4853, #14821, #24409 ),
 ( #37415, #24618, #8234, #8869, #41251, #37626, #30806, #31657, #31440, #12057, #21407, #15246, #25046, #21207, #1656, #27823 ),
 ( #31015, #40832, #34860, #34435, #37212, #5269, #38049, #18221, #11217, #31222, #15030, #28030, #37831, #18650, #8658, #28247 ),
 ( #21618, #18432, #5692, #2496, #15459, #28460, #24201, #25262, #16079, #32290, #32713, #35078, #22459, #29298, #39106, #22881 ),
 ( #3328, #5900, #22050, #3119, #19696, #16294, #18861, #9704, #26100, #12897, #22256, #9909, #38267, #12486, #31865, #3548 ),
 ( #35919, #19490, #28666, #29083, #2705, #15662, #2911, #32499, #16508, #142, #41466, #35281, #13108, #6729, #12273, #9084 ),
 ( #35488, #41678, #42103, #6106, #22671, #38688, #35704, #38476, #32075, #25481, #9294, #19282, #19069, #15874, #25681, #28881 ),
 ( #9494, #41893, #25885, #12691, #6310, #38892, #6515, #20117, #354, #20899, #1758, #16930, #3969, #34340, #13321, #21104 ),
 ( #4955, #14718, #26307, #24510, #8342, #768, #8130, #39317, #27720, #13745, #33140, #36128, #26738, #21310, #10123, #36542 ),
 ( #30920, #6943, #30702, #23305, #23094, #11320, #40729, #3759, #33920, #39747, #36343, #29930, #10545, #32929, #19913, #23514 ),
 ( #7360, #24309, #4750, #17703, #11529, #1552, #7158, #40528, #16717, #39531, #37314, #29515, #29721, #13537, #14507, #10336 ),
 ( #37517, #27521, #34128, #17914, #5169, #562, #26525, #36072, #39475, #6465, #35864, #22618, #12846, #3072, #32658, #23041 ),
 ( #29670, #35652, #19439, #16030, #16238, #32241, #26472, #16879, #29458, #3493, #32445, #26253, #16451, #33086, #13051, #35436 ),
 ( #39693, #39263, #29030, #19231, #29880, #297, #3277, #29241, #6677, #19643, #13269, #10069, #718, #85, #10280, #10493 ),
 ( #36285, #6889, #23251, #7105, #26042, #42051, #9857, #13692, #39052, #9650, #3917, #25831, #38841, #22827, #20065, #19857 ),
 ( #32872, #3704, #16663, #511, #26683, #13485, #6260, #40733, #927, #1557, #7934, #40325, #14514, #11118, #13900, #30925 ),
 ( #17503, #27724, #7309, #27311, #27526, #1133, #36697, #10904, #8136, #30500, #7518, #4544, #4756, #14100, #40532, #20480 ),
 ( #33298, #33506, #17708, #4337, #37114, #21109, #20905, #23462, #34134, #4960, #1343, #20695, #23677, #14299, #33719, #17919 ),
 ( #24107, #33926, #30291, #27100, #23894, #26890, #4126, #40111, #39901, #30707, #17300, #36911, #7728, #1763, #11326, #24313 ),
 ( #14723, #37320, #36489, #20269, #17086, #30087, #10697, #18127, #28146, #18970, #11748, #27935, #9194, #31132, #37522, #18336 ),
 ( #21523, #11534, #41369, #40942, #41153, #5593, #6008, #31340, #2816, #28780, #1969, #31767, #38169, #28362, #2609, #12173 ) ),
 .UNSPECIFIED., .F., .F., .F.,
 ( 4, 2, 2, 2, 2, 2, 2, 2, 2, 2, 2, 4 ),
 ( 4, 2, 2, 2, 2, 1, 1, 2, 4 ),
 ( 0.000000000000000000, 0.1320108428483948715, 0.1980162642725923072, 0.2640216856967897430, 0.3918749635278167553, 0.4558016024433302338, 0.5197282413588437677, 0.5807760813632503183, 0.6418239213676568689, 0.7639196013764699700, 0.8819598006882349850, 1.000000000000000000 ),
 ( 0.000000000000000000, 0.1250000000000000000, 0.2500000000000000000, 0.3750000000000000000, 0.5000000000000000000, 0.7500000000000000000, 0.8750000000000000000, 0.9375000000000000000, 1.000000000000000000 ),
 .UNSPECIFIED. ) ;
#39545=CARTESIAN_POINT ( 'NONE',  ( 3.875499641586223287, 157.0187206368471209, 1.749001665105742953 ) ) ;
#39546=LINE ( 'NONE', #17153, #37229 ) ;
#39547=AXIS2_PLACEMENT_3D ( 'NONE', #4921, #27063, #7267 ) ;
#39548=CARTESIAN_POINT ( 'NONE',  ( 15.73471677569731142, 120.8416612192341972, 0.3144170877231854955 ) ) ;
#39549=CARTESIAN_POINT ( 'NONE',  ( -8.291425676780491472, 12.16085651096402032, -1.523321141447528948 ) ) ;
#39550=CARTESIAN_POINT ( 'NONE',  ( 0.6714861817527252308, 156.3445873232922736, 0.4416347707370367748 ) ) ;
#39551=CARTESIAN_POINT ( 'NONE',  ( 7.717559979892206989, 158.5863655655865330, -0.7470610436598875692 ) ) ;
#39552=CARTESIAN_POINT ( 'NONE',  ( 2.948382749353823495, 50.63946620154572997, 1.837270642369387641 ) ) ;
#39555=CARTESIAN_POINT ( 'NONE',  ( -10.83072783392024618, 157.9016520041087688, -0.1964268902508805315 ) ) ;
#39556=ORIENTED_EDGE ( 'NONE', *, *, #1982, .F. ) ;
#39557=CARTESIAN_POINT ( 'NONE',  ( 8.137137598917451697, 121.0224714142185718, -1.005786695753826621 ) ) ;
#39559=CARTESIAN_POINT ( 'NONE',  ( -15.83982646870426336, 146.6055793175013093, -0.7699162700945604287 ) ) ;
#39560=CARTESIAN_POINT ( 'NONE',  ( 2.629318991877339418, -14.82094413389492615, 5.549789958447211013 ) ) ;
#39561=CARTESIAN_POINT ( 'NONE',  ( -15.72870526381844591, 122.9504679175852573, 0.8738493638518138873 ) ) ;
#39563=TOROIDAL_SURFACE ( 'NONE', #3504, 3.683000000000000718, 0.5080000000000000071 ) ;
#39564=CARTESIAN_POINT ( 'NONE',  ( 21.90252518039352836, 151.4352167165723415, 0.5139180553509253846 ) ) ;
#39565=VERTEX_POINT ( 'NONE', #11887 ) ;
#39566=CARTESIAN_POINT ( 'NONE',  ( 1.961646697876492373, -0.1315482170498871728, -4.191205975169975950 ) ) ;
#39568=DIRECTION ( 'NONE',  ( 0.9998004120163610509, 4.016384292689131511E-17, 0.01997839162482749689 ) ) ;
#39570=CARTESIAN_POINT ( 'NONE',  ( 4.826677069784417462, 119.0088915937735123, 1.091954489690918351 ) ) ;
#39571=CARTESIAN_POINT ( 'NONE',  ( 4.628409624684510781, -5.919234854628784959, 0.1277143096542201761 ) ) ;
#39572=CARTESIAN_POINT ( 'NONE',  ( 3.924194517545410932, 117.4679918459733585, 0.7389123598820265260 ) ) ;
#39575=CARTESIAN_POINT ( 'NONE',  ( 10.41147150295383739, 120.1444133044471556, -1.103258690517171514 ) ) ;
#39576=AXIS2_PLACEMENT_3D ( 'NONE', #32548, #22518, #32770 ) ;
#39577=CARTESIAN_POINT ( 'NONE',  ( -0.4757704999385121702, -3.320450887815510121, -4.596079559024887295 ) ) ;
#39578=CARTESIAN_POINT ( 'NONE',  ( -22.70157303802179882, 149.4207734315791072, -1.531927632650241566 ) ) ;
#39579=VERTEX_POINT ( 'NONE', #8695 ) ;
#39580=CARTESIAN_POINT ( 'NONE',  ( -9.439772580079139885, 124.2753396726362780, 0.1368060863603348387 ) ) ;
#39581=CARTESIAN_POINT ( 'NONE',  ( 5.379018416755689813, -14.82644845813459256, 3.481186560222681692 ) ) ;
#39584=CARTESIAN_POINT ( 'NONE',  ( -3.402419904042699006, 108.3861669196250688, -4.099931217281246987 ) ) ;
#39586=CARTESIAN_POINT ( 'NONE',  ( 1.237267194679675164, 118.7146927282448132, 0.6928808259403734793 ) ) ;
#39591=CARTESIAN_POINT ( 'NONE',  ( -12.83198513809782604, 156.8686255264331635, 0.8772202223719094416 ) ) ;
#39592=CARTESIAN_POINT ( 'NONE',  ( 3.683590692373001296, 21.29142263786511080, 7.571256661570916258 ) ) ;
#39594=CARTESIAN_POINT ( 'NONE',  ( 9.710114326862120393, 153.9716628027005925, 1.336640340121901582 ) ) ;
#39595=CARTESIAN_POINT ( 'NONE',  ( 0.9570688389943262653, 116.7004868406603322, -0.2253703713229211203 ) ) ;
#39602=CARTESIAN_POINT ( 'NONE',  ( -4.535200515210230598, 118.1197139754325036, 0.4752115866934419897 ) ) ;
#39606=CARTESIAN_POINT ( 'NONE',  ( -8.295186191818521237, 120.0125017958713727, -1.449258406794112997 ) ) ;
#39607=CARTESIAN_POINT ( 'NONE',  ( -5.194452014863664147, 116.1170857923940787, -1.235891685093609915 ) ) ;
#39608=CARTESIAN_POINT ( 'NONE',  ( 4.503786011748764473, 118.0871167092629577, 0.7873725921291204743 ) ) ;
#39609=CARTESIAN_POINT ( 'NONE',  ( -5.869717882709328372, 121.2452591720019370, -0.5958057796325608724 ) ) ;
#39610=CARTESIAN_POINT ( 'NONE',  ( -0.7572052446267691916, 115.7028915209885014, -1.755553211052053975 ) ) ;
#39611=CARTESIAN_POINT ( 'NONE',  ( 3.212429978159830668, 117.3993812122530329, -1.261639093947187540 ) ) ;
#39612=CARTESIAN_POINT ( 'NONE',  ( 4.518882305193341331, 111.2411499886600268, -2.961292089698490226 ) ) ;
#39613=CARTESIAN_POINT ( 'NONE',  ( -10.46581596931682689, 123.6668265419868646, -1.337773356492248489 ) ) ;
#39614=CARTESIAN_POINT ( 'NONE',  ( 5.243110457265114377, 104.6144662015457527, 1.505012106405181127 ) ) ;
#39615=CARTESIAN_POINT ( 'NONE',  ( -3.009276887026423264, 50.13146620154573441, 1.210121013456480377 ) ) ;
#39617=CARTESIAN_POINT ( 'NONE',  ( -11.83383823350433772, 152.0554358120322149, -0.04909464509748200090 ) ) ;
#39618=CARTESIAN_POINT ( 'NONE',  ( -2.424025297795170619, -5.104216246930970868, 3.935102955759355758 ) ) ;
#39619=CARTESIAN_POINT ( 'NONE',  ( 14.21090189159854056, 120.4756499382577886, 1.027290292067533306 ) ) ;
#39621=CARTESIAN_POINT ( 'NONE',  ( 2.572675278006325339, -15.15086880438208716, 4.677806725582212444 ) ) ;
#39622=CARTESIAN_POINT ( 'NONE',  ( -10.22873863908719194, 155.5514087735115822, 1.732306429912916945 ) ) ;
#39623=CARTESIAN_POINT ( 'NONE',  ( -0.8939936458071766623, -10.86866097718376523, 0.3889025406916932770 ) ) ;
#39624=CARTESIAN_POINT ( 'NONE',  ( -4.790162199822132649, 116.9482543694763166, -0.4383784235352165548 ) ) ;
#39626=CARTESIAN_POINT ( 'NONE',  ( 0.5584349385955980072, -2.506542431320444742, 0.8015440831694167212 ) ) ;
#39627=ADVANCED_FACE ( 'NONE', ( #39140 ), #39893, .T. ) ;
#39628=ORIENTED_EDGE ( 'NONE', *, *, #27602, .F. ) ;
#39630=CARTESIAN_POINT ( 'NONE',  ( 4.571503503190692541, 114.7252160460498516, 1.874454982749236498 ) ) ;
#39631=CARTESIAN_POINT ( 'NONE',  ( -0.005430166084385830948, 120.5648899400503069, 0.2717477157510632124 ) ) ;
#39632=CARTESIAN_POINT ( 'NONE',  ( 4.240324834746892257, -11.68880992198167945, 0.6883502328505933798 ) ) ;
#39633=CARTESIAN_POINT ( 'NONE',  ( 0.02768739821002418749, 156.9833357668885014, -1.385590625008458865 ) ) ;
#39634=CARTESIAN_POINT ( 'NONE',  ( -12.11054887026069871, 155.0146010091537221, -2.232606363771872715 ) ) ;
#39635=CARTESIAN_POINT ( 'NONE',  ( 4.808131379915037584, 104.6144662015457527, -0.4149153341867691802 ) ) ;
#39636=CARTESIAN_POINT ( 'NONE',  ( 3.115274840615241292, -13.78277351762104175, 1.693892316854531455 ) ) ;
#39637=CARTESIAN_POINT ( 'NONE',  ( -4.757248700571870437, 117.4032733054477688, -1.206458840171575009 ) ) ;
#39638=CARTESIAN_POINT ( 'NONE',  ( 12.97778284513260694, 133.8854804328748571, 0.04088747601382877045 ) ) ;
#39640=ORIENTED_EDGE ( 'NONE', *, *, #4211, .T. ) ;
#39642=CARTESIAN_POINT ( 'NONE',  ( 2.545864362986065110, 107.1172351171714467, 4.679951533430918964 ) ) ;
#39643=DIRECTION ( 'NONE',  ( 0.9998004120163609398, 4.016384292689130894E-17, 0.01997839162482749689 ) ) ;
#39646=CARTESIAN_POINT ( 'NONE',  ( 0.8998519745135501458, 116.4604358222411236, -0.05108568132534201112 ) ) ;
#39647=CARTESIAN_POINT ( 'NONE',  ( -2.677032024553447798, 107.2224589468338536, 4.627058715154634960 ) ) ;
#39648=TOROIDAL_SURFACE ( 'NONE', #37592, 4.826000000000000512, 0.5080000000000000071 ) ;
#39649=CARTESIAN_POINT ( 'NONE',  ( 1.753509963957065043, -15.55925396411267414, 5.871249478519287912 ) ) ;
#39651=CARTESIAN_POINT ( 'NONE',  ( 1.766327495819737248, 37.59738145967928347, -1.135536361765588032 ) ) ;
#39653=CARTESIAN_POINT ( 'NONE',  ( 20.63667788919575585, 149.2407879669073054, 2.389545083207231357 ) ) ;
#39654=CARTESIAN_POINT ( 'NONE',  ( -4.621355134897683570, 27.56591289442953041, -0.4301045952606497025 ) ) ;
#39655=CARTESIAN_POINT ( 'NONE',  ( -8.175057852536518510, 12.81247082500981094, 2.033924511151908199 ) ) ;
#39656=CARTESIAN_POINT ( 'NONE',  ( -5.501858137863374409, 117.7715637320503674, -1.036254152625051939 ) ) ;
#39657=CARTESIAN_POINT ( 'NONE',  ( -2.813253328531210240, 121.9077826007922312, -0.2952959765298339700 ) ) ;
#39658=CARTESIAN_POINT ( 'NONE',  ( 4.941661011542251458, 117.4083430605341647, 1.067727440994704624 ) ) ;
#39660=CARTESIAN_POINT ( 'NONE',  ( -5.018858541180816424, 105.1216645147153343, 1.817098519714964278 ) ) ;
#39662=CARTESIAN_POINT ( 'NONE',  ( 2.003160574663116034, 15.61121511114846960, 4.187759092076685619 ) ) ;
#39663=CARTESIAN_POINT ( 'NONE',  ( 5.008145224984434485, 117.3993836135855418, -0.7758584094373792706 ) ) ;
#39665=CARTESIAN_POINT ( 'NONE',  ( 3.317891647977158076, -14.03051783662405327, 3.455980060616059113 ) ) ;
#39666=CARTESIAN_POINT ( 'NONE',  ( 3.444826702830371179, 112.1633951907056996, -2.719597167543061023 ) ) ;
#39667=CARTESIAN_POINT ( 'NONE',  ( -22.95957815304936744, 148.8788797244430384, 0.5134943257494379854 ) ) ;
#39669=CARTESIAN_POINT ( 'NONE',  ( 4.976314832089088647, 117.4086780430578045, -0.8840892738920966831 ) ) ;
#39673=DIRECTION ( 'NONE',  ( -4.017660918040594346E-17, 1.000000000000000000, 2.376309959284834438E-19 ) ) ;
#39674=CARTESIAN_POINT ( 'NONE',  ( 5.328887433758706216, -15.24262819705347916, -0.4233796293290443269 ) ) ;
#39675=CARTESIAN_POINT ( 'NONE',  ( -15.41274837478120574, 125.4902479783272184, 1.384083614372567661 ) ) ;
#39676=CARTESIAN_POINT ( 'NONE',  ( 4.003603038177849349, 117.7793252414215317, -0.6798483224588709462 ) ) ;
#39677=CARTESIAN_POINT ( 'NONE',  ( 2.294499597581835193, -9.852027417895397932, -4.012603411698490774 ) ) ;
#39680=VERTEX_POINT ( 'NONE', #25297 ) ;
#39681=CARTESIAN_POINT ( 'NONE',  ( -4.970811386520536779, 117.4009602783328461, -0.9886943268754924130 ) ) ;
#39682=CARTESIAN_POINT ( 'NONE',  ( 1.907654281882038783, 121.7602717223048501, 0.3165470008995036055 ) ) ;
#39683=CARTESIAN_POINT ( 'NONE',  ( -8.983288137945276475, 154.9128698100208794, 1.355969927742461723 ) ) ;
#39684=CARTESIAN_POINT ( 'NONE',  ( -6.176553856875742987, 28.68700468106497681, 0.2098252341470465687 ) ) ;
#39686=CARTESIAN_POINT ( 'NONE',  ( 12.93728320859306358, 153.8477531742089468, -1.710492906883537945 ) ) ;
#39688=CARTESIAN_POINT ( 'NONE',  ( -4.941607502190771939, 118.3881331334009985, -1.039683250452205776 ) ) ;
#39690=CIRCLE ( 'NONE', #21277, 3.175000000000001155 ) ;
#39691=EDGE_CURVE ( 'NONE', #17404, #40141, #41488, .T. ) ;
#39693=CARTESIAN_POINT ( 'NONE',  ( 4.459699206147334394, 118.1245879234415526, -0.5577549297624452285 ) ) ;
#39694=CARTESIAN_POINT ( 'NONE',  ( 11.61789020275260320, 128.2970750771678752, -0.3952796010287947803 ) ) ;
#39696=CARTESIAN_POINT ( 'NONE',  ( 3.393951437975996743, -15.00105261681208901, 2.580228093083809071 ) ) ;
#39698=CIRCLE ( 'NONE', #37641, 3.683000000000001162 ) ;
#39700=CARTESIAN_POINT ( 'NONE',  ( 2.245307460665866728, 11.68515688572553479, 4.070821060848484940 ) ) ;
#39701=CARTESIAN_POINT ( 'NONE',  ( 16.78017617680110618, 148.3581316477378493, 2.036619618061131121 ) ) ;
#39702=CARTESIAN_POINT ( 'NONE',  ( -1.922869785242472762, 31.26939154837774026, 1.580357446662301157 ) ) ;
#39703=CARTESIAN_POINT ( 'NONE',  ( 1.616848224653315569, 9.589005055319924864, -4.350374724214612243 ) ) ;
#39704=CARTESIAN_POINT ( 'NONE',  ( 0.6369907463661377278, 120.9735524437166561, 0.07606544612864254984 ) ) ;
#39705=DIRECTION ( 'NONE',  ( -0.01997839162482761832, -1.040247600000950455E-18, 0.9998004120163610509 ) ) ;
#39707=CARTESIAN_POINT ( 'NONE',  ( 5.550207450195033587, 116.8112513961327608, -0.2456669984780832650 ) ) ;
#39718=CARTESIAN_POINT ( 'NONE',  ( -15.48609530480959862, 120.8153160915142337, 0.009749853210865312356 ) ) ;
#39721=ORIENTED_EDGE ( 'NONE', *, *, #12223, .F. ) ;
#39723=CARTESIAN_POINT ( 'NONE',  ( -6.061911998292836223, 121.4331685367002507, -0.1225658242750968657 ) ) ;
#39726=CARTESIAN_POINT ( 'NONE',  ( -4.223292309265045397, 155.8535809751167562, -0.1210084730045378199 ) ) ;
#39727=CARTESIAN_POINT ( 'NONE',  ( 5.718287093813156474, -14.23487671053640113, 2.942044405997081391 ) ) ;
#39728=CARTESIAN_POINT ( 'NONE',  ( -4.957730756931507443, 118.1424809852657773, 0.7901079947696818540 ) ) ;
#39729=CARTESIAN_POINT ( 'NONE',  ( 2.163044864548389512, 28.58015952483584599, -4.087059112497700042 ) ) ;
#39731=CARTESIAN_POINT ( 'NONE',  ( 13.33768363058602091, 156.9675713949798421, 0.6438986485269785343 ) ) ;
#39732=CARTESIAN_POINT ( 'NONE',  ( 5.933371281133245745, 155.4177045500023553, 0.2751541236311783600 ) ) ;
#39734=CARTESIAN_POINT ( 'NONE',  ( 0.8978640518332915432, -1.652899491467043180, 0.3817720442996600516 ) ) ;
#39735=CARTESIAN_POINT ( 'NONE',  ( -16.80483327138728455, 155.2524275687165982, -0.6336504121414450186 ) ) ;
#39739=CARTESIAN_POINT ( 'NONE',  ( 8.777645125800189518, 117.7559043064407831, 0.4625451175356548039 ) ) ;
#39740=CARTESIAN_POINT ( 'NONE',  ( -18.00062125403734115, 147.1528319293316542, 1.577578161537398493 ) ) ;
#39742=CARTESIAN_POINT ( 'NONE',  ( 15.09010836182842219, 154.7927800759015042, 2.085168164864714679 ) ) ;
#39743=CARTESIAN_POINT ( 'NONE',  ( 19.82182223277781574, 148.2167131080949787, -1.724547319354139407 ) ) ;
#39744=VECTOR ( 'NONE', #320, 1000.000000000000000 ) ;
#39745=CARTESIAN_POINT ( 'NONE',  ( 0.2779342515209439202, -14.33719732021959636, -0.9356842789569203012 ) ) ;
#39746=CARTESIAN_POINT ( 'NONE',  ( -10.62690833282013259, 119.8050749133877275, -1.415659332795228043 ) ) ;
#39747=CARTESIAN_POINT ( 'NONE',  ( 4.631749536040931758, 118.0396149105038148, -0.6219378133418650423 ) ) ;
#39750=CARTESIAN_POINT ( 'NONE',  ( 5.314256983240369436, 105.1224655745845240, -0.4585143440169748841 ) ) ;
#39751=EDGE_CURVE ( 'NONE', #21991, #3203, #5181, .T. ) ;
#39752=CARTESIAN_POINT ( 'NONE',  ( 16.69554899298717032, 147.2809512400332608, -1.108146210772844587 ) ) ;
#39753=CARTESIAN_POINT ( 'NONE',  ( -4.949223898456546422, 117.6231127316777645, 0.7510713373028163886 ) ) ;
#39754=ORIENTED_EDGE ( 'NONE', *, *, #32552, .F. ) ;
#39755=CARTESIAN_POINT ( 'NONE',  ( -10.55536611456385110, 121.9340018749941663, -1.633389464556823878 ) ) ;
#39756=CARTESIAN_POINT ( 'NONE',  ( 2.260827880841108417, -15.68886294521955271, 5.354637041555423416 ) ) ;
#39758=CARTESIAN_POINT ( 'NONE',  ( -5.208855653336853742, 31.38455280743060527, -0.6720767434146608377 ) ) ;
#39759=CARTESIAN_POINT ( 'NONE',  ( -4.638992326972686264, 118.0266412661314916, -0.7607261125604591889 ) ) ;
#39761=CARTESIAN_POINT ( 'NONE',  ( 4.105707650416926313, 118.2429491485453354, 0.3526241214267462065 ) ) ;
#39762=CARTESIAN_POINT ( 'NONE',  ( 3.977359857054884262, 157.1622345443605582, 1.793852766001656551 ) ) ;
#39764=CARTESIAN_POINT ( 'NONE',  ( 13.69580498508134347, 119.6466660129326272, 0.2573648061928516806 ) ) ;
#39766=CARTESIAN_POINT ( 'NONE',  ( -6.929632415086860675, 11.50928017261270497, -4.815005168835179816 ) ) ;
#39767=CARTESIAN_POINT ( 'NONE',  ( 15.47370139510873877, 143.5853813351167219, 1.046079274478294296 ) ) ;
#39768=CARTESIAN_POINT ( 'NONE',  ( 12.95464425824995836, 119.9671592456446803, -0.6090756887631914029 ) ) ;
#39769=DIRECTION ( 'NONE',  ( -0.9998004120163608288, 0.000000000000000000, -0.01997839162482749342 ) ) ;
#39771=DIRECTION ( 'NONE',  ( -0.9998004120163609398, -4.016384292689130894E-17, -0.01997839162482749689 ) ) ;
#39772=CARTESIAN_POINT ( 'NONE',  ( -15.65715779584560607, 120.8241032224722176, -0.2083191676592778541 ) ) ;
#39774=CARTESIAN_POINT ( 'NONE',  ( -5.444022911906507112, 120.6653284619048350, -0.7521495152940341766 ) ) ;
#39775=CARTESIAN_POINT ( 'NONE',  ( -8.644792878687130866, 118.5213301182957366, 0.7512959218659897020 ) ) ;
#39776=ORIENTED_EDGE ( 'NONE', *, *, #33934, .F. ) ;
#39778=CARTESIAN_POINT ( 'NONE',  ( -15.89665129872327576, 146.6311637152522565, -0.9120559015848336282 ) ) ;
#39779=CARTESIAN_POINT ( 'NONE',  ( 3.638845723804262189, -14.60113053194242383, 5.212470003951681363 ) ) ;
#39780=CARTESIAN_POINT ( 'NONE',  ( -17.77240244235150257, 153.9999837190418930, 1.018827867329159753 ) ) ;
#39781=CARTESIAN_POINT ( 'NONE',  ( -14.67500508080565780, 148.8517222229471315, -0.2932415260855779637 ) ) ;
#39782=CARTESIAN_POINT ( 'NONE',  ( 23.28768492013411873, 149.3500807853454546, 0.5424486132203802935 ) ) ;
#39784=CARTESIAN_POINT ( 'NONE',  ( 3.064284189169764971, -3.155149710853871525, 3.465721614369133174 ) ) ;
#39785=CARTESIAN_POINT ( 'NONE',  ( -6.439802422954663176E-14, 159.6054662015457382, 9.942593405483322146E-17 ) ) ;
#39788=CARTESIAN_POINT ( 'NONE',  ( 6.829987328009752723, 120.5672262496176614, 1.156243076138642634 ) ) ;
#39790=CARTESIAN_POINT ( 'NONE',  ( -4.627572956979934204, -1.171460759993483869, -0.2796867628226345492 ) ) ;
#39791=CARTESIAN_POINT ( 'NONE',  ( 3.898539657838472561, 117.3164332630744298, 0.6789226234856292619 ) ) ;
#39794=CARTESIAN_POINT ( 'NONE',  ( 0.01081828485854949978, 118.1092738308834669, -0.5413912121690739321 ) ) ;
#39795=CARTESIAN_POINT ( 'NONE',  ( 4.264856162967361364, -5.269518785209044154, -1.792273654951743067 ) ) ;
#39796=CARTESIAN_POINT ( 'NONE',  ( -22.22941764614908422, 150.1947564971097222, -1.617977611002929583 ) ) ;
#39799=ORIENTED_EDGE ( 'NONE', *, *, #25155, .F. ) ;
#39800=CARTESIAN_POINT ( 'NONE',  ( -9.391698128492089737, 124.2036136473707018, 0.1363215471561609049 ) ) ;
#39801=CARTESIAN_POINT ( 'NONE',  ( 6.240488881946434141, -13.64759869265259873, 1.419018975165988294 ) ) ;
#39803=CARTESIAN_POINT ( 'NONE',  ( -3.935359235824978708, 109.5187692929153656, -3.609514305193955774 ) ) ;
#39805=CARTESIAN_POINT ( 'NONE',  ( 0.9995654073148593222, 157.9544661020348997, 1.649992931013676500 ) ) ;
#39806=DIRECTION ( 'NONE',  ( -0.9998004120163609398, -4.016384292689130894E-17, -0.01997839162482749689 ) ) ;
#39808=CARTESIAN_POINT ( 'NONE',  ( -20.36908824613711033, 132.1502320877631007, 0.7851131432546855082 ) ) ;
#39809=CARTESIAN_POINT ( 'NONE',  ( -2.830841276205400270, 0.8888151952923978305, 7.984752373722160179 ) ) ;
#39810=CARTESIAN_POINT ( 'NONE',  ( 14.24959175664875843, 150.3563008155378213, 1.527850727897531513 ) ) ;
#39812=CARTESIAN_POINT ( 'NONE',  ( 0.008148259816486548221, 159.5682499516715040, -0.4077722408685185429 ) ) ;
#39816=CARTESIAN_POINT ( 'NONE',  ( -3.203180711741437481, 117.9394507697571584, 1.176600582426013952 ) ) ;
#39819=CARTESIAN_POINT ( 'NONE',  ( -4.505903132795666011, 118.1291298611057243, 0.5121121603323477434 ) ) ;
#39820=CARTESIAN_POINT ( 'NONE',  ( 3.946705940144926483, 109.6290786634770456, -3.598380483330867463 ) ) ;
#39823=CARTESIAN_POINT ( 'NONE',  ( 8.335401033256285785, 120.0665470143100322, -1.117875946357163253 ) ) ;
#39824=CARTESIAN_POINT ( 'NONE',  ( -6.508649675962092651, 120.6419738463991536, -0.3953840990482027085 ) ) ;
#39825=CARTESIAN_POINT ( 'NONE',  ( 4.574997526833646688, 118.0705043500909142, 0.7556435857121347466 ) ) ;
#39826=CARTESIAN_POINT ( 'NONE',  ( -7.104091076028453244, 121.8059686962219672, -0.6844636119373687100 ) ) ;
#39827=CARTESIAN_POINT ( 'NONE',  ( -1.198294787039654974, 115.7029448745467732, -1.741961060379599413 ) ) ;
#39828=CARTESIAN_POINT ( 'NONE',  ( 0.7552937574752076610, 117.3993842961046568, -1.459880452114538985 ) ) ;
#39829=CYLINDRICAL_SURFACE ( 'NONE', #37632, 5.588000000000006295 ) ;
#39830=CARTESIAN_POINT ( 'NONE',  ( -14.05412825714270397, 131.1061190467503934, -1.842221413061616797 ) ) ;
#39833=CARTESIAN_POINT ( 'NONE',  ( 8.644792878686919479, 118.5213301182956656, -0.7512959218659588378 ) ) ;
#39834=CARTESIAN_POINT ( 'NONE',  ( -3.792622695653071307, 121.0920089199514535, 0.02902016224539996636 ) ) ;
#39836=CARTESIAN_POINT ( 'NONE',  ( 18.24338043389141362, 154.1370782493726210, 1.275500441016771624 ) ) ;
#39837=CARTESIAN_POINT ( 'NONE',  ( -6.439703808512989190E-14, 63.33946620154573282, 4.463794035948134848E-29 ) ) ;
#39838=CARTESIAN_POINT ( 'NONE',  ( 2.245555723253176872, -15.32365336378345511, 5.046800657416122604 ) ) ;
#39839=CARTESIAN_POINT ( 'NONE',  ( -18.65843730539394230, 148.7425187291823363, 1.723213218779726441 ) ) ;
#39840=CARTESIAN_POINT ( 'NONE',  ( -0.3451692354163579113, -3.745485276186693469, -0.9107729336563508138 ) ) ;
#39841=CARTESIAN_POINT ( 'NONE',  ( -19.93082032328737085, 128.8226523212408949, -1.025501306202716734 ) ) ;
#39842=CARTESIAN_POINT ( 'NONE',  ( 0.7509867122348852231, -11.68634165275979342, 0.6197512838553165260 ) ) ;
#39844=ADVANCED_FACE ( 'NONE', ( #23981 ), #25556, .F. ) ;
#39846=CARTESIAN_POINT ( 'NONE',  ( 6.465481721428002260, 120.6581566633936404, 0.3941859656685693380 ) ) ;
#39848=CARTESIAN_POINT ( 'NONE',  ( -9.374368624788303350, 123.5785764018267514, 0.4819391486299057226 ) ) ;
#39849=CARTESIAN_POINT ( 'NONE',  ( 5.004296470405577679, -11.88282826624689825, 0.9770688040177184508 ) ) ;
#39850=CARTESIAN_POINT ( 'NONE',  ( 17.49548072478902583, 148.2779598588913643, -1.530134328283176304 ) ) ;
#39851=CARTESIAN_POINT ( 'NONE',  ( -9.864431837517996016, 120.7895603300898699, -1.595968683908903785 ) ) ;
#39852=CARTESIAN_POINT ( 'NONE',  ( -2.864695162152176788, 104.6144662015457669, 3.894373788578088469 ) ) ;
#39853=CARTESIAN_POINT ( 'NONE',  ( 2.467608985616319472, -14.95545905184315849, 4.893820528943690462 ) ) ;
#39854=CARTESIAN_POINT ( 'NONE',  ( -4.915268796012386865, 117.6231067272046289, -0.9482029235052464866 ) ) ;
#39855=CARTESIAN_POINT ( 'NONE',  ( 15.25729751669398659, 143.4548391324710224, 0.07249109134377358654 ) ) ;
#39857=CARTESIAN_POINT ( 'NONE',  ( -2.790041887114321995, 107.7052943677556556, 4.425947592945074227 ) ) ;
#39858=CARTESIAN_POINT ( 'NONE',  ( 4.439281039736937551, 110.9173483060885843, 3.020962623249374257 ) ) ;
#39860=CARTESIAN_POINT ( 'NONE',  ( -4.973569738608247803, 117.3993868453981548, -0.9750659555622913643 ) ) ;
#39861=CARTESIAN_POINT ( 'NONE',  ( 15.16801640535318363, 156.1230782244120121, 0.1031879763837426633 ) ) ;
#39862=DIRECTION ( 'NONE',  ( -5.206863593109713661E-17, 1.000000000000000000, -1.077750396879097183E-30 ) ) ;
#39863=CARTESIAN_POINT ( 'NONE',  ( 1.989873938678733412, -15.24182034147698950, 5.977043307750504297 ) ) ;
#39865=CARTESIAN_POINT ( 'NONE',  ( -2.603905383243863891, 31.86823266994409565, 1.021610582188352323 ) ) ;
#39866=CARTESIAN_POINT ( 'NONE',  ( 14.76979702826404406, 154.6636077862465015, 2.174438252133946481 ) ) ;
#39868=VERTEX_POINT ( 'NONE', #40205 ) ;
#39869=CARTESIAN_POINT ( 'NONE',  ( -0.4304388160753707671, 14.75877898171113145, 8.412599170943037663 ) ) ;
#39870=CARTESIAN_POINT ( 'NONE',  ( -8.600679198160465333, 118.5556138246751487, -1.111917903331490987 ) ) ;
#39871=CARTESIAN_POINT ( 'NONE',  ( -2.327304502367640193, 119.2037781873646622, -0.6856724729282701603 ) ) ;
#39874=CARTESIAN_POINT ( 'NONE',  ( -4.356736194631761094, 104.6144662015456959, 2.084086694369730264 ) ) ;
#39875=CARTESIAN_POINT ( 'NONE',  ( 4.634220987317881679, -1.855718946426311078, -0.01876340930339078644 ) ) ;
#39877=CARTESIAN_POINT ( 'NONE',  ( -4.851810479404537801, 115.6909491485453003, 1.282009238014815811 ) ) ;
#39878=CARTESIAN_POINT ( 'NONE',  ( 2.905753382753808900, -13.11311505661566557, 0.7091545436608904796 ) ) ;
#39879=CARTESIAN_POINT ( 'NONE',  ( 3.467804978690671280, 119.7720183225874138, -0.4097519885510783610 ) ) ;
#39880=CARTESIAN_POINT ( 'NONE',  ( -0.3479910049261774052, 116.9201722098172382, 0.3032510685202792766 ) ) ;
#39884=EDGE_LOOP ( 'NONE', ( #10906, #6444 ) ) ;
#39886=CARTESIAN_POINT ( 'NONE',  ( 4.883858777703569132, -15.45279978240890451, 0.9440085714135780792 ) ) ;
#39887=CARTESIAN_POINT ( 'NONE',  ( -19.90609901365559509, 149.5711785761137662, 1.665592367946398644 ) ) ;
#39888=CARTESIAN_POINT ( 'NONE',  ( -3.416230376366909294, -5.529048218071860532, 3.121479803864907865 ) ) ;
#39890=ORIENTED_EDGE ( 'NONE', *, *, #32998, .T. ) ;
#39892=CARTESIAN_POINT ( 'NONE',  ( 2.311675797007677335, 124.5312663981120380, 0.07107509915817157575 ) ) ;
#39893=B_SPLINE_SURFACE_WITH_KNOTS ( 'NONE', 3, 3, ( 
 ( #22708, #35523, #6761, #3362, #9324, #2943, #12722, #16112 ),
 ( #12517, #35109, #22287, #3149, #19523, #19104, #12309, #35949 ),
 ( #19729, #9120, #19315, #9945, #31904, #6549, #18895, #2533 ),
 ( #41503, #35737, #35312, #38718, #2740, #6345, #16329, #15907 ) ),
 .UNSPECIFIED., .F., .F., .F.,
 ( 4, 4 ),
 ( 4, 2, 2, 4 ),
 ( 0.000000000000000000, 1.000000000000000000 ),
 ( 0.000000000000000000, 0.2500000000000000000, 0.5000000000000000000, 1.000000000000000000 ),
 .UNSPECIFIED. ) ;
#39894=CARTESIAN_POINT ( 'NONE',  ( -11.17088054096573124, 124.6236798342360856, 0.9649352710901087926 ) ) ;
#39895=CARTESIAN_POINT ( 'NONE',  ( 1.526750911922509779, 118.1287369781418164, 0.9395972400893385368 ) ) ;
#39896=CARTESIAN_POINT ( 'NONE',  ( 18.43358770356677923, 147.0160646422468744, -1.663356549802410767 ) ) ;
#39897=CARTESIAN_POINT ( 'NONE',  ( -16.23079787743092339, 153.4734386769207504, -2.282812701028141600 ) ) ;
#39900=CIRCLE ( 'NONE', #30354, 3.175000000000001155 ) ;
#39901=CARTESIAN_POINT ( 'NONE',  ( 4.164354687101496921, 118.2394403266935115, -0.2263719665096066147 ) ) ;
#39903=CARTESIAN_POINT ( 'NONE',  ( 6.164480127824531586, 155.3548635187015350, -0.4492659787150437012 ) ) ;
#39907=CARTESIAN_POINT ( 'NONE',  ( 2.484037338616324142, -15.29988040857715959, 4.804498879097399033 ) ) ;
#39908=CARTESIAN_POINT ( 'NONE',  ( -4.932064943850939187, 117.4109299206517818, 0.9378731322835484052 ) ) ;
#39910=CARTESIAN_POINT ( 'NONE',  ( -4.503669762702418033, -0.7216326387320324276, 1.072590735790061922 ) ) ;
#39911=CARTESIAN_POINT ( 'NONE',  ( 3.477534164838054664, 156.5024071230465097, 1.413294873543960550 ) ) ;
#39913=CARTESIAN_POINT ( 'NONE',  ( 2.920597266354742150, 38.61197011361286258, -0.9696037573092457507 ) ) ;
#39914=CARTESIAN_POINT ( 'NONE',  ( 4.627880361116947228, 7.839802885307131319, -0.3238752845059330032 ) ) ;
#39915=CARTESIAN_POINT ( 'NONE',  ( 12.88021573494086525, 133.7932622986943159, 0.3045934876098303490 ) ) ;
#39916=FACE_OUTER_BOUND ( 'NONE', #9059, .T. ) ;
#39919=CARTESIAN_POINT ( 'NONE',  ( 2.177580517772025104, 116.2510284916901782, -0.1164253007932135875 ) ) ;
#39920=DIRECTION ( 'NONE',  ( -0.01997839162482737546, -1.040247600000940825E-18, 0.9998004120163610509 ) ) ;
#39924=CARTESIAN_POINT ( 'NONE',  ( -1.495267265506447174, 0.7142801726123456652, -8.304712878169773660 ) ) ;
#39926=DIRECTION ( 'NONE',  ( 5.206863593109713661E-17, -1.000000000000000000, 1.077750396879097183E-30 ) ) ;
#39929=CARTESIAN_POINT ( 'NONE',  ( 0.01254005783130787005, 120.1716774721351157, -0.6275557724548823657 ) ) ;
#39930=CARTESIAN_POINT ( 'NONE',  ( -15.22618061423900215, 120.7148350616293300, 0.1140551857323335305 ) ) ;
#39934=CARTESIAN_POINT ( 'NONE',  ( 7.795083226883911642, 122.5915480376389866, 0.009939133504787384804 ) ) ;
#39937=CARTESIAN_POINT ( 'NONE',  ( -15.21722582537775637, 143.4245298570049840, -0.3558394363636828706 ) ) ;
#39938=CARTESIAN_POINT ( 'NONE',  ( 5.379018416755689813, -14.82644845813459256, 3.481186560222681692 ) ) ;
#39939=CARTESIAN_POINT ( 'NONE',  ( -20.76034172958460644, 149.5879773183856685, 1.515053003442401680 ) ) ;
#39940=CARTESIAN_POINT ( 'NONE',  ( -4.420329592304260480, 21.65838872207745425, -1.398650104627336743 ) ) ;
#39941=CARTESIAN_POINT ( 'NONE',  ( 23.20196384716129856, 149.3105122542552863, 0.9177021184322482483 ) ) ;
#39942=CARTESIAN_POINT ( 'NONE',  ( 2.217927584814327613, -15.58779998727646898, 5.527464523343218694 ) ) ;
#39943=CARTESIAN_POINT ( 'NONE',  ( -1.648064503646425649, 29.87956589480163316, -4.325937074807028715 ) ) ;
#39944=CARTESIAN_POINT ( 'NONE',  ( -0.2091969695887432312, -7.904008462454454431, -0.9542532860826526964 ) ) ;
#39945=CARTESIAN_POINT ( 'NONE',  ( -14.74522353080556947, 120.3062992333385921, -0.5208356519839250076 ) ) ;
#39946=CARTESIAN_POINT ( 'NONE',  ( 4.937178538763392410, 117.4076076791066470, 1.082348873812597922 ) ) ;
#39948=CARTESIAN_POINT ( 'NONE',  ( -2.255705573375303974, 116.3134673151485430, 0.1365217663799836445 ) ) ;
#39949=CARTESIAN_POINT ( 'NONE',  ( -14.94938132205808579, 131.2528086460777388, 1.477614431843955467 ) ) ;
#39951=CARTESIAN_POINT ( 'NONE',  ( 3.077448401760547902, 117.9340107969418341, 0.8067720256249978350 ) ) ;
#39952=CARTESIAN_POINT ( 'NONE',  ( 18.20160870511324447, 135.6759721228443425, -1.705493676697015015 ) ) ;
#39953=CARTESIAN_POINT ( 'NONE',  ( 0.4551624184790937777, -5.041848893434334400, -0.8611515851349844652 ) ) ;
#39954=CARTESIAN_POINT ( 'NONE',  ( -21.34910226488280927, 149.1985357531029308, -2.237902092811237864 ) ) ;
#39957=AXIS2_PLACEMENT_3D ( 'NONE', #28236, #41242, #12047 ) ;
#39958=CARTESIAN_POINT ( 'NONE',  ( 3.853324095080354006, 105.1225530707694986, 3.704948206273974698 ) ) ;
#39959=CARTESIAN_POINT ( 'NONE',  ( 4.430366727502268454, 120.6578283891288379, -0.4452475156743748164 ) ) ;
#39960=CARTESIAN_POINT ( 'NONE',  ( -1.561582345843753217, 156.2588034088681184, -0.03120413162939504950 ) ) ;
#39962=CARTESIAN_POINT ( 'NONE',  ( -14.47078677760135257, 128.5519869857110393, -2.060874889273090815 ) ) ;
#39963=CARTESIAN_POINT ( 'NONE',  ( 2.005403748902764516, -15.69871118693741430, 5.609036204238825540 ) ) ;
#39964=CIRCLE ( 'NONE', #20884, 3.175000000000001155 ) ;
#39966=CARTESIAN_POINT ( 'NONE',  ( -4.543664835419952475, 118.0881836969183070, -0.7497823245519673607 ) ) ;
#39970=CARTESIAN_POINT ( 'NONE',  ( 4.111708801323036511, 118.2429491485453354, 0.3463700888942771727 ) ) ;
#39971=CARTESIAN_POINT ( 'NONE',  ( 15.87222905729431943, 135.0473088626721392, 2.190551936964585611 ) ) ;
#39973=CARTESIAN_POINT ( 'NONE',  ( 3.707388773974296559, 116.6237204831772232, 0.06043239539139045463 ) ) ;
#39974=CARTESIAN_POINT ( 'NONE',  ( -7.794209556482943668, 13.03656553185805222, 3.210957146378262461 ) ) ;
#39975=CARTESIAN_POINT ( 'NONE',  ( 9.418980095613568082, 123.9587481073520223, 0.7032982658115918273 ) ) ;
#39976=CARTESIAN_POINT ( 'NONE',  ( 16.18247977474483079, 122.8183540351560907, -0.6517309543831906193 ) ) ;
#39977=EDGE_CURVE ( 'NONE', #40944, #1213, #13312, .T. ) ;
#39979=CARTESIAN_POINT ( 'NONE',  ( 0.06584543127246964000, 115.6909491485452719, 1.765419582720901825 ) ) ;
#39980=EDGE_CURVE ( 'NONE', #29654, #29150, #24174, .T. ) ;
#39981=CARTESIAN_POINT ( 'NONE',  ( -14.87733005835129063, 120.3210621052586475, -0.2473824415510233188 ) ) ;
#39982=ORIENTED_EDGE ( 'NONE', *, *, #7838, .F. ) ;
#39984=CARTESIAN_POINT ( 'NONE',  ( 6.835380503559908227, 121.3218668833306992, -0.5961742291405608407 ) ) ;
#39986=ORIENTED_EDGE ( 'NONE', *, *, #9443, .F. ) ;
#39987=CARTESIAN_POINT ( 'NONE',  ( -1.598479218588914730, 156.2658572007470639, -0.3094434466263948913 ) ) ;
#39988=CARTESIAN_POINT ( 'NONE',  ( 4.668376822648329316, -11.99306229768662391, 1.198378876927704839 ) ) ;
#39989=CARTESIAN_POINT ( 'NONE',  ( -22.07843093565582038, 149.7938220333360846, 0.9986438184040021815 ) ) ;
#39991=CARTESIAN_POINT ( 'NONE',  ( 1.804784692667541268, 116.4728921782852922, 0.07541441754812436282 ) ) ;
#39994=CARTESIAN_POINT ( 'NONE',  ( 2.294499597581835193, -9.852027417895397932, -4.012603411698490774 ) ) ;
#39995=CARTESIAN_POINT ( 'NONE',  ( -5.757472737270721730, 159.1136035536173097, -0.1150480073142621795 ) ) ;
#40000=CARTESIAN_POINT ( 'NONE',  ( 4.914704081444464023, 119.0942267931248040, 1.098002887962306495 ) ) ;
#40001=CARTESIAN_POINT ( 'NONE',  ( 3.573240411403531436, -4.819783300376494495, -2.961220487682875824 ) ) ;
#40002=CARTESIAN_POINT ( 'NONE',  ( 2.005144469770952398, 117.2046888992736200, 0.5340627965622031237 ) ) ;
#40005=CARTESIAN_POINT ( 'NONE',  ( 9.293546136053006279, 157.2521837264336853, -1.575842917768122575 ) ) ;
#40006=CARTESIAN_POINT ( 'NONE',  ( -4.120466288800530563, -1.808681497221679590, -2.133573495687988597 ) ) ;
#40007=CARTESIAN_POINT ( 'NONE',  ( -2.946415863239081556, 117.2422168882539211, -0.6071713939981749908 ) ) ;
#40008=VERTEX_POINT ( 'NONE', #3795 ) ;
#40009=CARTESIAN_POINT ( 'NONE',  ( -9.679874449561454597, 124.8500477395539576, -0.02572261534930060309 ) ) ;
#40010=CARTESIAN_POINT ( 'NONE',  ( 5.122375111755775201, -14.64399685039916044, 3.991980633533394052 ) ) ;
#40011=( BOUNDED_CURVE ( )  B_SPLINE_CURVE ( 3, ( #12948, #3601, #410, #12745 ),
 .UNSPECIFIED., .F., .T. ) 
 B_SPLINE_CURVE_WITH_KNOTS ( ( 4, 4 ),
 ( 1.570796326794896558, 3.141592653589793116 ),
 .UNSPECIFIED. ) 
 CURVE ( )  GEOMETRIC_REPRESENTATION_ITEM ( )  RATIONAL_B_SPLINE_CURVE ( ( 1.000000000000000000, 0.8047378541243649375, 0.8047378541243649375, 1.000000000000000000 ) ) 
 REPRESENTATION_ITEM ( '' )  );
#40013=TOROIDAL_SURFACE ( 'NONE', #27044, 5.080000000000005400, 0.5080000000000000071 ) ;
#40014=CARTESIAN_POINT ( 'NONE',  ( -0.07510606132778108179, 117.9496054766374158, -1.407797200287234984 ) ) ;
#40016=CARTESIAN_POINT ( 'NONE',  ( 2.337245495867128486, 157.7073581658784178, 1.721377379916721129 ) ) ;
#40018=CARTESIAN_POINT ( 'NONE',  ( -0.3623072504456354981, 117.0882377308211773, 0.3576919811193871035 ) ) ;
#40019=CARTESIAN_POINT ( 'NONE',  ( 7.688107727944508696, 4.450669244509953160, -3.435853896805545649 ) ) ;
#40020=CARTESIAN_POINT ( 'NONE',  ( 8.359771539777417715, 154.6912814427390970, 1.273680951853117138 ) ) ;
#40021=DIRECTION ( 'NONE',  ( -0.9998004120163609398, 0.000000000000000000, -0.01997839162482749689 ) ) ;
#40022=CARTESIAN_POINT ( 'NONE',  ( 15.62635203013925889, 121.2802728028965475, -0.2997488694636321060 ) ) ;
#40029=CARTESIAN_POINT ( 'NONE',  ( -4.385328315531485721, 118.1846248134211379, 0.4263140361897638231 ) ) ;
#40033=CARTESIAN_POINT ( 'NONE',  ( 6.170393643008810436, 119.5853013911638811, -1.006946838071717032 ) ) ;
#40034=CARTESIAN_POINT ( 'NONE',  ( -3.916844122728852184, 109.8065891650451249, -3.681372831196203066 ) ) ;
#40035=CARTESIAN_POINT ( 'NONE',  ( 4.491247496296435493, 118.1274053408948390, 0.6814523630037505608 ) ) ;
#40036=CARTESIAN_POINT ( 'NONE',  ( -15.61785206596079689, 148.1291547725267037, -1.273309296088947828 ) ) ;
#40038=CARTESIAN_POINT ( 'NONE',  ( -0.8519111957592009343, 115.7029491485453576, -1.752612029837606666 ) ) ;
#40040=FACE_OUTER_BOUND ( 'NONE', #5090, .T. ) ;
#40041=CARTESIAN_POINT ( 'NONE',  ( -8.650892266477143266, 122.3401343867201945, -1.081441824013609443 ) ) ;
#40044=CARTESIAN_POINT ( 'NONE',  ( 7.931359276468123554, 121.9896588117074998, -0.6306316981394162191 ) ) ;
#40045=CARTESIAN_POINT ( 'NONE',  ( -0.001427691597722236970, 156.3034662015458593, 0.07144752562581345445 ) ) ;
#40046=CARTESIAN_POINT ( 'NONE',  ( -6.550797450135577910E-14, 84.67546620154573134, 2.164564701558966795E-29 ) ) ;
#40047=CARTESIAN_POINT ( 'NONE',  ( 5.829268545577174443, 117.2350771734024164, 0.5950018394081721951 ) ) ;
#40049=CARTESIAN_POINT ( 'NONE',  ( 3.065366080762625955, -14.95244456720379311, 3.762810261076596330 ) ) ;
#40050=CARTESIAN_POINT ( 'NONE',  ( -18.50543525367162090, 148.3462492009778373, 1.698196615343024796 ) ) ;
#40051=CARTESIAN_POINT ( 'NONE',  ( -0.5824522774871869757, -3.319493544524417583, -0.7801697309090062094 ) ) ;
#40052=CARTESIAN_POINT ( 'NONE',  ( -5.580240031299428694, 159.0849926622337023, -0.6989143883095924048 ) ) ;
#40053=CARTESIAN_POINT ( 'NONE',  ( -0.7070771686734943495, -4.675651901196332005, 0.6724949525944122763 ) ) ;
#40056=CARTESIAN_POINT ( 'NONE',  ( 5.908534618823872542, 118.9825038774357466, 0.5858829404670616858 ) ) ;
#40057=CARTESIAN_POINT ( 'NONE',  ( -4.443995521150195138, 155.8637389808261275, 0.5396741685193008342 ) ) ;
#40058=CARTESIAN_POINT ( 'NONE',  ( 2.417269819423324861, -15.13903239461346395, 5.861448462117607505 ) ) ;
#40059=CARTESIAN_POINT ( 'NONE',  ( 16.84814155439267935, 148.3581316477378493, -1.364645798843572733 ) ) ;
#40060=ORIENTED_EDGE ( 'NONE', *, *, #1932, .T. ) ;
#40061=CARTESIAN_POINT ( 'NONE',  ( -15.19444909298876567, 153.0676604005411434, -2.356382943223728876 ) ) ;
#40063=CARTESIAN_POINT ( 'NONE',  ( -1.157812389576497347, 104.6144662015457669, 4.694735647536337098 ) ) ;
#40064=CARTESIAN_POINT ( 'NONE',  ( 3.075357915497110017, -13.94103813162880989, 1.416127232796946966 ) ) ;
#40065=CARTESIAN_POINT ( 'NONE',  ( -4.944211420742701257, 117.5327897045929859, -0.9782740106667096036 ) ) ;
#40066=CARTESIAN_POINT ( 'NONE',  ( 13.61628268276109210, 150.2179846313823930, 0.04905232040057783127 ) ) ;
#40068=CARTESIAN_POINT ( 'NONE',  ( -2.561166057192335366, 106.9230564690795546, 4.673879012131969546 ) ) ;
#40069=CARTESIAN_POINT ( 'NONE',  ( 4.679650109289619664, 111.8766742161798220, 2.628376281732180075 ) ) ;
#40072=CARTESIAN_POINT ( 'NONE',  ( 18.71881220850874072, 125.2636347375217838, 0.1974931939226153843 ) ) ;
#40073=CIRCLE ( 'NONE', #30505, 0.5080000000000002292 ) ;
#40074=FACE_BOUND ( 'NONE', #8055, .T. ) ;
#40075=CARTESIAN_POINT ( 'NONE',  ( 2.064435910936676777, -15.27355197655908015, 5.962396817882995137 ) ) ;
#40077=CARTESIAN_POINT ( 'NONE',  ( -4.845170713328630363, 117.7576911979032559, -0.9526118176995749254 ) ) ;
#40078=CARTESIAN_POINT ( 'NONE',  ( 14.40940766795059069, 123.3930721568691382, 1.837956572252896104 ) ) ;
#40080=CARTESIAN_POINT ( 'NONE',  ( -7.524129562762011503, 22.75916136179084859, 3.848622047589015160 ) ) ;
#40081=CARTESIAN_POINT ( 'NONE',  ( -8.593394099080960302, 118.5896537841807969, -1.127171445019202300 ) ) ;
#40082=CARTESIAN_POINT ( 'NONE',  ( -3.662133038521701245, 120.6652674781340551, -0.4257566204602384330 ) ) ;
#40084=CARTESIAN_POINT ( 'NONE',  ( -0.4201689423133995183, 106.0154168944984434, -5.283495245356437664 ) ) ;
#40085=CARTESIAN_POINT ( 'NONE',  ( -0.007670926888326720997, 121.5961256765098284, 0.3838845493045228707 ) ) ;
#40086=CARTESIAN_POINT ( 'NONE',  ( 0.3994026957563919789, 5.465888722076803319, 4.619092260001838923 ) ) ;
#40088=CARTESIAN_POINT ( 'NONE',  ( -4.789447579930971699, 118.5264896598256854, 0.8320597001846437024 ) ) ;
#40089=CARTESIAN_POINT ( 'NONE',  ( 2.946624452826990925, -14.63926610985447141, 4.195571020465345136 ) ) ;
#40090=CARTESIAN_POINT ( 'NONE',  ( 5.854942301702412699, 124.9344662015456890, 0.1169956811762815629 ) ) ;
#40091=CARTESIAN_POINT ( 'NONE',  ( -5.566083668711205412, 159.0643023895801491, 0.5661052595122398889 ) ) ;
#40092=CARTESIAN_POINT ( 'NONE',  ( -4.171639465256384405, 28.89343014676064669, 2.695540212632123289 ) ) ;
#40095=CARTESIAN_POINT ( 'NONE',  ( -5.282613984594703105, 105.1224582691644258, -0.7587507295933431095 ) ) ;
#40096=CARTESIAN_POINT ( 'NONE',  ( 4.512673509771836677, -15.64532105467335299, 2.834742450761120303 ) ) ;
#40097=CARTESIAN_POINT ( 'NONE',  ( -3.234792161733187843, 118.6508749770327995, 0.7732002099368725512 ) ) ;
#40098=CARTESIAN_POINT ( 'NONE',  ( -0.7219274401084647685, 31.37879824840181442, -0.6700674276139703123 ) ) ;
#40101=CARTESIAN_POINT ( 'NONE',  ( 0.5374927741465299613, 112.6282971158091470, 2.756357034314327770 ) ) ;
#40103=CARTESIAN_POINT ( 'NONE',  ( -17.00728043862078565, 146.2370505443881257, 1.250989154318494556 ) ) ;
#40106=CARTESIAN_POINT ( 'NONE',  ( 4.259301615573734878, 119.5670751559891585, -0.7808790134437380015 ) ) ;
#40108=CARTESIAN_POINT ( 'NONE',  ( -8.976454200711149412, 119.5326672034033777, -1.412516637748555404 ) ) ;
#40111=CARTESIAN_POINT ( 'NONE',  ( 4.163732346407177154, 118.2394253532318373, -0.2271039051975612677 ) ) ;
#40112=CARTESIAN_POINT ( 'NONE',  ( 0.6220149250934452478, 120.7813932625355307, -0.1825499261673580731 ) ) ;
#40113=B_SPLINE_CURVE_WITH_KNOTS ( 'NONE', 3,
 ( #4599, #11958, #17353, #30342, #39753, #40375, #28145, #40168 ),
 .UNSPECIFIED., .F., .F.,
 ( 4, 2, 2, 4 ),
 ( 0.7435342612792388284, 0.8019765719082849742, 0.8679843812721900198, 1.000000000000000000 ),
 .UNSPECIFIED. ) ;
#40114=ORIENTED_EDGE ( 'NONE', *, *, #28132, .T. ) ;
#40115=CARTESIAN_POINT ( 'NONE',  ( 3.252851485128089415, -14.73889851401814788, 2.797586445667359811 ) ) ;
#40118=CARTESIAN_POINT ( 'NONE',  ( 3.019445949670579665, 11.99742794009110014, 3.522755186455234000 ) ) ;
#40119=CARTESIAN_POINT ( 'NONE',  ( 8.769168840778068130, 122.1986804192922875, 1.175795117382457677 ) ) ;
#40120=CARTESIAN_POINT ( 'NONE',  ( -2.889499560705188319, 30.91168237226732884, 0.4695966336271347741 ) ) ;
#40121=CARTESIAN_POINT ( 'NONE',  ( -0.1065646865916160396, 105.8844662015456777, 5.332932678536313809 ) ) ;
#40123=CARTESIAN_POINT ( 'NONE',  ( -1.287880193524239658, 20.15907059199006923, -4.440276399826991849 ) ) ;
#40124=CARTESIAN_POINT ( 'NONE',  ( 15.26387433774249835, 148.0131224598485744, 0.4327379813662103891 ) ) ;
#40125=CARTESIAN_POINT ( 'NONE',  ( -2.483897188070747664, 106.8186250688659555, 4.725446615029760267 ) ) ;
#40126=EDGE_CURVE ( 'NONE', #19701, #39565, #19133, .T. ) ;
#40127=AXIS2_PLACEMENT_3D ( 'NONE', #21954, #17560, #21740 ) ;
#40130=CARTESIAN_POINT ( 'NONE',  ( -2.171138432512356609, 116.2511519099119681, -0.2036645720446532970 ) ) ;
#40135=CARTESIAN_POINT ( 'NONE',  ( 7.667154907385915763, 6.987472373264454362, 3.492918021822637442 ) ) ;
#40137=DIRECTION ( 'NONE',  ( 0.0004113621477241937948, -0.9999999153568039922, 8.219994698375953989E-06 ) ) ;
#40140=CARTESIAN_POINT ( 'NONE',  ( -0.003746264460361951702, 116.6481217037470373, 0.1874783927187338162 ) ) ;
#40141=VERTEX_POINT ( 'NONE', #24825 ) ;
#40146=CARTESIAN_POINT ( 'NONE',  ( 0.0005468344958371703160, 156.3034662015456604, -0.02736583427618478198 ) ) ;
#40147=CARTESIAN_POINT ( 'NONE',  ( 5.611355841363750763, -14.32207541480874724, 3.167021961541031327 ) ) ;
#40148=CARTESIAN_POINT ( 'NONE',  ( -20.89924265627231748, 149.3152741295656369, 1.514357740512881190 ) ) ;
#40149=CARTESIAN_POINT ( 'NONE',  ( 15.20946960781365043, 120.7148350616293300, 0.7222319099908602880 ) ) ;
#40150=CARTESIAN_POINT ( 'NONE',  ( 15.37733514790036438, 147.8388096571506765, 0.5071817389179859026 ) ) ;
#40152=CARTESIAN_POINT ( 'NONE',  ( 0.3959014520675726012, 0.7218480974852773402, -0.8918910426260873159 ) ) ;
#40153=CARTESIAN_POINT ( 'NONE',  ( -22.94033276177410485, 150.1476136049543868, -0.7879714733284356454 ) ) ;
#40157=CARTESIAN_POINT ( 'NONE',  ( 2.212278878456643838, 116.2471469023566470, 0.1464055763033723367 ) ) ;
#40158=CARTESIAN_POINT ( 'NONE',  ( -16.98902716506020028, 149.6223975874448229, 1.623990461445593114 ) ) ;
#40160=CARTESIAN_POINT ( 'NONE',  ( 19.06420633224110261, 149.2349160008635351, -1.736338202726219304 ) ) ;
#40161=CARTESIAN_POINT ( 'NONE',  ( 0.9553521702984651975, -6.993735180969975929, 0.1873809170862112405 ) ) ;
#40162=CARTESIAN_POINT ( 'NONE',  ( -21.43631064271318465, 148.9071063441643048, -2.241374363660425306 ) ) ;
#40164=CARTESIAN_POINT ( 'NONE',  ( 4.372915526554613130, 104.6144662015457527, 2.049786579545553877 ) ) ;
#40165=ADVANCED_FACE ( 'NONE', ( #14810 ), #8222, .T. ) ;
#40166=AXIS2_PLACEMENT_3D ( 'NONE', #9604, #9816, #16188 ) ;
#40167=CARTESIAN_POINT ( 'NONE',  ( 15.22619620759357950, 139.4722935914273307, -0.9828944228028647645 ) ) ;
#40168=CARTESIAN_POINT ( 'NONE',  ( -5.008552712180506461, 117.3993836135855560, 0.7755994290793736257 ) ) ;
#40170=CARTESIAN_POINT ( 'NONE',  ( -10.24420426168412490, 122.2012759285571946, -1.550633339661970478 ) ) ;
#40171=CARTESIAN_POINT ( 'NONE',  ( 4.998192975942944649, -15.53260140147937030, 2.284796345537305928 ) ) ;
#40172=CARTESIAN_POINT ( 'NONE',  ( -4.801687489738192482, 117.4019780203432646, 1.015655943361054581 ) ) ;
#40173=CARTESIAN_POINT ( 'NONE',  ( -4.418207565432228812, 118.1647756611046276, -0.6321334375057892085 ) ) ;
#40176=CARTESIAN_POINT ( 'NONE',  ( 13.94976549039465397, 152.5802402909829425, 2.190326936676450842 ) ) ;
#40178=CARTESIAN_POINT ( 'NONE',  ( 23.34372044207203700, 149.0681261006882039, 0.4664630893996631333 ) ) ;
#40181=CARTESIAN_POINT ( 'NONE',  ( 3.595709101656964890, 5.917279480223868404, 7.636340781540109646 ) ) ;
#40182=CARTESIAN_POINT ( 'NONE',  ( 7.055095707297161844, 122.0164807696326790, 0.4009610655988182781 ) ) ;
#40183=CARTESIAN_POINT ( 'NONE',  ( 22.70688998881770360, 149.0844379882532849, -0.7271790501850812216 ) ) ;
#40184=CARTESIAN_POINT ( 'NONE',  ( -3.174366308152013705, 104.1064662015457287, -0.06343139340882732180 ) ) ;
#40189=CARTESIAN_POINT ( 'NONE',  ( -20.42271720105693333, 129.0384130229076334, -0.2828206407990417892 ) ) ;
#40192=CARTESIAN_POINT ( 'NONE',  ( -7.886840516052592065, 122.0567478468350799, -0.9062200922211768317 ) ) ;
#40193=CARTESIAN_POINT ( 'NONE',  ( -8.625062891301432444, 118.6226016915422719, 0.7970602507507228429 ) ) ;
#40194=ORIENTED_EDGE ( 'NONE', *, *, #27489, .T. ) ;
#40195=CARTESIAN_POINT ( 'NONE',  ( 0.8425567758001710761, 115.6909491485452719, -1.725004630648912185 ) ) ;
#40196=CARTESIAN_POINT ( 'NONE',  ( -15.80292465353841713, 145.7390459690742830, -0.7709107363076876940 ) ) ;
#40197=CARTESIAN_POINT ( 'NONE',  ( 4.664530445857379526, -12.43571634592606578, 1.922475882534872449 ) ) ;
#40198=CARTESIAN_POINT ( 'NONE',  ( -15.97727112977748831, 122.8751182158008959, 0.7600457325971274880 ) ) ;
#40199=CARTESIAN_POINT ( 'NONE',  ( -6.642767299088215313E-14, 101.1854662015457365, -1.199848199765585135E-18 ) ) ;
#40200=CARTESIAN_POINT ( 'NONE',  ( 2.754305024641273025, 116.5489981622532127, 0.1298538421819644684 ) ) ;
#40203=CARTESIAN_POINT ( 'NONE',  ( -4.595132424582489605, -6.828429371805166959, -0.5093739664528403877 ) ) ;
#40204=CARTESIAN_POINT ( 'NONE',  ( -22.66375647020928952, 150.6386093215955100, -0.4528757910175258972 ) ) ;
#40205=CARTESIAN_POINT ( 'NONE',  ( -3.174366308152013261, 101.6934662015457320, -0.06343139340882730792 ) ) ;
#40208=CARTESIAN_POINT ( 'NONE',  ( 5.325320179608937998, 119.5216941149903676, 1.109481133952169296 ) ) ;
#40209=CARTESIAN_POINT ( 'NONE',  ( 1.463615122064738427, -3.970138727222522590, -4.384008014421088895 ) ) ;
#40210=CARTESIAN_POINT ( 'NONE',  ( 6.844670616442288136, 117.9658002137636856, 0.9618333202595321652 ) ) ;
#40212=CARTESIAN_POINT ( 'NONE',  ( 17.07772634048045646, 128.5677977248401476, -1.430458439683570893 ) ) ;
#40213=CARTESIAN_POINT ( 'NONE',  ( -3.663749374568059380, -0.07195744677916669774, 2.838909333946205482 ) ) ;
#40214=CARTESIAN_POINT ( 'NONE',  ( -3.898539657838600903, 117.3164332630744298, -0.6789226234856290398 ) ) ;
#40218=CARTESIAN_POINT ( 'NONE',  ( -10.45649748849141680, 153.0728660266736370, 0.08902316335936741321 ) ) ;
#40219=EDGE_CURVE ( 'NONE', #17174, #35234, #5852, .T. ) ;
#40220=CARTESIAN_POINT ( 'NONE',  ( 2.293780832555937010, -15.47183500671027367, 5.912194120686782739 ) ) ;
#40226=CARTESIAN_POINT ( 'NONE',  ( 12.00151653869053803, 122.4500365997666336, 1.784698555944021159 ) ) ;
#40228=CARTESIAN_POINT ( 'NONE',  ( 5.078986093043054595, 66.64146620154573952, 0.1014902294541243921 ) ) ;
#40229=CARTESIAN_POINT ( 'NONE',  ( -21.51828904745235960, 136.6907720476960435, 0.8331038389761595830 ) ) ;
#40230=CARTESIAN_POINT ( 'NONE',  ( -6.994280559954464849, 7.701067304790329082, -4.726517096957497444 ) ) ;
#40231=CARTESIAN_POINT ( 'NONE',  ( 16.11589901136876790, 145.8839827664328368, 1.295141180005177750 ) ) ;
#40234=CARTESIAN_POINT ( 'NONE',  ( 22.34885681094289822, 150.7328461917231550, -0.2743282927392729498 ) ) ;
#40237=VECTOR ( 'NONE', #2808, 1000.000000000000114 ) ;
#40240=CARTESIAN_POINT ( 'NONE',  ( -4.533795937410928900, 118.1203770736758116, 0.4771152162569446409 ) ) ;
#40241=CARTESIAN_POINT ( 'NONE',  ( 3.070893729975305853, 107.8345691433024172, -4.352706817367781866 ) ) ;
#40243=ORIENTED_EDGE ( 'NONE', *, *, #8453, .T. ) ;
#40245=CARTESIAN_POINT ( 'NONE',  ( 8.333504027011557014, 120.0758091897315722, -1.117991676638815601 ) ) ;
#40246=CARTESIAN_POINT ( 'NONE',  ( 0.1065646865915093611, 105.8844662015456777, -5.332932678536313809 ) ) ;
#40248=CARTESIAN_POINT ( 'NONE',  ( 4.558520316232089975, 118.0156047093444585, 0.8817180759835696602 ) ) ;
#40249=CARTESIAN_POINT ( 'NONE',  ( -9.619667158014763686, 123.8920215319950842, -0.8772578247576549026 ) ) ;
#40250=CARTESIAN_POINT ( 'NONE',  ( -0.3620645665610385255, 115.7033447612903103, -1.764050604746122852 ) ) ;
#40251=CARTESIAN_POINT ( 'NONE',  ( 3.413761347186222483, 117.3993835099294643, -1.238230392815611758 ) ) ;
#40252=CARTESIAN_POINT ( 'NONE',  ( 5.103137870717143088, 114.3519703858145959, -1.758966173294684632 ) ) ;
#40253=CARTESIAN_POINT ( 'NONE',  ( -1.456364663600036691, 120.2326517397585377, -0.4672470943647332731 ) ) ;
#40254=CARTESIAN_POINT ( 'NONE',  ( -5.332935397695336199, 116.0444662015457311, -0.1065647409268299234 ) ) ;
#40256=EDGE_CURVE ( 'NONE', #12250, #15268, #16818, .T. ) ;
#40258=CARTESIAN_POINT ( 'NONE',  ( -2.869904849639449029, 156.1076442532932731, 0.07316186139488585483 ) ) ;
#40260=CARTESIAN_POINT ( 'NONE',  ( 18.03394523526729643, 125.1493905788104684, 1.135097528960560487 ) ) ;
#40262=CARTESIAN_POINT ( 'NONE',  ( 3.216867006742271329, -14.81339725456490264, 3.133484537391586944 ) ) ;
#40263=CARTESIAN_POINT ( 'NONE',  ( -18.22015820038736678, 148.8986565181125457, 1.699282175587853549 ) ) ;
#40265=CARTESIAN_POINT ( 'NONE',  ( 0.9728917428133897483, -6.565010040704528649, -0.08600706860408523224 ) ) ;
#40266=CARTESIAN_POINT ( 'NONE',  ( -16.67457936879075930, 122.7093839631038463, -0.9722687365115703084 ) ) ;
#40267=CARTESIAN_POINT ( 'NONE',  ( -0.2169513509689728059, 19.34598098455444770, 0.9497947498389193166 ) ) ;
#40270=CARTESIAN_POINT ( 'NONE',  ( 2.490049542275739825, 107.2224589468338536, 4.730309301830580182 ) ) ;
#40271=CARTESIAN_POINT ( 'NONE',  ( -6.498933901768386256, 121.5572409441427482, 0.3210307352789210089 ) ) ;
#40272=CARTESIAN_POINT ( 'NONE',  ( 4.422138279315844578, -13.30579995099732926, 3.341551838899307736 ) ) ;
#40273=CARTESIAN_POINT ( 'NONE',  ( 2.030192889891265118, 156.8313070664539168, -1.335154060002984089 ) ) ;
#40275=CARTESIAN_POINT ( 'NONE',  ( -1.756936351882958158, 104.6144662015457527, 4.504134836993110014 ) ) ;
#40276=CIRCLE ( 'NONE', #21854, 3.683000000000001162 ) ;
#40278=CARTESIAN_POINT ( 'NONE',  ( 3.114041961411902371, -14.44963006906317737, 3.768961988127400353 ) ) ;
#40279=CARTESIAN_POINT ( 'NONE',  ( -4.899464968550142352, 117.6324563737643700, -0.9916011361669829771 ) ) ;
#40281=CARTESIAN_POINT ( 'NONE',  ( 14.20283082469467217, 138.9094276006951247, 0.1579304324436909823 ) ) ;
#40284=CARTESIAN_POINT ( 'NONE',  ( 0.4360227397040848385, 118.4074432378348689, 0.6062663470103506480 ) ) ;
#40286=CARTESIAN_POINT ( 'NONE',  ( 1.969680065291609994, 117.3993837346511384, 1.449778539274672262 ) ) ;
#40287=CARTESIAN_POINT ( 'NONE',  ( 0.03245814172805068509, 158.1186941186938952, -1.624338139048501217 ) ) ;
#40288=CARTESIAN_POINT ( 'NONE',  ( 3.286349204026739468, 159.4678586119998442, -0.07386938312792008798 ) ) ;
#40289=DIRECTION ( 'NONE',  ( -0.9998004120163608288, 0.000000000000000000, -0.01997839162482749342 ) ) ;
#40290=CARTESIAN_POINT ( 'NONE',  ( 1.893654310830311882, -15.30438151921108236, 5.998987748567822464 ) ) ;
#40292=CARTESIAN_POINT ( 'NONE',  ( 0.1949087904810302418, 33.82644263972942156, 0.4054292462034596034 ) ) ;
#40293=CARTESIAN_POINT ( 'NONE',  ( 20.49864673575774532, 149.5144255282053223, 2.384675166241297717 ) ) ;
#40295=CARTESIAN_POINT ( 'NONE',  ( -6.161128625374170831, 23.17997237347384853, 5.746845633999829950 ) ) ;
#40296=CARTESIAN_POINT ( 'NONE',  ( 5.534489273878227422, 117.7316410755767038, -0.8034299031018331538 ) ) ;
#40297=CARTESIAN_POINT ( 'NONE',  ( -4.252685754339997182, 122.9893884486272526, -0.2003490066864923314 ) ) ;
#40298=DIRECTION ( 'NONE',  ( 4.017660918040594346E-17, -1.000000000000000000, -2.376309959284834438E-19 ) ) ;
#40300=CARTESIAN_POINT ( 'NONE',  ( -0.01331772328581275200, 119.9741034315943864, 0.6664733318052136202 ) ) ;
#40301=AXIS2_PLACEMENT_3D ( 'NONE', #21546, #28806, #31154 ) ;
#40302=CARTESIAN_POINT ( 'NONE',  ( -4.012847786888796620, 11.73797844546971270, -2.294585225469591983 ) ) ;
#40304=CARTESIAN_POINT ( 'NONE',  ( -3.685234504066145167, 108.9296531859112633, -3.861079628948677289 ) ) ;
#40305=CARTESIAN_POINT ( 'NONE',  ( 3.213330078112610177, -12.77372567451348573, 1.108568753689092690 ) ) ;
#40306=CARTESIAN_POINT ( 'NONE',  ( 2.922973558833750207, 114.3344743418335128, -2.013556875909916943 ) ) ;
#40307=CARTESIAN_POINT ( 'NONE',  ( -6.616924617768071466E-14, 97.37546620154573418, 7.965525879364083286E-30 ) ) ;
#40309=ORIENTED_EDGE ( 'NONE', *, *, #34161, .T. ) ;
#40310=CARTESIAN_POINT ( 'NONE',  ( -2.763873622044191958, 104.6144662015457243, -3.957344514305136673 ) ) ;
#40311=CARTESIAN_POINT ( 'NONE',  ( 2.515823494799488191, -15.76102479606726625, 5.403604998519412561 ) ) ;
#40312=CARTESIAN_POINT ( 'NONE',  ( -6.324931890614157837, 157.3995435888475072, 1.705594245970836642 ) ) ;
#40313=CARTESIAN_POINT ( 'NONE',  ( -0.3664848240473963514, 30.73350494673895739, -0.9073219246443798847 ) ) ;
#40318=CARTESIAN_POINT ( 'NONE',  ( 2.813253328531081898, 121.9077826007922312, 0.2952959765298341366 ) ) ;
#40320=CARTESIAN_POINT ( 'NONE',  ( -3.332096981533035684, 156.3062290909284116, 1.017430637527963810 ) ) ;
#40321=DIRECTION ( 'NONE',  ( -0.9998004120163610509, -4.016384292689131511E-17, -0.01997839162482749689 ) ) ;
#40322=CARTESIAN_POINT ( 'NONE',  ( 3.942276470047239467, 157.0187206368471209, -1.592783893122187155 ) ) ;
#40323=CARTESIAN_POINT ( 'NONE',  ( -19.16059698253096144, 135.9655892003723636, -2.351238754465550862 ) ) ;
#40325=CARTESIAN_POINT ( 'NONE',  ( 4.408657250832476393, 118.1814690201069311, -0.3998733507563780321 ) ) ;
#40326=CARTESIAN_POINT ( 'NONE',  ( 7.681492011331848779, 122.2986020547093915, -0.2830363146464229263 ) ) ;
#40328=CARTESIAN_POINT ( 'NONE',  ( 3.162461164278121739, -14.57801340048104777, 3.369881103115548893 ) ) ;
#40332=CARTESIAN_POINT ( 'NONE',  ( 4.409325496788552456, -14.99073161069602911, -1.440227693534741782 ) ) ;
#40333=CARTESIAN_POINT ( 'NONE',  ( 16.56824576912627478, 144.0643239018434940, 1.930375849691871926 ) ) ;
#40334=CARTESIAN_POINT ( 'NONE',  ( -3.890668369019033790, 28.55756886444902065, 1.917437575001416539 ) ) ;
#40335=CARTESIAN_POINT ( 'NONE',  ( -4.812498123319443266, 116.8297769931967309, 0.8564213435964300736 ) ) ;
#40336=CARTESIAN_POINT ( 'NONE',  ( -3.366035089439492811, 13.68705809737886447, 3.178168622443589886 ) ) ;
#40337=CARTESIAN_POINT ( 'NONE',  ( 9.190025975545930592, 124.2403664864748549, 0.2180328680397459196 ) ) ;
#40338=CARTESIAN_POINT ( 'NONE',  ( 5.328530153152057913, 115.6909491485453145, 0.4168410533107074212 ) ) ;
#40341=CARTESIAN_POINT ( 'NONE',  ( 8.796826986025713779, 117.7047326868996180, 0.02773673846713334279 ) ) ;
#40342=CARTESIAN_POINT ( 'NONE',  ( -5.078986093043186045, 94.32746620154571815, -0.1014902294541231709 ) ) ;
#40344=CARTESIAN_POINT ( 'NONE',  ( 1.930844028328119188, -15.65960119559217745, 5.531553210582127456 ) ) ;
#40346=CARTESIAN_POINT ( 'NONE',  ( -6.572471397769512613, 1.803772144246908127, -5.323917895317753946 ) ) ;
#40348=LINE ( 'NONE', #7959, #34146 ) ;
#40350=CARTESIAN_POINT ( 'NONE',  ( -6.504806966450658722E-14, 124.9344662015457317, 5.107768156065721555E-17 ) ) ;
#40351=CARTESIAN_POINT ( 'NONE',  ( -23.04498962259538075, 149.8694456586574972, -0.007884547560928519341 ) ) ;
#40356=CARTESIAN_POINT ( 'NONE',  ( -5.308493528853332144, 121.3525139070573147, -0.1060763342189515873 ) ) ;
#40357=CARTESIAN_POINT ( 'NONE',  ( 5.253792623460133981, -14.56763799980149976, 3.797339299194151696 ) ) ;
#40358=CARTESIAN_POINT ( 'NONE',  ( -6.856369467415258434, 157.9234729166680040, 1.555392933271967149 ) ) ;
#40360=CARTESIAN_POINT ( 'NONE',  ( 23.06466230714210752, 149.5685596498530288, 1.055262110361127270 ) ) ;
#40361=CARTESIAN_POINT ( 'NONE',  ( 0.3722574617741854497, 117.2097358735305050, -0.3924287308447400591 ) ) ;
#40362=CARTESIAN_POINT ( 'NONE',  ( 4.496586626007489151, 27.28078351817337222, -1.068494511273165193 ) ) ;
#40363=CARTESIAN_POINT ( 'NONE',  ( 0.002426349801082275555, 116.5266044092193880, -0.1214244658147704548 ) ) ;
#40366=CARTESIAN_POINT ( 'NONE',  ( -8.797438454481680381, 117.7000120450088048, -0.04557994465076498081 ) ) ;
#40367=CARTESIAN_POINT ( 'NONE',  ( -13.85457725998124801, 128.5353789189983900, 1.357273257441081071 ) ) ;
#40369=CARTESIAN_POINT ( 'NONE',  ( 5.879203592408400958, 119.4106843418347950, -0.9594678464101259463 ) ) ;
#40370=CARTESIAN_POINT ( 'NONE',  ( 0.7944722411588411859, -7.641519016208866866, 0.5639076281424253434 ) ) ;
#40371=CARTESIAN_POINT ( 'NONE',  ( -2.834005798679621435, 158.8946464937287999, -1.432308184773209980 ) ) ;
#40374=CARTESIAN_POINT ( 'NONE',  ( 9.903729432088722362, 123.6875948057429895, -0.6970279851166613083 ) ) ;
#40375=CARTESIAN_POINT ( 'NONE',  ( -4.981834297919686350, 117.5302800348309518, 0.7676192988303492948 ) ) ;
#40377=CARTESIAN_POINT ( 'NONE',  ( -11.35704730865809253, 122.8492764348241337, -1.683887364911069051 ) ) ;
#40378=CARTESIAN_POINT ( 'NONE',  ( 5.293312112441732609, -15.32963308811979886, 0.4416779358531437993 ) ) ;
#40380=CARTESIAN_POINT ( 'NONE',  ( -4.398970153489806023, 118.1654313746710159, -0.6513127681900948707 ) ) ;
#40383=CARTESIAN_POINT ( 'NONE',  ( 2.462641994822346803, 119.6096776070104681, 0.7191205607878171646 ) ) ;
#40385=CARTESIAN_POINT ( 'NONE',  ( 14.91134437181069927, 120.3281135998953459, 0.2979641475761142244 ) ) ;
#40386=CARTESIAN_POINT ( 'NONE',  ( 8.383109624418931816, 7.835852165998051788, -1.087619381312709077 ) ) ;
#40387=CARTESIAN_POINT ( 'NONE',  ( 1.571702145576592935, 120.8584627942791627, 0.1987642453017053890 ) ) ;
#40389=CARTESIAN_POINT ( 'NONE',  ( 18.09030135340791290, 154.0913862843578670, -0.7524810965364957527 ) ) ;
#40391=CARTESIAN_POINT ( 'NONE',  ( -0.02551629668048742416, 118.7629491485454025, 1.276939826301574987 ) ) ;
#40394=CARTESIAN_POINT ( 'NONE',  ( -15.52360445758517216, 120.7153972339879715, -0.2596658046059212577 ) ) ;
#40397=CARTESIAN_POINT ( 'NONE',  ( 5.895458498755588472, 121.3261075308788719, -0.1611362123841119653 ) ) ;
#40400=CARTESIAN_POINT ( 'NONE',  ( -5.586884702347496123, 92.04146620154574521, -0.1116392523995361624 ) ) ;
#40401=CARTESIAN_POINT ( 'NONE',  ( -2.922188055539197915, 156.0861408873597327, -0.2775485887099102267 ) ) ;
#40402=CARTESIAN_POINT ( 'NONE',  ( 4.778187575955942457, -13.11831155531867310, 3.026993680286476973 ) ) ;
#40403=CARTESIAN_POINT ( 'NONE',  ( -19.46267448186344495, 131.9512773411433670, 1.172478082078345585 ) ) ;
#40404=CARTESIAN_POINT ( 'NONE',  ( -6.431420355030265265E-14, 156.3034662015457172, 9.897580308537652682E-17 ) ) ;
#40405=CARTESIAN_POINT ( 'NONE',  ( 23.10027255048446548, 149.8968678342272653, 0.6153025774343642285 ) ) ;
#40406=CARTESIAN_POINT ( 'NONE',  ( 12.82793160447645953, 133.7433403788203066, 0.3179556874975825731 ) ) ;
#40408=CARTESIAN_POINT ( 'NONE',  ( 0.9733856798199480576, 17.99895565637743999, 0.09873697238165508872 ) ) ;
#40409=CARTESIAN_POINT ( 'NONE',  ( -8.075047650969624513, 158.6620026115301698, -0.1796671307923021765 ) ) ;
#40412=DIRECTION ( 'NONE',  ( 0.02487920782528813338, -0.9876883405951415451, 0.1544434099286914330 ) ) ;
#40413=VERTEX_POINT ( 'NONE', #38881 ) ;
#40414=CARTESIAN_POINT ( 'NONE',  ( -6.814166505432768695, 120.4085755475616253, 0.9136569436695998192 ) ) ;
#40415=CARTESIAN_POINT ( 'NONE',  ( -3.663749374568059380, -0.07195744677916669774, 2.838909333946205482 ) ) ;
#40416=CARTESIAN_POINT ( 'NONE',  ( 21.80715381475361170, 148.2155681941778482, 2.148825447453798443 ) ) ;
#40418=CARTESIAN_POINT ( 'NONE',  ( 20.71566368020593174, 149.2407879669073054, -1.563226885547172706 ) ) ;
#40420=CARTESIAN_POINT ( 'NONE',  ( -3.074427775304182209, -11.96646105551300643, -3.469969274305642060 ) ) ;
#40421=CARTESIAN_POINT ( 'NONE',  ( -21.90872843939991554, 150.3855106993079005, -1.734217137259093100 ) ) ;
#40423=VERTEX_POINT ( 'NONE', #28870 ) ;
#40424=CARTESIAN_POINT ( 'NONE',  ( -4.275377040554547037, 155.8374496918941077, 0.1508172661092593292 ) ) ;
#40426=CARTESIAN_POINT ( 'NONE',  ( 6.307811598796486230, -13.53853427790793695, 1.133914056348525934 ) ) ;
#40427=DIRECTION ( 'NONE',  ( -4.017660918040594346E-17, 1.000000000000000000, 2.376309959284834438E-19 ) ) ;
#40429=DIRECTION ( 'NONE',  ( 4.017660918040594346E-17, -1.000000000000000000, -2.376309959284834438E-19 ) ) ;
#40432=CARTESIAN_POINT ( 'NONE',  ( 14.20181026158647519, 125.7140216354555804, 2.028863013303968899 ) ) ;
#40436=CARTESIAN_POINT ( 'NONE',  ( -1.024802081479867066, 117.0751458430253393, 0.3787107017154778266 ) ) ;
#40437=CARTESIAN_POINT ( 'NONE',  ( -8.002357889267953439, 8.121853428443936096, -2.619265908643666929 ) ) ;
#40438=CARTESIAN_POINT ( 'NONE',  ( 13.61103386154286810, 134.2686865373913463, 1.213594671188916951 ) ) ;
#40440=CARTESIAN_POINT ( 'NONE',  ( 23.05353557640024675, 148.9204423966469335, -0.3945749818456246172 ) ) ;
#40444=CARTESIAN_POINT ( 'NONE',  ( -6.784104592523965728E-14, 136.3644662015457527, 7.159772606002533724E-18 ) ) ;
#40448=CARTESIAN_POINT ( 'NONE',  ( 23.36555825341164550, 148.7788340588663800, 0.4668994608413311043 ) ) ;
#40449=CARTESIAN_POINT ( 'NONE',  ( -4.121280158250598014, 118.2429491485453497, 0.1829298354757566414 ) ) ;
#40450=CARTESIAN_POINT ( 'NONE',  ( 0.1066493941974242521, 105.7853621660184444, -5.332931186019217229 ) ) ;
#40451=ORIENTED_EDGE ( 'NONE', *, *, #11857, .F. ) ;
#40454=CARTESIAN_POINT ( 'NONE',  ( 4.381439635116813669, 119.4686423241179085, -0.7540022720711342386 ) ) ;
#40455=CARTESIAN_POINT ( 'NONE',  ( -5.771537640388904045, 118.4310156723767307, -0.6642225483502960381 ) ) ;
#40456=CARTESIAN_POINT ( 'NONE',  ( 4.286528689365628253, 118.2141904594688384, 0.5114333612981697419 ) ) ;
#40457=CARTESIAN_POINT ( 'NONE',  ( -16.14702439603941286, 146.0959698922748942, -1.294960982472433519 ) ) ;
#40458=CARTESIAN_POINT ( 'NONE',  ( -1.357158281331605432, 115.7027986320083812, -1.737098550677430131 ) ) ;
#40459=ADVANCED_FACE ( 'NONE', ( #5890 ), #8642, .T. ) ;
#40460=CARTESIAN_POINT ( 'NONE',  ( 8.216926545874459364, 117.5004104479096583, 0.1641937475849289951 ) ) ;
#40461=EDGE_LOOP ( 'NONE', ( #28925, #2877, #22971, #27937 ) ) ;
#40462=CARTESIAN_POINT ( 'NONE',  ( 5.222556791543245147, 115.4535745449993982, -1.305545271932168960 ) ) ;
#40463=CARTESIAN_POINT ( 'NONE',  ( -5.855671506236725499, 121.0368588677253143, -0.7388637662663294359 ) ) ;
#40467=CARTESIAN_POINT ( 'NONE',  ( -14.11998566707450564, 138.8091548059119020, -0.08316428514401870420 ) ) ;
#40468=CARTESIAN_POINT ( 'NONE',  ( 22.26995438616699374, 150.5193240506149550, 1.407572089812798799 ) ) ;
#40470=CARTESIAN_POINT ( 'NONE',  ( 2.459637058406862309, -15.11974833578012856, 4.824092508607692231 ) ) ;
#40471=CARTESIAN_POINT ( 'NONE',  ( 21.26362230212569671, 150.1117090729339623, -1.276404781699089774 ) ) ;
#40472=CARTESIAN_POINT ( 'NONE',  ( -5.875153347143380778, 119.9178398404649926, 0.8959128733076282547 ) ) ;
#40473=CARTESIAN_POINT ( 'NONE',  ( -0.8332992110815757858, -10.66407516643697306, 0.5056687530665907593 ) ) ;
#40474=CARTESIAN_POINT ( 'NONE',  ( -4.811924804297874836, 117.0737178285515654, -0.5427311436463462258 ) ) ;
#40475=CARTESIAN_POINT ( 'NONE',  ( -0.5956917769015268593, 15.89737491555829685, -0.7703063551142234067 ) ) ;
#40478=CARTESIAN_POINT ( 'NONE',  ( -8.277497327055032272, 122.7564308547279666, 0.2971990107970639561 ) ) ;
#40479=CARTESIAN_POINT ( 'NONE',  ( 4.295506980234458538, -13.52603301450379369, 3.694598940018447575 ) ) ;
#40480=CARTESIAN_POINT ( 'NONE',  ( 0.02615319344468031854, 156.8698190429800832, -1.308812744920978099 ) ) ;
#40482=CARTESIAN_POINT ( 'NONE',  ( 3.040151308551036990, 115.7029506951511735, 1.666347003474312638 ) ) ;
#40483=CARTESIAN_POINT ( 'NONE',  ( 3.226040172055379518, -13.73821525131127608, 2.149215086980220235 ) ) ;
#40485=CARTESIAN_POINT ( 'NONE',  ( 8.961118498052918824, 123.9105667600146177, 0.1452814789513761640 ) ) ;
#40487=CARTESIAN_POINT ( 'NONE',  ( 15.97272115206776633, 153.3736753708079732, 2.320099718173297632 ) ) ;
#40488=CARTESIAN_POINT ( 'NONE',  ( 5.166455574615658186, 114.8007926982540994, 1.419721048087801307 ) ) ;
#40489=CARTESIAN_POINT ( 'NONE',  ( -9.138499898145774125, 117.7878261280527710, -0.1826089763859923554 ) ) ;
#40492=CARTESIAN_POINT ( 'NONE',  ( 17.11470313646601227, 122.7072422303320707, 0.09880859551014498088 ) ) ;
#40495=CARTESIAN_POINT ( 'NONE',  ( 2.048596186826366683, -15.20054017908126198, 5.929173703500263848 ) ) ;
#40496=CARTESIAN_POINT ( 'NONE',  ( 4.812022206586005879, 117.4092931151362933, 1.196645100868244604 ) ) ;
#40497=DIRECTION ( 'NONE',  ( -4.017660918040594346E-17, 1.000000000000000000, 2.376309959284834438E-19 ) ) ;
#40498=CARTESIAN_POINT ( 'NONE',  ( -4.677964096319726650, 117.9838868299774362, 0.6915560018011523979 ) ) ;
#40500=CARTESIAN_POINT ( 'NONE',  ( -6.940074030747619638, 22.95585651114365788, 4.785772612677765991 ) ) ;
#40501=EDGE_CURVE ( 'NONE', #5241, #24814, #28657, .T. ) ;
#40502=CARTESIAN_POINT ( 'NONE',  ( 2.700640353861210929, 117.7589353780938808, -0.7017837913142891404 ) ) ;
#40503=CARTESIAN_POINT ( 'NONE',  ( -1.464138133146304366, 108.1711930243730109, -4.389422119207357476 ) ) ;
#40504=CARTESIAN_POINT ( 'NONE',  ( 4.946784285683848204, 117.5302610941451178, 0.9662579091233235440 ) ) ;
#40505=CARTESIAN_POINT ( 'NONE',  ( -4.666417123046072035, 117.8349074441706534, -1.040161417730997462 ) ) ;
#40506=CARTESIAN_POINT ( 'NONE',  ( -4.888105396971740291, 104.6144662015479270, 2.142115408852796499 ) ) ;
#40507=CARTESIAN_POINT ( 'NONE',  ( -2.395914033174281865, 1.367755174955888275, -3.957843245732672877 ) ) ;
#40510=CARTESIAN_POINT ( 'NONE',  ( -5.066192932591571108, 115.6909491485453003, 1.197525932795551640 ) ) ;
#40511=CARTESIAN_POINT ( 'NONE',  ( 3.853068500771395399, -13.31557002055877525, 3.124774401994960815 ) ) ;
#40512=CARTESIAN_POINT ( 'NONE',  ( 4.073291749555208341, 117.6466181296975151, -0.7504383534773489961 ) ) ;
#40513=CARTESIAN_POINT ( 'NONE',  ( -1.505490909297014790, 33.15442552098056694, 4.097489486992727414 ) ) ;
#40515=CARTESIAN_POINT ( 'NONE',  ( -0.7499141588179909501, 115.7030497829226903, 1.729243208713743041 ) ) ;
#40516=ORIENTED_EDGE ( 'NONE', *, *, #38287, .T. ) ;
#40517=CARTESIAN_POINT ( 'NONE',  ( -2.893454522978812893, 104.6144662015457243, -3.863863340516500600 ) ) ;
#40518=CARTESIAN_POINT ( 'NONE',  ( 3.501109451447479870, -15.63356008979879874, 3.898959153382382858 ) ) ;
#40519=CARTESIAN_POINT ( 'NONE',  ( -19.74506706576321236, 148.5147687316951135, 1.724011100433736177 ) ) ;
#40521=CARTESIAN_POINT ( 'NONE',  ( -0.5455758836206960893, 21.45819190514113117, -0.8097498057291211415 ) ) ;
#40523=ORIENTED_EDGE ( 'NONE', *, *, #31332, .F. ) ;
#40525=CARTESIAN_POINT ( 'NONE',  ( 2.282361306983733407, 118.7862729053988318, 0.7764855222020032866 ) ) ;
#40526=CARTESIAN_POINT ( 'NONE',  ( -15.62653493684497796, 149.1167355181319181, 1.114087811593069910 ) ) ;
#40527=CARTESIAN_POINT ( 'NONE',  ( -6.474089935681887051E-14, 69.94346620154573202, 3.752704589293910110E-29 ) ) ;
#40528=CARTESIAN_POINT ( 'NONE',  ( 4.574931840464235400, 118.0742404603594053, -0.6030673501148580140 ) ) ;
#40529=CARTESIAN_POINT ( 'NONE',  ( 3.413396786258054316, 119.6896249646678569, -0.6770706109030819597 ) ) ;
#40530=CARTESIAN_POINT ( 'NONE',  ( -13.02489573621956076, 155.4510764517707742, -2.156236249524808635 ) ) ;
#40531=CARTESIAN_POINT ( 'NONE',  ( -5.008987216574991130, 117.3966124399498199, 0.7756614662348499944 ) ) ;
#40532=CARTESIAN_POINT ( 'NONE',  ( 4.318480543059425969, 118.2119050262681981, -0.3228229928774009605 ) ) ;
#40533=CARTESIAN_POINT ( 'NONE',  ( 9.417214020844189903, 124.0858766813489780, -0.2349654282845519138 ) ) ;
#40535=CARTESIAN_POINT ( 'NONE',  ( 2.770264620702337588, -13.86593384134129892, 0.2159450460461957433 ) ) ;
#40536=CARTESIAN_POINT ( 'NONE',  ( -4.958806897238241085, 117.4102282907815606, 0.9054230299057887121 ) ) ;
#40539=CARTESIAN_POINT ( 'NONE',  ( -0.09930934064637705894, -13.04092083763876175, -4.623607705436294957 ) ) ;
#40540=CARTESIAN_POINT ( 'NONE',  ( 4.351716102370827066, 120.3584862571861436, 0.7474562918332060546 ) ) ;
#40541=CARTESIAN_POINT ( 'NONE',  ( -3.748619050207897985, 28.91994025391836942, 2.520532616727765518 ) ) ;
#40542=CARTESIAN_POINT ( 'NONE',  ( -0.1065646865916159702, 105.8844662015456777, 5.332932678536312032 ) ) ;
#40543=CARTESIAN_POINT ( 'NONE',  ( -3.812863311134618183, 2.017465188139291765, -2.614655560905410958 ) ) ;
#40544=CARTESIAN_POINT ( 'NONE',  ( 11.06205061746896234, 128.0319838675845290, 0.2615737156286701004 ) ) ;
#40547=CARTESIAN_POINT ( 'NONE',  ( -8.790893838487704670, 117.7047839374624516, -0.3241293065953896879 ) ) ;
#40550=CARTESIAN_POINT ( 'NONE',  ( -1.506244733641594280, 106.1067062490223947, 5.119529036520902743 ) ) ;
#40552=CARTESIAN_POINT ( 'NONE',  ( -5.746845633966660039, 1.589972373264088246, -6.161128625535090109 ) ) ;
#40555=CARTESIAN_POINT ( 'NONE',  ( 1.852819980464847305, -15.24972552306870455, 5.408883774200016425 ) ) ;
#40556=CARTESIAN_POINT ( 'NONE',  ( 0.01046636458941188792, 120.7331730230139755, -0.5237796829256086140 ) ) ;
#40557=CARTESIAN_POINT ( 'NONE',  ( -15.85309526068962427, 121.4040080620525117, 0.2080479070310633782 ) ) ;
#40558=ORIENTED_EDGE ( 'NONE', *, *, #32619, .T. ) ;
#40563=CARTESIAN_POINT ( 'NONE',  ( -6.439798515484507670E-14, 156.3034662015457172, 9.575285601066443938E-17 ) ) ;
#40564=CARTESIAN_POINT ( 'NONE',  ( 3.432440172432007053, -15.40242305089609154, 5.447709670318832131 ) ) ;
#40565=CARTESIAN_POINT ( 'NONE',  ( -1.161715739485909671, 117.9723128000925669, 0.5854012653586094794 ) ) ;
#40566=CARTESIAN_POINT ( 'NONE',  ( 6.890728787288526114, 117.8105958006179890, -0.6119090536800845248 ) ) ;
#40567=CARTESIAN_POINT ( 'NONE',  ( -1.178223178616622402, 14.53665720681882689, 4.476207649055042204 ) ) ;
#40568=CARTESIAN_POINT ( 'NONE',  ( -13.37536684427251110, 156.9592627042916604, -0.5421920129525307219 ) ) ;
#40572=CARTESIAN_POINT ( 'NONE',  ( 2.183041108267496977, 116.1870934937200985, 0.05032534355729129799 ) ) ;
#40573=CARTESIAN_POINT ( 'NONE',  ( -17.81274246965193342, 147.0764175921665640, 1.531068679518140518 ) ) ;
#40575=CARTESIAN_POINT ( 'NONE',  ( 19.17469122182624375, 148.2829752965438956, -1.735408567215429132 ) ) ;
#40576=CARTESIAN_POINT ( 'NONE',  ( -3.058686590880046907, 117.8293475852256904, -0.7841115193421154261 ) ) ;
#40578=CARTESIAN_POINT ( 'NONE',  ( 16.33963436279736214, 146.4745453488731357, -0.7896242330311487034 ) ) ;
#40580=CARTESIAN_POINT ( 'NONE',  ( -18.09674421129296817, 146.7121067869193496, -2.346545542165937803 ) ) ;
#40581=CARTESIAN_POINT ( 'NONE',  ( 3.501109451447479870, -15.63356008979879874, 3.898959153382382858 ) ) ;
#40582=CARTESIAN_POINT ( 'NONE',  ( -4.512835031468954483, 118.1143071752745612, -0.7003032011746382901 ) ) ;
#40584=CARTESIAN_POINT ( 'NONE',  ( -4.908928425608774404, 117.5479188556219441, 0.9160482988203918486 ) ) ;
#40585=CARTESIAN_POINT ( 'NONE',  ( 8.234130529647114116, 121.1361926620737393, 1.330377128061140057 ) ) ;
#40586=CARTESIAN_POINT ( 'NONE',  ( 2.744962145539584952, 116.5337465564440578, 0.01469834071105289089 ) ) ;
#40588=CARTESIAN_POINT ( 'NONE',  ( 8.218723488459346527, -2.309819447571417772, 1.932697321913255717 ) ) ;
#40589=CARTESIAN_POINT ( 'NONE',  ( 4.529648377620876687, 121.1059516323014549, 0.2990124396216896074 ) ) ;
#40593=FACE_OUTER_BOUND ( 'NONE', #20792, .T. ) ;
#40594=CARTESIAN_POINT ( 'NONE',  ( -5.332935397695332647, 62.83146620154573014, -0.1065647409268298401 ) ) ;
#40596=CARTESIAN_POINT ( 'NONE',  ( -23.34248308131520488, 149.0646716566344026, -0.3893018266236027980 ) ) ;
#40599=CARTESIAN_POINT ( 'NONE',  ( -5.858775649260424601, 121.3022210319751082, -0.4117851423131264066 ) ) ;
#40600=CARTESIAN_POINT ( 'NONE',  ( -8.413874481325345656, 119.6811429777991265, 1.089663159344654630 ) ) ;
#40602=CARTESIAN_POINT ( 'NONE',  ( 0.6390139148044564621, 115.7029491485453576, -1.736660153015813890 ) ) ;
#40603=CARTESIAN_POINT ( 'NONE',  ( -1.583718294068570343, 120.9073379818811134, -0.1636693232558001920 ) ) ;
#40604=CARTESIAN_POINT ( 'NONE',  ( 2.226119369219526689, -15.10343733042141068, 5.886803469647748699 ) ) ;
#40605=CARTESIAN_POINT ( 'NONE',  ( -15.81089186882093856, 155.0373533369262589, 1.166412807380551531 ) ) ;
#40608=CARTESIAN_POINT ( 'NONE',  ( 22.52498503541040975, 150.7873321363286152, 0.6028683204863922729 ) ) ;
#40609=CARTESIAN_POINT ( 'NONE',  ( 15.78228220284642269, 146.2362006864767636, 0.3825322408708758948 ) ) ;
#40610=DIRECTION ( 'NONE',  ( 0.9998004120163610509, 4.016384292689131511E-17, 0.01997839162482749689 ) ) ;
#40611=CARTESIAN_POINT ( 'NONE',  ( -0.4908008364610317309, 30.95719094559541418, -0.8433761395939078920 ) ) ;
#40612=CARTESIAN_POINT ( 'NONE',  ( -13.43562511198114784, 156.9186530619738562, -0.2898375456858039434 ) ) ;
#40617=CARTESIAN_POINT ( 'NONE',  ( -6.275263529460059608, 119.2322458688779250, 1.005175755799972315 ) ) ;
#40618=CARTESIAN_POINT ( 'NONE',  ( -3.538659794179211726, -11.74154716455626257, -2.972011832598964176 ) ) ;
#40619=CARTESIAN_POINT ( 'NONE',  ( 18.27285712481717539, 128.6097515361309149, 1.839992588890194458 ) ) ;
#40622=CARTESIAN_POINT ( 'NONE',  ( 20.46161261025634204, 147.6366098820875266, -1.667455336067830585 ) ) ;
#40623=CARTESIAN_POINT ( 'NONE',  ( -1.191460153279743750, 25.61543958765020434, -8.344265960924422743 ) ) ;
#40624=CARTESIAN_POINT ( 'NONE',  ( -5.450899203174041752, 159.0107326448372191, -0.9576670044529981274 ) ) ;
#40625=CARTESIAN_POINT ( 'NONE',  ( 4.969807616941213091, 117.5383056595475466, -0.8108227939444502264 ) ) ;
#40628=CARTESIAN_POINT ( 'NONE',  ( -10.40586874195283151, 126.0814211662656419, 0.04952998093763452681 ) ) ;
#40629=CARTESIAN_POINT ( 'NONE',  ( 4.513795256570364067, -15.26848473984131260, 4.551867270201407578 ) ) ;
#40630=CARTESIAN_POINT ( 'NONE',  ( -6.345283257703988156, 28.99440867395404453, 0.1037513055964221220 ) ) ;
#40631=CARTESIAN_POINT ( 'NONE',  ( -6.640726327341849406E-14, 100.6774662015457409, -1.320564745697255449E-18 ) ) ;
#40633=CARTESIAN_POINT ( 'NONE',  ( 11.88178580215906344, 154.9039014673913073, 2.222676336029907773 ) ) ;
#40636=CARTESIAN_POINT ( 'NONE',  ( -0.3686011943524581391, 118.1627388489639827, -0.9054303920307451570 ) ) ;
#40638=CARTESIAN_POINT ( 'NONE',  ( -1.559908931542489885, 116.9323294830472122, 1.291681667928520794 ) ) ;
#40639=CARTESIAN_POINT ( 'NONE',  ( 0.7792876995799051798, 11.14506788600763443, 8.385000233822015758 ) ) ;
#40640=CARTESIAN_POINT ( 'NONE',  ( -0.01341678693510457362, 156.4123495908283985, 0.6714308817992611367 ) ) ;
#40641=CARTESIAN_POINT ( 'NONE',  ( -4.727076074248890869, 118.5930653697794384, -1.020453353391729712 ) ) ;
#40642=CARTESIAN_POINT ( 'NONE',  ( 23.05883864707322672, 142.5499849734818838, -0.2756568390806648505 ) ) ;
#40643=LINE ( 'NONE', #4032, #36962 ) ;
#40647=DIRECTION ( 'NONE',  ( 0.01997839162482749689, 1.040247600000945640E-18, -0.9998004120163610509 ) ) ;
#40648=CARTESIAN_POINT ( 'NONE',  ( -4.245060323073253983, 118.2245461714415882, 0.3158324249594203215 ) ) ;
#40649=CARTESIAN_POINT ( 'NONE',  ( 3.009276887026298031, 39.20946620154573736, -1.210121013456480599 ) ) ;
#40651=ORIENTED_EDGE ( 'NONE', *, *, #11284, .T. ) ;
#40653=CARTESIAN_POINT ( 'NONE',  ( 4.064929033868455832, 119.1709280882609647, -0.7633918317421104494 ) ) ;
#40654=CARTESIAN_POINT ( 'NONE',  ( -6.733859895264124873, 121.2177056076135528, -0.3428974583126987996 ) ) ;
#40655=CARTESIAN_POINT ( 'NONE',  ( 4.384565885174443345, 118.1629857386982252, 0.6642191121717796465 ) ) ;
#40656=CARTESIAN_POINT ( 'NONE',  ( -0.6075365842366953206, 120.7136710450757988, -0.2388278564565361750 ) ) ;
#40658=CARTESIAN_POINT ( 'NONE',  ( 0.1174553389596492831, 118.1651004037305057, -0.8901345560001526769 ) ) ;
#40660=CARTESIAN_POINT ( 'NONE',  ( 3.935102970030661673, 16.48578375386999539, 2.424025302511324309 ) ) ;
#40661=CARTESIAN_POINT ( 'NONE',  ( -16.15947664645545245, 148.3349945484709451, -1.756847814979443534 ) ) ;
#40666=CARTESIAN_POINT ( 'NONE',  ( 7.787415783305453587, 122.6040299132955766, 0.2655587982165120153 ) ) ;
#40668=CARTESIAN_POINT ( 'NONE',  ( 22.65971377182555457, 149.0844379882532849, 1.633711759839209465 ) ) ;
#40670=CARTESIAN_POINT ( 'NONE',  ( 3.198224922426783579, -14.19254063666773291, 2.189163805996276579 ) ) ;
#40671=CARTESIAN_POINT ( 'NONE',  ( 13.92608219098127442, 121.7708260186165177, -1.076920499313079649 ) ) ;
#40672=CARTESIAN_POINT ( 'NONE',  ( -14.49813937024316779, 152.7616507467334372, 1.711219460879524146 ) ) ;
#40673=CARTESIAN_POINT ( 'NONE',  ( -4.596079559025361583, 18.26954911218466648, 0.4757704999388879807 ) ) ;
#40674=CARTESIAN_POINT ( 'NONE',  ( -7.852582050918316625, 158.6543443936584481, -0.7853876145049528690 ) ) ;
#40676=CARTESIAN_POINT ( 'NONE',  ( 0.6142125404598580696, 23.44653936994281906, -0.7587870835084352672 ) ) ;
#40679=CARTESIAN_POINT ( 'NONE',  ( -10.74829939017208424, 126.1521286088116369, 0.3663887985317103024 ) ) ;
#40680=CARTESIAN_POINT ( 'NONE',  ( 4.362034286260056071, -13.41731938665795276, 3.520857194803681534 ) ) ;
#40681=CARTESIAN_POINT ( 'NONE',  ( 16.92314199871282909, 144.1809451582817587, -1.383154804529856730 ) ) ;
#40682=ORIENTED_EDGE ( 'NONE', *, *, #18885, .T. ) ;
#40683=CARTESIAN_POINT ( 'NONE',  ( 3.087900938566228604, 115.7029548885307690, 1.663163182406099949 ) ) ;
#40685=CARTESIAN_POINT ( 'NONE',  ( 3.001448597307602828, -14.49079452896849496, 4.301892286087903194 ) ) ;
#40686=CARTESIAN_POINT ( 'NONE',  ( -4.869070970386411012, 117.7192101133515081, -0.9437256607972734912 ) ) ;
#40687=EDGE_CURVE ( 'NONE', #32704, #35171, #7314, .T. ) ;
#40688=CARTESIAN_POINT ( 'NONE',  ( 13.59948517815232982, 150.2262467139961473, 0.1464537565166199873 ) ) ;
#40690=CARTESIAN_POINT ( 'NONE',  ( 19.08488522674161558, 150.4642993720107143, 2.434974558521498356 ) ) ;
#40692=CARTESIAN_POINT ( 'NONE',  ( -5.351939987885121930, 28.02203698121795128, 0.4484657473410642026 ) ) ;
#40694=CARTESIAN_POINT ( 'NONE',  ( 3.754954749907335465, 116.6824454826851820, -0.08209545411912760882 ) ) ;
#40697=CARTESIAN_POINT ( 'NONE',  ( 1.943636354525413168, -15.05866079806446400, 5.749033333573775550 ) ) ;
#40699=CARTESIAN_POINT ( 'NONE',  ( -4.999442924991678083, 117.3993846698902672, -0.8265828626092326381 ) ) ;
#40700=CARTESIAN_POINT ( 'NONE',  ( -4.675172209724520300, 117.9626846738122623, 0.7309470385922346436 ) ) ;
#40703=CARTESIAN_POINT ( 'NONE',  ( -8.451782431670267215, 119.2584666972338283, -1.350551005905172408 ) ) ;
#40704=CARTESIAN_POINT ( 'NONE',  ( 0.1065646865915094443, 105.8844662015457061, -5.332932678536314697 ) ) ;
#40705=CARTESIAN_POINT ( 'NONE',  ( 4.902823790339319032, 117.6536153060737320, 0.9411696025594519233 ) ) ;
#40707=CARTESIAN_POINT ( 'NONE',  ( -0.3785707606483163512, 120.7331730230137623, 0.5164240810526173897 ) ) ;
#40708=CARTESIAN_POINT ( 'NONE',  ( -2.136650056307613621, 10.86338872207680950, -4.114640003288728920 ) ) ;
#40710=CARTESIAN_POINT ( 'NONE',  ( -5.158148607181098022, 114.7154334724729097, -1.455730150661056044 ) ) ;
#40711=CARTESIAN_POINT ( 'NONE',  ( 2.626143189074743756, -14.75305764222682647, 4.894789397842846945 ) ) ;
#40712=CARTESIAN_POINT ( 'NONE',  ( 4.812498123319315368, 116.8297769931967309, -0.8564213435964298515 ) ) ;
#40714=CARTESIAN_POINT ( 'NONE',  ( -5.034401795890290465, 27.85181560600499395, 0.5116811242461191123 ) ) ;
#40715=B_SPLINE_CURVE_WITH_KNOTS ( 'NONE', 5,
 ( #15851, #17067, #36470, #6863, #28645, #26874 ),
 .UNSPECIFIED., .F., .F.,
 ( 6, 6 ),
 ( 0.7824693819017078944, 1.000000000000000000 ),
 .UNSPECIFIED. ) ;
#40716=CARTESIAN_POINT ( 'NONE',  ( -0.2391844021489926142, 115.7030485465296579, 1.756103904555268214 ) ) ;
#40717=CARTESIAN_POINT ( 'NONE',  ( -4.460028654926622593, 22.53297844546955631, 1.214995109042491528 ) ) ;
#40719=CARTESIAN_POINT ( 'NONE',  ( -3.857417139088993530, 104.6144662015498881, -3.700432031744215866 ) ) ;
#40720=CARTESIAN_POINT ( 'NONE',  ( 1.896617635523351053, -15.61750365820154052, 5.464805439086081407 ) ) ;
#40721=CARTESIAN_POINT ( 'NONE',  ( -11.29660330931812240, 121.3367100885591015, 1.243740200939189133 ) ) ;
#40722=CARTESIAN_POINT ( 'NONE',  ( 0.3817720443006957232, 19.93710050853265869, -0.8978640518339636722 ) ) ;
#40723=EDGE_LOOP ( 'NONE', ( #37763, #29975, #14269, #41352 ) ) ;
#40724=ORIENTED_EDGE ( 'NONE', *, *, #33879, .F. ) ;
#40726=CARTESIAN_POINT ( 'NONE',  ( 3.894863181655531026, 121.5791280715047122, 0.3237234463424497610 ) ) ;
#40727=CARTESIAN_POINT ( 'NONE',  ( -4.430366727502396351, 120.6578283891288379, 0.4452475156743749274 ) ) ;
#40729=CARTESIAN_POINT ( 'NONE',  ( 4.605784392446712339, 118.0409339601070684, -0.6501282048334815489 ) ) ;
#40730=CARTESIAN_POINT ( 'NONE',  ( 6.628409759326957307, 120.2999964176511014, -0.9194780514890085188 ) ) ;
#40731=CARTESIAN_POINT ( 'NONE',  ( -20.38365538121576037, 147.8414448467482600, -2.482674703111230841 ) ) ;
#40733=CARTESIAN_POINT ( 'NONE',  ( 4.385175369536176149, 118.1846130434793736, -0.4263825146163124358 ) ) ;
#40734=CARTESIAN_POINT ( 'NONE',  ( 0.6772589037150074098, 156.3292479207028407, -0.3306685775513073522 ) ) ;
#40735=ORIENTED_EDGE ( 'NONE', *, *, #27165, .F. ) ;
#40736=CARTESIAN_POINT ( 'NONE',  ( 1.852819980464847305, -15.24972552306870455, 5.408883774200016425 ) ) ;
#40741=ADVANCED_FACE ( 'NONE', ( #7148 ), #12042, .F. ) ;
#40743=CARTESIAN_POINT ( 'NONE',  ( -4.120466288800530563, -1.808681497221679590, -2.133573495687988597 ) ) ;
#40744=CARTESIAN_POINT ( 'NONE',  ( 16.71293428529030578, 146.3384789841921361, 1.780605135160314489 ) ) ;
#40745=CARTESIAN_POINT ( 'NONE',  ( -3.151460842193158474, 28.87231940813492770, 1.610289367860948229 ) ) ;
#40746=CARTESIAN_POINT ( 'NONE',  ( -2.741226102065176029, 109.4146836159258669, 3.767795064178312892 ) ) ;
#40747=CARTESIAN_POINT ( 'NONE',  ( -4.288638401707804526, -7.253218809911426312, -1.756103832032595680 ) ) ;
#40748=CARTESIAN_POINT ( 'NONE',  ( 7.557080711912756321, 122.4263405438208991, 0.1815966937148654481 ) ) ;
#40750=CARTESIAN_POINT ( 'NONE',  ( -2.668541714186689617, -2.899408749949365038, -8.001679540268986202 ) ) ;
#40752=CARTESIAN_POINT ( 'NONE',  ( 2.154724539067322642, 116.5279165083215531, -0.3115280795628784238 ) ) ;
#40754=CARTESIAN_POINT ( 'NONE',  ( 3.682264917456191888, 101.1854662015457365, 0.07358041635423968885 ) ) ;
#40755=CARTESIAN_POINT ( 'NONE',  ( -5.586884702347495235, 68.92746620154572668, -0.1116392523995361763 ) ) ;
#40757=CARTESIAN_POINT ( 'NONE',  ( -1.112825283668275045, 5.041181605477844663, 8.348645504544187190 ) ) ;
#40758=CARTESIAN_POINT ( 'NONE',  ( -0.01811622957310190032, 118.1588881536610529, 0.9066104818223087447 ) ) ;
#40760=CARTESIAN_POINT ( 'NONE',  ( 2.233078627056604759, -15.14192004606506536, 5.083345892419886880 ) ) ;
#40761=CARTESIAN_POINT ( 'NONE',  ( 0.4232488410868608941, 124.9344662015457317, 0.008457519121177021690 ) ) ;
#40762=CARTESIAN_POINT ( 'NONE',  ( -5.670663496354099387, 159.1134716836843381, 0.2862304005612826274 ) ) ;
#40768=CARTESIAN_POINT ( 'NONE',  ( -11.03183784343237583, 128.0124916018596650, -0.2204423744267034746 ) ) ;
#40769=CARTESIAN_POINT ( 'NONE',  ( 5.769960013412655186, -14.74427453315851899, 2.495425615322755419 ) ) ;
#40770=CARTESIAN_POINT ( 'NONE',  ( -11.79681931163876385, 156.4111399680655552, 1.533406117021610449 ) ) ;
#40771=CARTESIAN_POINT ( 'NONE',  ( 3.922549711534259576, 117.3164332630744298, -0.5226386447273274616 ) ) ;
#40772=CARTESIAN_POINT ( 'NONE',  ( 2.488009491785908800, 18.85968022696138391, -3.895047602898422223 ) ) ;
#40773=CARTESIAN_POINT ( 'NONE',  ( -11.56079167746340097, 118.7825156662901378, -0.6096482884850569217 ) ) ;
#40774=ADVANCED_FACE ( 'NONE', ( #16497 ), #36117, .T. ) ;
#40777=CARTESIAN_POINT ( 'NONE',  ( 5.558084639757285395, 116.7153428098866641, 0.2417474866754134033 ) ) ;
#40779=CARTESIAN_POINT ( 'NONE',  ( -17.71558884668074896, 147.6919162452172145, 1.529690151225475692 ) ) ;
#40781=CARTESIAN_POINT ( 'NONE',  ( 19.07204494652734184, 148.5750135429820205, -1.735237764431467822 ) ) ;
#40782=CARTESIAN_POINT ( 'NONE',  ( -13.88956208308366591, 122.0315337860429423, -1.683705570428295273 ) ) ;
#40784=CARTESIAN_POINT ( 'NONE',  ( 15.79191249938946839, 148.1776054874778197, -0.7900072561285058637 ) ) ;
#40786=CARTESIAN_POINT ( 'NONE',  ( -2.153957835384924469, 157.2504501563031738, -1.632675037709188315 ) ) ;
#40787=CARTESIAN_POINT ( 'NONE',  ( 4.539898764682361865, -15.38453816280940778, 0.3562021009913567959 ) ) ;
#40788=CARTESIAN_POINT ( 'NONE',  ( -4.528373626541791985, 118.0896223068915276, -0.7655945527491994085 ) ) ;
#40789=EDGE_CURVE ( 'NONE', #26194, #35651, #969, .T. ) ;
#40792=CARTESIAN_POINT ( 'NONE',  ( 1.354060893033489643, 119.5584937100158243, 0.6194060083641332870 ) ) ;
#40795=CARTESIAN_POINT ( 'NONE',  ( -7.401523468229766145, -5.981721843848114339, 4.095665678060115944 ) ) ;
#40796=CARTESIAN_POINT ( 'NONE',  ( 4.329655997251290245, 155.8404949922767742, 0.5159277680907120578 ) ) ;
#40800=CARTESIAN_POINT ( 'NONE',  ( 3.837460294590816279, 108.9298176806530165, -3.710659438875620886 ) ) ;
#40804=CARTESIAN_POINT ( 'NONE',  ( -16.19138771801004495, 121.3864332154274877, -0.1624333549846387614 ) ) ;
#40807=CARTESIAN_POINT ( 'NONE',  ( -5.910993448784967796, 121.3707704662934219, -0.3328318058967496551 ) ) ;
#40809=ORIENTED_EDGE ( 'NONE', *, *, #38613, .F. ) ;
#40810=CARTESIAN_POINT ( 'NONE',  ( 0.7079803121674352884, 118.7629491485454025, -1.246627914299262896 ) ) ;
#40811=CARTESIAN_POINT ( 'NONE',  ( -10.39558336183872989, 126.0814211662656419, -0.4651924986760611058 ) ) ;
#40812=CARTESIAN_POINT ( 'NONE',  ( 2.652408316642993480, -15.27006336626107696, 5.836003982494253783 ) ) ;
#40813=CARTESIAN_POINT ( 'NONE',  ( -3.977532531966777807, 117.6225627337916393, 0.6337845664926936573 ) ) ;
#40814=CARTESIAN_POINT ( 'NONE',  ( 0.2297947187657226054, 117.3993836757579317, -1.488868525946095422 ) ) ;
#40815=CARTESIAN_POINT ( 'NONE',  ( 16.18495160125058874, 121.3864332154274877, 0.4845229560194669327 ) ) ;
#40816=CARTESIAN_POINT ( 'NONE',  ( 8.946522384465550815, 123.9641338091273894, 0.2230221356586828685 ) ) ;
#40818=CARTESIAN_POINT ( 'NONE',  ( -0.2773724154211913984, 24.90860930217742464, 0.9350043038818249830 ) ) ;
#40819=CARTESIAN_POINT ( 'NONE',  ( -11.70340384973345849, 118.7242475115495495, -0.3301557443347882259 ) ) ;
#40822=ORIENTED_EDGE ( 'NONE', *, *, #34765, .T. ) ;
#40825=CARTESIAN_POINT ( 'NONE',  ( -8.365703719145541228, 119.9183728994499916, 1.113763724379078557 ) ) ;
#40826=CARTESIAN_POINT ( 'NONE',  ( 1.173990663012069113, -13.46572784750561880, -4.469126434461346165 ) ) ;
#40827=CARTESIAN_POINT ( 'NONE',  ( 21.45663756426498381, 150.2128557559047692, 2.007674378541679072 ) ) ;
#40829=CARTESIAN_POINT ( 'NONE',  ( 8.970048054448124475, 157.0267672960688969, -1.675204009492540447 ) ) ;
#40830=CARTESIAN_POINT ( 'NONE',  ( 0.04286443493920111952, 25.39157861068392208, -8.424000189867014043 ) ) ;
#40831=CARTESIAN_POINT ( 'NONE',  ( -16.14352587498456160, 122.8183540351560907, -1.297681478882586115 ) ) ;
#40832=CARTESIAN_POINT ( 'NONE',  ( 4.757004511144192094, 117.7257274568053873, -0.9115379262560657780 ) ) ;
#40833=EDGE_LOOP ( 'NONE', ( #30791, #7937, #16950, #16124 ) ) ;
#40834=CARTESIAN_POINT ( 'NONE',  ( -15.81463230642823170, 145.9351319680867221, 0.01551611691150908343 ) ) ;
#40835=CARTESIAN_POINT ( 'NONE',  ( -0.4661379286531509014, 118.8635629087341954, -0.6143748731645414241 ) ) ;
#40836=CARTESIAN_POINT ( 'NONE',  ( 4.192023472006414231, -15.34368243816432198, 4.862536176465709126 ) ) ;
#40838=CARTESIAN_POINT ( 'NONE',  ( -2.751821739654949805, 117.9496046090067125, -1.327625076587163111 ) ) ;
#40839=ORIENTED_EDGE ( 'NONE', *, *, #24307, .T. ) ;
#40841=CARTESIAN_POINT ( 'NONE',  ( 1.279006062069942384, 119.0230276286704054, 0.6822954352362461394 ) ) ;
#40844=CARTESIAN_POINT ( 'NONE',  ( -5.239701418611195649, 115.6909491485453003, -1.023982712389427840 ) ) ;
#40845=CARTESIAN_POINT ( 'NONE',  ( -2.908797093395109723, 122.3314979878274045, 0.1372540494999659189 ) ) ;
#40846=CARTESIAN_POINT ( 'NONE',  ( -2.668541714186689617, -2.899408749949365038, -8.001679540268986202 ) ) ;
#40847=CARTESIAN_POINT ( 'NONE',  ( 16.13275712328120548, 147.4171829256358137, 1.433441054525536273 ) ) ;
#40849=CARTESIAN_POINT ( 'NONE',  ( 22.91546036685015153, 149.1739538623130272, -0.5130544771887697308 ) ) ;
#40852=CARTESIAN_POINT ( 'NONE',  ( -4.528182882554109945, 31.49130102246704155, -0.6941393877658236233 ) ) ;
#40853=CARTESIAN_POINT ( 'NONE',  ( 1.897380780832737202, -15.05783359004130517, 5.662421594695138616 ) ) ;
#40854=CARTESIAN_POINT ( 'NONE',  ( -4.282516613351655010, 118.2128436458740168, 0.3623403077545777617 ) ) ;
#40858=( BOUNDED_CURVE ( )  B_SPLINE_CURVE ( 3, ( #24335, #24757, #31579, #2205 ),
 .UNSPECIFIED., .F., .T. ) 
 B_SPLINE_CURVE_WITH_KNOTS ( ( 4, 4 ),
 ( 0.000000000000000000, 1.570796326794895670 ),
 .UNSPECIFIED. ) 
 CURVE ( )  GEOMETRIC_REPRESENTATION_ITEM ( )  RATIONAL_B_SPLINE_CURVE ( ( 1.000000000000000000, 0.8047378541243652705, 0.8047378541243652705, 1.000000000000000000 ) ) 
 REPRESENTATION_ITEM ( '' )  );
#40859=CARTESIAN_POINT ( 'NONE',  ( -4.024596240589787044, 119.1709112288356494, -0.9240400258402845513 ) ) ;
#40860=CARTESIAN_POINT ( 'NONE',  ( -5.332935397695336199, 116.0444662015457311, -0.1065647409268299234 ) ) ;
#40861=CARTESIAN_POINT ( 'NONE',  ( 4.394896113366216994, 118.1799268271195160, 0.5694229943158597429 ) ) ;
#40862=CARTESIAN_POINT ( 'NONE',  ( -16.02106284285062898, 145.8417561620165372, -1.176135107295964932 ) ) ;
#40864=AXIS2_PLACEMENT_3D ( 'NONE', #21150, #34180, #24563 ) ;
#40865=CARTESIAN_POINT ( 'NONE',  ( 0.8838529761740171464, 116.4325158421065680, 0.01766148591713737059 ) ) ;
#40866=ORIENTED_EDGE ( 'NONE', *, *, #15701, .T. ) ;
#40867=CARTESIAN_POINT ( 'NONE',  ( -4.631227783250409402, 22.10816835407601744, -0.05711764529929251599 ) ) ;
#40868=CARTESIAN_POINT ( 'NONE',  ( -6.788801044988821864, 155.5980657034081105, -1.487835262196283814 ) ) ;
#40872=CARTESIAN_POINT ( 'NONE',  ( 6.991496846172011281, 121.9383932547358427, 0.2731297716818573140 ) ) ;
#40873=CARTESIAN_POINT ( 'NONE',  ( -4.621022795674669226, 27.76579825817536218, 0.1735962381356405959 ) ) ;
#40874=CARTESIAN_POINT ( 'NONE',  ( 22.49588706318638387, 149.6594668941642681, 1.627141970658571912 ) ) ;
#40876=CARTESIAN_POINT ( 'NONE',  ( 2.857130780617909149, -14.87311083204414786, 4.269097905712053276 ) ) ;
#40877=CARTESIAN_POINT ( 'NONE',  ( 20.03018601867063708, 150.7967616730061593, -1.468133569223299739 ) ) ;
#40878=AXIS2_PLACEMENT_3D ( 'NONE', #12797, #42001, #36025 ) ;
#40879=CARTESIAN_POINT ( 'NONE',  ( -5.764372972839621134, 156.8407539676644546, 1.669942767410474094 ) ) ;
#40880=CARTESIAN_POINT ( 'NONE',  ( -4.583145339711863109, 27.87760190725156662, 0.5120832130453706332 ) ) ;
#40881=CARTESIAN_POINT ( 'NONE',  ( -22.80460045200421959, 149.7823008822066697, -1.306974408439632196 ) ) ;
#40882=CARTESIAN_POINT ( 'NONE',  ( 0.6656887758738300187, 13.74536131906779879, -0.7131539583378491143 ) ) ;
#40883=VERTEX_POINT ( 'NONE', #343 ) ;
#40885=CARTESIAN_POINT ( 'NONE',  ( -7.108627447324336934, 121.8675249661327626, 0.3373703349335459567 ) ) ;
#40886=CARTESIAN_POINT ( 'NONE',  ( 4.090168366125579880, -14.63905918998462141, 5.005671547667302157 ) ) ;
#40887=CARTESIAN_POINT ( 'NONE',  ( 17.30282355392125027, 146.5563353440282981, -1.366477706345457843 ) ) ;
#40889=CARTESIAN_POINT ( 'NONE',  ( 2.393094646133926862, 115.7029491485453434, 1.700721971483515560 ) ) ;
#40890=CARTESIAN_POINT ( 'NONE',  ( 2.744913772555794385, -12.89811552070117884, 0.2544447123532062038 ) ) ;
#40891=CARTESIAN_POINT ( 'NONE',  ( -4.717230826267398314, 117.7257772426691105, -1.100749342947852538 ) ) ;
#40892=CARTESIAN_POINT ( 'NONE',  ( 15.53315888837586201, 147.5314071815517138, 0.1823436108899492425 ) ) ;
#40894=CARTESIAN_POINT ( 'NONE',  ( 14.32444608545400300, 154.4775811199918110, 2.255247442408088165 ) ) ;
#40897=CARTESIAN_POINT ( 'NONE',  ( 0.008148259816488066104, 159.5682499516715040, -0.4077722408685185429 ) ) ;
#40898=CARTESIAN_POINT ( 'NONE',  ( 11.62351318166542669, 118.7506923092098674, -0.05658863777226865593 ) ) ;
#40901=CARTESIAN_POINT ( 'NONE',  ( 1.804633460655494570, -15.08373741368226817, 5.749549428864549228 ) ) ;
#40904=CARTESIAN_POINT ( 'NONE',  ( -4.809624879280043785, 117.8762316427875163, 0.6704367731218271453 ) ) ;
#40908=CARTESIAN_POINT ( 'NONE',  ( 5.750380026109916720, 118.5999988179069362, -0.9867663322649924407 ) ) ;
#40909=CARTESIAN_POINT ( 'NONE',  ( -2.972890788444433330, 110.6400929099055332, -3.409217096083849263 ) ) ;
#40910=CARTESIAN_POINT ( 'NONE',  ( 4.959929520007769987, 117.4682222762912573, 0.9863292331654268663 ) ) ;
#40911=DIRECTION ( 'NONE',  ( -4.017660918040594346E-17, 1.000000000000000000, 2.376309959284834438E-19 ) ) ;
#40912=CARTESIAN_POINT ( 'NONE',  ( -0.3886773557329153972, 118.1497763966932695, 1.061209395727771732 ) ) ;
#40913=CARTESIAN_POINT ( 'NONE',  ( 1.104432469574216480, -9.427232690354344413, -4.492858291722996888 ) ) ;
#40915=CARTESIAN_POINT ( 'NONE',  ( -6.550797450135577910E-14, 84.67546620154573134, 2.164564701558966795E-29 ) ) ;
#40916=CARTESIAN_POINT ( 'NONE',  ( 3.507226199677831779, -13.17319675123219902, 2.199731216082013940 ) ) ;
#40917=CARTESIAN_POINT ( 'NONE',  ( 5.114723271350645639, 118.2545999410811106, -0.5144770513779389765 ) ) ;
#40918=CARTESIAN_POINT ( 'NONE',  ( -7.784012322544769269, 122.6313477034873074, -0.1555430911242075831 ) ) ;
#40919=CARTESIAN_POINT ( 'NONE',  ( 1.400765281975942855, 35.96429942923645484, 2.374657561808434458 ) ) ;
#40920=CARTESIAN_POINT ( 'NONE',  ( -0.5330231537557663657, 115.7033788390540963, 1.742913876867271838 ) ) ;
#40921=CARTESIAN_POINT ( 'NONE',  ( -3.789191232057584902, 13.46218022696137773, 2.646434746401360893 ) ) ;
#40923=CARTESIAN_POINT ( 'NONE',  ( 2.417140579268110656, 105.1243918821411825, -4.755895391891847623 ) ) ;
#40924=CARTESIAN_POINT ( 'NONE',  ( 4.529877808639974468, -15.43662617131508163, 0.9000745948097405025 ) ) ;
#40925=CARTESIAN_POINT ( 'NONE',  ( -19.34566907036586159, 149.3473233412102275, 1.724881794388704925 ) ) ;
#40926=CARTESIAN_POINT ( 'NONE',  ( 0.7990752137124343957, 23.01725015362593396, -0.5559626729366093922 ) ) ;
#40928=CARTESIAN_POINT ( 'NONE',  ( -0.9549105556349912760, 13.03813504644791976, -0.2014467441264284064 ) ) ;
#40929=ORIENTED_EDGE ( 'NONE', *, *, #9182, .F. ) ;
#40932=CARTESIAN_POINT ( 'NONE',  ( 1.618304973946058878, 119.5945091202099348, 0.6420790694971424406 ) ) ;
#40934=CARTESIAN_POINT ( 'NONE',  ( -16.60605961460005275, 147.5857818452174115, 1.108006280952565037 ) ) ;
#40936=CARTESIAN_POINT ( 'NONE',  ( 3.383663933261424006, -14.10150345098371005, 4.318103191797684204 ) ) ;
#40937=CARTESIAN_POINT ( 'NONE',  ( 9.808453647369967499, 155.3230018269108825, -1.667681936676747689 ) ) ;
#40938=CIRCLE ( 'NONE', #25929, 5.588000000000006295 ) ;
#40939=CARTESIAN_POINT ( 'NONE',  ( -19.42875987905505042, 141.0981142166620259, -2.503406319619450038 ) ) ;
#40941=EDGE_CURVE ( 'NONE', #10310, #1232, #39247, .T. ) ;
#40942=CARTESIAN_POINT ( 'NONE',  ( 4.074910602682932925, 118.2429491485453354, -0.1454311599470142491 ) ) ;
#40943=CARTESIAN_POINT ( 'NONE',  ( 1.630522158633523011, 156.2764358050213787, -0.3353572448990092547 ) ) ;
#40944=VERTEX_POINT ( 'NONE', #10112 ) ;
#40945=CARTESIAN_POINT ( 'NONE',  ( 3.162130362391316840, -14.71481139081727640, 3.323541290955854599 ) ) ;
#40947=CARTESIAN_POINT ( 'NONE',  ( -0.9149567752697743694, 32.47697140010484418, 3.785418454572508473 ) ) ;
#40950=CARTESIAN_POINT ( 'NONE',  ( -3.769861741716944881, -2.021032284792064093, -2.673854242032364326 ) ) ;
#40951=CARTESIAN_POINT ( 'NONE',  ( 5.138962689587240007, 120.6777149489875569, 0.7548553450424397848 ) ) ;
#40952=CARTESIAN_POINT ( 'NONE',  ( 2.962760531859824464, 39.20946620154573026, 1.117747612521613254 ) ) ;
#40953=CARTESIAN_POINT ( 'NONE',  ( -3.089687104934498940, 107.8271213589905386, 4.353618003723240371 ) ) ;
#40954=TOROIDAL_SURFACE ( 'NONE', #25941, 3.683000000000000718, 0.5080000000000000071 ) ;
#40955=CARTESIAN_POINT ( 'NONE',  ( -4.274281473441157608, 3.541781053574249327, 1.790774723582081451 ) ) ;
#40956=CARTESIAN_POINT ( 'NONE',  ( -1.820350978615107751, 35.44831059284695129, 0.3018992756893351115 ) ) ;
#40957=CARTESIAN_POINT ( 'NONE',  ( 7.448509604456053701, -5.047432113992361025, -3.928768625439613693 ) ) ;
#40959=CARTESIAN_POINT ( 'NONE',  ( -5.520563110719297839, 116.8899318124889959, -0.5663404003195862124 ) ) ;
#40960=CARTESIAN_POINT ( 'NONE',  ( -0.3260985403866875632, 116.4813942609866899, -1.528836360202051381 ) ) ;
#40963=CARTESIAN_POINT ( 'NONE',  ( 8.369700380136936957, -11.69135346447765933, 0.7700151973242596037 ) ) ;
#40964=CARTESIAN_POINT ( 'NONE',  ( 0.1782134618826983208, 117.3993841988815205, 1.495935623649740309 ) ) ;
#40966=CARTESIAN_POINT ( 'NONE',  ( -6.439703808512989190E-14, 63.33946620154573282, 4.464395889055755859E-29 ) ) ;
#40967=EDGE_CURVE ( 'NONE', #22781, #12250, #29659, .T. ) ;
#40968=CARTESIAN_POINT ( 'NONE',  ( 0.1450076288960709392, 106.1446358501009826, -5.226538226828138178 ) ) ;
#40969=CARTESIAN_POINT ( 'NONE',  ( -22.71658102202245999, 150.3666470947781022, 0.1371106802449220952 ) ) ;
#40970=ORIENTED_EDGE ( 'NONE', *, *, #29229, .F. ) ;
#40976=CARTESIAN_POINT ( 'NONE',  ( -4.610571905486848365, 121.2017135396456098, -0.05649303170681751335 ) ) ;
#40977=CARTESIAN_POINT ( 'NONE',  ( 3.031078967112608158, -15.50598464685963584, 5.611516622434578494 ) ) ;
#40978=CARTESIAN_POINT ( 'NONE',  ( -20.82688902969348987, 148.9555414352193168, 1.562960617212841408 ) ) ;
#40980=CARTESIAN_POINT ( 'NONE',  ( 21.25505906629468100, 136.5942649496780632, -0.9712689567086302267 ) ) ;
#40981=CARTESIAN_POINT ( 'NONE',  ( -0.6244342276652131707, 19.93415720681881353, -4.586363120317934694 ) ) ;
#40982=CARTESIAN_POINT ( 'NONE',  ( -1.396185014843847272, 159.5914066142653098, -0.2870382629871535141 ) ) ;
#40985=CARTESIAN_POINT ( 'NONE',  ( -2.186569186605118009, 116.2037677190601386, -0.01283534594974703423 ) ) ;
#40986=CARTESIAN_POINT ( 'NONE',  ( -4.329049305160163286, 120.0471566133196291, 0.6733469523851640659 ) ) ;
#40988=CARTESIAN_POINT ( 'NONE',  ( 6.185003182635295360, 157.2590385278250267, -1.713690555389224102 ) ) ;
#40989=CARTESIAN_POINT ( 'NONE',  ( -14.04349332752986257, 121.9525460547650226, -1.645664411013196382 ) ) ;
#40992=CARTESIAN_POINT ( 'NONE',  ( 6.511415066510850558, 121.4051597255373025, -0.4520850151541541684 ) ) ;
#40994=CARTESIAN_POINT ( 'NONE',  ( -3.724242145611234012, 156.8112981010400802, -1.651639321868204391 ) ) ;
#40995=CARTESIAN_POINT ( 'NONE',  ( 4.228667402019948618, -15.40433107038223426, 0.8683934293704824725 ) ) ;
#40996=CARTESIAN_POINT ( 'NONE',  ( -4.378978151537658903, 118.1614286189266778, -0.6690952136889736224 ) ) ;
#40999=DIRECTION ( 'NONE',  ( 0.01997839162482749689, 1.040247600000945640E-18, -0.9998004120163610509 ) ) ;
#41000=CARTESIAN_POINT ( 'NONE',  ( 13.78152227852067213, 152.5163154464351294, 2.142015651154440814 ) ) ;
#41001=DIRECTION ( 'NONE',  ( 0.9998004120163609398, 0.000000000000000000, 0.01997839162482749689 ) ) ;
#41002=CARTESIAN_POINT ( 'NONE',  ( -4.785772612713214080, 1.365856510964248649, -6.940074030798050408 ) ) ;
#41003=CARTESIAN_POINT ( 'NONE',  ( 6.012785076883544910, 155.3544091381320982, 0.3765917842305994134 ) ) ;
#41007=VERTEX_POINT ( 'NONE', #16356 ) ;
#41009=CARTESIAN_POINT ( 'NONE',  ( -7.788926316761409119, 122.5994947058344593, -0.3062370965690639490 ) ) ;
#41012=CARTESIAN_POINT ( 'NONE',  ( -18.71881220850887217, 125.2636347375217838, -0.1974931939226152733 ) ) ;
#41015=CARTESIAN_POINT ( 'NONE',  ( 6.916265728684992453, 121.8189303826054726, -0.2423212107496697243 ) ) ;
#41016=CARTESIAN_POINT ( 'NONE',  ( -7.882738460396780056, 122.2119657951150629, 0.4812898729222708227 ) ) ;
#41018=CARTESIAN_POINT ( 'NONE',  ( 0.3155153238127385018, 115.7029491485453150, -1.753375921699725115 ) ) ;
#41019=CARTESIAN_POINT ( 'NONE',  ( -11.24781102592754145, 128.1602342495223468, -0.5025223919565848796 ) ) ;
#41020=CARTESIAN_POINT ( 'NONE',  ( 5.396235140300779776, -11.83248475511457976, 0.6634469457710948648 ) ) ;
#41021=CARTESIAN_POINT ( 'NONE',  ( -10.89609060007118835, 119.5270080912504653, 0.8636533125102806574 ) ) ;
#41022=DIRECTION ( 'NONE',  ( 0.9998004120163609398, 0.000000000000000000, 0.01997839162482749689 ) ) ;
#41024=CARTESIAN_POINT ( 'NONE',  ( 23.42751387171875521, 146.8275480241000253, 0.6231101672962392479 ) ) ;
#41026=CARTESIAN_POINT ( 'NONE',  ( 4.609146067579531270, 121.2017137070652097, 0.1277310477265502786 ) ) ;
#41028=CARTESIAN_POINT ( 'NONE',  ( 0.7179688673824197176, 19.28876970375581479, -0.6613080194383522681 ) ) ;
#41029=CARTESIAN_POINT ( 'NONE',  ( -20.46883641438838453, 129.0748834149669904, -0.4693348210411829591 ) ) ;
#41033=CARTESIAN_POINT ( 'NONE',  ( 5.762928754573319878, 118.2277084192942738, 1.125902124160973905 ) ) ;
#41035=CARTESIAN_POINT ( 'NONE',  ( 22.07943683853326178, 148.3267584643486146, 2.032026126618132533 ) ) ;
#41037=CARTESIAN_POINT ( 'NONE',  ( 6.779039758441031793, 118.9580315507705706, -0.9776869392460786345 ) ) ;
#41038=CARTESIAN_POINT ( 'NONE',  ( 5.629075615873821548, 21.71503808657377022, 6.277010319805454763 ) ) ;
#41039=CARTESIAN_POINT ( 'NONE',  ( -21.87689675406264556, 150.0588410196355937, -1.874897916013938737 ) ) ;
#41040=CARTESIAN_POINT ( 'NONE',  ( 4.899310882224675368, 117.5479452163036171, -0.9252960604191319272 ) ) ;
#41041=CARTESIAN_POINT ( 'NONE',  ( 7.449435858333443683, 123.6645382909113664, 0.1834419053087676110 ) ) ;
#41043=CARTESIAN_POINT ( 'NONE',  ( -0.6527697516718347082, 156.3069099058775748, 0.1169209421757348294 ) ) ;
#41044=CARTESIAN_POINT ( 'NONE',  ( -18.66896445097611590, 144.8948545501563103, -2.490227693099508421 ) ) ;
#41045=CARTESIAN_POINT ( 'NONE',  ( 4.849545180983690251, -15.35966036743073637, 3.882997576023691444 ) ) ;
#41049=ORIENTED_EDGE ( 'NONE', *, *, #11000, .T. ) ;
#41050=CARTESIAN_POINT ( 'NONE',  ( 13.10180873912553068, 153.9517556018257096, 2.260155593826742582 ) ) ;
#41052=CARTESIAN_POINT ( 'NONE',  ( -4.611806494114576438, 117.9324678712513759, -0.9633187536371230486 ) ) ;
#41054=CARTESIAN_POINT ( 'NONE',  ( -1.490732016122501502, 115.2915405621345144, 1.797152713846303040 ) ) ;
#41055=CARTESIAN_POINT ( 'NONE',  ( 7.865828698536367902, -6.344330755464622662, 3.006797519310529854 ) ) ;
#41056=CARTESIAN_POINT ( 'NONE',  ( 9.347632431636288430, 123.5785764018267514, 0.8560492856234919179 ) ) ;
#41058=CARTESIAN_POINT ( 'NONE',  ( 20.86923087398506027, 132.2939277659177151, -0.4710007621541094647 ) ) ;
#41062=CARTESIAN_POINT ( 'NONE',  ( 1.848046085800037375, -15.12359198595263088, 5.521975501593074043 ) ) ;
#41063=CARTESIAN_POINT ( 'NONE',  ( -4.289101050795583348, 118.2138500885050689, 0.3554350998168962494 ) ) ;
#41064=CARTESIAN_POINT ( 'NONE',  ( -23.45208337669183152, 146.8499405026647651, -0.4686284387228153991 ) ) ;
#41068=CARTESIAN_POINT ( 'NONE',  ( 8.324009791931711533, 120.1221279132020783, -1.118190249840247397 ) ) ;
#41069=CARTESIAN_POINT ( 'NONE',  ( 5.336581877858352030, 116.0444662015457595, -0.07592003752709637621 ) ) ;
#41071=CARTESIAN_POINT ( 'NONE',  ( 4.398790584699274753, 118.1654141809896288, 0.6513841008152672085 ) ) ;
#41072=CARTESIAN_POINT ( 'NONE',  ( -9.518183030555464441, 123.9284174147966269, -0.7933090623874851088 ) ) ;
#41074=CARTESIAN_POINT ( 'NONE',  ( 15.73471677569731142, 120.8416612192341972, 0.3144170877231856065 ) ) ;
#41077=CARTESIAN_POINT ( 'NONE',  ( 4.622858883031034871, 26.85595184169372374, 0.2084198311932836112 ) ) ;
#41081=DIRECTION ( 'NONE',  ( -0.9998004120163608288, 0.000000000000000000, -0.01997839162482750383 ) ) ;
#41082=CARTESIAN_POINT ( 'NONE',  ( 6.083407471064808725, 121.3513819447846060, 0.4752266484690387260 ) ) ;
#41083=CARTESIAN_POINT ( 'NONE',  ( -4.487480840803009130, 27.34045677879159442, -1.100063755011520872 ) ) ;
#41084=CARTESIAN_POINT ( 'NONE',  ( 22.83601474261759989, 146.5373477140321938, 1.546791039490589492 ) ) ;
#41085=CARTESIAN_POINT ( 'NONE',  ( 0.2217520613055987411, 104.6144662015457101, -4.831251598276631753 ) ) ;
#41086=CARTESIAN_POINT ( 'NONE',  ( 2.849840736555561360, -14.15504780656048922, 0.1227973400909937313 ) ) ;
#41087=CARTESIAN_POINT ( 'NONE',  ( 20.77691070360829784, 149.9184980045912425, -1.462349339025473371 ) ) ;
#41088=CARTESIAN_POINT ( 'NONE',  ( -17.81946051592207070, 148.9562551477873740, 1.662425298156809506 ) ) ;
#41089=CARTESIAN_POINT ( 'NONE',  ( 0.3943543298815788134, 25.17882533764851871, -4.623353113333005915 ) ) ;
#41090=CARTESIAN_POINT ( 'NONE',  ( -14.80341400616319625, 120.8492938200443092, -1.052940121379140725 ) ) ;
#41092=CARTESIAN_POINT ( 'NONE',  ( -0.9708255322354510941, 17.08399857615920325, -0.1324238259073569901 ) ) ;
#41093=VERTEX_POINT ( 'NONE', #41394 ) ;
#41095=CARTESIAN_POINT ( 'NONE',  ( -7.650102001921326611, 122.3449549946481056, 0.2051776793030278268 ) ) ;
#41096=CARTESIAN_POINT ( 'NONE',  ( 4.521557965551993519, -14.38033123432501448, 4.565926699156682922 ) ) ;
#41097=CARTESIAN_POINT ( 'NONE',  ( 16.73823235880707472, 147.9788754379930822, -1.246688593732825590 ) ) ;
#41100=CARTESIAN_POINT ( 'NONE',  ( 0.7365107854829129330, 115.7029383640674212, 1.756173502283182364 ) ) ;
#41101=ORIENTED_EDGE ( 'NONE', *, *, #22719, .F. ) ;
#41102=CARTESIAN_POINT ( 'NONE',  ( -4.896113279795653916, 117.6590624440263468, -0.9620818870509636467 ) ) ;
#41103=CARTESIAN_POINT ( 'NONE',  ( 4.591655703643790609, 121.2030596905490540, 0.06445270968432179060 ) ) ;
#41105=CARTESIAN_POINT ( 'NONE',  ( 12.79701950029124902, 155.3440856034525837, 2.194532851538729457 ) ) ;
#41109=CARTESIAN_POINT ( 'NONE',  ( 0.02615207601215727498, 159.0391464308674756, -1.308756824028193044 ) ) ;
#41110=CARTESIAN_POINT ( 'NONE',  ( 5.816519783795321530, 117.0096406922080376, -0.1181936270109637949 ) ) ;
#41111=DIRECTION ( 'NONE',  ( 0.9998004120163608288, 4.016384292689131511E-17, 0.01997839162482749342 ) ) ;
#41112=CARTESIAN_POINT ( 'NONE',  ( 1.691696049192186857, -15.24586544832738610, 5.783975733521854679 ) ) ;
#41115=CARTESIAN_POINT ( 'NONE',  ( -4.729254454615190895, 117.9669711668249619, 0.6196972108808941337 ) ) ;
#41119=CARTESIAN_POINT ( 'NONE',  ( 3.245646068532854311, 118.3825688634768625, -0.7783404868572983970 ) ) ;
#41120=CARTESIAN_POINT ( 'NONE',  ( -3.333432127168630021, 112.1633951907056996, -2.855042910325920502 ) ) ;
#41121=CARTESIAN_POINT ( 'NONE',  ( 4.861520819079757416, 117.7423039542964318, 0.9146368285113327667 ) ) ;
#41122=CARTESIAN_POINT ( 'NONE',  ( -4.755622421505391273, 117.4716786420896284, -1.195466823065375994 ) ) ;
#41123=CARTESIAN_POINT ( 'NONE',  ( -0.06282972276048238991, 111.5577547982949227, 3.144256248693377387 ) ) ;
#41127=CARTESIAN_POINT ( 'NONE',  ( 3.247910276010201880, -14.18928037215049009, 3.960261243354706640 ) ) ;
#41128=CARTESIAN_POINT ( 'NONE',  ( 0.3401008104887150441, 105.9117620634264370, -5.317146732969808554 ) ) ;
#41129=CARTESIAN_POINT ( 'NONE',  ( -16.92358334414620913, 148.6336825499269310, -2.141768463193927552 ) ) ;
#41130=ADVANCED_FACE ( 'NONE', ( #35007 ), #5283, .T. ) ;
#41131=CARTESIAN_POINT ( 'NONE',  ( 5.135883789155748502, 116.9356663392523501, -0.1807461257199506066 ) ) ;
#41132=CARTESIAN_POINT ( 'NONE',  ( -3.299905295350023415, 32.79871628568109543, 4.342002458138856547 ) ) ;
#41133=CARTESIAN_POINT ( 'NONE',  ( -1.799679211148575542, 115.7029357389137090, 1.654552292944202030 ) ) ;
#41134=CARTESIAN_POINT ( 'NONE',  ( -1.576536484031922480, 10.66345178295009788, -4.350723848753511369 ) ) ;
#41135=CARTESIAN_POINT ( 'NONE',  ( 7.949750681159606813, 158.6775731370129279, 0.5882489250746236742 ) ) ;
#41137=CARTESIAN_POINT ( 'NONE',  ( -1.824400206236523658, 104.6144662015369278, -5.024575765548627615 ) ) ;
#41138=CARTESIAN_POINT ( 'NONE',  ( 4.210067206397440032, -15.44688347603401191, 1.362376457177303157 ) ) ;
#41139=CARTESIAN_POINT ( 'NONE',  ( -12.77186547895210467, 122.8260676081006153, 1.334005200199291252 ) ) ;
#41140=CARTESIAN_POINT ( 'NONE',  ( -0.9746272421432693456, 17.39786500698104277, 0.06925455797152506310 ) ) ;
#41141=CARTESIAN_POINT ( 'NONE',  ( 0.9750733387068674096, 18.20995955126885590, -0.03652159252302569076 ) ) ;
#41144=DIRECTION ( 'NONE',  ( -4.017660918040594346E-17, 1.000000000000000000, 2.376309959284832031E-19 ) ) ;
#41145=CARTESIAN_POINT ( 'NONE',  ( 0.9980778803427338142, 110.6314368487224300, 3.458106935563856066 ) ) ;
#41146=CARTESIAN_POINT ( 'NONE',  ( -9.968563030426437876, 123.7598584631124794, 0.7002966798862196862 ) ) ;
#41148=CARTESIAN_POINT ( 'NONE',  ( 2.953219771904812774, -14.51063682438745417, 4.500484459945554683 ) ) ;
#41149=CARTESIAN_POINT ( 'NONE',  ( 17.86368224974575369, 148.4245508482893854, -1.618106657999740072 ) ) ;
#41150=CARTESIAN_POINT ( 'NONE',  ( -19.41896158923250226, 149.6234262069624492, -2.479904253118717428 ) ) ;
#41152=CARTESIAN_POINT ( 'NONE',  ( -4.218275339060285845, 155.8585684991085714, -0.08429118021179402009 ) ) ;
#41153=CARTESIAN_POINT ( 'NONE',  ( 4.074910602682932925, 118.2429491485453354, -0.1454311599470142491 ) ) ;
#41154=CARTESIAN_POINT ( 'NONE',  ( 12.26386414673826053, 130.6044139104978115, -0.2969705276545479555 ) ) ;
#41155=ORIENTED_EDGE ( 'NONE', *, *, #34773, .F. ) ;
#41156=CARTESIAN_POINT ( 'NONE',  ( 2.849840736555561360, -14.15504780656048922, 0.1227973400909937313 ) ) ;
#41158=CARTESIAN_POINT ( 'NONE',  ( -3.890668369019033790, 28.55756886444902065, 1.917437575001416539 ) ) ;
#41159=B_SPLINE_CURVE_WITH_KNOTS ( 'NONE', 3,
 ( #35832, #6648, #3458, #38809, #9621, #32210, #6029, #35621, #6231, #16205, #39229 ),
 .UNSPECIFIED., .F., .F.,
 ( 4, 1, 1, 1, 1, 1, 1, 1, 4 ),
 ( 0.000000000000000000, 0.1249999999999979600, 0.2500000000000013878, 0.3749999999999938383, 0.4999999999999972800, 0.6249999999999980016, 0.7499999999999986677, 0.8749999999999993339, 1.000000000000000000 ),
 .UNSPECIFIED. ) ;
#41161=CARTESIAN_POINT ( 'NONE',  ( 2.901706292870370518, -4.507343114274551255, -3.632229383212865592 ) ) ;
#41162=CARTESIAN_POINT ( 'NONE',  ( 9.375340687752114377, 122.9055586947561522, 1.148039706409768490 ) ) ;
#41163=CARTESIAN_POINT ( 'NONE',  ( 2.866728174840395216, 37.98889525090484653, 1.397978221435859147 ) ) ;
#41164=CARTESIAN_POINT ( 'NONE',  ( -7.643874070029948342, 124.9344662015457317, -0.1527427953284559992 ) ) ;
#41165=CARTESIAN_POINT ( 'NONE',  ( 1.968029828064305153, -3.592386099649644837, 4.203610184747879508 ) ) ;
#41166=CARTESIAN_POINT ( 'NONE',  ( 9.049782359939477772, 124.0675141969884692, 0.1808361888366267212 ) ) ;
#41168=TOROIDAL_SURFACE ( 'NONE', #22772, 3.683000000000000718, 0.5080000000000000071 ) ;
#41169=CARTESIAN_POINT ( 'NONE',  ( -7.266063235143556120, -1.810023253287891487, -4.326994388187479501 ) ) ;
#41171=CARTESIAN_POINT ( 'NONE',  ( 2.154416292954056455, 116.4931154949332068, -0.2946284726465266401 ) ) ;
#41172=CARTESIAN_POINT ( 'NONE',  ( -0.3746108773303726824, 122.5569158606515003, -0.2627672029693575717 ) ) ;
#41175=CARTESIAN_POINT ( 'NONE',  ( -6.853500063829680577, -7.707324007402828414, -4.930749982112237362 ) ) ;
#41176=CARTESIAN_POINT ( 'NONE',  ( 0.07395884426403227796, 117.3993836134447690, 1.494938254265739896 ) ) ;
#41179=EDGE_CURVE ( 'NONE', #37741, #13569, #16128, .T. ) ;
#41180=CARTESIAN_POINT ( 'NONE',  ( 0.3798947725661321884, 120.3637084677653633, -0.5835535210198282696 ) ) ;
#41181=CARTESIAN_POINT ( 'NONE',  ( -20.50889283491270376, 152.5656283612522657, 0.2944088047499980876 ) ) ;
#41184=ORIENTED_EDGE ( 'NONE', *, *, #32111, .T. ) ;
#41186=CARTESIAN_POINT ( 'NONE',  ( -8.903120925483809955, 123.9008333197534029, -0.1338047255859078355 ) ) ;
#41187=CARTESIAN_POINT ( 'NONE',  ( 6.397261194921658678, -14.09295207620744961, -0.07176229933514734205 ) ) ;
#41188=CARTESIAN_POINT ( 'NONE',  ( -14.21869788239195032, 123.4894365733723447, 1.306911315328640910 ) ) ;
#41189=CARTESIAN_POINT ( 'NONE',  ( 7.640054841935559615, 158.5456267226934131, -0.8603666243017552562 ) ) ;
#41190=CARTESIAN_POINT ( 'NONE',  ( -0.1328416520900886078, 24.48205809745167372, 4.627450821846854190 ) ) ;
#41191=CARTESIAN_POINT ( 'NONE',  ( -10.73501234801834769, 157.9381345072164038, -0.5669044750022471657 ) ) ;
#41194=EDGE_LOOP ( 'NONE', ( #21510, #3867, #42094, #22508 ) ) ;
#41195=CARTESIAN_POINT ( 'NONE',  ( -5.562361497059077564, 116.7271819370821078, 0.05426658518331221870 ) ) ;
#41196=CARTESIAN_POINT ( 'NONE',  ( -6.640726327341849406E-14, 100.6774662015457409, -1.320564745697255449E-18 ) ) ;
#41198=CARTESIAN_POINT ( 'NONE',  ( -2.533752743582094347, 119.8406177399916714, 0.5716348071481811566 ) ) ;
#41200=CARTESIAN_POINT ( 'NONE',  ( 12.19007131875806493, 155.0146010091537221, -1.747022140133383195 ) ) ;
#41201=CARTESIAN_POINT ( 'NONE',  ( -20.99120442346859861, 145.7918284779248665, -2.367408383378773795 ) ) ;
#41203=CARTESIAN_POINT ( 'NONE',  ( 0.006077178772615180087, 120.4695998130595598, -0.3041268764237434197 ) ) ;
#41205=EDGE_CURVE ( 'NONE', #22781, #39868, #24286, .T. ) ;
#41207=CARTESIAN_POINT ( 'NONE',  ( -18.11471409803314359, 146.9188445454784357, -2.346026295494533009 ) ) ;
#41208=CARTESIAN_POINT ( 'NONE',  ( 4.228161069935173266, -15.38163066151135361, 0.6048619776675213666 ) ) ;
#41209=CARTESIAN_POINT ( 'NONE',  ( -4.255713500455158282, 118.2236181106063242, -0.4577248347117505167 ) ) ;
#41212=CARTESIAN_POINT ( 'NONE',  ( -4.801647862231239294, 117.4032733357421137, 1.015449305854420503 ) ) ;
#41213=CARTESIAN_POINT ( 'NONE',  ( 7.341258159293141183, 120.8389031223305352, 1.207285925005196825 ) ) ;
#41214=DIRECTION ( 'NONE',  ( -4.017660918040594346E-17, 1.000000000000000000, 2.376309959284834438E-19 ) ) ;
#41216=CARTESIAN_POINT ( 'NONE',  ( -6.147169039531121371, -7.901875862888119606, -5.777837204501876656 ) ) ;
#41217=CARTESIAN_POINT ( 'NONE',  ( 4.265939155584976383, 155.8374496918941077, 0.3214930909109447454 ) ) ;
#41221=CARTESIAN_POINT ( 'NONE',  ( -0.5465841182417748856, 117.9394513981711299, 1.387505131010090098 ) ) ;
#41223=CARTESIAN_POINT ( 'NONE',  ( -7.850986424014909204, 122.2449432668186660, -0.7695275123436272624 ) ) ;
#41226=CARTESIAN_POINT ( 'NONE',  ( -23.27479113596638527, 149.3390083238215595, -0.2346540593346968795 ) ) ;
#41229=CARTESIAN_POINT ( 'NONE',  ( 6.940171632852439210, 121.9095277527773220, -0.09994676863305257397 ) ) ;
#41230=CARTESIAN_POINT ( 'NONE',  ( -8.325883379001959739, 120.1130057568718144, 1.118334525995478224 ) ) ;
#41232=CARTESIAN_POINT ( 'NONE',  ( 1.114896128613473536, 115.7029400299447985, -1.703466781126056873 ) ) ;
#41233=CARTESIAN_POINT ( 'NONE',  ( -7.835359239711140233, 154.6110463214094182, -0.4315757689284724918 ) ) ;
#41234=CARTESIAN_POINT ( 'NONE',  ( 4.746351668907457189, -13.71804649124164222, 3.839566941389735977 ) ) ;
#41235=CARTESIAN_POINT ( 'NONE',  ( -21.87215423617524479, 148.4185114426368841, 1.275166548224079044 ) ) ;
#41236=CARTESIAN_POINT ( 'NONE',  ( -5.274544067074297793, 115.7029491485453718, 0.8135768287290677803 ) ) ;
#41237=CARTESIAN_POINT ( 'NONE',  ( 14.79880180360888708, 120.3086691715681695, 0.4511713404943136219 ) ) ;
#41238=CARTESIAN_POINT ( 'NONE',  ( 15.52687642492882070, 147.5330934759543879, 0.3102639428822866474 ) ) ;
#41240=CARTESIAN_POINT ( 'NONE',  ( 0.1081409728947390902, 20.38375149489202443, -0.9727671068919315767 ) ) ;
#41241=CARTESIAN_POINT ( 'NONE',  ( -16.14716650825978306, 121.2501203052637493, -0.3739013473229989559 ) ) ;
#41242=DIRECTION ( 'NONE',  ( -5.206863593109713661E-17, 1.000000000000000000, -1.077750396879097183E-30 ) ) ;
#41244=ORIENTED_EDGE ( 'NONE', *, *, #22149, .F. ) ;
#41245=CARTESIAN_POINT ( 'NONE',  ( -8.350588457312666080, 119.9924236745955994, 1.117253148572291188 ) ) ;
#41246=CARTESIAN_POINT ( 'NONE',  ( 3.517175496330608997, 50.63946620154572997, -1.199971990511068398 ) ) ;
#41247=CARTESIAN_POINT ( 'NONE',  ( 21.19565729220476058, 150.1117090729339623, 2.124842235463313855 ) ) ;
#41248=CARTESIAN_POINT ( 'NONE',  ( 14.21869788239182242, 123.4894365733723447, -1.306911315328640910 ) ) ;
#41249=CARTESIAN_POINT ( 'NONE',  ( 4.409325496788552456, -14.99073161069602911, -1.440227693534741782 ) ) ;
#41250=CARTESIAN_POINT ( 'NONE',  ( -22.33586214876087794, 148.6363688457942942, -1.892951199575521937 ) ) ;
#41251=CARTESIAN_POINT ( 'NONE',  ( 4.814721792459936367, 117.6728147345521336, -0.9185617900964898608 ) ) ;
#41252=CARTESIAN_POINT ( 'NONE',  ( 2.481140172163616153, 107.2306503360107541, 4.727365043318366489 ) ) ;
#41254=CARTESIAN_POINT ( 'NONE',  ( -15.79259660498981788, 146.2429432508320417, -0.1870566092231161215 ) ) ;
#41255=CARTESIAN_POINT ( 'NONE',  ( -17.42401203395167286, 135.4862447717955547, -2.417378365323842537 ) ) ;
#41256=CARTESIAN_POINT ( 'NONE',  ( 6.174787192795118784, -14.39888150296345160, 1.159817306988995211 ) ) ;
#41257=CARTESIAN_POINT ( 'NONE',  ( -6.442660433036017764, 29.32943145771791649, -0.01012415147099491285 ) ) ;
#41260=AXIS2_PLACEMENT_3D ( 'NONE', #20550, #23542, #3992 ) ;
#41262=CARTESIAN_POINT ( 'NONE',  ( 18.66896445097598445, 144.8948545501563103, 2.490227693099508421 ) ) ;
#41265=ADVANCED_FACE ( 'NONE', ( #31793 ), #77, .T. ) ;
#41267=CARTESIAN_POINT ( 'NONE',  ( -0.1065646865916159008, 105.8844662015456777, 5.332932678536313809 ) ) ;
#41269=CARTESIAN_POINT ( 'NONE',  ( 7.448509604456053701, -5.047432113992361025, -3.928768625439613693 ) ) ;
#41270=CARTESIAN_POINT ( 'NONE',  ( -0.004350076772803485731, 120.7058980590201429, 0.2176956299261764427 ) ) ;
#41271=CARTESIAN_POINT ( 'NONE',  ( -6.618965589514436111E-14, 97.88346620154572975, 1.207165459396359365E-19 ) ) ;
#41272=CARTESIAN_POINT ( 'NONE',  ( 11.41934419072014784, 118.9229013597968247, -0.3849275771520423439 ) ) ;
#41275=CARTESIAN_POINT ( 'NONE',  ( -8.797619116256065297, 117.6845724412130636, -0.1949819775001481181 ) ) ;
#41276=CARTESIAN_POINT ( 'NONE',  ( -5.078986093043185157, 66.64146620154573952, -0.1014902294541238092 ) ) ;
#41277=CARTESIAN_POINT ( 'NONE',  ( -4.269871265972513541, 118.2237297664921272, 0.2881146102117009833 ) ) ;
#41278=CARTESIAN_POINT ( 'NONE',  ( -22.76738278397264281, 137.3906169244638136, -0.4549464913834381230 ) ) ;
#41281=CARTESIAN_POINT ( 'NONE',  ( -8.272338380459794749, 120.1238670769245402, -1.449810942576005290 ) ) ;
#41282=CARTESIAN_POINT ( 'NONE',  ( -4.559649833866270541, 116.0444662015457169, -3.750543233647261498 ) ) ;
#41284=CARTESIAN_POINT ( 'NONE',  ( -6.480921187770144698, 121.5572409441427482, -0.5803991303062125962 ) ) ;
#41289=CARTESIAN_POINT ( 'NONE',  ( 4.537321141924904211, 26.63107350737006840, 0.8823464973398146283 ) ) ;
#41293=TOROIDAL_SURFACE ( 'NONE', #15422, 3.683000000000000718, 0.5080000000000000071 ) ;
#41295=CARTESIAN_POINT ( 'NONE',  ( -6.065156332796640015, 121.4250553548456963, 0.04358041984482485115 ) ) ;
#41296=CARTESIAN_POINT ( 'NONE',  ( -3.182929088426432074, 26.46582164074821009, -3.363547984189534379 ) ) ;
#41297=CARTESIAN_POINT ( 'NONE',  ( 16.30933243092136919, 122.7783120765077030, 1.207982166786797373 ) ) ;
#41299=CARTESIAN_POINT ( 'NONE',  ( 2.101618670382315646, -15.21789252882688182, 5.187277112784037136 ) ) ;
#41300=CARTESIAN_POINT ( 'NONE',  ( 21.59954917983685263, 148.3057046726078170, -1.384394358321686447 ) ) ;
#41301=CARTESIAN_POINT ( 'NONE',  ( -17.48755558824501932, 140.3598469681121514, 1.687825538285184779 ) ) ;
#41302=CARTESIAN_POINT ( 'NONE',  ( -0.8806307086779237014, 20.21867702141905099, 4.540528814573361771 ) ) ;
#41303=CARTESIAN_POINT ( 'NONE',  ( -22.58684024723483930, 150.0155710288180444, -1.417619447182237424 ) ) ;
#41304=CARTESIAN_POINT ( 'NONE',  ( -0.5928395319016861453, 6.288998576159460008, -0.7801151024821093571 ) ) ;
#41307=CARTESIAN_POINT ( 'NONE',  ( -15.78585801821222745, 147.2673792861271522, 0.2768292828507334935 ) ) ;
#41308=CARTESIAN_POINT ( 'NONE',  ( 5.728675787863017455, -12.92793046001887447, 1.911514839944304045 ) ) ;
#41309=CARTESIAN_POINT ( 'NONE',  ( 0.007600002268302612565, 120.2037396364829505, -0.3803351912374558497 ) ) ;
#41310=ORIENTED_EDGE ( 'NONE', *, *, #18348, .F. ) ;
#41311=CARTESIAN_POINT ( 'NONE',  ( 2.437877199975485798, 115.7029724319875044, 1.698779354361399596 ) ) ;
#41314=CARTESIAN_POINT ( 'NONE',  ( -4.811753004953239987, 117.8278766848995360, -0.8913836744279551860 ) ) ;
#41315=CARTESIAN_POINT ( 'NONE',  ( 15.72550100231850223, 145.6881679641610674, 0.3142329346387552902 ) ) ;
#41317=CARTESIAN_POINT ( 'NONE',  ( 16.37183938475173761, 128.5611466799914240, 2.176631273311136372 ) ) ;
#41318=CARTESIAN_POINT ( 'NONE',  ( 2.884051542275651414, 156.0957788938021054, 0.05763021347587640730 ) ) ;
#41321=EDGE_CURVE ( 'NONE', #40883, #20726, #35713, .T. ) ;
#41322=CARTESIAN_POINT ( 'NONE',  ( 0.006534791579796636780, 156.3267223255430167, -0.3270276925529294054 ) ) ;
#41324=CARTESIAN_POINT ( 'NONE',  ( 3.277668934457457883, 159.4655167044000166, -0.1355973003551878275 ) ) ;
#41328=CARTESIAN_POINT ( 'NONE',  ( 2.060994295209965355, -15.07716207348598658, 5.759911643239397527 ) ) ;
#41331=CARTESIAN_POINT ( 'NONE',  ( -4.804031589438218397, 117.8804387572236720, 0.6820340777931721554 ) ) ;
#41335=CARTESIAN_POINT ( 'NONE',  ( -8.556729359846826810, 118.7615713437664482, -1.197783989955824246 ) ) ;
#41336=CARTESIAN_POINT ( 'NONE',  ( -6.647360066588118066, 123.1390089711370166, -0.2039998645198904670 ) ) ;
#41337=CARTESIAN_POINT ( 'NONE',  ( 4.844883236810956006, 117.7536488614241819, 0.9521362604971945753 ) ) ;
#41338=CARTESIAN_POINT ( 'NONE',  ( 3.131015516031846690, -14.62848841321586946, 3.524024012273756501 ) ) ;
#41339=CARTESIAN_POINT ( 'NONE',  ( -0.7761819157718372608, 120.0979018405971175, 0.5779541898223676810 ) ) ;
#41341=CARTESIAN_POINT ( 'NONE',  ( 2.862861873098513588, -10.07698056833738320, -3.640125809621840069 ) ) ;
#41343=CARTESIAN_POINT ( 'NONE',  ( -5.586884702347497900, 130.0144662015457300, -0.1116392523995361624 ) ) ;
#41344=CARTESIAN_POINT ( 'NONE',  ( 3.187032726610941946, -14.26951854355915117, 4.096494115788091861 ) ) ;
#41345=CARTESIAN_POINT ( 'NONE',  ( 5.736215069875311379, 118.4654530710369329, -0.4324765805296820753 ) ) ;
#41346=CARTESIAN_POINT ( 'NONE',  ( -8.120140396194459598, 121.3802920439979118, -1.244985559442681078 ) ) ;
#41349=CARTESIAN_POINT ( 'NONE',  ( -0.7744676708938487142, 115.7029696127382579, 1.727560791094020720 ) ) ;
#41350=CARTESIAN_POINT ( 'NONE',  ( -3.234384296441582318, 11.31316835407710819, -3.315160845070126427 ) ) ;
#41351=CARTESIAN_POINT ( 'NONE',  ( 16.70755423740138568, 155.2649736186859570, 0.8698744534657081307 ) ) ;
#41352=ORIENTED_EDGE ( 'NONE', *, *, #15989, .F. ) ;
#41353=CARTESIAN_POINT ( 'NONE',  ( 1.939419507827386813, 104.6144662015435927, -4.972011625062160434 ) ) ;
#41354=CARTESIAN_POINT ( 'NONE',  ( 4.433333709997448580, -15.52846643035468688, 1.874498299855786421 ) ) ;
#41355=CARTESIAN_POINT ( 'NONE',  ( -12.45504352496370792, 122.8403290575659526, 1.325700600460794742 ) ) ;
#41356=CARTESIAN_POINT ( 'NONE',  ( -0.7739057699295280868, 27.87760190725158083, 0.5882008851359883383 ) ) ;
#41357=CARTESIAN_POINT ( 'NONE',  ( 0.3789452347801735566, 6.767153838948093636, 0.8990310622920915096 ) ) ;
#41360=CARTESIAN_POINT ( 'NONE',  ( -4.963705370159209984, 117.4628516566523047, -0.9731298996446248184 ) ) ;
#41361=CARTESIAN_POINT ( 'NONE',  ( 3.552294876605459173, 120.2162445758188056, 0.4839898749706283976 ) ) ;
#41362=CARTESIAN_POINT ( 'NONE',  ( -16.50777979357284408, 146.8700648836752691, 0.9466601202970256201 ) ) ;
#41363=CARTESIAN_POINT ( 'NONE',  ( -8.487687333566288572, 123.3253871723413368, -0.1696041924978711757 ) ) ;
#41364=CARTESIAN_POINT ( 'NONE',  ( 3.350179296191433398, -14.02378440268806159, 3.677192885962260682 ) ) ;
#41365=CARTESIAN_POINT ( 'NONE',  ( 0.9105297513473562532, 157.1001331247151143, -1.431354397858309646 ) ) ;
#41366=CARTESIAN_POINT ( 'NONE',  ( -19.54281269640877028, 149.4594839399872512, -2.484111515072796816 ) ) ;
#41367=CARTESIAN_POINT ( 'NONE',  ( 4.795219958910193370, 117.6022194698829679, -0.9837822912906766248 ) ) ;
#41368=CARTESIAN_POINT ( 'NONE',  ( 3.092642723064080279, -14.67800799544728285, 3.675123631970977911 ) ) ;
#41369=CARTESIAN_POINT ( 'NONE',  ( 4.074910602682932925, 118.2429491485453354, -0.1454311599470142491 ) ) ;
#41370=CARTESIAN_POINT ( 'NONE',  ( 10.49519746661477804, 153.0637448873655728, -0.1985316654307168194 ) ) ;
#41371=ORIENTED_EDGE ( 'NONE', *, *, #22807, .F. ) ;
#41372=CARTESIAN_POINT ( 'NONE',  ( 4.986952782468003775, 117.3993836136630904, 0.9005337760477702957 ) ) ;
#41375=CARTESIAN_POINT ( 'NONE',  ( 5.010381036134592847, 117.3993854210250447, 0.7490851615034684885 ) ) ;
#41377=CARTESIAN_POINT ( 'NONE',  ( 6.371402057089752269, 24.08812572624405135, -5.527521448792488634 ) ) ;
#41378=CARTESIAN_POINT ( 'NONE',  ( 3.522522545432599017, 120.3814187630814132, 0.6186928868410388471 ) ) ;
#41380=CARTESIAN_POINT ( 'NONE',  ( 16.27668397883899232, 121.4070763266325628, 0.2738251655545990149 ) ) ;
#41381=CARTESIAN_POINT ( 'NONE',  ( -5.461839458676769787, 117.5340897209903517, 0.6076615112082689452 ) ) ;
#41383=CARTESIAN_POINT ( 'NONE',  ( -2.395914033174281865, 1.367755174955888275, -3.957843245732672877 ) ) ;
#41384=CARTESIAN_POINT ( 'NONE',  ( 15.72385166996613570, 146.8976323831864477, 0.3141999770531622160 ) ) ;
#41385=CARTESIAN_POINT ( 'NONE',  ( 7.953355231451894269, -5.272462086923463076, -2.798479926915725891 ) ) ;
#41387=CARTESIAN_POINT ( 'NONE',  ( 2.156070218774666092, 116.4399559780022884, -0.2666908309453368542 ) ) ;
#41388=CARTESIAN_POINT ( 'NONE',  ( 0.1065646865915095692, 105.8844662015456919, -5.332932678536313809 ) ) ;
#41390=CARTESIAN_POINT ( 'NONE',  ( -0.2616981356411249848, 38.12352966651759090, 1.602708108658221553 ) ) ;
#41391=CARTESIAN_POINT ( 'NONE',  ( 5.678980076864418969, -10.27674996446047828, -6.244917620322217644 ) ) ;
#41392=CARTESIAN_POINT ( 'NONE',  ( 0.1786959197596161841, 117.9394491163083387, 1.410396274712311548 ) ) ;
#41394=CARTESIAN_POINT ( 'NONE',  ( 3.682264917456192777, 85.18346620154574111, 0.07358041635424013294 ) ) ;
#41395=CARTESIAN_POINT ( 'NONE',  ( 1.012635771704780252, 123.9312678891798640, -0.06995516121779309093 ) ) ;
#41396=CARTESIAN_POINT ( 'NONE',  ( -3.247806582137030773, 159.4494809562368971, 0.3030341850868441544 ) ) ;
#41397=VERTEX_POINT ( 'NONE', #19530 ) ;
#41401=CARTESIAN_POINT ( 'NONE',  ( -10.95295744368173985, 127.9616006207616152, -0.1130554581393018038 ) ) ;
#41402=CARTESIAN_POINT ( 'NONE',  ( 5.208953926857062378, -15.24612122244077561, 3.266433406317167165 ) ) ;
#41403=CARTESIAN_POINT ( 'NONE',  ( -20.59420924110326823, 148.8605967840894095, 1.615102827552612252 ) ) ;
#41404=CARTESIAN_POINT ( 'NONE',  ( 14.85424080674754244, 121.7713424311148032, -0.8456621969668064454 ) ) ;
#41405=CARTESIAN_POINT ( 'NONE',  ( -4.460028654926622593, 22.53297844546955631, 1.214995109042491528 ) ) ;
#41406=CARTESIAN_POINT ( 'NONE',  ( -20.61342602778661970, 152.5829384802601396, -0.8505107393516943004 ) ) ;
#41409=CARTESIAN_POINT ( 'NONE',  ( -0.0002200197270987085075, 124.8375573595198063, 0.01101068683960104017 ) ) ;
#41410=DIRECTION ( 'NONE',  ( -0.9998004120163609398, 0.000000000000000000, -0.01997839162482749689 ) ) ;
#41411=CARTESIAN_POINT ( 'NONE',  ( -13.59099248324878850, 128.5255724691869830, 1.296117023882649155 ) ) ;
#41414=CARTESIAN_POINT ( 'NONE',  ( 17.77426102521089035, 149.9241642446907292, -1.728420094174573096 ) ) ;
#41415=CARTESIAN_POINT ( 'NONE',  ( -19.90801791207606897, 136.1824594150436383, -2.220825683169745712 ) ) ;
#41417=CARTESIAN_POINT ( 'NONE',  ( 9.963230294258153208, 124.0638329749226330, -0.5989708749582570713 ) ) ;
#41418=ORIENTED_EDGE ( 'NONE', *, *, #4040, .F. ) ;
#41419=CARTESIAN_POINT ( 'NONE',  ( -17.72773402338109605, 148.0643276405518804, -2.286219595833943963 ) ) ;
#41420=CARTESIAN_POINT ( 'NONE',  ( 4.512298201359578265, -15.31825885905126228, -0.4677400858729020006 ) ) ;
#41424=CARTESIAN_POINT ( 'NONE',  ( -4.869895933236811025, 117.5471251575243912, 0.9485355776679378348 ) ) ;
#41425=CARTESIAN_POINT ( 'NONE',  ( 5.836546232834177061, 120.2771794157441008, 1.045480238269852702 ) ) ;
#41426=CARTESIAN_POINT ( 'NONE',  ( 2.912792906754999578, 38.59631781016217644, -1.173005823891349442 ) ) ;
#41427=CARTESIAN_POINT ( 'NONE',  ( -7.020956707233273697, 3.738713905105897517, 4.673168047251142099 ) ) ;
#41428=CARTESIAN_POINT ( 'NONE',  ( 8.617107517140063067, 123.3364012560002578, 0.3915851211929423648 ) ) ;
#41437=CARTESIAN_POINT ( 'NONE',  ( 3.160389755237984044, 118.7629491485453741, 1.175221893788974015 ) ) ;
#41438=DIRECTION ( 'NONE',  ( 4.017660918040594346E-17, -1.000000000000000000, -2.376309959284834438E-19 ) ) ;
#41440=CARTESIAN_POINT ( 'NONE',  ( -22.52215935351600251, 150.7865899205276321, -0.2217371156544977739 ) ) ;
#41443=CARTESIAN_POINT ( 'NONE',  ( 7.806368754331440840, 122.5465026837492672, -0.09257337652142975937 ) ) ;
#41445=EDGE_LOOP ( 'NONE', ( #30364, #14543 ) ) ;
#41446=CARTESIAN_POINT ( 'NONE',  ( 0.6753195804803343583, 115.7031287183464769, -1.734273028809747208 ) ) ;
#41447=CARTESIAN_POINT ( 'NONE',  ( -9.171413160121694830, 124.0935018032023436, -0.3437271393031030575 ) ) ;
#41448=CARTESIAN_POINT ( 'NONE',  ( 3.373230072307711325, -14.96631539557509427, 5.513067843180951222 ) ) ;
#41449=CARTESIAN_POINT ( 'NONE',  ( -0.4065252312485121977, 117.6538564835029206, 0.4930844833531826676 ) ) ;
#41450=CARTESIAN_POINT ( 'NONE',  ( -6.606344270946872901E-14, 95.34346620154573770, 1.014423412895214384E-29 ) ) ;
#41451=CARTESIAN_POINT ( 'NONE',  ( 3.748677658115056044, 116.6824454826851820, 0.2320358872840704023 ) ) ;
#41452=CARTESIAN_POINT ( 'NONE',  ( -0.001427378018337739293, 156.3034662015458593, 0.07143183283045266563 ) ) ;
#41453=CARTESIAN_POINT ( 'NONE',  ( -4.997976212577941446, 117.5941873918911256, 0.6211058249704617396 ) ) ;
#41454=CARTESIAN_POINT ( 'NONE',  ( 0.8051319862491574941, 7.640635046448309708, 0.5515409728216702501 ) ) ;
#41456=CARTESIAN_POINT ( 'NONE',  ( -0.2977815589729818080, 116.4565202671238069, -0.07303518451646368037 ) ) ;
#41460=CARTESIAN_POINT ( 'NONE',  ( -8.440481546668859636, 119.5496565118663028, 1.072135216671611380 ) ) ;
#41461=CARTESIAN_POINT ( 'NONE',  ( -1.404924415901314561, -12.60368214249519703, -4.422195601339041993 ) ) ;
#41462=CARTESIAN_POINT ( 'NONE',  ( -0.02615207601228607126, 159.0391464308674756, 1.308756824028193266 ) ) ;
#41463=CARTESIAN_POINT ( 'NONE',  ( 11.27973791692641470, 156.1341193432522800, -1.681596738997434670 ) ) ;
#41464=CARTESIAN_POINT ( 'NONE',  ( 3.793251108634954516, -14.54000584982637001, -2.652246991476435056 ) ) ;
#41465=CARTESIAN_POINT ( 'NONE',  ( -17.05973152613374211, 125.2153959547233910, -1.608365543201426551 ) ) ;
#41466=CARTESIAN_POINT ( 'NONE',  ( 4.782691188464728960, 117.8918938667789718, -0.7200855588195160806 ) ) ;
#41467=CARTESIAN_POINT ( 'NONE',  ( 5.148946675963925301, 115.4673366222922368, 1.510641186666999980 ) ) ;
#41468=CARTESIAN_POINT ( 'NONE',  ( -15.73072674608061483, 146.8994026175788008, -0.1860059585639195767 ) ) ;
#41469=CARTESIAN_POINT ( 'NONE',  ( -2.337245495867256828, 157.7073581658784178, -1.721377379916720907 ) ) ;
#41471=CARTESIAN_POINT ( 'NONE',  ( 5.218378134725943696, -15.03467804911627681, 3.623131781705042354 ) ) ;
#41475=CARTESIAN_POINT ( 'NONE',  ( -0.9713960331287118111, 118.1651005049585024, -0.8791694678672022922 ) ) ;
#41477=CARTESIAN_POINT ( 'NONE',  ( 18.07722773961200602, 140.6071502257508143, 2.476399831607924540 ) ) ;
#41480=CARTESIAN_POINT ( 'NONE',  ( -1.667199326422704297, 119.8612358676174949, 0.5251152081720656950 ) ) ;
#41481=CARTESIAN_POINT ( 'NONE',  ( 1.876134371277577761, -7.842104223405461205, 8.241158351834352302 ) ) ;
#41482=CARTESIAN_POINT ( 'NONE',  ( 9.255566420661640592, 123.6186430441458981, 0.7743267827205287945 ) ) ;
#41483=ADVANCED_FACE ( 'NONE', ( #39358 ), #33195, .T. ) ;
#41484=CARTESIAN_POINT ( 'NONE',  ( 18.27977197196852543, 154.1370782493726210, -0.5456809356757469365 ) ) ;
#41487=CARTESIAN_POINT ( 'NONE',  ( 5.562407744872654547, 116.6996333493932809, 0.1111501445372368169 ) ) ;
#41488=B_SPLINE_CURVE_WITH_KNOTS ( 'NONE', 3,
 ( #28907, #22496, #25508, #41922, #176, #38508, #13146, #42134, #28493, #25921, #38929, #38300, #5934 ),
 .UNSPECIFIED., .F., .F.,
 ( 4, 1, 1, 1, 1, 1, 1, 1, 1, 1, 4 ),
 ( 0.000000000000000000, 0.1250000000000002498, 0.2500000000000004996, 0.3750000000000000555, 0.4109712969816595729, 0.4999999999999996669, 0.6249999999999995559, 0.7500000000000001110, 0.8232913890944979496, 0.8750000000000001110, 1.000000000000000000 ),
 .UNSPECIFIED. ) ;
#41491=CARTESIAN_POINT ( 'NONE',  ( -23.36121599382910219, 148.8756354988261990, -0.4668126921608655722 ) ) ;
#41492=EDGE_LOOP ( 'NONE', ( #31044, #7336, #15196, #2437 ) ) ;
#41494=CARTESIAN_POINT ( 'NONE',  ( -4.406358471284682388, 119.5322704129101794, -0.9262837095330083148 ) ) ;
#41495=CARTESIAN_POINT ( 'NONE',  ( 4.530977940126489578, 116.0444662015457595, 3.792717828883179543 ) ) ;
#41496=CARTESIAN_POINT ( 'NONE',  ( -9.322631400391710343, 123.9819092696984910, -0.6064563484049504405 ) ) ;
#41497=CARTESIAN_POINT ( 'NONE',  ( 4.801338745261147345, 117.3993836135855275, -1.016148444996444189 ) ) ;
#41498=CARTESIAN_POINT ( 'NONE',  ( 23.36121599382897074, 148.8756354988261990, 0.4668126921608657942 ) ) ;
#41499=ORIENTED_EDGE ( 'NONE', *, *, #15449, .F. ) ;
#41500=CARTESIAN_POINT ( 'NONE',  ( 3.043391175932955495, 18.63480288530714191, -3.501419995799015528 ) ) ;
#41503=CARTESIAN_POINT ( 'NONE',  ( -4.801647862234980302, 117.4032733357427105, 1.015449305853463491 ) ) ;
#41506=CARTESIAN_POINT ( 'NONE',  ( 7.789195200054391144, 122.5918894314571759, 0.3010967474846231173 ) ) ;
#41508=CARTESIAN_POINT ( 'NONE',  ( 2.794707274389933715, 24.31675177525179876, -3.679445548267922916 ) ) ;
#41509=CARTESIAN_POINT ( 'NONE',  ( 22.77131365710826572, 149.1304179266472261, 1.534847161028223939 ) ) ;
#41511=CARTESIAN_POINT ( 'NONE',  ( 21.56827676951018091, 148.6087350971780836, -1.383610176320234864 ) ) ;
#41512=CARTESIAN_POINT ( 'NONE',  ( -11.50890483677805420, 122.9335272575421669, 1.234163556480095236 ) ) ;
#41513=CARTESIAN_POINT ( 'NONE',  ( 0.2779342515209439202, -14.33719732021959636, -0.9356842789569203012 ) ) ;
#41514=CARTESIAN_POINT ( 'NONE',  ( -19.64956762203127738, 128.7577553591919752, -1.229466013835583516 ) ) ;
#41516=CARTESIAN_POINT ( 'NONE',  ( 0.7587898337924254832, 1.856531735440085207, 0.6142162870750064174 ) ) ;
#41517=ORIENTED_EDGE ( 'NONE', *, *, #9429, .F. ) ;
#41519=CARTESIAN_POINT ( 'NONE',  ( -15.74292597311053044, 147.5983985311728759, 0.4089823612135941588 ) ) ;
#41520=CARTESIAN_POINT ( 'NONE',  ( 5.214050246812039546, -13.77884693253300696, 3.484500232556287269 ) ) ;
#41521=CARTESIAN_POINT ( 'NONE',  ( 10.16557698404459131, 154.1059161911440469, -1.245122368702753723 ) ) ;
#41525=CARTESIAN_POINT ( 'NONE',  ( -4.724244202807499349, 117.6625551699878827, -1.131988795082268240 ) ) ;
#41526=CARTESIAN_POINT ( 'NONE',  ( 2.836071964827284297, 121.0300505300837415, 0.05667146733340982373 ) ) ;
#41527=CIRCLE ( 'NONE', #6822, 0.5080000000000002292 ) ;
#41528=ORIENTED_EDGE ( 'NONE', *, *, #11578, .T. ) ;
#41529=CARTESIAN_POINT ( 'NONE',  ( 18.11894642568437774, 135.6759721228443425, 2.431264806327576800 ) ) ;
#41530=CARTESIAN_POINT ( 'NONE',  ( 9.104209967887914701, 153.9432936505793066, 0.1819237819739444872 ) ) ;
#41531=CARTESIAN_POINT ( 'NONE',  ( -6.503981220335420706E-14, 66.64146620154573952, -9.408573323119121831E-18 ) ) ;
#41532=CARTESIAN_POINT ( 'NONE',  ( 4.869448445130315051, 117.5470895026042086, -0.9486559672550266553 ) ) ;
#41533=CARTESIAN_POINT ( 'NONE',  ( 23.28378132671070944, 148.8247458934765461, 0.01018146431420876089 ) ) ;
#41534=CARTESIAN_POINT ( 'NONE',  ( 0.1036566276968575451, 106.2435128697216271, -5.187401519901567504 ) ) ;
#41537=VECTOR ( 'NONE', #10687, 1000.000000000000227 ) ;
#41538=CARTESIAN_POINT ( 'NONE',  ( 1.688396205330639610, -15.30713883100645667, 5.828064177876307816 ) ) ;
#41540=DIRECTION ( 'NONE',  ( 4.017660918040594346E-17, -1.000000000000000000, -2.376309959284834438E-19 ) ) ;
#41541=CARTESIAN_POINT ( 'NONE',  ( -4.567869538816805353, 118.0323994909192180, 0.6817792069717166781 ) ) ;
#41544=FACE_BOUND ( 'NONE', #26619, .T. ) ;
#41545=CARTESIAN_POINT ( 'NONE',  ( -5.949495757309211541, 119.2098673763693597, -1.265899271510292134 ) ) ;
#41546=CARTESIAN_POINT ( 'NONE',  ( -0.5964146925941966604, 106.0274289318137306, -5.278528196272315398 ) ) ;
#41547=AXIS2_PLACEMENT_3D ( 'NONE', #29463, #3498, #16457 ) ;
#41548=CARTESIAN_POINT ( 'NONE',  ( 4.723903736628679795, 117.9428513194235109, 0.8168244294066706601 ) ) ;
#41549=FACE_OUTER_BOUND ( 'NONE', #3095, .T. ) ;
#41550=CARTESIAN_POINT ( 'NONE',  ( -0.3884485718552637690, 122.8649044353670803, 0.2114733659581322922 ) ) ;
#41551=CARTESIAN_POINT ( 'NONE',  ( 4.560443952884764229, -11.68867000232777542, 0.6947937212093100445 ) ) ;
#41552=DIRECTION ( 'NONE',  ( 0.9998004120163608288, 0.000000000000000000, 0.01997839162482760791 ) ) ;
#41553=CARTESIAN_POINT ( 'NONE',  ( 5.078986093043053707, 91.53346620154573543, 0.1014902294541244060 ) ) ;
#41554=CARTESIAN_POINT ( 'NONE',  ( 6.805961295028007285, 123.7298400107579255, 0.09869924339446559114 ) ) ;
#41555=CARTESIAN_POINT ( 'NONE',  ( -17.19591734316819753, 148.1877419978735873, -2.150982665507991776 ) ) ;
#41557=CARTESIAN_POINT ( 'NONE',  ( -4.639629343391110439, 32.09505926734769332, 4.043355921567692413 ) ) ;
#41558=CARTESIAN_POINT ( 'NONE',  ( -2.240964803089219970, 115.7026167895974424, 1.621435518166598699 ) ) ;
#41559=CARTESIAN_POINT ( 'NONE',  ( -0.2480930319908794535, 10.21371511114847053, -4.635561276548324727 ) ) ;
#41560=CARTESIAN_POINT ( 'NONE',  ( 20.55326960831561678, 152.5775223076369400, 0.9856637426460335139 ) ) ;
#41562=CARTESIAN_POINT ( 'NONE',  ( -0.8083810056768732100, 105.1229538481459826, -5.283364377078966889 ) ) ;
#41563=CARTESIAN_POINT ( 'NONE',  ( 1.834459164715513291, -15.41678468052755413, 5.387059099755636460 ) ) ;
#41564=CARTESIAN_POINT ( 'NONE',  ( -18.94125265848544970, 149.4003703399637288, 1.737001818219200855 ) ) ;
#41565=CARTESIAN_POINT ( 'NONE',  ( 0.4978855121113271442, 23.66801414613304289, -0.8366695591092367934 ) ) ;
#41566=EDGE_CURVE ( 'NONE', #27127, #5804, #35231, .T. ) ;
#41567=CARTESIAN_POINT ( 'NONE',  ( -0.7518944845272079736, 4.819152178039351142, 0.6255420797857809134 ) ) ;
#41571=PLANE ( 'NONE',  #12665 ) ;
#41572=CARTESIAN_POINT ( 'NONE',  ( 2.616318351458453595, 112.7379566594982663, 2.676765618731040242 ) ) ;
#41573=CARTESIAN_POINT ( 'NONE',  ( -16.49265603038163519, 146.0252812507985141, 0.9509463687623793682 ) ) ;
#41574=CARTESIAN_POINT ( 'NONE',  ( -0.03519895178523997636, 115.7029491485446613, 1.761499482104069703 ) ) ;
#41575=CARTESIAN_POINT ( 'NONE',  ( 3.480220535011376182, -13.66934472092314046, 3.064489479733436106 ) ) ;
#41576=CARTESIAN_POINT ( 'NONE',  ( 15.94706863659606633, 135.0473088626721392, -1.554726643320764934 ) ) ;
#41577=CARTESIAN_POINT ( 'NONE',  ( -15.34515231418518155, 125.4902479783272184, -1.998699669873516438 ) ) ;
#41578=CARTESIAN_POINT ( 'NONE',  ( 4.610436209567292387, 117.9340757871244847, 0.9619774773656434297 ) ) ;
#41580=CARTESIAN_POINT ( 'NONE',  ( 8.314112694112955282, 119.9197418425491435, 1.454013855707701142 ) ) ;
#41581=CARTESIAN_POINT ( 'NONE',  ( -6.346781410994640993, 30.04503731349425166, 1.591420273447385014 ) ) ;
#41582=CARTESIAN_POINT ( 'NONE',  ( 15.46148294186153471, 147.8441550597069352, -0.1409636975754417765 ) ) ;
#41584=CARTESIAN_POINT ( 'NONE',  ( 3.116451998213339625, -14.00698646007624149, 1.619014592372306716 ) ) ;
#41585=CARTESIAN_POINT ( 'NONE',  ( -15.70103477329412911, 145.5797129992483292, -0.3137440411564564879 ) ) ;
#41587=CARTESIAN_POINT ( 'NONE',  ( 4.878198950886749152, 117.7629972649382069, 0.7300118938262585289 ) ) ;
#41589=CARTESIAN_POINT ( 'NONE',  ( -8.411989387141455055, 18.26859176889432490, 0.3690887223902433734 ) ) ;
#41590=CARTESIAN_POINT ( 'NONE',  ( 1.860601238663017298, 156.5995568990359175, 1.190227115183317697 ) ) ;
#41592=CARTESIAN_POINT ( 'NONE',  ( 18.84845417996773875, 125.3331924886369961, 0.3579177782036730981 ) ) ;
#41593=CARTESIAN_POINT ( 'NONE',  ( -7.117363349590201338, 122.4243137415680280, -0.03262055675632253432 ) ) ;
#41595=CARTESIAN_POINT ( 'NONE',  ( 15.38000172822621536, 147.8312228277220868, 0.3073290368998169431 ) ) ;
#41596=CARTESIAN_POINT ( 'NONE',  ( 0.09500447679424951775, 1.427469433126556053, 8.421719372511704549 ) ) ;
#41597=CARTESIAN_POINT ( 'NONE',  ( -5.492508718897443742, 117.1018086211233538, -0.7425764315396081727 ) ) ;
#41598=CARTESIAN_POINT ( 'NONE',  ( -0.3855071059148542090, 123.1683257372383054, -0.1933446952578522504 ) ) ;
#41602=CARTESIAN_POINT ( 'NONE',  ( -5.045332104996713696, -5.333490553104357268, 6.775881858851239947 ) ) ;
#41605=CARTESIAN_POINT ( 'NONE',  ( 3.221527947697278904, -14.19553219070161809, 2.775880300951635071 ) ) ;
#41606=CARTESIAN_POINT ( 'NONE',  ( 0.7593927098682741184, 117.6736730875354766, -1.153084249965024455 ) ) ;
#41607=CARTESIAN_POINT ( 'NONE',  ( -5.603706277412657144, 159.0849926622337023, 0.4754325247485732819 ) ) ;
#41608=ORIENTED_EDGE ( 'NONE', *, *, #27318, .T. ) ;
#41613=CARTESIAN_POINT ( 'NONE',  ( 4.434149479847604880, -15.45467793902401077, 4.427262213160148896 ) ) ;
#41614=CARTESIAN_POINT ( 'NONE',  ( -2.213227627077626547, 118.1205262787358663, 0.6644466414026561907 ) ) ;
#41615=CARTESIAN_POINT ( 'NONE',  ( 21.81261666999463955, 141.9756885651356413, -1.158660305423542702 ) ) ;
#41617=CARTESIAN_POINT ( 'NONE',  ( 2.801506786573456420, 9.139157206818806500, -3.684590140147142368 ) ) ;
#41620=CARTESIAN_POINT ( 'NONE',  ( -0.07831152689652476351, 109.4728569552520838, 3.919029035233729363 ) ) ;
#41621=DIRECTION ( 'NONE',  ( 4.017660918040594346E-17, -1.000000000000000000, -2.376309959284834438E-19 ) ) ;
#41622=CARTESIAN_POINT ( 'NONE',  ( -10.73673663838201264, 123.5542795626547417, 1.004701191943994765 ) ) ;
#41624=( BOUNDED_SURFACE ( )  B_SPLINE_SURFACE ( 3, 2, ( 
 ( #6631, #23201, #36236 ),
 ( #29192, #20023, #26211 ),
 ( #19596, #32607, #10024 ),
 ( #16835, #22995, #30248 ),
 ( #37075, #37273, #27479 ),
 ( #29836, #7894, #26851 ),
 ( #14057, #24267, #4084 ),
 ( #7266, #13643, #33464 ),
 ( #39642, #23636, #17460 ),
 ( #17256, #23851, #1090 ),
 ( #24060, #4499, #8093 ),
 ( #30042, #20855, #11282 ),
 ( #33676, #27267, #30665 ),
 ( #882, #30458, #33883 ),
 ( #13852, #27062, #14469 ),
 ( #39858, #4711, #21066 ),
 ( #40069, #10654, #1302 ),
 ( #36655, #17665, #7478 ),
 ( #40488, #1513, #4293 ),
 ( #34091, #4920, #20227 ) ),
 .UNSPECIFIED., .F., .F., .T. ) 
 B_SPLINE_SURFACE_WITH_KNOTS ( ( 4, 2, 2, 2, 2, 2, 2, 2, 2, 4 ),
 ( 3, 3 ),
 ( -3.230922474006803213E-17, 0.0008043537003517264297, 0.001608707400703485169, 0.002413061101055244233, 0.003217414801407002863, 0.004021768501758761494, 0.004826122202110520558, 0.006434829602814037819, 0.009652244404221074076, 0.01286965920562810860 ),
 ( 0.000000000000000000, 1.000000000000000000 ),
 .UNSPECIFIED. ) 
 GEOMETRIC_REPRESENTATION_ITEM ( )  RATIONAL_B_SPLINE_SURFACE ( (
 ( 1.000000000000000000, 0.9815197824473230748, 1.000000000000000000),
 ( 1.000000000000000000, 0.9811767838541908260, 1.000000000000000000),
 ( 1.000000000000000000, 0.9804039767750601930, 1.000000000000000000),
 ( 1.000000000000000000, 0.9775760511956556043, 1.000000000000000000),
 ( 1.000000000000000000, 0.9755247961213088237, 1.000000000000000000),
 ( 1.000000000000000000, 0.9705275854490454934, 1.000000000000000000),
 ( 1.000000000000000000, 0.9675790768636264305, 1.000000000000000000),
 ( 1.000000000000000000, 0.9611010073734985726, 1.000000000000000000),
 ( 1.000000000000000000, 0.9576315359772256119, 1.000000000000000000),
 ( 1.000000000000000000, 0.9503812888618250465, 1.000000000000000000),
 ( 1.000000000000000000, 0.9466096088173908685, 1.000000000000000000),
 ( 1.000000000000000000, 0.9387890754394591086, 1.000000000000000000),
 ( 1.000000000000000000, 0.9347210935279032240, 1.000000000000000000),
 ( 1.000000000000000000, 0.9222591698797557580, 1.000000000000000000),
 ( 1.000000000000000000, 0.9133676415885699784, 1.000000000000000000),
 ( 1.000000000000000000, 0.8858621071863931329, 1.000000000000000000),
 ( 1.000000000000000000, 0.8667308185392221809, 1.000000000000000000),
 ( 1.000000000000000000, 0.8330124393846976005, 1.000000000000000000),
 ( 1.000000000000000000, 0.8190729568369321534, 1.000000000000000000),
 ( 1.000000000000000000, 0.8123912451051846784, 1.000000000000000000) ) ) 
 REPRESENTATION_ITEM ( '' )  SURFACE ( )  );
#41625=CARTESIAN_POINT ( 'NONE',  ( 18.78841748004269974, 148.4604323410545987, -1.722921296925317147 ) ) ;
#41627=CARTESIAN_POINT ( 'NONE',  ( -20.57609261220312646, 150.0789294893613999, -2.287104906598478316 ) ) ;
#41629=CARTESIAN_POINT ( 'NONE',  ( 12.53742732955027606, 130.7145975665201831, -0.5304871790577961876 ) ) ;
#41631=CARTESIAN_POINT ( 'NONE',  ( -11.43271672892790569, 123.4929228318607386, -1.641276387634013068 ) ) ;
#41632=CARTESIAN_POINT ( 'NONE',  ( 3.879565938682602244, -15.27118588775909558, 0.8622231344456012803 ) ) ;
#41634=CARTESIAN_POINT ( 'NONE',  ( -4.065972646788793554, 118.2429491485453070, -0.3080848862740693250 ) ) ;
#41638=CARTESIAN_POINT ( 'NONE',  ( -4.924535406822394989, 117.6632503266924061, 0.7817655496803809223 ) ) ;
#41639=CARTESIAN_POINT ( 'NONE',  ( 17.82368987960353124, 147.7668373613703352, 2.290061161587757077 ) ) ;
#41641=CARTESIAN_POINT ( 'NONE',  ( -4.598301960400187127, 22.30806413504685537, 0.5496829067130363233 ) ) ;
#41642=CARTESIAN_POINT ( 'NONE',  ( -0.003550340867794020156, 156.3099534201614631, 0.1776735749810082476 ) ) ;
#41645=EDGE_LOOP ( 'NONE', ( #20660, #32382, #18042, #9431 ) ) ;
#41646=CARTESIAN_POINT ( 'NONE',  ( -0.1336288617286333358, 117.3993836134496433, 1.490790157883304712 ) ) ;
#41649=CARTESIAN_POINT ( 'NONE',  ( -8.744658474984799312, 117.8904183912612638, -0.6682122386599032016 ) ) ;
#41652=CARTESIAN_POINT ( 'NONE',  ( -13.61761151811294290, 119.6358206793323404, -0.1207630679856301070 ) ) ;
#41653=ORIENTED_EDGE ( 'NONE', *, *, #41697, .T. ) ;
#41655=CARTESIAN_POINT ( 'NONE',  ( -6.024938603336340570, 121.4387431788835983, -0.1605761971259225818 ) ) ;
#41658=CARTESIAN_POINT ( 'NONE',  ( 1.749836090240503017, 115.7029018622145600, -1.658193655284022183 ) ) ;
#41659=CARTESIAN_POINT ( 'NONE',  ( -4.248167858406196373, 155.8413357349917021, -0.2489887396171406586 ) ) ;
#41660=CARTESIAN_POINT ( 'NONE',  ( 2.071654280177509300, -15.34349575202162441, 5.977339193430266207 ) ) ;
#41661=CARTESIAN_POINT ( 'NONE',  ( -14.11223987312423311, 121.6707806233237363, 1.016201875498928153 ) ) ;
#41664=CARTESIAN_POINT ( 'NONE',  ( 23.37685013984155091, 146.7932648766621639, 0.8013420975766075705 ) ) ;
#41665=CARTESIAN_POINT ( 'NONE',  ( 3.788429304677606968, 121.0920094295889129, 0.1804846034801776133 ) ) ;
#41667=CARTESIAN_POINT ( 'NONE',  ( -0.9148265087109853644, 12.81245955126885505, -0.3394028602373861392 ) ) ;
#41668=CARTESIAN_POINT ( 'NONE',  ( -23.35646125964504094, 148.8716009884483071, -0.5438655406665984238 ) ) ;
#41670=CARTESIAN_POINT ( 'NONE',  ( -8.798071503382049130, 117.6842349159514640, -0.1758064068840608507 ) ) ;
#41672=CARTESIAN_POINT ( 'NONE',  ( 5.588576474492088941, 117.6380689354371185, 0.9556595479870083620 ) ) ;
#41674=CARTESIAN_POINT ( 'NONE',  ( 13.72986513748882764, 121.3979351292862816, 1.556522170903472890 ) ) ;
#41675=CARTESIAN_POINT ( 'NONE',  ( 3.234792161733059501, 118.6508749770327995, -0.7732002099368724402 ) ) ;
#41676=CARTESIAN_POINT ( 'NONE',  ( -5.788041011255496748, 9.848169244510268427, 6.116426545680356597 ) ) ;
#41677=CARTESIAN_POINT ( 'NONE',  ( 0.008308726997671040185, 117.3658353995175503, -0.4158026747930028688 ) ) ;
#41678=CARTESIAN_POINT ( 'NONE',  ( 4.639512378974469442, 117.9546344694811495, -0.7582059329740499232 ) ) ;
#41679=CARTESIAN_POINT ( 'NONE',  ( 2.934015389105384841, 107.8085536575111689, 4.480064466837520243 ) ) ;
#41680=AXIS2_PLACEMENT_3D ( 'NONE', #31565, #25389, #35192 ) ;
#41681=CARTESIAN_POINT ( 'NONE',  ( -2.899431565053971482, 156.0891579660883508, 0.02704053119243729833 ) ) ;
#41682=CARTESIAN_POINT ( 'NONE',  ( -18.41451321397408947, 140.7300538122508726, -2.503121031321716039 ) ) ;
#41683=CARTESIAN_POINT ( 'NONE',  ( 5.598737995799250911, -15.07077801197512201, 2.339151774602123979 ) ) ;
#41684=CARTESIAN_POINT ( 'NONE',  ( 5.240064600364064518, 115.6909491485453145, 1.019995478573027414 ) ) ;
#41685=CARTESIAN_POINT ( 'NONE',  ( -1.569852930085959608, 117.3993836557238239, -1.461717798063053797 ) ) ;
#41687=CARTESIAN_POINT ( 'NONE',  ( 18.62504088965185289, 146.9271955717142930, 2.448500584228244126 ) ) ;
#41690=CARTESIAN_POINT ( 'NONE',  ( -3.226952561781478934, 118.4615047536228047, 0.6622324852003674822 ) ) ;
#41691=CARTESIAN_POINT ( 'NONE',  ( 1.958624548881832350, -3.744965520567712147, -8.202033116754515518 ) ) ;
#41692=CARTESIAN_POINT ( 'NONE',  ( 15.56852431296066186, 143.6313904367523833, 1.174399326838564406 ) ) ;
#41693=CARTESIAN_POINT ( 'NONE',  ( 19.68299761936897596, 128.7577553591919752, -0.4435077540095086479 ) ) ;
#41697=EDGE_CURVE ( 'NONE', #31392, #450, #5978, .T. ) ;
#41698=CARTESIAN_POINT ( 'NONE',  ( -4.074955089416341991, 118.2429491485453497, 0.1454234154749720065 ) ) ;
#41699=AXIS2_PLACEMENT_3D ( 'NONE', #27218, #17203, #16989 ) ;
#41700=CARTESIAN_POINT ( 'NONE',  ( -21.90559427349704080, 151.4293160993575498, -0.4377259060014663805 ) ) ;
#41701=VERTEX_POINT ( 'NONE', #1024 ) ;
#41702=CARTESIAN_POINT ( 'NONE',  ( -4.749839897611219719, 119.8691466069420386, -0.9036556220809790485 ) ) ;
#41703=CARTESIAN_POINT ( 'NONE',  ( 6.003782516340518072, -14.18168619767446970, 2.149731705819561078 ) ) ;
#41704=CARTESIAN_POINT ( 'NONE',  ( -12.02994987064033161, 151.9703418938154584, -0.9209848757141018138 ) ) ;
#41706=CARTESIAN_POINT ( 'NONE',  ( 16.17518884899999421, 121.2571949256804089, 0.3403554851049458430 ) ) ;
#41709=CARTESIAN_POINT ( 'NONE',  ( -4.157303687089163979, 2.242350289152962528, -2.029258473605290103 ) ) ;
#41712=CYLINDRICAL_SURFACE ( 'NONE', #10864, 3.175000000000001155 ) ;
#41714=CARTESIAN_POINT ( 'NONE',  ( -6.104897796072584981, 120.8184930544039162, 0.6511854637274143709 ) ) ;
#41716=CARTESIAN_POINT ( 'NONE',  ( -0.01645572339174201579, 159.4324016994384010, 0.8235116888278194436 ) ) ;
#41717=CARTESIAN_POINT ( 'NONE',  ( 4.430104212713525058, 104.6144662015457527, -1.942668526382494543 ) ) ;
#41718=CARTESIAN_POINT ( 'NONE',  ( 2.829627719599027369, -13.65247383265987757, 0.5238048331051645690 ) ) ;
#41719=CARTESIAN_POINT ( 'NONE',  ( 1.228124343680933261, 158.9035955689636523, -1.375095950729813943 ) ) ;
#41721=CARTESIAN_POINT ( 'NONE',  ( -13.17493328878366299, 125.9194590699508893, 1.341157253524417170 ) ) ;
#41722=CARTESIAN_POINT ( 'NONE',  ( 4.382351430540762927, 4.226039240006542741, -1.512498627010908647 ) ) ;
#41723=CARTESIAN_POINT ( 'NONE',  ( -21.82912119472394252, 136.8312970274703844, -1.482621438090450106 ) ) ;
#41725=EDGE_CURVE ( 'NONE', #35651, #26787, #22933, .T. ) ;
#41727=CARTESIAN_POINT ( 'NONE',  ( -15.85992372348541579, 147.2950763206921181, 0.4080883723285145814 ) ) ;
#41728=CARTESIAN_POINT ( 'NONE',  ( 2.063686733023943898, -15.30319371230426384, 5.972472134935498111 ) ) ;
#41729=CARTESIAN_POINT ( 'NONE',  ( -5.008552712180506461, 117.3993836135855560, 0.7755994290793736257 ) ) ;
#41731=CARTESIAN_POINT ( 'NONE',  ( -4.586119793225739372, 118.0663795823288353, -0.7418019183852817555 ) ) ;
#41732=CARTESIAN_POINT ( 'NONE',  ( 14.67586190579446814, 148.8475317811793559, 0.2426438148417039697 ) ) ;
#41735=CARTESIAN_POINT ( 'NONE',  ( 12.85210230480885585, 122.5866728308148055, 1.831397601346916648 ) ) ;
#41739=CARTESIAN_POINT ( 'NONE',  ( -18.18789719519578441, 154.1160801429439857, 0.6523539814353516153 ) ) ;
#41741=CARTESIAN_POINT ( 'NONE',  ( 4.897476660045440688, 117.4787344905149098, -0.9609658134757302905 ) ) ;
#41742=CARTESIAN_POINT ( 'NONE',  ( 13.35275951139058215, 156.9675713949798421, -0.1105600748258539628 ) ) ;
#41743=EDGE_CURVE ( 'NONE', #13790, #6891, #36266, .T. ) ;
#41745=AXIS2_PLACEMENT_3D ( 'NONE', #40199, #13774, #7192 ) ;
#41748=CARTESIAN_POINT ( 'NONE',  ( 1.998290986358403076, -15.32462849664768889, 5.352800482084254519 ) ) ;
#41752=CARTESIAN_POINT ( 'NONE',  ( -4.634698098077384643, 118.0229612706176852, 0.6599311673777064069 ) ) ;
#41755=CARTESIAN_POINT ( 'NONE',  ( -0.9591419137607016809, 118.7629491485454025, -1.264665336164764176 ) ) ;
#41756=CARTESIAN_POINT ( 'NONE',  ( 8.418152194937446708, 119.6600584949201789, -1.087643031981900821 ) ) ;
#41757=CARTESIAN_POINT ( 'NONE',  ( -5.124638537096644519, 121.7269124416356192, -0.3048162158978747760 ) ) ;
#41758=CARTESIAN_POINT ( 'NONE',  ( 4.716237012333075462, 117.9479786380103832, 0.8297904974140549728 ) ) ;
#41759=CARTESIAN_POINT ( 'NONE',  ( 2.768561164044480272, -13.57843041371762460, 0.3119852368007841603 ) ) ;
#41760=CARTESIAN_POINT ( 'NONE',  ( -14.94238115049602555, 139.3652335140928074, -1.424457715676853420 ) ) ;
#41762=CARTESIAN_POINT ( 'NONE',  ( -3.234620543671446136, 115.7029687495403465, -1.652800550241499078 ) ) ;
#41765=CARTESIAN_POINT ( 'NONE',  ( 7.280302209287049742, 123.0424313102424492, 0.07662657258806362948 ) ) ;
#41766=CARTESIAN_POINT ( 'NONE',  ( -7.123980356064119945, 155.7895407640516510, -1.727872795330590128 ) ) ;
#41767=CARTESIAN_POINT ( 'NONE',  ( 23.42514220145532988, 142.8382549600662799, 0.4680900899251592140 ) ) ;
#41768=CARTESIAN_POINT ( 'NONE',  ( -5.495523183683927115, 31.57050297546189199, 3.325088329614593885 ) ) ;
#41769=CARTESIAN_POINT ( 'NONE',  ( -2.411564736306322398, 115.7029271828744328, 1.607687481377515049 ) ) ;
#41770=CARTESIAN_POINT ( 'NONE',  ( 0.7007450612751181529, 9.901275517365906609, -4.597291952374415125 ) ) ;
#41771=CARTESIAN_POINT ( 'NONE',  ( 18.41332411163117655, 154.1649927243852858, 1.048538238682171997 ) ) ;
#41773=CARTESIAN_POINT ( 'NONE',  ( 4.564577935816950038, 105.1216013620187937, -2.766951086067501731 ) ) ;
#41775=CARTESIAN_POINT ( 'NONE',  ( 3.037377538037926428, -15.29769487807139328, 4.066060606540134792 ) ) ;
#41776=CARTESIAN_POINT ( 'NONE',  ( -13.67124846526819404, 154.1626644387825991, 1.747499485815532383 ) ) ;
#41777=CARTESIAN_POINT ( 'NONE',  ( -0.9708255322354510941, 17.08399857615920325, -0.1324238259073569901 ) ) ;
#41778=CARTESIAN_POINT ( 'NONE',  ( 0.1248384507886338285, 1.166626901725996035, -0.9703616065359238485 ) ) ;
#41780=ORIENTED_EDGE ( 'NONE', *, *, #34161, .F. ) ;
#41782=CARTESIAN_POINT ( 'NONE',  ( 3.948369173669610266, 116.4303826247378026, 1.336099082351541956 ) ) ;
#41783=CARTESIAN_POINT ( 'NONE',  ( -11.42136869062017546, 126.1532465342912985, 0.7903108812046737430 ) ) ;
#41785=CARTESIAN_POINT ( 'NONE',  ( 3.507226199677831779, -13.17319675123219902, 2.199731216082013940 ) ) ;
#41786=CARTESIAN_POINT ( 'NONE',  ( 0.009931517865167266770, 119.6374844068871397, -0.4970137656763585210 ) ) ;
#41789=CARTESIAN_POINT ( 'NONE',  ( -18.11894642568450919, 135.6759721228443425, -2.431264806327576800 ) ) ;
#41791=CARTESIAN_POINT ( 'NONE',  ( 7.920580043951711779, 121.8826771451813613, 1.006826982956816163 ) ) ;
#41792=CARTESIAN_POINT ( 'NONE',  ( -4.834802360910630981, 32.27718159487177729, 0.9856153350916395661 ) ) ;
#41793=CARTESIAN_POINT ( 'NONE',  ( 0.002455802209136731355, 120.8958299794632438, -0.1228983847502213983 ) ) ;
#41797=EDGE_CURVE ( 'NONE', #9538, #9715, #6638, .T. ) ;
#41799=AXIS2_PLACEMENT_3D ( 'NONE', #2353, #25536, #38537 ) ;
#41800=CARTESIAN_POINT ( 'NONE',  ( 5.005814566362175810, 117.5914570300447224, -0.5468859341934453333 ) ) ;
#41801=CARTESIAN_POINT ( 'NONE',  ( -1.191460153279743750, 25.61543958765020434, -8.344265960924422743 ) ) ;
#41802=CARTESIAN_POINT ( 'NONE',  ( 8.439375761976323886, 122.5794309061019618, 0.8715591655942096505 ) ) ;
#41803=DIRECTION ( 'NONE',  ( 0.9998004120163608288, 0.000000000000000000, 0.01997839162482760791 ) ) ;
#41804=CARTESIAN_POINT ( 'NONE',  ( 23.34248308131507343, 149.0646716566344026, 0.3893018266236030200 ) ) ;
#41806=CARTESIAN_POINT ( 'NONE',  ( -5.755298473670496406, 118.4539739381501988, 0.4326931426192711094 ) ) ;
#41810=CARTESIAN_POINT ( 'NONE',  ( 9.163388821854780986, 124.2347608867413413, 0.1831063163140475014 ) ) ;
#41811=CARTESIAN_POINT ( 'NONE',  ( 4.854614700615579537, 158.3981005702974016, 1.674235554132198711 ) ) ;
#41812=CARTESIAN_POINT ( 'NONE',  ( 7.497756367663003019, 26.09243224653669913, 3.946719672664338319 ) ) ;
#41813=CARTESIAN_POINT ( 'NONE',  ( -2.155743978310675324, 116.6960643046747350, -0.4748305728995025898 ) ) ;
#41814=CARTESIAN_POINT ( 'NONE',  ( -1.051265659380997475, 124.5996987749017109, -0.05046802306060373805 ) ) ;
#41817=ADVANCED_FACE ( 'NONE', ( #31171 ), #40013, .T. ) ;
#41818=DIRECTION ( 'NONE',  ( 0.9998004120163610509, 4.016384292689131511E-17, 0.01997839162482749689 ) ) ;
#41819=CARTESIAN_POINT ( 'NONE',  ( -3.699395962244802050, 104.6144662015720144, 3.858360345332156882 ) ) ;
#41820=CARTESIAN_POINT ( 'NONE',  ( 3.655561289726139140, 27.93047918286777076, -2.829280713513928180 ) ) ;
#41822=CARTESIAN_POINT ( 'NONE',  ( -6.654617103318593247E-14, 104.6144662015457243, 1.534725424433578570E-31 ) ) ;
#41823=CARTESIAN_POINT ( 'NONE',  ( 3.075357915497110017, -13.94103813162880989, 1.416127232796946966 ) ) ;
#41824=CARTESIAN_POINT ( 'NONE',  ( 0.3780739950604312671, 121.2597428844643161, -0.4280417039577731342 ) ) ;
#41825=CARTESIAN_POINT ( 'NONE',  ( -0.005431400947739175623, 116.8580640273661118, 0.2718095133625909043 ) ) ;
#41830=CARTESIAN_POINT ( 'NONE',  ( 2.247313541653549240, -15.69307202063721718, 5.732350583303913893 ) ) ;
#41831=CARTESIAN_POINT ( 'NONE',  ( -1.201082828432692873, 118.2527139659984101, 0.6198154079389068816 ) ) ;
#41832=CARTESIAN_POINT ( 'NONE',  ( 1.297493386698500339, 159.2526592949493534, -1.079139715401668198 ) ) ;
#41833=CARTESIAN_POINT ( 'NONE',  ( -4.157303687089163979, 2.242350289152962528, -2.029258473605290103 ) ) ;
#41837=CARTESIAN_POINT ( 'NONE',  ( -0.01180776362034474322, 120.3637084677655764, 0.5909087754569243289 ) ) ;
#41838=( LENGTH_UNIT ( ) NAMED_UNIT ( * ) SI_UNIT ( .MILLI., .METRE. ) );
#41839=CARTESIAN_POINT ( 'NONE',  ( -17.26811951358317643, 148.1877419978735873, 1.462309189260816877 ) ) ;
#41841=CARTESIAN_POINT ( 'NONE',  ( 12.95103886519473768, 123.9867020804889961, -1.362965731555214832 ) ) ;
#41842=CARTESIAN_POINT ( 'NONE',  ( -1.137402291071538230, 117.9723128000925669, -0.6313431152059613138 ) ) ;
#41844=ORIENTED_EDGE ( 'NONE', *, *, #5898, .F. ) ;
#41845=CARTESIAN_POINT ( 'NONE',  ( 12.68314523066099575, 130.7634385742845780, -0.6346334167959435391 ) ) ;
#41847=CARTESIAN_POINT ( 'NONE',  ( -5.064401052258248548, 119.9665122172617231, -0.9903757029826917302 ) ) ;
#41848=CARTESIAN_POINT ( 'NONE',  ( 3.351832917607362461, -15.21525542808549503, 3.277475278119628133 ) ) ;
#41849=CARTESIAN_POINT ( 'NONE',  ( -5.586884702347495235, 66.64146620154573952, -0.1116392523995361763 ) ) ;
#41851=CARTESIAN_POINT ( 'NONE',  ( -4.755838299276228476, 117.7575533002713541, 0.8920572051838923100 ) ) ;
#41852=CARTESIAN_POINT ( 'NONE',  ( 1.368713796474816391, 119.6596719632383383, 0.6021288208518276175 ) ) ;
#41854=ADVANCED_FACE ( 'NONE', ( #9236 ), #24779, .T. ) ;
#41855=CARTESIAN_POINT ( 'NONE',  ( 1.141857472271699425, 24.90688314728939190, 4.478778191171412182 ) ) ;
#41856=CARTESIAN_POINT ( 'NONE',  ( 14.70702164887880770, 148.8393470518043955, 0.6194100056173929003 ) ) ;
#41866=CARTESIAN_POINT ( 'NONE',  ( -0.3092006194328519864, 116.5226405152084652, 0.1184213420814131668 ) ) ;
#41869=CARTESIAN_POINT ( 'NONE',  ( -6.930752631510202377, 121.9162265043544835, -0.3522179438235389370 ) ) ;
#41870=CARTESIAN_POINT ( 'NONE',  ( -5.586884702347496123, 81.62746620154572952, -0.1116392523995361624 ) ) ;
#41872=CARTESIAN_POINT ( 'NONE',  ( 2.568899511553136783, 115.7029491485453292, -1.594678113571031286 ) ) ;
#41873=CARTESIAN_POINT ( 'NONE',  ( -15.78659908163013093, 146.5797798787131399, -0.5456203974801296930 ) ) ;
#41874=CARTESIAN_POINT ( 'NONE',  ( 5.096701352355580639, -14.12304281641942083, 3.871056799387667002 ) ) ;
#41875=CARTESIAN_POINT ( 'NONE',  ( -7.150008447151775748, 158.1912585135832785, 1.373277972272069825 ) ) ;
#41877=CARTESIAN_POINT ( 'NONE',  ( 15.99642297876436459, 121.2237126890796191, 0.5535212332769011701 ) ) ;
#41878=CARTESIAN_POINT ( 'NONE',  ( 3.778529602317638680, 121.0927827002991819, 0.1453591938630250935 ) ) ;
#41880=CARTESIAN_POINT ( 'NONE',  ( -0.5393284202071846334, 5.265691905141185458, 0.8139242273222374591 ) ) ;
#41881=CARTESIAN_POINT ( 'NONE',  ( -0.3005257795023814071, 116.4832816433156069, -0.09989594597631674955 ) ) ;
#41885=STYLED_ITEM ( 'NONE', ( #1878 ), #38535 ) ;
#41886=CARTESIAN_POINT ( 'NONE',  ( -5.555942344568563840, 117.1561234432993643, 0.5128540820207154738 ) ) ;
#41887=EDGE_LOOP ( 'NONE', ( #20554, #1921, #41517, #7468 ) ) ;
#41889=CARTESIAN_POINT ( 'NONE',  ( 3.058686590879918565, 117.8293475852256904, 0.7841115193421155372 ) ) ;
#41890=CARTESIAN_POINT ( 'NONE',  ( 5.005942668485452884, 118.7197616721209670, -0.8869178833313972055 ) ) ;
#41891=CARTESIAN_POINT ( 'NONE',  ( 8.241158353334730791, 13.74789577914289929, -1.876134369653635448 ) ) ;
#41892=CARTESIAN_POINT ( 'NONE',  ( -12.60858107845361786, 120.1953580586475567, -1.309872962259287732 ) ) ;
#41893=CARTESIAN_POINT ( 'NONE',  ( 4.623501416330991987, 117.9757844860477718, -0.7388109444679361593 ) ) ;
#41894=CARTESIAN_POINT ( 'NONE',  ( 4.396974916608523465, 111.2411499886600268, 3.139452135551013434 ) ) ;
#41895=CARTESIAN_POINT ( 'NONE',  ( -15.38626016046121237, 147.8278496344100859, -0.1795882337043282206 ) ) ;
#41896=CARTESIAN_POINT ( 'NONE',  ( -18.29546242682556567, 149.1773161885088825, -2.457454238777247557 ) ) ;
#41897=CARTESIAN_POINT ( 'NONE',  ( 4.231574481101612051, -15.55479495760878095, 4.522910428756792278 ) ) ;
#41898=CARTESIAN_POINT ( 'NONE',  ( 4.973152232786927307, 117.3993868326352015, 0.9753084504214339923 ) ) ;
#41901=B_SPLINE_SURFACE_WITH_KNOTS ( 'NONE', 5, 5, ( 
 ( #23290, #36113, #33332, #3743, #3955, #548, #32698, #20517, #16916, #339, #29499, #39942 ),
 ( #4162, #33546, #26292, #26510, #39300, #36328, #10108, #10321, #7144, #23079, #965, #13934 ),
 ( #26930, #4504, #27067, #20234, #1309, #17882, #1520, #17048, #7900, #24275, #11083, #20444 ),
 ( #36452, #10660, #33260, #30884, #24070, #37279, #17671, #26856, #14265, #888, #4089, #1095 ),
 ( #14682, #14476, #1724, #33471, #27486, #11290, #39649, #10454, #37082, #20656, #7272, #27276 ),
 ( #40075, #7484, #10870, #40290, #30254, #21072, #13861, #17467, #4718, #23424, #7695, #30051 ),
 ( #33682, #39863, #20863, #23641, #30464, #8099, #14063, #23858, #36663, #33888, #34098, #30672 ),
 ( #40495, #4301, #4925, #36877, #17264, #41538, #34308, #11705, #34512, #38124, #31092, #37699 ),
 ( #27689, #1933, #24693, #5339, #8521, #41112, #25334, #21278, #12131, #8307, #37907, #18295 ),
 ( #11918, #31294, #12345, #11491, #22111, #5967, #24907, #5762, #37482, #38336, #8729, #2139 ),
 ( #21691, #18927, #5136, #34717, #24477, #28532, #18087, #28318, #21479, #14891, #8941, #9154 ),
 ( #31724, #31938, #31508, #27893, #40901, #35140, #5546, #15100, #28101, #18503, #2355, #15313 ),
 ( #2774, #41328, #2568, #40697, #25122, #21906, #34936, #18715, #15528, #12754, #38958, #41748 ),
 ( #6580, #7012, #9355, #9769, #3610, #13388, #29584, #41953, #22733, #3177, #38540, #19547 ),
 ( #19758, #35343, #26165, #418, #29364, #38749, #26375, #12549, #28935, #22317, #36192, #202 ) ),
 .UNSPECIFIED., .F., .F., .F.,
 ( 6, 3, 3, 3, 6 ),
 ( 6, 3, 3, 6 ),
 ( -0.3376510965135046116, -0.1035049821101841905, 0.07539719332481736869, 0.1467263880009520016, 0.3285558174568177781 ),
 ( -0.3370903632277621464, -0.1505698787908571201, 0.08591144153787821924, 0.3290542212108050757 ),
 .UNSPECIFIED. ) ;
#41902=CARTESIAN_POINT ( 'NONE',  ( -0.03212616895158381530, 157.6269964811067155, 1.607724863813389415 ) ) ;
#41903=DIRECTION ( 'NONE',  ( 0.9998004120163609398, 0.000000000000000000, 0.01997839162482749689 ) ) ;
#41905=CARTESIAN_POINT ( 'NONE',  ( -2.174325380064969337, 109.8863472468248119, 3.630110603364346655 ) ) ;
#41906=CARTESIAN_POINT ( 'NONE',  ( 3.722543281321895936, 25.13347685689727484, 7.580879713197038683 ) ) ;
#41907=CARTESIAN_POINT ( 'NONE',  ( 9.371428955827163065, 153.8930958044198576, 0.9350090023289894248 ) ) ;
#41909=CARTESIAN_POINT ( 'NONE',  ( 0.9959262657076558556, 116.9078805053781025, -0.3180477371503354633 ) ) ;
#41912=CARTESIAN_POINT ( 'NONE',  ( -0.8865878252963214079, 116.4323782974132513, -0.004867729696705670045 ) ) ;
#41914=CARTESIAN_POINT ( 'NONE',  ( -8.163272593483668516, 120.6601310837433374, -1.404696122763769761 ) ) ;
#41915=CARTESIAN_POINT ( 'NONE',  ( 4.691512992717155051, -14.98359649487970913, 4.483035719664550278 ) ) ;
#41916=CARTESIAN_POINT ( 'NONE',  ( -9.476112355320577052, 124.1929984354129175, -0.6154534730440988088 ) ) ;
#41918=CARTESIAN_POINT ( 'NONE',  ( 16.86202032626302483, 155.2029898760372646, 0.3369432954968345495 ) ) ;
#41919=EDGE_LOOP ( 'NONE', ( #11413, #1014, #7181, #4786 ) ) ;
#41920=CARTESIAN_POINT ( 'NONE',  ( 3.345514242732226418, 6.565394131763864216, 3.211428121085859733 ) ) ;
#41922=CARTESIAN_POINT ( 'NONE',  ( -18.63504953328976299, 154.1157618415863624, -0.3723726386282264489 ) ) ;
#41924=CARTESIAN_POINT ( 'NONE',  ( -5.586884702347497011, 117.3144662015457271, -0.1116392523995361624 ) ) ;
#41925=CARTESIAN_POINT ( 'NONE',  ( -6.999189161217031163, 121.8522563078195589, 0.1888263321353615132 ) ) ;
#41926=CARTESIAN_POINT ( 'NONE',  ( 2.245307460665866728, 11.68515688572553479, 4.070821060848484940 ) ) ;
#41927=CARTESIAN_POINT ( 'NONE',  ( 21.90872843939978409, 150.3855106993079005, 1.734217137259093322 ) ) ;
#41929=CARTESIAN_POINT ( 'NONE',  ( 4.575565686387192521, 113.7932280819714208, 2.209540002265822700 ) ) ;
#41930=CARTESIAN_POINT ( 'NONE',  ( 21.09608681602914615, 148.7375953542188256, -1.514114011542639249 ) ) ;
#41931=CARTESIAN_POINT ( 'NONE',  ( 3.547999066118234346, 14.38381850277834317, -2.990331240093012877 ) ) ;
#41932=CARTESIAN_POINT ( 'NONE',  ( -3.159869787290223719, 159.3937097445585778, -0.6918644357365442144 ) ) ;
#41936=CARTESIAN_POINT ( 'NONE',  ( -9.493134470504971389, 124.1929984354129175, 0.2364027771656556087 ) ) ;
#41938=CARTESIAN_POINT ( 'NONE',  ( 3.203739484688298500, -15.10556029324786032, 5.619401687775556375 ) ) ;
#41940=CARTESIAN_POINT ( 'NONE',  ( -4.627789221742965253, 118.0321741321441777, -0.7763224823049538204 ) ) ;
#41941=CARTESIAN_POINT ( 'NONE',  ( 15.21351360038791789, 143.4186079242267340, 0.3040022078858843346 ) ) ;
#41942=ORIENTED_EDGE ( 'NONE', *, *, #27222, .F. ) ;
#41943=CARTESIAN_POINT ( 'NONE',  ( 13.90099558903402510, 123.5874490550988014, 1.899532866591826741 ) ) ;
#41946=CARTESIAN_POINT ( 'NONE',  ( -21.34935411394468119, 151.2846570542378117, 0.7363345373129177585 ) ) ;
#41948=CARTESIAN_POINT ( 'NONE',  ( 4.997691741573370372, 117.4661756457942090, -0.7742298431118354030 ) ) ;
#41949=CARTESIAN_POINT ( 'NONE',  ( 0.004355829920537035785, 116.7171338949676738, -0.2179835409713598016 ) ) ;
#41950=CARTESIAN_POINT ( 'NONE',  ( -5.237832120027548832, 115.7029491485453860, -1.023639123012231034 ) ) ;
#41953=CARTESIAN_POINT ( 'NONE',  ( 1.790976758586900752, -15.16497236253652758, 5.485886819307857820 ) ) ;
#41956=CARTESIAN_POINT ( 'NONE',  ( -4.644072755505800565, 118.0368553417439443, 0.6066355437525197125 ) ) ;
#41957=CIRCLE ( 'NONE', #41260, 5.080000000000006288 ) ;
#41961=CARTESIAN_POINT ( 'NONE',  ( 8.410696399698803560, 119.6968806642600214, -1.092398566202036569 ) ) ;
#41962=CARTESIAN_POINT ( 'NONE',  ( -3.889650775106716196, 109.8300753404742096, -3.673692233826463482 ) ) ;
#41963=CARTESIAN_POINT ( 'NONE',  ( 4.648831033999298867, 117.8874912827738797, 1.000901579481272119 ) ) ;
#41964=CARTESIAN_POINT ( 'NONE',  ( 1.852819980464847305, -15.24972552306870455, 5.408883774200016425 ) ) ;
#41965=CARTESIAN_POINT ( 'NONE',  ( -16.19371004148921855, 147.7868695473139553, -1.594401216537396415 ) ) ;
#41966=CARTESIAN_POINT ( 'NONE',  ( -3.605926315104273971, 115.7029500413796228, -1.621950352474985868 ) ) ;
#41969=CARTESIAN_POINT ( 'NONE',  ( 2.162697817503714592, 106.7001829816230725, -4.879784414745867771 ) ) ;
#41970=CARTESIAN_POINT ( 'NONE',  ( -5.840731033150244222, 120.5744318282211651, -0.9509518217554207009 ) ) ;
#41972=CARTESIAN_POINT ( 'NONE',  ( -1.004127523102863684, 36.15709238714742924, 2.777694508738604906 ) ) ;
#41973=CARTESIAN_POINT ( 'NONE',  ( -2.338242410153924755, 115.7028053385901956, 1.613663431231236567 ) ) ;
#41974=CARTESIAN_POINT ( 'NONE',  ( -1.825063964020108065, -4.879331645356781877, 4.256838567046823840 ) ) ;
#41975=CARTESIAN_POINT ( 'NONE',  ( 13.27770485956316904, 119.7426348059052685, 0.8357656065649389232 ) ) ;
#41978=CARTESIAN_POINT ( 'NONE',  ( 3.302563718500166612, -15.23312206205887342, 3.441858572223985391 ) ) ;
#41979=CARTESIAN_POINT ( 'NONE',  ( -4.356286657365888715, 157.6046910967438066, 1.678189947947347216 ) ) ;
#41980=CARTESIAN_POINT ( 'NONE',  ( 0.6674325042100914818, 1.652014723813869823, 0.7093539244141242595 ) ) ;
#41982=CARTESIAN_POINT ( 'NONE',  ( 0.7576854961709549308, -2.078890728193560467, 0.6140693529290401909 ) ) ;
#41983=EDGE_CURVE ( 'NONE', #15637, #31392, #25694, .T. ) ;
#41987=CARTESIAN_POINT ( 'NONE',  ( 3.169910341315082647, 118.2446163226072713, 0.8422023655252532937 ) ) ;
#41988=CARTESIAN_POINT ( 'NONE',  ( -0.7532517793759884173, 156.4767055779393559, 0.8130599351363750893 ) ) ;
#41990=CARTESIAN_POINT ( 'NONE',  ( 4.309079644119920616, -12.27988108232860931, 1.651494482198018199 ) ) ;
#41991=CARTESIAN_POINT ( 'NONE',  ( 9.495682976374265394, 155.1592096034013366, -1.579384785498886945 ) ) ;
#41992=AXIS2_PLACEMENT_3D ( 'NONE', #20588, #32988, #39806 ) ;
#41993=CARTESIAN_POINT ( 'NONE',  ( -8.537619249161426893, 156.7723266660784986, -2.072230564756332161 ) ) ;
#41995=CARTESIAN_POINT ( 'NONE',  ( 1.979187190576821465, -15.21425526833739639, 5.301287498526151332 ) ) ;
#41996=CARTESIAN_POINT ( 'NONE',  ( -4.968091682766383244, 32.48584459999275253, 1.440197358048235010 ) ) ;
#41997=CARTESIAN_POINT ( 'NONE',  ( 6.492420186392267922, 121.7431354732680973, -0.05225946255319164485 ) ) ;
#42000=CARTESIAN_POINT ( 'NONE',  ( -3.009276887026423264, 50.13146620154573441, 1.210121013456480377 ) ) ;
#42001=DIRECTION ( 'NONE',  ( 5.206863593109713661E-17, -1.000000000000000000, 1.077750396879097183E-30 ) ) ;
#42002=CARTESIAN_POINT ( 'NONE',  ( -4.581648513977574666, 27.87760232565343088, 0.5121129833925254227 ) ) ;
#42003=CARTESIAN_POINT ( 'NONE',  ( 6.495892026627585913, 121.2869106855140018, 0.7936256953933333858 ) ) ;
#42005=CARTESIAN_POINT ( 'NONE',  ( 0.0002734175338629627090, 159.6054662015457382, -0.01368293144939973158 ) ) ;
#42006=CARTESIAN_POINT ( 'NONE',  ( -4.518882305193469229, 111.2411499886600268, 2.961292089698490226 ) ) ;
#42007=VECTOR ( 'NONE', #29869, 1000.000000000000000 ) ;
#42008=CARTESIAN_POINT ( 'NONE',  ( -6.538677740023618411E-14, 75.27746620154573520, -7.356392042280733227E-18 ) ) ;
#42009=CARTESIAN_POINT ( 'NONE',  ( 4.560281875334545099, -11.68902278883368595, 0.6958564903332965512 ) ) ;
#42010=CARTESIAN_POINT ( 'NONE',  ( -2.834545168019937389, 33.34007952871795766, 0.9740110680454012737 ) ) ;
#42012=CARTESIAN_POINT ( 'NONE',  ( 13.83539046132045414, 122.2371923977168109, 1.727333621972642064 ) ) ;
#42013=CARTESIAN_POINT ( 'NONE',  ( -2.961220487682185709, 16.77021669962341477, -3.573240411402743621 ) ) ;
#42014=CARTESIAN_POINT ( 'NONE',  ( 8.348643983786249834, 26.63118458923209175, 1.112826146890550483 ) ) ;
#42015=CARTESIAN_POINT ( 'NONE',  ( 8.747260340425302871, 117.9889815745654715, -0.4087459456760704213 ) ) ;
#42016=CARTESIAN_POINT ( 'NONE',  ( -1.574582893473529532, 118.9836165220538504, -0.7747311016372977477 ) ) ;
#42019=CARTESIAN_POINT ( 'NONE',  ( -1.777383475896760157, 104.6144662015478985, 5.032164064983053464 ) ) ;
#42020=CARTESIAN_POINT ( 'NONE',  ( -3.854280124997887746, 21.23357344512866973, -2.551540157904111261 ) ) ;
#42023=CARTESIAN_POINT ( 'NONE',  ( 3.176652145978316355, -13.92691374863060183, 2.072386176210903486 ) ) ;
#42024=CARTESIAN_POINT ( 'NONE',  ( 1.389742127967388718, 109.2701902778323557, -3.915166117862841411 ) ) ;
#42025=CARTESIAN_POINT ( 'NONE',  ( -23.09710566998045067, 146.6371693212631158, 0.4017528712124326384 ) ) ;
#42033=CARTESIAN_POINT ( 'NONE',  ( 5.755466747078162193, -14.97439463182292840, 1.832642420680269613 ) ) ;
#42034=CARTESIAN_POINT ( 'NONE',  ( -13.21705611421152149, 122.1656469061080514, 1.250183119358982742 ) ) ;
#42035=CARTESIAN_POINT ( 'NONE',  ( 3.977532531966649465, 117.6225627337916393, -0.6337845664926935463 ) ) ;
#42036=CARTESIAN_POINT ( 'NONE',  ( 4.219463811995017188, -1.205994944679912306, -1.932895124392335573 ) ) ;
#42040=CARTESIAN_POINT ( 'NONE',  ( -0.09934209769104777876, 106.7790779034713324, 4.971484795507142174 ) ) ;
#42041=CARTESIAN_POINT ( 'NONE',  ( -4.792200577477630397, 117.5371802918334225, 0.9878184568134641408 ) ) ;
#42042=CARTESIAN_POINT ( 'NONE',  ( -9.186197600956550247, 155.0058477609193801, 1.458900829815476197 ) ) ;
#42045=CARTESIAN_POINT ( 'NONE',  ( 9.549337214233879934, 121.2752502669211339, -1.156350410895870207 ) ) ;
#42046=CARTESIAN_POINT ( 'NONE',  ( -20.38236371569470506, 141.4490678312372722, -2.395676066357400824 ) ) ;
#42049=EDGE_CURVE ( 'NONE', #13325, #11900, #32601, .T. ) ;
#42051=CARTESIAN_POINT ( 'NONE',  ( 4.421201411745116161, 118.1651805457867539, -0.4751133233741948736 ) ) ;
#42052=CARTESIAN_POINT ( 'NONE',  ( 3.102522256439363080, 156.1450793681712241, -0.6153187215006972188 ) ) ;
#42053=ORIENTED_EDGE ( 'NONE', *, *, #5898, .T. ) ;
#42054=CARTESIAN_POINT ( 'NONE',  ( -1.387234972287347379, 119.7856413326322667, -0.5781392410077788035 ) ) ;
#42055=CARTESIAN_POINT ( 'NONE',  ( 3.434117431421463973, -14.91634622600368587, 0.6670077989445850619 ) ) ;
#42059=CARTESIAN_POINT ( 'NONE',  ( -4.949223898456546422, 117.6231127316777645, 0.7510713373028163886 ) ) ;
#42060=CARTESIAN_POINT ( 'NONE',  ( 17.31991401741507630, 147.8988302317391117, 2.155506138210265821 ) ) ;
#42061=CARTESIAN_POINT ( 'NONE',  ( -2.317791448294674872, 31.60761946039689008, 1.124105164688197211 ) ) ;
#42062=CARTESIAN_POINT ( 'NONE',  ( 0.2927481059715184020, -9.205330264445118260, -8.420370646799414160 ) ) ;
#42063=CARTESIAN_POINT ( 'NONE',  ( 13.60737276370606885, 150.2179846313823930, 0.4949411041190266980 ) ) ;
#42071=DIRECTION ( 'NONE',  ( -0.9998004120163609398, -4.016384292689130894E-17, -0.01997839162482749689 ) ) ;
#42074=EDGE_CURVE ( 'NONE', #16433, #1232, #10707, .T. ) ;
#42076=CARTESIAN_POINT ( 'NONE',  ( -6.916478980584567005, 117.2343425291504104, 0.1085122952249095302 ) ) ;
#42077=EDGE_CURVE ( 'NONE', #17780, #24610, #28411, .T. ) ;
#42080=CARTESIAN_POINT ( 'NONE',  ( -6.942438739474686926, 121.9314933722027234, -0.3079128108755967430 ) ) ;
#42082=CARTESIAN_POINT ( 'NONE',  ( 2.676737444774203833, 115.7033390179947787, -1.585144796910018306 ) ) ;
#42083=CARTESIAN_POINT ( 'NONE',  ( -11.89867495700692857, 130.3805625696445816, -0.3456363086864548961 ) ) ;
#42084=CARTESIAN_POINT ( 'NONE',  ( 5.208971126070756519, -14.02307540452116186, 3.677211492609324228 ) ) ;
#42085=CARTESIAN_POINT ( 'NONE',  ( -21.50873886539585556, 148.9071063441643048, 1.383230070950766999 ) ) ;
#42087=CARTESIAN_POINT ( 'NONE',  ( 4.752142575032201499, 116.8068435238802465, 0.2604826270010439093 ) ) ;
#42088=CARTESIAN_POINT ( 'NONE',  ( 4.619048842463770121, 121.2009516319313178, 0.1635582688743358881 ) ) ;
#42090=CARTESIAN_POINT ( 'NONE',  ( 0.3213417908193094141, 16.26526798020547204, 0.9222100932699727194 ) ) ;
#42091=CARTESIAN_POINT ( 'NONE',  ( -22.97436839085991878, 150.1579452496398801, -0.6125673049107096535 ) ) ;
#42094=ORIENTED_EDGE ( 'NONE', *, *, #10470, .F. ) ;
#42095=CARTESIAN_POINT ( 'NONE',  ( 8.629495036404707164, 118.4212787258601338, 1.048420227482702582 ) ) ;
#42098=CARTESIAN_POINT ( 'NONE',  ( 15.52234330115196137, 154.9569273371780298, 1.915578030012927258 ) ) ;
#42099=CARTESIAN_POINT ( 'NONE',  ( 2.272333812996608415, 118.4336326928681729, -0.6977090181727382268 ) ) ;
#42100=CARTESIAN_POINT ( 'NONE',  ( -7.544985805786585509, 7.895591250050960852, -3.771097921825450783 ) ) ;
#42102=CARTESIAN_POINT ( 'NONE',  ( -15.52234330115209104, 154.9569273371780298, -1.915578030012927258 ) ) ;
#42103=CARTESIAN_POINT ( 'NONE',  ( 4.645634966785371134, 117.9566108303512095, -0.7541813577493102771 ) ) ;
#42105=CARTESIAN_POINT ( 'NONE',  ( 5.045732318125604188, 114.3381464724725447, 1.964647476694348471 ) ) ;
#42106=CARTESIAN_POINT ( 'NONE',  ( -15.77260762454802467, 146.5697412905949477, -0.2637713227210858324 ) ) ;
#42107=CARTESIAN_POINT ( 'NONE',  ( -11.42611330002560877, 154.6851215890897038, -2.167138196937119066 ) ) ;
#42108=CARTESIAN_POINT ( 'NONE',  ( 5.007622726684139991, -15.39085649315211057, 3.402342850907996041 ) ) ;
#42111=ORIENTED_EDGE ( 'NONE', *, *, #24028, .T. ) ;
#42112=CARTESIAN_POINT ( 'NONE',  ( 6.601024023181092382, 120.1594786313440011, 1.214938174674062843 ) ) ;
#42113=CARTESIAN_POINT ( 'NONE',  ( -15.72385166996626715, 146.8976323831864477, -0.3141999770531619940 ) ) ;
#42117=CARTESIAN_POINT ( 'NONE',  ( -4.831936455160952271, 120.7138498849978987, 0.2122769985084471123 ) ) ;
#42118=CARTESIAN_POINT ( 'NONE',  ( 5.478597439045088890, 28.15663318097115209, -6.435035585623773535 ) ) ;
#42119=CARTESIAN_POINT ( 'NONE',  ( 16.06762827093114154, 146.3760696504137684, 1.175121962453930857 ) ) ;
#42120=CARTESIAN_POINT ( 'NONE',  ( 15.21238092238748507, 121.1469641333237917, -0.4626880538419668731 ) ) ;
#42122=CARTESIAN_POINT ( 'NONE',  ( 4.581716828367337513, -15.30239761468843973, -0.5121115983836379559 ) ) ;
#42123=CARTESIAN_POINT ( 'NONE',  ( -17.29948542670054223, 122.7677429521249053, -0.3279718759250787041 ) ) ;
#42124=ORIENTED_EDGE ( 'NONE', *, *, #17305, .T. ) ;
#42125=CARTESIAN_POINT ( 'NONE',  ( -4.985608112044036311, 120.1171868300749281, -0.8736999896306448798 ) ) ;
#42126=DIRECTION ( 'NONE',  ( 4.017660918040594346E-17, -1.000000000000000000, -2.376309959284834438E-19 ) ) ;
#42127=CARTESIAN_POINT ( 'NONE',  ( -13.34275001191909205, 134.1388935151753401, -0.9731691531512424165 ) ) ;
#42128=CARTESIAN_POINT ( 'NONE',  ( 4.309079644119920616, -12.27988108232860931, 1.651494482198018199 ) ) ;
#42130=CARTESIAN_POINT ( 'NONE',  ( 20.50094783971091772, 129.0975500345852822, 0.4299227524276376111 ) ) ;
#42132=CARTESIAN_POINT ( 'NONE',  ( -3.640175008984333882, 11.51306413504884318, -2.862805987297033727 ) ) ;
#42133=CARTESIAN_POINT ( 'NONE',  ( -3.013063373304370796, 105.1243314539317453, 4.412133481903750543 ) ) ;
#42134=CARTESIAN_POINT ( 'NONE',  ( -10.83330528665015891, 157.8980211815716928, -0.2164752214609687586 ) ) ;
#42136=LINE ( 'NONE', #41924, #466 ) ;
#42137=CARTESIAN_POINT ( 'NONE',  ( -7.829604799548672389, 122.4485675125339839, 0.2503763010704491143 ) ) ;
#42139=CARTESIAN_POINT ( 'NONE',  ( 3.490194016315742331, 12.22236127277748174, 3.029891289224248219 ) ) ;
#42140=CARTESIAN_POINT ( 'NONE',  ( 12.91997107708620263, 119.9671592456446803, 1.126112081325366665 ) ) ;
#42144=CARTESIAN_POINT ( 'NONE',  ( 0.01023305610364113119, 117.8848902025789158, -0.5121039721716187376 ) ) ;
#42145=CARTESIAN_POINT ( 'NONE',  ( -4.623654898565560778, 8.549082320728111029, 0.09932813335659773646 ) ) ;
#42146=CARTESIAN_POINT ( 'NONE',  ( -0.3408176794666137877, 116.9919054422455531, -0.3412737040790791432 ) ) ;
#42148=CARTESIAN_POINT ( 'NONE',  ( -5.269990328701569915, 121.3020066425206807, 0.06069006697729623090 ) ) ;
#42149=CARTESIAN_POINT ( 'NONE',  ( 5.341071565670632459, -14.32387631201759248, 3.633538872802142716 ) ) ;
#42151=ORIENTED_EDGE ( 'NONE', *, *, #1982, .T. ) ;
#42152=CARTESIAN_POINT ( 'NONE',  ( 17.05522983032404483, 131.5760549582342094, 2.311017189013932605 ) ) ;
#42154=CARTESIAN_POINT ( 'NONE',  ( -5.526300601521442424, 159.0395019988757781, 0.6540312330581289357 ) ) ;
#42155=CIRCLE ( 'NONE', #21723, 5.334000000000001407 ) ;
#42156=CARTESIAN_POINT ( 'NONE',  ( 0.006534887713546109859, 159.5822087645323393, -0.3270325034788579277 ) ) ;
#42158=CARTESIAN_POINT ( 'NONE',  ( -6.583861033951825950E-14, 91.02546620154572565, 1.480257718193877056E-29 ) ) ;
#42161=CARTESIAN_POINT ( 'NONE',  ( 8.399484405886864735, 119.7521803362377568, -1.098797162006715844 ) ) ;
ENDSEC;
END-ISO-10303-21;
